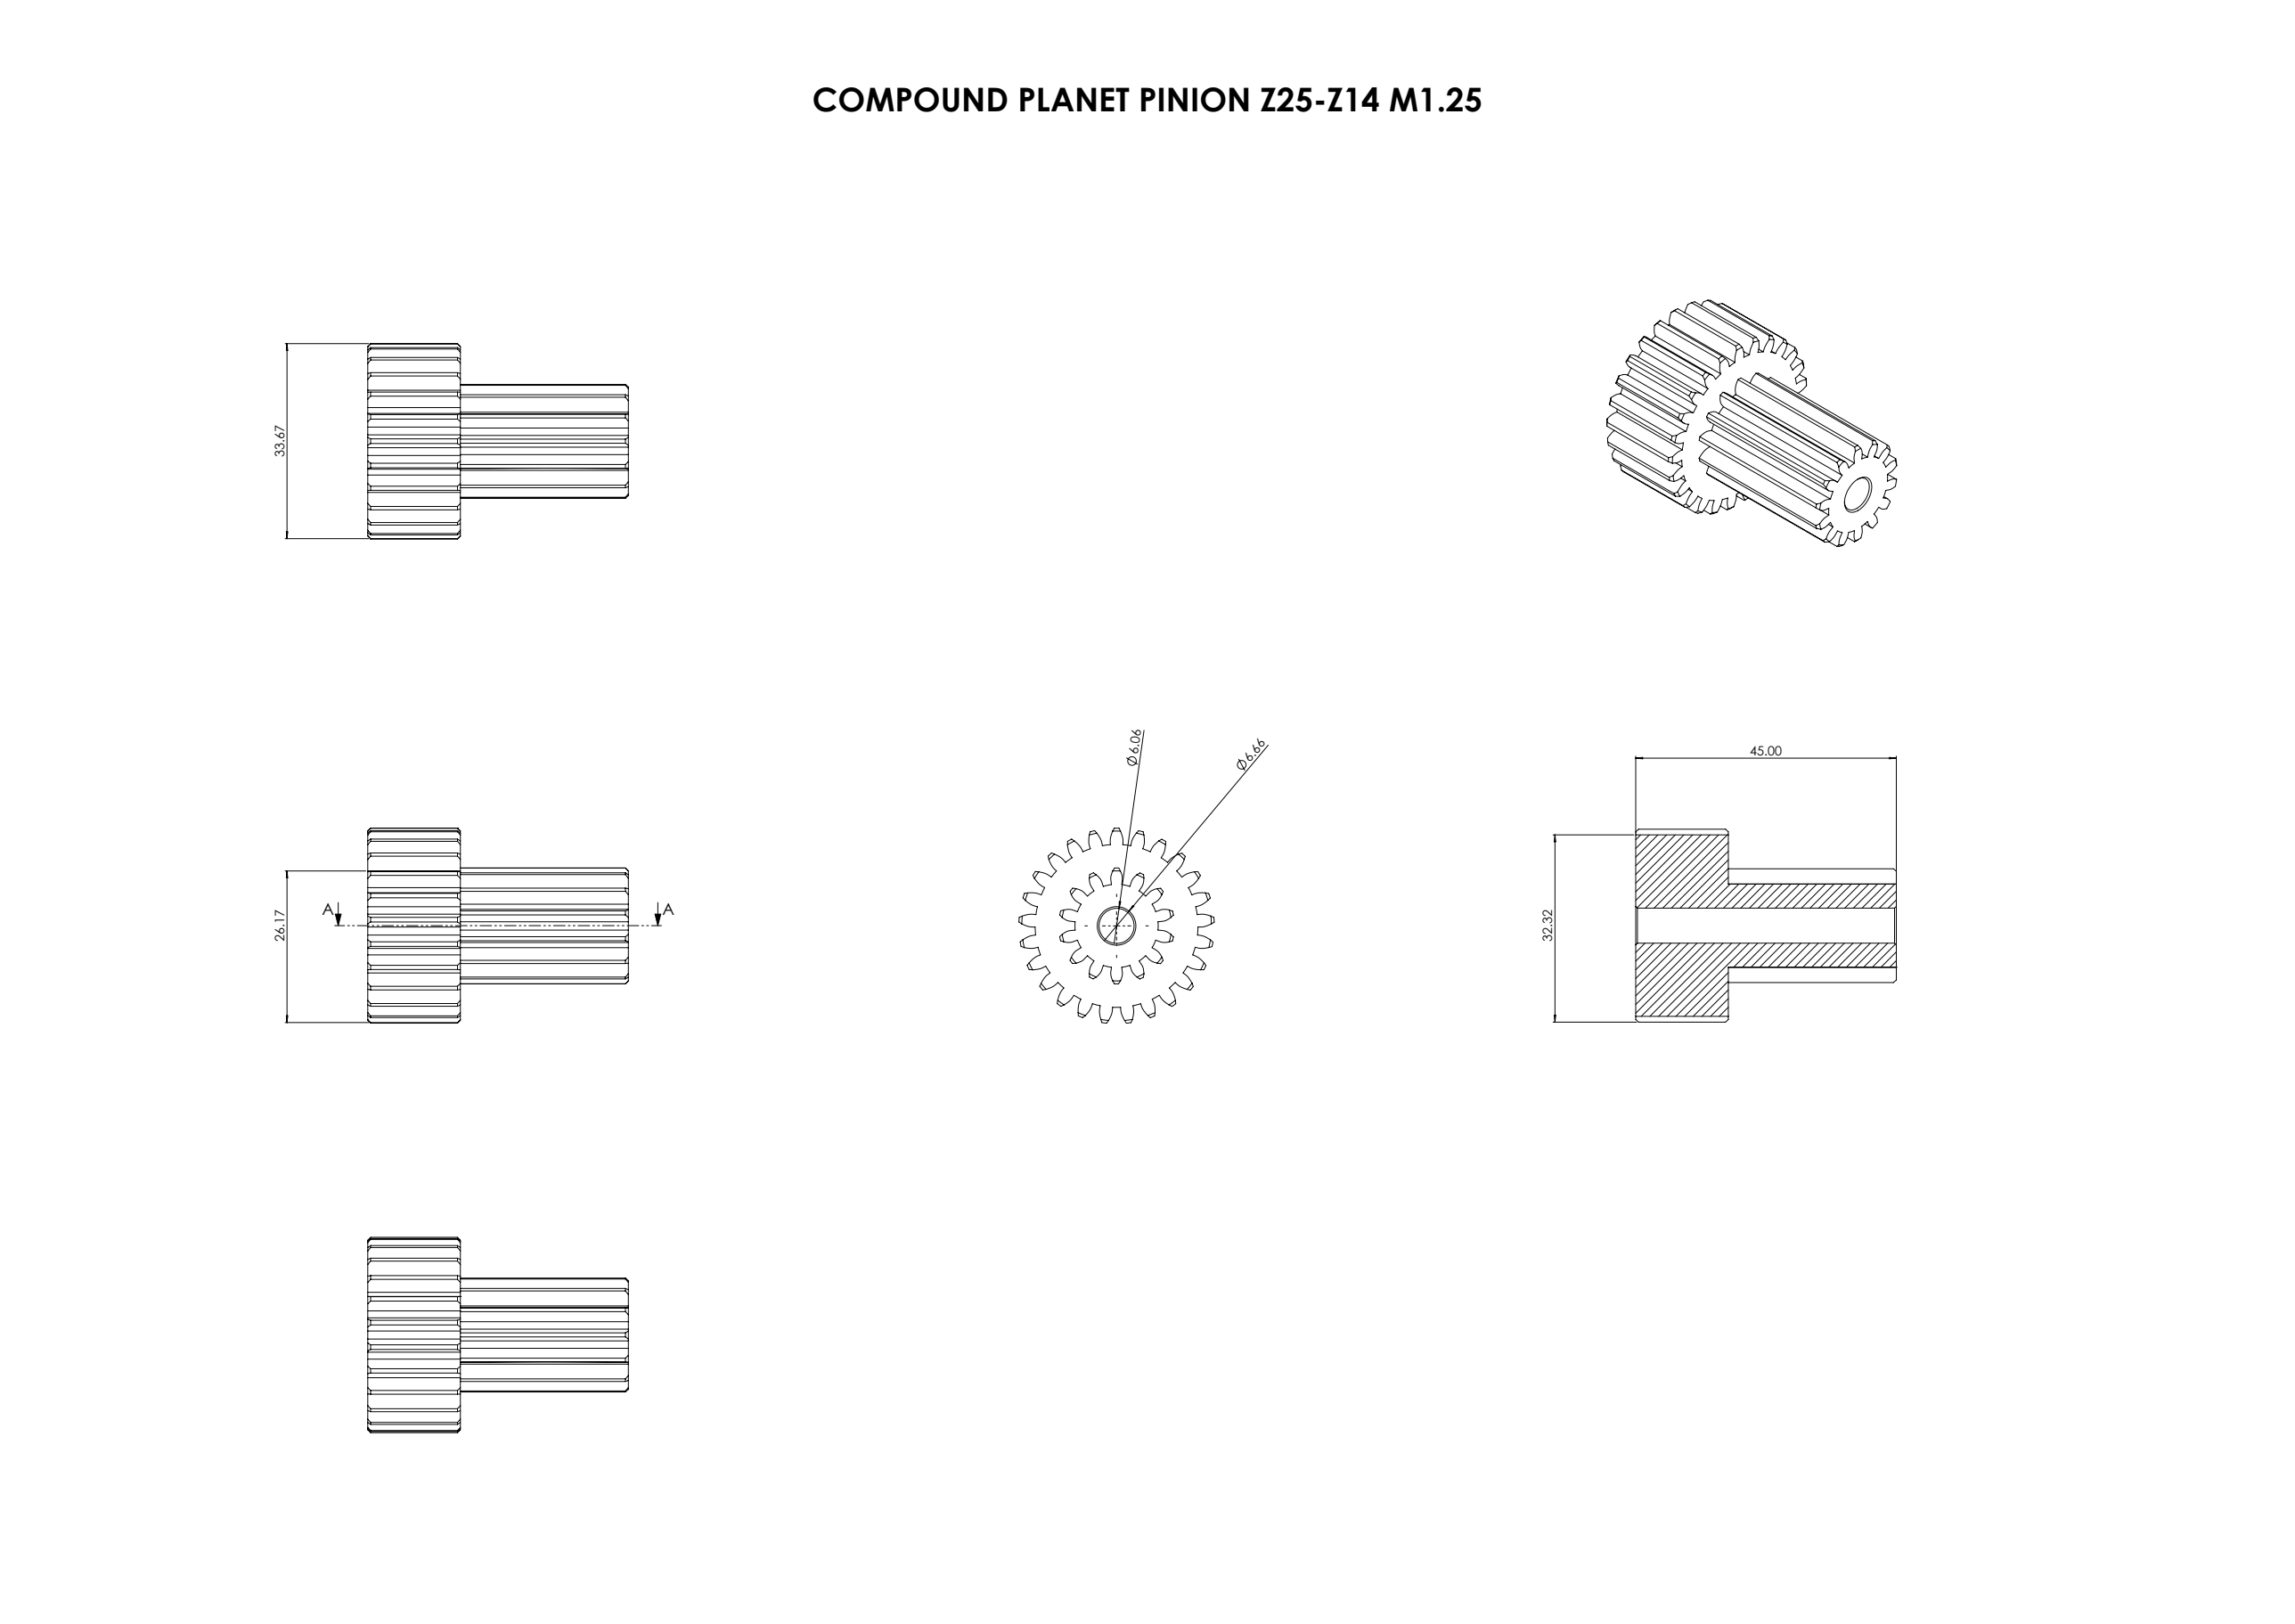
ISO-10303-21;
HEADER;
/* Generated by software containing ST-Developer
 * from STEP Tools, Inc. (www.steptools.com) 
 */

FILE_DESCRIPTION(
/* description */ (''),
/* implementation_level */ '2;1');

FILE_NAME(
/* name */ '03_Compound_Planet_Pinion_Z25-Z14_M1.25.step',
/* time_stamp */ '2026-10-11T13:00:10-07:00',
/* author */ (''),
/* organization */ (''),
/* preprocessor_version */ 'ST-DEVELOPER v20.2',
/* originating_system */ 'Autodesk Translation Framework v15.15.0.0',
/* authorisation */ '');

FILE_SCHEMA (('AUTOMOTIVE_DESIGN { 1 0 10303 214 3 1 1 }'));
ENDSEC;

DATA;
#10=MECHANICAL_DESIGN_GEOMETRIC_PRESENTATION_REPRESENTATION('',(#360),#65563);
#338=SHAPE_REPRESENTATION_RELATIONSHIP('SRR','None',#65616,#349);
#349=ADVANCED_BREP_SHAPE_REPRESENTATION('',(#371),#65554);
#360=STYLED_ITEM('',(#65802),#371);
#371=MANIFOLD_SOLID_BREP('Body1',#20010);
#423=CONICAL_SURFACE('',#21299,3.18,0.785398163397451);
#424=CONICAL_SURFACE('',#21335,3.18,0.785398163397444);
#425=CONICAL_SURFACE('',#21390,9.75,0.785398163397451);
#426=CONICAL_SURFACE('',#21474,9.75,0.785398163397451);
#427=CONICAL_SURFACE('',#21476,9.75,0.785398163397451);
#428=CONICAL_SURFACE('',#21482,9.75,0.785398163397451);
#429=CONICAL_SURFACE('',#21484,9.75,0.785398163397451);
#430=CONICAL_SURFACE('',#21490,9.75,0.785398163397451);
#431=CONICAL_SURFACE('',#21492,9.75,0.785398163397451);
#432=CONICAL_SURFACE('',#21498,9.75,0.785398163397451);
#433=CONICAL_SURFACE('',#21500,9.75,0.785398163397451);
#434=CONICAL_SURFACE('',#21506,9.75,0.785398163397451);
#435=CONICAL_SURFACE('',#21508,9.75,0.785398163397451);
#436=CONICAL_SURFACE('',#21514,9.75,0.785398163397451);
#437=CONICAL_SURFACE('',#21516,9.75,0.785398163397451);
#438=CONICAL_SURFACE('',#21521,16.625,0.785398163397451);
#439=CONICAL_SURFACE('',#21525,16.625,0.785398163397451);
#440=CONICAL_SURFACE('',#21527,16.625,0.785398163397451);
#441=CONICAL_SURFACE('',#21531,16.625,0.785398163397451);
#442=CONICAL_SURFACE('',#21533,16.625,0.785398163397451);
#443=CONICAL_SURFACE('',#21537,16.625,0.785398163397451);
#444=CONICAL_SURFACE('',#21539,16.625,0.785398163397451);
#445=CONICAL_SURFACE('',#21543,16.625,0.785398163397451);
#446=CONICAL_SURFACE('',#21545,16.625,0.785398163397451);
#447=CONICAL_SURFACE('',#21549,16.625,0.785398163397451);
#448=CONICAL_SURFACE('',#21551,16.625,0.785398163397451);
#449=CONICAL_SURFACE('',#21555,16.625,0.785398163397451);
#450=CONICAL_SURFACE('',#21557,16.625,0.785398163397451);
#451=CONICAL_SURFACE('',#21561,16.625,0.785398163397451);
#452=CONICAL_SURFACE('',#21563,16.625,0.785398163397451);
#453=CONICAL_SURFACE('',#21567,16.625,0.785398163397451);
#454=CONICAL_SURFACE('',#21569,16.625,0.785398163397451);
#455=CONICAL_SURFACE('',#21573,16.625,0.785398163397451);
#456=CONICAL_SURFACE('',#21575,16.625,0.785398163397451);
#457=CONICAL_SURFACE('',#21579,16.625,0.785398163397451);
#458=CONICAL_SURFACE('',#21581,16.625,0.785398163397451);
#459=CONICAL_SURFACE('',#21585,16.625,0.785398163397451);
#460=CONICAL_SURFACE('',#21587,16.625,0.785398163397451);
#461=CONICAL_SURFACE('',#21591,16.625,0.785398163397451);
#462=CONICAL_SURFACE('',#21593,16.625,0.785398163397451);
#463=CONICAL_SURFACE('',#21597,16.625,0.785398163397451);
#464=CONICAL_SURFACE('',#21599,16.625,0.785398163397451);
#465=CONICAL_SURFACE('',#21603,16.625,0.785398163397451);
#466=CONICAL_SURFACE('',#21605,16.625,0.785398163397451);
#467=CONICAL_SURFACE('',#21609,16.625,0.785398163397451);
#468=CONICAL_SURFACE('',#21611,16.625,0.785398163397451);
#469=CONICAL_SURFACE('',#21615,16.625,0.785398163397451);
#470=CONICAL_SURFACE('',#21617,16.625,0.785398163397451);
#471=CONICAL_SURFACE('',#21621,16.625,0.785398163397451);
#472=CONICAL_SURFACE('',#21623,16.625,0.785398163397451);
#473=CONICAL_SURFACE('',#21627,16.625,0.785398163397451);
#474=CONICAL_SURFACE('',#21629,16.625,0.785398163397451);
#475=CONICAL_SURFACE('',#21633,16.625,0.785398163397451);
#476=CONICAL_SURFACE('',#21635,16.625,0.785398163397451);
#477=CONICAL_SURFACE('',#21639,16.625,0.785398163397451);
#478=CONICAL_SURFACE('',#21641,16.625,0.785398163397451);
#479=CONICAL_SURFACE('',#21645,16.625,0.785398163397451);
#480=CONICAL_SURFACE('',#21647,16.625,0.785398163397451);
#481=CONICAL_SURFACE('',#21651,16.625,0.785398163397451);
#482=CONICAL_SURFACE('',#21653,16.625,0.785398163397451);
#483=CONICAL_SURFACE('',#21657,16.625,0.785398163397451);
#484=CONICAL_SURFACE('',#21659,16.625,0.785398163397451);
#485=CONICAL_SURFACE('',#21663,16.625,0.785398163397451);
#486=CONICAL_SURFACE('',#21665,16.625,0.785398163397451);
#487=CONICAL_SURFACE('',#21669,16.625,0.785398163397451);
#488=CONICAL_SURFACE('',#21672,9.75,0.785398163397451);
#530=(
BOUNDED_SURFACE()
B_SPLINE_SURFACE(5,1,((#51613,#51614),(#51615,#51616),(#51617,#51618),(#51619,
#51620),(#51621,#51622),(#51623,#51624),(#51625,#51626),(#51627,#51628),
(#51629,#51630),(#51631,#51632),(#51633,#51634),(#51635,#51636),(#51637,
#51638),(#51639,#51640),(#51641,#51642),(#51643,#51644),(#51645,#51646),
(#51647,#51648),(#51649,#51650),(#51651,#51652),(#51653,#51654),(#51655,
#51656),(#51657,#51658),(#51659,#51660),(#51661,#51662),(#51663,#51664),
(#51665,#51666),(#51667,#51668),(#51669,#51670),(#51671,#51672),(#51673,
#51674),(#51675,#51676),(#51677,#51678),(#51679,#51680),(#51681,#51682),
(#51683,#51684),(#51685,#51686),(#51687,#51688),(#51689,#51690),(#51691,
#51692)),.UNSPECIFIED.,.F.,.F.,.F.)
B_SPLINE_SURFACE_WITH_KNOTS((6,1,1,1,1,1,1,1,1,1,1,1,1,1,1,1,1,1,1,1,1,
1,1,1,1,1,1,1,1,1,1,1,1,1,1,6),(2,2),(-1.,-0.971428571428572,-0.942857142857143,
-0.914285714285714,-0.885714285714286,-0.857142857142857,-0.828571428571429,
-0.8,-0.771428571428572,-0.742857142857143,-0.714285714285714,-0.685714285714286,
-0.657142857142857,-0.628571428571429,-0.6,-0.571428571428572,-0.542857142857143,
-0.514285714285714,-0.485714285714286,-0.457142857142857,-0.428571428571429,
-0.4,-0.371428571428571,-0.342857142857143,-0.314285714285714,-0.285714285714286,
-0.257142857142857,-0.228571428571429,-0.2,-0.171428571428571,-0.142857142857143,
-0.114285714285714,-0.0857142857142857,-0.0571428571428571,-0.0285714285714286,
0.),(0.,2.9),.UNSPECIFIED.)
GEOMETRIC_REPRESENTATION_ITEM()
RATIONAL_B_SPLINE_SURFACE(((1.,1.),(1.,1.),(1.,1.),(1.,1.),(1.,1.),(1.,
1.),(1.,1.),(1.,1.),(1.,1.),(1.,1.),(1.,1.),(1.,1.),(1.,1.),(1.,1.),(1.,
1.),(1.,1.),(1.,1.),(1.,1.),(1.,1.),(1.,1.),(1.,1.),(1.,1.),(1.,1.),(1.,
1.),(1.,1.),(1.,1.),(1.,1.),(1.,1.),(1.,1.),(1.,1.),(1.,1.),(1.,1.),(1.,
1.),(1.,1.),(1.,1.),(1.,1.),(1.,1.),(1.,1.),(1.,1.),(1.,1.)))
REPRESENTATION_ITEM('')
SURFACE()
);
#531=(
BOUNDED_SURFACE()
B_SPLINE_SURFACE(5,1,((#51748,#51749),(#51750,#51751),(#51752,#51753),(#51754,
#51755),(#51756,#51757),(#51758,#51759),(#51760,#51761),(#51762,#51763),
(#51764,#51765),(#51766,#51767),(#51768,#51769),(#51770,#51771),(#51772,
#51773),(#51774,#51775),(#51776,#51777),(#51778,#51779),(#51780,#51781),
(#51782,#51783),(#51784,#51785),(#51786,#51787),(#51788,#51789),(#51790,
#51791),(#51792,#51793),(#51794,#51795),(#51796,#51797),(#51798,#51799),
(#51800,#51801),(#51802,#51803),(#51804,#51805),(#51806,#51807),(#51808,
#51809),(#51810,#51811),(#51812,#51813),(#51814,#51815),(#51816,#51817),
(#51818,#51819),(#51820,#51821),(#51822,#51823),(#51824,#51825),(#51826,
#51827)),.UNSPECIFIED.,.F.,.F.,.F.)
B_SPLINE_SURFACE_WITH_KNOTS((6,1,1,1,1,1,1,1,1,1,1,1,1,1,1,1,1,1,1,1,1,
1,1,1,1,1,1,1,1,1,1,1,1,1,1,6),(2,2),(-1.,-0.971428571428572,-0.942857142857143,
-0.914285714285714,-0.885714285714286,-0.857142857142857,-0.828571428571429,
-0.8,-0.771428571428572,-0.742857142857143,-0.714285714285714,-0.685714285714286,
-0.657142857142857,-0.628571428571429,-0.6,-0.571428571428572,-0.542857142857143,
-0.514285714285714,-0.485714285714286,-0.457142857142857,-0.428571428571429,
-0.4,-0.371428571428571,-0.342857142857143,-0.314285714285714,-0.285714285714286,
-0.257142857142857,-0.228571428571429,-0.2,-0.171428571428571,-0.142857142857143,
-0.114285714285714,-0.0857142857142857,-0.0571428571428571,-0.0285714285714286,
0.),(0.,2.9),.UNSPECIFIED.)
GEOMETRIC_REPRESENTATION_ITEM()
RATIONAL_B_SPLINE_SURFACE(((1.,1.),(1.,1.),(1.,1.),(1.,1.),(1.,1.),(1.,
1.),(1.,1.),(1.,1.),(1.,1.),(1.,1.),(1.,1.),(1.,1.),(1.,1.),(1.,1.),(1.,
1.),(1.,1.),(1.,1.),(1.,1.),(1.,1.),(1.,1.),(1.,1.),(1.,1.),(1.,1.),(1.,
1.),(1.,1.),(1.,1.),(1.,1.),(1.,1.),(1.,1.),(1.,1.),(1.,1.),(1.,1.),(1.,
1.),(1.,1.),(1.,1.),(1.,1.),(1.,1.),(1.,1.),(1.,1.),(1.,1.)))
REPRESENTATION_ITEM('')
SURFACE()
);
#532=(
BOUNDED_SURFACE()
B_SPLINE_SURFACE(5,1,((#51889,#51890),(#51891,#51892),(#51893,#51894),(#51895,
#51896),(#51897,#51898),(#51899,#51900),(#51901,#51902),(#51903,#51904),
(#51905,#51906),(#51907,#51908),(#51909,#51910),(#51911,#51912),(#51913,
#51914),(#51915,#51916),(#51917,#51918),(#51919,#51920),(#51921,#51922),
(#51923,#51924),(#51925,#51926),(#51927,#51928),(#51929,#51930),(#51931,
#51932),(#51933,#51934),(#51935,#51936),(#51937,#51938),(#51939,#51940),
(#51941,#51942),(#51943,#51944),(#51945,#51946),(#51947,#51948),(#51949,
#51950),(#51951,#51952),(#51953,#51954),(#51955,#51956),(#51957,#51958),
(#51959,#51960),(#51961,#51962),(#51963,#51964),(#51965,#51966),(#51967,
#51968)),.UNSPECIFIED.,.F.,.F.,.F.)
B_SPLINE_SURFACE_WITH_KNOTS((6,1,1,1,1,1,1,1,1,1,1,1,1,1,1,1,1,1,1,1,1,
1,1,1,1,1,1,1,1,1,1,1,1,1,1,6),(2,2),(-1.,-0.971428571428572,-0.942857142857143,
-0.914285714285714,-0.885714285714286,-0.857142857142857,-0.828571428571429,
-0.8,-0.771428571428572,-0.742857142857143,-0.714285714285714,-0.685714285714286,
-0.657142857142857,-0.628571428571429,-0.6,-0.571428571428572,-0.542857142857143,
-0.514285714285714,-0.485714285714286,-0.457142857142857,-0.428571428571429,
-0.4,-0.371428571428571,-0.342857142857143,-0.314285714285714,-0.285714285714286,
-0.257142857142857,-0.228571428571429,-0.2,-0.171428571428571,-0.142857142857143,
-0.114285714285714,-0.0857142857142857,-0.0571428571428571,-0.0285714285714286,
0.),(0.,2.9),.UNSPECIFIED.)
GEOMETRIC_REPRESENTATION_ITEM()
RATIONAL_B_SPLINE_SURFACE(((1.,1.),(1.,1.),(1.,1.),(1.,1.),(1.,1.),(1.,
1.),(1.,1.),(1.,1.),(1.,1.),(1.,1.),(1.,1.),(1.,1.),(1.,1.),(1.,1.),(1.,
1.),(1.,1.),(1.,1.),(1.,1.),(1.,1.),(1.,1.),(1.,1.),(1.,1.),(1.,1.),(1.,
1.),(1.,1.),(1.,1.),(1.,1.),(1.,1.),(1.,1.),(1.,1.),(1.,1.),(1.,1.),(1.,
1.),(1.,1.),(1.,1.),(1.,1.),(1.,1.),(1.,1.),(1.,1.),(1.,1.)))
REPRESENTATION_ITEM('')
SURFACE()
);
#533=(
BOUNDED_SURFACE()
B_SPLINE_SURFACE(5,1,((#52018,#52019),(#52020,#52021),(#52022,#52023),(#52024,
#52025),(#52026,#52027),(#52028,#52029),(#52030,#52031),(#52032,#52033),
(#52034,#52035),(#52036,#52037),(#52038,#52039),(#52040,#52041),(#52042,
#52043),(#52044,#52045),(#52046,#52047),(#52048,#52049),(#52050,#52051),
(#52052,#52053),(#52054,#52055),(#52056,#52057),(#52058,#52059),(#52060,
#52061),(#52062,#52063),(#52064,#52065),(#52066,#52067),(#52068,#52069),
(#52070,#52071),(#52072,#52073),(#52074,#52075),(#52076,#52077),(#52078,
#52079),(#52080,#52081),(#52082,#52083),(#52084,#52085),(#52086,#52087),
(#52088,#52089),(#52090,#52091),(#52092,#52093),(#52094,#52095),(#52096,
#52097)),.UNSPECIFIED.,.F.,.F.,.F.)
B_SPLINE_SURFACE_WITH_KNOTS((6,1,1,1,1,1,1,1,1,1,1,1,1,1,1,1,1,1,1,1,1,
1,1,1,1,1,1,1,1,1,1,1,1,1,1,6),(2,2),(-1.,-0.971428571428572,-0.942857142857143,
-0.914285714285714,-0.885714285714286,-0.857142857142857,-0.828571428571429,
-0.8,-0.771428571428572,-0.742857142857143,-0.714285714285714,-0.685714285714286,
-0.657142857142857,-0.628571428571429,-0.6,-0.571428571428572,-0.542857142857143,
-0.514285714285714,-0.485714285714286,-0.457142857142857,-0.428571428571429,
-0.4,-0.371428571428571,-0.342857142857143,-0.314285714285714,-0.285714285714286,
-0.257142857142857,-0.228571428571429,-0.2,-0.171428571428571,-0.142857142857143,
-0.114285714285714,-0.0857142857142857,-0.0571428571428571,-0.0285714285714286,
0.),(0.,2.9),.UNSPECIFIED.)
GEOMETRIC_REPRESENTATION_ITEM()
RATIONAL_B_SPLINE_SURFACE(((1.,1.),(1.,1.),(1.,1.),(1.,1.),(1.,1.),(1.,
1.),(1.,1.),(1.,1.),(1.,1.),(1.,1.),(1.,1.),(1.,1.),(1.,1.),(1.,1.),(1.,
1.),(1.,1.),(1.,1.),(1.,1.),(1.,1.),(1.,1.),(1.,1.),(1.,1.),(1.,1.),(1.,
1.),(1.,1.),(1.,1.),(1.,1.),(1.,1.),(1.,1.),(1.,1.),(1.,1.),(1.,1.),(1.,
1.),(1.,1.),(1.,1.),(1.,1.),(1.,1.),(1.,1.),(1.,1.),(1.,1.)))
REPRESENTATION_ITEM('')
SURFACE()
);
#534=(
BOUNDED_SURFACE()
B_SPLINE_SURFACE(5,1,((#54512,#54513),(#54514,#54515),(#54516,#54517),(#54518,
#54519),(#54520,#54521),(#54522,#54523),(#54524,#54525),(#54526,#54527),
(#54528,#54529),(#54530,#54531),(#54532,#54533),(#54534,#54535),(#54536,
#54537),(#54538,#54539),(#54540,#54541),(#54542,#54543),(#54544,#54545),
(#54546,#54547),(#54548,#54549),(#54550,#54551),(#54552,#54553),(#54554,
#54555),(#54556,#54557),(#54558,#54559),(#54560,#54561),(#54562,#54563),
(#54564,#54565),(#54566,#54567),(#54568,#54569),(#54570,#54571),(#54572,
#54573),(#54574,#54575),(#54576,#54577),(#54578,#54579),(#54580,#54581),
(#54582,#54583),(#54584,#54585),(#54586,#54587),(#54588,#54589),(#54590,
#54591)),.UNSPECIFIED.,.F.,.F.,.F.)
B_SPLINE_SURFACE_WITH_KNOTS((6,1,1,1,1,1,1,1,1,1,1,1,1,1,1,1,1,1,1,1,1,
1,1,1,1,1,1,1,1,1,1,1,1,1,1,6),(2,2),(-1.,-0.971428571428572,-0.942857142857143,
-0.914285714285714,-0.885714285714286,-0.857142857142857,-0.828571428571429,
-0.8,-0.771428571428572,-0.742857142857143,-0.714285714285714,-0.685714285714286,
-0.657142857142857,-0.628571428571429,-0.6,-0.571428571428572,-0.542857142857143,
-0.514285714285714,-0.485714285714286,-0.457142857142857,-0.428571428571429,
-0.4,-0.371428571428571,-0.342857142857143,-0.314285714285714,-0.285714285714286,
-0.257142857142857,-0.228571428571429,-0.2,-0.171428571428571,-0.142857142857143,
-0.114285714285714,-0.0857142857142857,-0.0571428571428571,-0.0285714285714286,
0.),(0.,2.9),.UNSPECIFIED.)
GEOMETRIC_REPRESENTATION_ITEM()
RATIONAL_B_SPLINE_SURFACE(((1.,1.),(1.,1.),(1.,1.),(1.,1.),(1.,1.),(1.,
1.),(1.,1.),(1.,1.),(1.,1.),(1.,1.),(1.,1.),(1.,1.),(1.,1.),(1.,1.),(1.,
1.),(1.,1.),(1.,1.),(1.,1.),(1.,1.),(1.,1.),(1.,1.),(1.,1.),(1.,1.),(1.,
1.),(1.,1.),(1.,1.),(1.,1.),(1.,1.),(1.,1.),(1.,1.),(1.,1.),(1.,1.),(1.,
1.),(1.,1.),(1.,1.),(1.,1.),(1.,1.),(1.,1.),(1.,1.),(1.,1.)))
REPRESENTATION_ITEM('')
SURFACE()
);
#535=(
BOUNDED_SURFACE()
B_SPLINE_SURFACE(5,1,((#54595,#54596),(#54597,#54598),(#54599,#54600),(#54601,
#54602),(#54603,#54604),(#54605,#54606),(#54607,#54608),(#54609,#54610),
(#54611,#54612),(#54613,#54614),(#54615,#54616),(#54617,#54618),(#54619,
#54620),(#54621,#54622),(#54623,#54624),(#54625,#54626),(#54627,#54628),
(#54629,#54630),(#54631,#54632),(#54633,#54634),(#54635,#54636),(#54637,
#54638),(#54639,#54640),(#54641,#54642),(#54643,#54644),(#54645,#54646),
(#54647,#54648),(#54649,#54650),(#54651,#54652),(#54653,#54654),(#54655,
#54656),(#54657,#54658),(#54659,#54660),(#54661,#54662),(#54663,#54664),
(#54665,#54666),(#54667,#54668),(#54669,#54670),(#54671,#54672),(#54673,
#54674)),.UNSPECIFIED.,.F.,.F.,.F.)
B_SPLINE_SURFACE_WITH_KNOTS((6,1,1,1,1,1,1,1,1,1,1,1,1,1,1,1,1,1,1,1,1,
1,1,1,1,1,1,1,1,1,1,1,1,1,1,6),(2,2),(-1.,-0.971428571428572,-0.942857142857143,
-0.914285714285714,-0.885714285714286,-0.857142857142857,-0.828571428571429,
-0.8,-0.771428571428572,-0.742857142857143,-0.714285714285714,-0.685714285714286,
-0.657142857142857,-0.628571428571429,-0.6,-0.571428571428572,-0.542857142857143,
-0.514285714285714,-0.485714285714286,-0.457142857142857,-0.428571428571429,
-0.4,-0.371428571428571,-0.342857142857143,-0.314285714285714,-0.285714285714286,
-0.257142857142857,-0.228571428571429,-0.2,-0.171428571428571,-0.142857142857143,
-0.114285714285714,-0.0857142857142857,-0.0571428571428571,-0.0285714285714286,
0.),(0.,2.9),.UNSPECIFIED.)
GEOMETRIC_REPRESENTATION_ITEM()
RATIONAL_B_SPLINE_SURFACE(((1.,1.),(1.,1.),(1.,1.),(1.,1.),(1.,1.),(1.,
1.),(1.,1.),(1.,1.),(1.,1.),(1.,1.),(1.,1.),(1.,1.),(1.,1.),(1.,1.),(1.,
1.),(1.,1.),(1.,1.),(1.,1.),(1.,1.),(1.,1.),(1.,1.),(1.,1.),(1.,1.),(1.,
1.),(1.,1.),(1.,1.),(1.,1.),(1.,1.),(1.,1.),(1.,1.),(1.,1.),(1.,1.),(1.,
1.),(1.,1.),(1.,1.),(1.,1.),(1.,1.),(1.,1.),(1.,1.),(1.,1.)))
REPRESENTATION_ITEM('')
SURFACE()
);
#536=(
BOUNDED_SURFACE()
B_SPLINE_SURFACE(5,1,((#54691,#54692),(#54693,#54694),(#54695,#54696),(#54697,
#54698),(#54699,#54700),(#54701,#54702),(#54703,#54704),(#54705,#54706),
(#54707,#54708),(#54709,#54710),(#54711,#54712),(#54713,#54714),(#54715,
#54716),(#54717,#54718),(#54719,#54720),(#54721,#54722),(#54723,#54724),
(#54725,#54726),(#54727,#54728),(#54729,#54730),(#54731,#54732),(#54733,
#54734),(#54735,#54736),(#54737,#54738),(#54739,#54740),(#54741,#54742),
(#54743,#54744),(#54745,#54746),(#54747,#54748),(#54749,#54750),(#54751,
#54752),(#54753,#54754),(#54755,#54756),(#54757,#54758),(#54759,#54760),
(#54761,#54762),(#54763,#54764),(#54765,#54766),(#54767,#54768),(#54769,
#54770)),.UNSPECIFIED.,.F.,.F.,.F.)
B_SPLINE_SURFACE_WITH_KNOTS((6,1,1,1,1,1,1,1,1,1,1,1,1,1,1,1,1,1,1,1,1,
1,1,1,1,1,1,1,1,1,1,1,1,1,1,6),(2,2),(-1.,-0.971428571428572,-0.942857142857143,
-0.914285714285714,-0.885714285714286,-0.857142857142857,-0.828571428571429,
-0.8,-0.771428571428572,-0.742857142857143,-0.714285714285714,-0.685714285714286,
-0.657142857142857,-0.628571428571429,-0.6,-0.571428571428572,-0.542857142857143,
-0.514285714285714,-0.485714285714286,-0.457142857142857,-0.428571428571429,
-0.4,-0.371428571428571,-0.342857142857143,-0.314285714285714,-0.285714285714286,
-0.257142857142857,-0.228571428571429,-0.2,-0.171428571428571,-0.142857142857143,
-0.114285714285714,-0.0857142857142857,-0.0571428571428571,-0.0285714285714286,
0.),(0.,2.9),.UNSPECIFIED.)
GEOMETRIC_REPRESENTATION_ITEM()
RATIONAL_B_SPLINE_SURFACE(((1.,1.),(1.,1.),(1.,1.),(1.,1.),(1.,1.),(1.,
1.),(1.,1.),(1.,1.),(1.,1.),(1.,1.),(1.,1.),(1.,1.),(1.,1.),(1.,1.),(1.,
1.),(1.,1.),(1.,1.),(1.,1.),(1.,1.),(1.,1.),(1.,1.),(1.,1.),(1.,1.),(1.,
1.),(1.,1.),(1.,1.),(1.,1.),(1.,1.),(1.,1.),(1.,1.),(1.,1.),(1.,1.),(1.,
1.),(1.,1.),(1.,1.),(1.,1.),(1.,1.),(1.,1.),(1.,1.),(1.,1.)))
REPRESENTATION_ITEM('')
SURFACE()
);
#537=(
BOUNDED_SURFACE()
B_SPLINE_SURFACE(5,1,((#54787,#54788),(#54789,#54790),(#54791,#54792),(#54793,
#54794),(#54795,#54796),(#54797,#54798),(#54799,#54800),(#54801,#54802),
(#54803,#54804),(#54805,#54806),(#54807,#54808),(#54809,#54810),(#54811,
#54812),(#54813,#54814),(#54815,#54816),(#54817,#54818),(#54819,#54820),
(#54821,#54822),(#54823,#54824),(#54825,#54826),(#54827,#54828),(#54829,
#54830),(#54831,#54832),(#54833,#54834),(#54835,#54836),(#54837,#54838),
(#54839,#54840),(#54841,#54842),(#54843,#54844),(#54845,#54846),(#54847,
#54848),(#54849,#54850),(#54851,#54852),(#54853,#54854),(#54855,#54856),
(#54857,#54858),(#54859,#54860),(#54861,#54862),(#54863,#54864),(#54865,
#54866)),.UNSPECIFIED.,.F.,.F.,.F.)
B_SPLINE_SURFACE_WITH_KNOTS((6,1,1,1,1,1,1,1,1,1,1,1,1,1,1,1,1,1,1,1,1,
1,1,1,1,1,1,1,1,1,1,1,1,1,1,6),(2,2),(-1.,-0.971428571428572,-0.942857142857143,
-0.914285714285714,-0.885714285714286,-0.857142857142857,-0.828571428571429,
-0.8,-0.771428571428572,-0.742857142857143,-0.714285714285714,-0.685714285714286,
-0.657142857142857,-0.628571428571429,-0.6,-0.571428571428572,-0.542857142857143,
-0.514285714285714,-0.485714285714286,-0.457142857142857,-0.428571428571429,
-0.4,-0.371428571428571,-0.342857142857143,-0.314285714285714,-0.285714285714286,
-0.257142857142857,-0.228571428571429,-0.2,-0.171428571428571,-0.142857142857143,
-0.114285714285714,-0.0857142857142857,-0.0571428571428571,-0.0285714285714286,
0.),(0.,2.9),.UNSPECIFIED.)
GEOMETRIC_REPRESENTATION_ITEM()
RATIONAL_B_SPLINE_SURFACE(((1.,1.),(1.,1.),(1.,1.),(1.,1.),(1.,1.),(1.,
1.),(1.,1.),(1.,1.),(1.,1.),(1.,1.),(1.,1.),(1.,1.),(1.,1.),(1.,1.),(1.,
1.),(1.,1.),(1.,1.),(1.,1.),(1.,1.),(1.,1.),(1.,1.),(1.,1.),(1.,1.),(1.,
1.),(1.,1.),(1.,1.),(1.,1.),(1.,1.),(1.,1.),(1.,1.),(1.,1.),(1.,1.),(1.,
1.),(1.,1.),(1.,1.),(1.,1.),(1.,1.),(1.,1.),(1.,1.),(1.,1.)))
REPRESENTATION_ITEM('')
SURFACE()
);
#538=(
BOUNDED_SURFACE()
B_SPLINE_SURFACE(5,1,((#54898,#54899),(#54900,#54901),(#54902,#54903),(#54904,
#54905),(#54906,#54907),(#54908,#54909),(#54910,#54911),(#54912,#54913),
(#54914,#54915),(#54916,#54917),(#54918,#54919),(#54920,#54921),(#54922,
#54923),(#54924,#54925),(#54926,#54927),(#54928,#54929),(#54930,#54931),
(#54932,#54933),(#54934,#54935),(#54936,#54937),(#54938,#54939),(#54940,
#54941),(#54942,#54943),(#54944,#54945),(#54946,#54947),(#54948,#54949),
(#54950,#54951),(#54952,#54953),(#54954,#54955),(#54956,#54957),(#54958,
#54959),(#54960,#54961),(#54962,#54963),(#54964,#54965),(#54966,#54967),
(#54968,#54969),(#54970,#54971),(#54972,#54973),(#54974,#54975),(#54976,
#54977)),.UNSPECIFIED.,.F.,.F.,.F.)
B_SPLINE_SURFACE_WITH_KNOTS((6,1,1,1,1,1,1,1,1,1,1,1,1,1,1,1,1,1,1,1,1,
1,1,1,1,1,1,1,1,1,1,1,1,1,1,6),(2,2),(-1.,-0.971428571428572,-0.942857142857143,
-0.914285714285714,-0.885714285714286,-0.857142857142857,-0.828571428571429,
-0.8,-0.771428571428572,-0.742857142857143,-0.714285714285714,-0.685714285714286,
-0.657142857142857,-0.628571428571429,-0.6,-0.571428571428572,-0.542857142857143,
-0.514285714285714,-0.485714285714286,-0.457142857142857,-0.428571428571429,
-0.4,-0.371428571428571,-0.342857142857143,-0.314285714285714,-0.285714285714286,
-0.257142857142857,-0.228571428571429,-0.2,-0.171428571428571,-0.142857142857143,
-0.114285714285714,-0.0857142857142857,-0.0571428571428571,-0.0285714285714286,
0.),(0.,2.9),.UNSPECIFIED.)
GEOMETRIC_REPRESENTATION_ITEM()
RATIONAL_B_SPLINE_SURFACE(((1.,1.),(1.,1.),(1.,1.),(1.,1.),(1.,1.),(1.,
1.),(1.,1.),(1.,1.),(1.,1.),(1.,1.),(1.,1.),(1.,1.),(1.,1.),(1.,1.),(1.,
1.),(1.,1.),(1.,1.),(1.,1.),(1.,1.),(1.,1.),(1.,1.),(1.,1.),(1.,1.),(1.,
1.),(1.,1.),(1.,1.),(1.,1.),(1.,1.),(1.,1.),(1.,1.),(1.,1.),(1.,1.),(1.,
1.),(1.,1.),(1.,1.),(1.,1.),(1.,1.),(1.,1.),(1.,1.),(1.,1.)))
REPRESENTATION_ITEM('')
SURFACE()
);
#539=(
BOUNDED_SURFACE()
B_SPLINE_SURFACE(5,1,((#54981,#54982),(#54983,#54984),(#54985,#54986),(#54987,
#54988),(#54989,#54990),(#54991,#54992),(#54993,#54994),(#54995,#54996),
(#54997,#54998),(#54999,#55000),(#55001,#55002),(#55003,#55004),(#55005,
#55006),(#55007,#55008),(#55009,#55010),(#55011,#55012),(#55013,#55014),
(#55015,#55016),(#55017,#55018),(#55019,#55020),(#55021,#55022),(#55023,
#55024),(#55025,#55026),(#55027,#55028),(#55029,#55030),(#55031,#55032),
(#55033,#55034),(#55035,#55036),(#55037,#55038),(#55039,#55040),(#55041,
#55042),(#55043,#55044),(#55045,#55046),(#55047,#55048),(#55049,#55050),
(#55051,#55052),(#55053,#55054),(#55055,#55056),(#55057,#55058),(#55059,
#55060)),.UNSPECIFIED.,.F.,.F.,.F.)
B_SPLINE_SURFACE_WITH_KNOTS((6,1,1,1,1,1,1,1,1,1,1,1,1,1,1,1,1,1,1,1,1,
1,1,1,1,1,1,1,1,1,1,1,1,1,1,6),(2,2),(-1.,-0.971428571428572,-0.942857142857143,
-0.914285714285714,-0.885714285714286,-0.857142857142857,-0.828571428571429,
-0.8,-0.771428571428572,-0.742857142857143,-0.714285714285714,-0.685714285714286,
-0.657142857142857,-0.628571428571429,-0.6,-0.571428571428572,-0.542857142857143,
-0.514285714285714,-0.485714285714286,-0.457142857142857,-0.428571428571429,
-0.4,-0.371428571428571,-0.342857142857143,-0.314285714285714,-0.285714285714286,
-0.257142857142857,-0.228571428571429,-0.2,-0.171428571428571,-0.142857142857143,
-0.114285714285714,-0.0857142857142857,-0.0571428571428571,-0.0285714285714286,
0.),(0.,2.9),.UNSPECIFIED.)
GEOMETRIC_REPRESENTATION_ITEM()
RATIONAL_B_SPLINE_SURFACE(((1.,1.),(1.,1.),(1.,1.),(1.,1.),(1.,1.),(1.,
1.),(1.,1.),(1.,1.),(1.,1.),(1.,1.),(1.,1.),(1.,1.),(1.,1.),(1.,1.),(1.,
1.),(1.,1.),(1.,1.),(1.,1.),(1.,1.),(1.,1.),(1.,1.),(1.,1.),(1.,1.),(1.,
1.),(1.,1.),(1.,1.),(1.,1.),(1.,1.),(1.,1.),(1.,1.),(1.,1.),(1.,1.),(1.,
1.),(1.,1.),(1.,1.),(1.,1.),(1.,1.),(1.,1.),(1.,1.),(1.,1.)))
REPRESENTATION_ITEM('')
SURFACE()
);
#540=(
BOUNDED_SURFACE()
B_SPLINE_SURFACE(5,1,((#55077,#55078),(#55079,#55080),(#55081,#55082),(#55083,
#55084),(#55085,#55086),(#55087,#55088),(#55089,#55090),(#55091,#55092),
(#55093,#55094),(#55095,#55096),(#55097,#55098),(#55099,#55100),(#55101,
#55102),(#55103,#55104),(#55105,#55106),(#55107,#55108),(#55109,#55110),
(#55111,#55112),(#55113,#55114),(#55115,#55116),(#55117,#55118),(#55119,
#55120),(#55121,#55122),(#55123,#55124),(#55125,#55126),(#55127,#55128),
(#55129,#55130),(#55131,#55132),(#55133,#55134),(#55135,#55136),(#55137,
#55138),(#55139,#55140),(#55141,#55142),(#55143,#55144),(#55145,#55146),
(#55147,#55148),(#55149,#55150),(#55151,#55152),(#55153,#55154),(#55155,
#55156)),.UNSPECIFIED.,.F.,.F.,.F.)
B_SPLINE_SURFACE_WITH_KNOTS((6,1,1,1,1,1,1,1,1,1,1,1,1,1,1,1,1,1,1,1,1,
1,1,1,1,1,1,1,1,1,1,1,1,1,1,6),(2,2),(-1.,-0.971428571428572,-0.942857142857143,
-0.914285714285714,-0.885714285714286,-0.857142857142857,-0.828571428571429,
-0.8,-0.771428571428572,-0.742857142857143,-0.714285714285714,-0.685714285714286,
-0.657142857142857,-0.628571428571429,-0.6,-0.571428571428572,-0.542857142857143,
-0.514285714285714,-0.485714285714286,-0.457142857142857,-0.428571428571429,
-0.4,-0.371428571428571,-0.342857142857143,-0.314285714285714,-0.285714285714286,
-0.257142857142857,-0.228571428571429,-0.2,-0.171428571428571,-0.142857142857143,
-0.114285714285714,-0.0857142857142857,-0.0571428571428571,-0.0285714285714286,
0.),(0.,2.9),.UNSPECIFIED.)
GEOMETRIC_REPRESENTATION_ITEM()
RATIONAL_B_SPLINE_SURFACE(((1.,1.),(1.,1.),(1.,1.),(1.,1.),(1.,1.),(1.,
1.),(1.,1.),(1.,1.),(1.,1.),(1.,1.),(1.,1.),(1.,1.),(1.,1.),(1.,1.),(1.,
1.),(1.,1.),(1.,1.),(1.,1.),(1.,1.),(1.,1.),(1.,1.),(1.,1.),(1.,1.),(1.,
1.),(1.,1.),(1.,1.),(1.,1.),(1.,1.),(1.,1.),(1.,1.),(1.,1.),(1.,1.),(1.,
1.),(1.,1.),(1.,1.),(1.,1.),(1.,1.),(1.,1.),(1.,1.),(1.,1.)))
REPRESENTATION_ITEM('')
SURFACE()
);
#541=(
BOUNDED_SURFACE()
B_SPLINE_SURFACE(5,1,((#55173,#55174),(#55175,#55176),(#55177,#55178),(#55179,
#55180),(#55181,#55182),(#55183,#55184),(#55185,#55186),(#55187,#55188),
(#55189,#55190),(#55191,#55192),(#55193,#55194),(#55195,#55196),(#55197,
#55198),(#55199,#55200),(#55201,#55202),(#55203,#55204),(#55205,#55206),
(#55207,#55208),(#55209,#55210),(#55211,#55212),(#55213,#55214),(#55215,
#55216),(#55217,#55218),(#55219,#55220),(#55221,#55222),(#55223,#55224),
(#55225,#55226),(#55227,#55228),(#55229,#55230),(#55231,#55232),(#55233,
#55234),(#55235,#55236),(#55237,#55238),(#55239,#55240),(#55241,#55242),
(#55243,#55244),(#55245,#55246),(#55247,#55248),(#55249,#55250),(#55251,
#55252)),.UNSPECIFIED.,.F.,.F.,.F.)
B_SPLINE_SURFACE_WITH_KNOTS((6,1,1,1,1,1,1,1,1,1,1,1,1,1,1,1,1,1,1,1,1,
1,1,1,1,1,1,1,1,1,1,1,1,1,1,6),(2,2),(-1.,-0.971428571428572,-0.942857142857143,
-0.914285714285714,-0.885714285714286,-0.857142857142857,-0.828571428571429,
-0.8,-0.771428571428572,-0.742857142857143,-0.714285714285714,-0.685714285714286,
-0.657142857142857,-0.628571428571429,-0.6,-0.571428571428572,-0.542857142857143,
-0.514285714285714,-0.485714285714286,-0.457142857142857,-0.428571428571429,
-0.4,-0.371428571428571,-0.342857142857143,-0.314285714285714,-0.285714285714286,
-0.257142857142857,-0.228571428571429,-0.2,-0.171428571428571,-0.142857142857143,
-0.114285714285714,-0.0857142857142857,-0.0571428571428571,-0.0285714285714286,
0.),(0.,2.9),.UNSPECIFIED.)
GEOMETRIC_REPRESENTATION_ITEM()
RATIONAL_B_SPLINE_SURFACE(((1.,1.),(1.,1.),(1.,1.),(1.,1.),(1.,1.),(1.,
1.),(1.,1.),(1.,1.),(1.,1.),(1.,1.),(1.,1.),(1.,1.),(1.,1.),(1.,1.),(1.,
1.),(1.,1.),(1.,1.),(1.,1.),(1.,1.),(1.,1.),(1.,1.),(1.,1.),(1.,1.),(1.,
1.),(1.,1.),(1.,1.),(1.,1.),(1.,1.),(1.,1.),(1.,1.),(1.,1.),(1.,1.),(1.,
1.),(1.,1.),(1.,1.),(1.,1.),(1.,1.),(1.,1.),(1.,1.),(1.,1.)))
REPRESENTATION_ITEM('')
SURFACE()
);
#542=(
BOUNDED_SURFACE()
B_SPLINE_SURFACE(5,1,((#55278,#55279),(#55280,#55281),(#55282,#55283),(#55284,
#55285),(#55286,#55287),(#55288,#55289),(#55290,#55291),(#55292,#55293),
(#55294,#55295),(#55296,#55297),(#55298,#55299),(#55300,#55301),(#55302,
#55303),(#55304,#55305),(#55306,#55307),(#55308,#55309),(#55310,#55311),
(#55312,#55313),(#55314,#55315),(#55316,#55317),(#55318,#55319),(#55320,
#55321),(#55322,#55323),(#55324,#55325),(#55326,#55327),(#55328,#55329),
(#55330,#55331),(#55332,#55333),(#55334,#55335),(#55336,#55337),(#55338,
#55339),(#55340,#55341),(#55342,#55343),(#55344,#55345),(#55346,#55347),
(#55348,#55349),(#55350,#55351),(#55352,#55353),(#55354,#55355),(#55356,
#55357)),.UNSPECIFIED.,.F.,.F.,.F.)
B_SPLINE_SURFACE_WITH_KNOTS((6,1,1,1,1,1,1,1,1,1,1,1,1,1,1,1,1,1,1,1,1,
1,1,1,1,1,1,1,1,1,1,1,1,1,1,6),(2,2),(-1.,-0.971428571428572,-0.942857142857143,
-0.914285714285714,-0.885714285714286,-0.857142857142857,-0.828571428571429,
-0.8,-0.771428571428572,-0.742857142857143,-0.714285714285714,-0.685714285714286,
-0.657142857142857,-0.628571428571429,-0.6,-0.571428571428572,-0.542857142857143,
-0.514285714285714,-0.485714285714286,-0.457142857142857,-0.428571428571429,
-0.4,-0.371428571428571,-0.342857142857143,-0.314285714285714,-0.285714285714286,
-0.257142857142857,-0.228571428571429,-0.2,-0.171428571428571,-0.142857142857143,
-0.114285714285714,-0.0857142857142857,-0.0571428571428571,-0.0285714285714286,
0.),(0.,2.9),.UNSPECIFIED.)
GEOMETRIC_REPRESENTATION_ITEM()
RATIONAL_B_SPLINE_SURFACE(((1.,1.),(1.,1.),(1.,1.),(1.,1.),(1.,1.),(1.,
1.),(1.,1.),(1.,1.),(1.,1.),(1.,1.),(1.,1.),(1.,1.),(1.,1.),(1.,1.),(1.,
1.),(1.,1.),(1.,1.),(1.,1.),(1.,1.),(1.,1.),(1.,1.),(1.,1.),(1.,1.),(1.,
1.),(1.,1.),(1.,1.),(1.,1.),(1.,1.),(1.,1.),(1.,1.),(1.,1.),(1.,1.),(1.,
1.),(1.,1.),(1.,1.),(1.,1.),(1.,1.),(1.,1.),(1.,1.),(1.,1.)))
REPRESENTATION_ITEM('')
SURFACE()
);
#543=(
BOUNDED_SURFACE()
B_SPLINE_SURFACE(5,1,((#55361,#55362),(#55363,#55364),(#55365,#55366),(#55367,
#55368),(#55369,#55370),(#55371,#55372),(#55373,#55374),(#55375,#55376),
(#55377,#55378),(#55379,#55380),(#55381,#55382),(#55383,#55384),(#55385,
#55386),(#55387,#55388),(#55389,#55390),(#55391,#55392),(#55393,#55394),
(#55395,#55396),(#55397,#55398),(#55399,#55400),(#55401,#55402),(#55403,
#55404),(#55405,#55406),(#55407,#55408),(#55409,#55410),(#55411,#55412),
(#55413,#55414),(#55415,#55416),(#55417,#55418),(#55419,#55420),(#55421,
#55422),(#55423,#55424),(#55425,#55426),(#55427,#55428),(#55429,#55430),
(#55431,#55432),(#55433,#55434),(#55435,#55436),(#55437,#55438),(#55439,
#55440)),.UNSPECIFIED.,.F.,.F.,.F.)
B_SPLINE_SURFACE_WITH_KNOTS((6,1,1,1,1,1,1,1,1,1,1,1,1,1,1,1,1,1,1,1,1,
1,1,1,1,1,1,1,1,1,1,1,1,1,1,6),(2,2),(-1.,-0.971428571428572,-0.942857142857143,
-0.914285714285714,-0.885714285714286,-0.857142857142857,-0.828571428571429,
-0.8,-0.771428571428572,-0.742857142857143,-0.714285714285714,-0.685714285714286,
-0.657142857142857,-0.628571428571429,-0.6,-0.571428571428572,-0.542857142857143,
-0.514285714285714,-0.485714285714286,-0.457142857142857,-0.428571428571429,
-0.4,-0.371428571428571,-0.342857142857143,-0.314285714285714,-0.285714285714286,
-0.257142857142857,-0.228571428571429,-0.2,-0.171428571428571,-0.142857142857143,
-0.114285714285714,-0.0857142857142857,-0.0571428571428571,-0.0285714285714286,
0.),(0.,2.9),.UNSPECIFIED.)
GEOMETRIC_REPRESENTATION_ITEM()
RATIONAL_B_SPLINE_SURFACE(((1.,1.),(1.,1.),(1.,1.),(1.,1.),(1.,1.),(1.,
1.),(1.,1.),(1.,1.),(1.,1.),(1.,1.),(1.,1.),(1.,1.),(1.,1.),(1.,1.),(1.,
1.),(1.,1.),(1.,1.),(1.,1.),(1.,1.),(1.,1.),(1.,1.),(1.,1.),(1.,1.),(1.,
1.),(1.,1.),(1.,1.),(1.,1.),(1.,1.),(1.,1.),(1.,1.),(1.,1.),(1.,1.),(1.,
1.),(1.,1.),(1.,1.),(1.,1.),(1.,1.),(1.,1.),(1.,1.),(1.,1.)))
REPRESENTATION_ITEM('')
SURFACE()
);
#544=(
BOUNDED_SURFACE()
B_SPLINE_SURFACE(5,1,((#55457,#55458),(#55459,#55460),(#55461,#55462),(#55463,
#55464),(#55465,#55466),(#55467,#55468),(#55469,#55470),(#55471,#55472),
(#55473,#55474),(#55475,#55476),(#55477,#55478),(#55479,#55480),(#55481,
#55482),(#55483,#55484),(#55485,#55486),(#55487,#55488),(#55489,#55490),
(#55491,#55492),(#55493,#55494),(#55495,#55496),(#55497,#55498),(#55499,
#55500),(#55501,#55502),(#55503,#55504),(#55505,#55506),(#55507,#55508),
(#55509,#55510),(#55511,#55512),(#55513,#55514),(#55515,#55516),(#55517,
#55518),(#55519,#55520),(#55521,#55522),(#55523,#55524),(#55525,#55526),
(#55527,#55528),(#55529,#55530),(#55531,#55532),(#55533,#55534),(#55535,
#55536)),.UNSPECIFIED.,.F.,.F.,.F.)
B_SPLINE_SURFACE_WITH_KNOTS((6,1,1,1,1,1,1,1,1,1,1,1,1,1,1,1,1,1,1,1,1,
1,1,1,1,1,1,1,1,1,1,1,1,1,1,6),(2,2),(-1.,-0.971428571428572,-0.942857142857143,
-0.914285714285714,-0.885714285714286,-0.857142857142857,-0.828571428571429,
-0.8,-0.771428571428572,-0.742857142857143,-0.714285714285714,-0.685714285714286,
-0.657142857142857,-0.628571428571429,-0.6,-0.571428571428572,-0.542857142857143,
-0.514285714285714,-0.485714285714286,-0.457142857142857,-0.428571428571429,
-0.4,-0.371428571428571,-0.342857142857143,-0.314285714285714,-0.285714285714286,
-0.257142857142857,-0.228571428571429,-0.2,-0.171428571428571,-0.142857142857143,
-0.114285714285714,-0.0857142857142857,-0.0571428571428571,-0.0285714285714286,
0.),(0.,2.9),.UNSPECIFIED.)
GEOMETRIC_REPRESENTATION_ITEM()
RATIONAL_B_SPLINE_SURFACE(((1.,1.),(1.,1.),(1.,1.),(1.,1.),(1.,1.),(1.,
1.),(1.,1.),(1.,1.),(1.,1.),(1.,1.),(1.,1.),(1.,1.),(1.,1.),(1.,1.),(1.,
1.),(1.,1.),(1.,1.),(1.,1.),(1.,1.),(1.,1.),(1.,1.),(1.,1.),(1.,1.),(1.,
1.),(1.,1.),(1.,1.),(1.,1.),(1.,1.),(1.,1.),(1.,1.),(1.,1.),(1.,1.),(1.,
1.),(1.,1.),(1.,1.),(1.,1.),(1.,1.),(1.,1.),(1.,1.),(1.,1.)))
REPRESENTATION_ITEM('')
SURFACE()
);
#545=(
BOUNDED_SURFACE()
B_SPLINE_SURFACE(5,1,((#55553,#55554),(#55555,#55556),(#55557,#55558),(#55559,
#55560),(#55561,#55562),(#55563,#55564),(#55565,#55566),(#55567,#55568),
(#55569,#55570),(#55571,#55572),(#55573,#55574),(#55575,#55576),(#55577,
#55578),(#55579,#55580),(#55581,#55582),(#55583,#55584),(#55585,#55586),
(#55587,#55588),(#55589,#55590),(#55591,#55592),(#55593,#55594),(#55595,
#55596),(#55597,#55598),(#55599,#55600),(#55601,#55602),(#55603,#55604),
(#55605,#55606),(#55607,#55608),(#55609,#55610),(#55611,#55612),(#55613,
#55614),(#55615,#55616),(#55617,#55618),(#55619,#55620),(#55621,#55622),
(#55623,#55624),(#55625,#55626),(#55627,#55628),(#55629,#55630),(#55631,
#55632)),.UNSPECIFIED.,.F.,.F.,.F.)
B_SPLINE_SURFACE_WITH_KNOTS((6,1,1,1,1,1,1,1,1,1,1,1,1,1,1,1,1,1,1,1,1,
1,1,1,1,1,1,1,1,1,1,1,1,1,1,6),(2,2),(-1.,-0.971428571428572,-0.942857142857143,
-0.914285714285714,-0.885714285714286,-0.857142857142857,-0.828571428571429,
-0.8,-0.771428571428572,-0.742857142857143,-0.714285714285714,-0.685714285714286,
-0.657142857142857,-0.628571428571429,-0.6,-0.571428571428572,-0.542857142857143,
-0.514285714285714,-0.485714285714286,-0.457142857142857,-0.428571428571429,
-0.4,-0.371428571428571,-0.342857142857143,-0.314285714285714,-0.285714285714286,
-0.257142857142857,-0.228571428571429,-0.2,-0.171428571428571,-0.142857142857143,
-0.114285714285714,-0.0857142857142857,-0.0571428571428571,-0.0285714285714286,
0.),(0.,2.9),.UNSPECIFIED.)
GEOMETRIC_REPRESENTATION_ITEM()
RATIONAL_B_SPLINE_SURFACE(((1.,1.),(1.,1.),(1.,1.),(1.,1.),(1.,1.),(1.,
1.),(1.,1.),(1.,1.),(1.,1.),(1.,1.),(1.,1.),(1.,1.),(1.,1.),(1.,1.),(1.,
1.),(1.,1.),(1.,1.),(1.,1.),(1.,1.),(1.,1.),(1.,1.),(1.,1.),(1.,1.),(1.,
1.),(1.,1.),(1.,1.),(1.,1.),(1.,1.),(1.,1.),(1.,1.),(1.,1.),(1.,1.),(1.,
1.),(1.,1.),(1.,1.),(1.,1.),(1.,1.),(1.,1.),(1.,1.),(1.,1.)))
REPRESENTATION_ITEM('')
SURFACE()
);
#546=(
BOUNDED_SURFACE()
B_SPLINE_SURFACE(5,1,((#55661,#55662),(#55663,#55664),(#55665,#55666),(#55667,
#55668),(#55669,#55670),(#55671,#55672),(#55673,#55674),(#55675,#55676),
(#55677,#55678),(#55679,#55680),(#55681,#55682),(#55683,#55684),(#55685,
#55686),(#55687,#55688),(#55689,#55690),(#55691,#55692),(#55693,#55694),
(#55695,#55696),(#55697,#55698),(#55699,#55700),(#55701,#55702),(#55703,
#55704),(#55705,#55706),(#55707,#55708),(#55709,#55710),(#55711,#55712),
(#55713,#55714),(#55715,#55716),(#55717,#55718),(#55719,#55720),(#55721,
#55722),(#55723,#55724),(#55725,#55726),(#55727,#55728),(#55729,#55730),
(#55731,#55732),(#55733,#55734),(#55735,#55736),(#55737,#55738),(#55739,
#55740)),.UNSPECIFIED.,.F.,.F.,.F.)
B_SPLINE_SURFACE_WITH_KNOTS((6,1,1,1,1,1,1,1,1,1,1,1,1,1,1,1,1,1,1,1,1,
1,1,1,1,1,1,1,1,1,1,1,1,1,1,6),(2,2),(-1.,-0.971428571428572,-0.942857142857143,
-0.914285714285714,-0.885714285714286,-0.857142857142857,-0.828571428571429,
-0.8,-0.771428571428572,-0.742857142857143,-0.714285714285714,-0.685714285714286,
-0.657142857142857,-0.628571428571429,-0.6,-0.571428571428572,-0.542857142857143,
-0.514285714285714,-0.485714285714286,-0.457142857142857,-0.428571428571429,
-0.4,-0.371428571428571,-0.342857142857143,-0.314285714285714,-0.285714285714286,
-0.257142857142857,-0.228571428571429,-0.2,-0.171428571428571,-0.142857142857143,
-0.114285714285714,-0.0857142857142857,-0.0571428571428571,-0.0285714285714286,
0.),(0.,2.9),.UNSPECIFIED.)
GEOMETRIC_REPRESENTATION_ITEM()
RATIONAL_B_SPLINE_SURFACE(((1.,1.),(1.,1.),(1.,1.),(1.,1.),(1.,1.),(1.,
1.),(1.,1.),(1.,1.),(1.,1.),(1.,1.),(1.,1.),(1.,1.),(1.,1.),(1.,1.),(1.,
1.),(1.,1.),(1.,1.),(1.,1.),(1.,1.),(1.,1.),(1.,1.),(1.,1.),(1.,1.),(1.,
1.),(1.,1.),(1.,1.),(1.,1.),(1.,1.),(1.,1.),(1.,1.),(1.,1.),(1.,1.),(1.,
1.),(1.,1.),(1.,1.),(1.,1.),(1.,1.),(1.,1.),(1.,1.),(1.,1.)))
REPRESENTATION_ITEM('')
SURFACE()
);
#547=(
BOUNDED_SURFACE()
B_SPLINE_SURFACE(5,1,((#55744,#55745),(#55746,#55747),(#55748,#55749),(#55750,
#55751),(#55752,#55753),(#55754,#55755),(#55756,#55757),(#55758,#55759),
(#55760,#55761),(#55762,#55763),(#55764,#55765),(#55766,#55767),(#55768,
#55769),(#55770,#55771),(#55772,#55773),(#55774,#55775),(#55776,#55777),
(#55778,#55779),(#55780,#55781),(#55782,#55783),(#55784,#55785),(#55786,
#55787),(#55788,#55789),(#55790,#55791),(#55792,#55793),(#55794,#55795),
(#55796,#55797),(#55798,#55799),(#55800,#55801),(#55802,#55803),(#55804,
#55805),(#55806,#55807),(#55808,#55809),(#55810,#55811),(#55812,#55813),
(#55814,#55815),(#55816,#55817),(#55818,#55819),(#55820,#55821),(#55822,
#55823)),.UNSPECIFIED.,.F.,.F.,.F.)
B_SPLINE_SURFACE_WITH_KNOTS((6,1,1,1,1,1,1,1,1,1,1,1,1,1,1,1,1,1,1,1,1,
1,1,1,1,1,1,1,1,1,1,1,1,1,1,6),(2,2),(-1.,-0.971428571428572,-0.942857142857143,
-0.914285714285714,-0.885714285714286,-0.857142857142857,-0.828571428571429,
-0.8,-0.771428571428572,-0.742857142857143,-0.714285714285714,-0.685714285714286,
-0.657142857142857,-0.628571428571429,-0.6,-0.571428571428572,-0.542857142857143,
-0.514285714285714,-0.485714285714286,-0.457142857142857,-0.428571428571429,
-0.4,-0.371428571428571,-0.342857142857143,-0.314285714285714,-0.285714285714286,
-0.257142857142857,-0.228571428571429,-0.2,-0.171428571428571,-0.142857142857143,
-0.114285714285714,-0.0857142857142857,-0.0571428571428571,-0.0285714285714286,
0.),(0.,2.9),.UNSPECIFIED.)
GEOMETRIC_REPRESENTATION_ITEM()
RATIONAL_B_SPLINE_SURFACE(((1.,1.),(1.,1.),(1.,1.),(1.,1.),(1.,1.),(1.,
1.),(1.,1.),(1.,1.),(1.,1.),(1.,1.),(1.,1.),(1.,1.),(1.,1.),(1.,1.),(1.,
1.),(1.,1.),(1.,1.),(1.,1.),(1.,1.),(1.,1.),(1.,1.),(1.,1.),(1.,1.),(1.,
1.),(1.,1.),(1.,1.),(1.,1.),(1.,1.),(1.,1.),(1.,1.),(1.,1.),(1.,1.),(1.,
1.),(1.,1.),(1.,1.),(1.,1.),(1.,1.),(1.,1.),(1.,1.),(1.,1.)))
REPRESENTATION_ITEM('')
SURFACE()
);
#548=(
BOUNDED_SURFACE()
B_SPLINE_SURFACE(5,1,((#55840,#55841),(#55842,#55843),(#55844,#55845),(#55846,
#55847),(#55848,#55849),(#55850,#55851),(#55852,#55853),(#55854,#55855),
(#55856,#55857),(#55858,#55859),(#55860,#55861),(#55862,#55863),(#55864,
#55865),(#55866,#55867),(#55868,#55869),(#55870,#55871),(#55872,#55873),
(#55874,#55875),(#55876,#55877),(#55878,#55879),(#55880,#55881),(#55882,
#55883),(#55884,#55885),(#55886,#55887),(#55888,#55889),(#55890,#55891),
(#55892,#55893),(#55894,#55895),(#55896,#55897),(#55898,#55899),(#55900,
#55901),(#55902,#55903),(#55904,#55905),(#55906,#55907),(#55908,#55909),
(#55910,#55911),(#55912,#55913),(#55914,#55915),(#55916,#55917),(#55918,
#55919)),.UNSPECIFIED.,.F.,.F.,.F.)
B_SPLINE_SURFACE_WITH_KNOTS((6,1,1,1,1,1,1,1,1,1,1,1,1,1,1,1,1,1,1,1,1,
1,1,1,1,1,1,1,1,1,1,1,1,1,1,6),(2,2),(-1.,-0.971428571428572,-0.942857142857143,
-0.914285714285714,-0.885714285714286,-0.857142857142857,-0.828571428571429,
-0.8,-0.771428571428572,-0.742857142857143,-0.714285714285714,-0.685714285714286,
-0.657142857142857,-0.628571428571429,-0.6,-0.571428571428572,-0.542857142857143,
-0.514285714285714,-0.485714285714286,-0.457142857142857,-0.428571428571429,
-0.4,-0.371428571428571,-0.342857142857143,-0.314285714285714,-0.285714285714286,
-0.257142857142857,-0.228571428571429,-0.2,-0.171428571428571,-0.142857142857143,
-0.114285714285714,-0.0857142857142857,-0.0571428571428571,-0.0285714285714286,
0.),(0.,2.9),.UNSPECIFIED.)
GEOMETRIC_REPRESENTATION_ITEM()
RATIONAL_B_SPLINE_SURFACE(((1.,1.),(1.,1.),(1.,1.),(1.,1.),(1.,1.),(1.,
1.),(1.,1.),(1.,1.),(1.,1.),(1.,1.),(1.,1.),(1.,1.),(1.,1.),(1.,1.),(1.,
1.),(1.,1.),(1.,1.),(1.,1.),(1.,1.),(1.,1.),(1.,1.),(1.,1.),(1.,1.),(1.,
1.),(1.,1.),(1.,1.),(1.,1.),(1.,1.),(1.,1.),(1.,1.),(1.,1.),(1.,1.),(1.,
1.),(1.,1.),(1.,1.),(1.,1.),(1.,1.),(1.,1.),(1.,1.),(1.,1.)))
REPRESENTATION_ITEM('')
SURFACE()
);
#549=(
BOUNDED_SURFACE()
B_SPLINE_SURFACE(5,1,((#55936,#55937),(#55938,#55939),(#55940,#55941),(#55942,
#55943),(#55944,#55945),(#55946,#55947),(#55948,#55949),(#55950,#55951),
(#55952,#55953),(#55954,#55955),(#55956,#55957),(#55958,#55959),(#55960,
#55961),(#55962,#55963),(#55964,#55965),(#55966,#55967),(#55968,#55969),
(#55970,#55971),(#55972,#55973),(#55974,#55975),(#55976,#55977),(#55978,
#55979),(#55980,#55981),(#55982,#55983),(#55984,#55985),(#55986,#55987),
(#55988,#55989),(#55990,#55991),(#55992,#55993),(#55994,#55995),(#55996,
#55997),(#55998,#55999),(#56000,#56001),(#56002,#56003),(#56004,#56005),
(#56006,#56007),(#56008,#56009),(#56010,#56011),(#56012,#56013),(#56014,
#56015)),.UNSPECIFIED.,.F.,.F.,.F.)
B_SPLINE_SURFACE_WITH_KNOTS((6,1,1,1,1,1,1,1,1,1,1,1,1,1,1,1,1,1,1,1,1,
1,1,1,1,1,1,1,1,1,1,1,1,1,1,6),(2,2),(-1.,-0.971428571428572,-0.942857142857143,
-0.914285714285714,-0.885714285714286,-0.857142857142857,-0.828571428571429,
-0.8,-0.771428571428572,-0.742857142857143,-0.714285714285714,-0.685714285714286,
-0.657142857142857,-0.628571428571429,-0.6,-0.571428571428572,-0.542857142857143,
-0.514285714285714,-0.485714285714286,-0.457142857142857,-0.428571428571429,
-0.4,-0.371428571428571,-0.342857142857143,-0.314285714285714,-0.285714285714286,
-0.257142857142857,-0.228571428571429,-0.2,-0.171428571428571,-0.142857142857143,
-0.114285714285714,-0.0857142857142857,-0.0571428571428571,-0.0285714285714286,
0.),(0.,2.9),.UNSPECIFIED.)
GEOMETRIC_REPRESENTATION_ITEM()
RATIONAL_B_SPLINE_SURFACE(((1.,1.),(1.,1.),(1.,1.),(1.,1.),(1.,1.),(1.,
1.),(1.,1.),(1.,1.),(1.,1.),(1.,1.),(1.,1.),(1.,1.),(1.,1.),(1.,1.),(1.,
1.),(1.,1.),(1.,1.),(1.,1.),(1.,1.),(1.,1.),(1.,1.),(1.,1.),(1.,1.),(1.,
1.),(1.,1.),(1.,1.),(1.,1.),(1.,1.),(1.,1.),(1.,1.),(1.,1.),(1.,1.),(1.,
1.),(1.,1.),(1.,1.),(1.,1.),(1.,1.),(1.,1.),(1.,1.),(1.,1.)))
REPRESENTATION_ITEM('')
SURFACE()
);
#550=(
BOUNDED_SURFACE()
B_SPLINE_SURFACE(5,1,((#56041,#56042),(#56043,#56044),(#56045,#56046),(#56047,
#56048),(#56049,#56050),(#56051,#56052),(#56053,#56054),(#56055,#56056),
(#56057,#56058),(#56059,#56060),(#56061,#56062),(#56063,#56064),(#56065,
#56066),(#56067,#56068),(#56069,#56070),(#56071,#56072),(#56073,#56074),
(#56075,#56076),(#56077,#56078),(#56079,#56080),(#56081,#56082),(#56083,
#56084),(#56085,#56086),(#56087,#56088),(#56089,#56090),(#56091,#56092),
(#56093,#56094),(#56095,#56096),(#56097,#56098),(#56099,#56100),(#56101,
#56102),(#56103,#56104),(#56105,#56106),(#56107,#56108),(#56109,#56110),
(#56111,#56112),(#56113,#56114),(#56115,#56116),(#56117,#56118),(#56119,
#56120)),.UNSPECIFIED.,.F.,.F.,.F.)
B_SPLINE_SURFACE_WITH_KNOTS((6,1,1,1,1,1,1,1,1,1,1,1,1,1,1,1,1,1,1,1,1,
1,1,1,1,1,1,1,1,1,1,1,1,1,1,6),(2,2),(-1.,-0.971428571428572,-0.942857142857143,
-0.914285714285714,-0.885714285714286,-0.857142857142857,-0.828571428571429,
-0.8,-0.771428571428572,-0.742857142857143,-0.714285714285714,-0.685714285714286,
-0.657142857142857,-0.628571428571429,-0.6,-0.571428571428572,-0.542857142857143,
-0.514285714285714,-0.485714285714286,-0.457142857142857,-0.428571428571429,
-0.4,-0.371428571428571,-0.342857142857143,-0.314285714285714,-0.285714285714286,
-0.257142857142857,-0.228571428571429,-0.2,-0.171428571428571,-0.142857142857143,
-0.114285714285714,-0.0857142857142857,-0.0571428571428571,-0.0285714285714286,
0.),(0.,2.9),.UNSPECIFIED.)
GEOMETRIC_REPRESENTATION_ITEM()
RATIONAL_B_SPLINE_SURFACE(((1.,1.),(1.,1.),(1.,1.),(1.,1.),(1.,1.),(1.,
1.),(1.,1.),(1.,1.),(1.,1.),(1.,1.),(1.,1.),(1.,1.),(1.,1.),(1.,1.),(1.,
1.),(1.,1.),(1.,1.),(1.,1.),(1.,1.),(1.,1.),(1.,1.),(1.,1.),(1.,1.),(1.,
1.),(1.,1.),(1.,1.),(1.,1.),(1.,1.),(1.,1.),(1.,1.),(1.,1.),(1.,1.),(1.,
1.),(1.,1.),(1.,1.),(1.,1.),(1.,1.),(1.,1.),(1.,1.),(1.,1.)))
REPRESENTATION_ITEM('')
SURFACE()
);
#551=(
BOUNDED_SURFACE()
B_SPLINE_SURFACE(5,1,((#56124,#56125),(#56126,#56127),(#56128,#56129),(#56130,
#56131),(#56132,#56133),(#56134,#56135),(#56136,#56137),(#56138,#56139),
(#56140,#56141),(#56142,#56143),(#56144,#56145),(#56146,#56147),(#56148,
#56149),(#56150,#56151),(#56152,#56153),(#56154,#56155),(#56156,#56157),
(#56158,#56159),(#56160,#56161),(#56162,#56163),(#56164,#56165),(#56166,
#56167),(#56168,#56169),(#56170,#56171),(#56172,#56173),(#56174,#56175),
(#56176,#56177),(#56178,#56179),(#56180,#56181),(#56182,#56183),(#56184,
#56185),(#56186,#56187),(#56188,#56189),(#56190,#56191),(#56192,#56193),
(#56194,#56195),(#56196,#56197),(#56198,#56199),(#56200,#56201),(#56202,
#56203)),.UNSPECIFIED.,.F.,.F.,.F.)
B_SPLINE_SURFACE_WITH_KNOTS((6,1,1,1,1,1,1,1,1,1,1,1,1,1,1,1,1,1,1,1,1,
1,1,1,1,1,1,1,1,1,1,1,1,1,1,6),(2,2),(-1.,-0.971428571428572,-0.942857142857143,
-0.914285714285714,-0.885714285714286,-0.857142857142857,-0.828571428571429,
-0.8,-0.771428571428572,-0.742857142857143,-0.714285714285714,-0.685714285714286,
-0.657142857142857,-0.628571428571429,-0.6,-0.571428571428572,-0.542857142857143,
-0.514285714285714,-0.485714285714286,-0.457142857142857,-0.428571428571429,
-0.4,-0.371428571428571,-0.342857142857143,-0.314285714285714,-0.285714285714286,
-0.257142857142857,-0.228571428571429,-0.2,-0.171428571428571,-0.142857142857143,
-0.114285714285714,-0.0857142857142857,-0.0571428571428571,-0.0285714285714286,
0.),(0.,2.9),.UNSPECIFIED.)
GEOMETRIC_REPRESENTATION_ITEM()
RATIONAL_B_SPLINE_SURFACE(((1.,1.),(1.,1.),(1.,1.),(1.,1.),(1.,1.),(1.,
1.),(1.,1.),(1.,1.),(1.,1.),(1.,1.),(1.,1.),(1.,1.),(1.,1.),(1.,1.),(1.,
1.),(1.,1.),(1.,1.),(1.,1.),(1.,1.),(1.,1.),(1.,1.),(1.,1.),(1.,1.),(1.,
1.),(1.,1.),(1.,1.),(1.,1.),(1.,1.),(1.,1.),(1.,1.),(1.,1.),(1.,1.),(1.,
1.),(1.,1.),(1.,1.),(1.,1.),(1.,1.),(1.,1.),(1.,1.),(1.,1.)))
REPRESENTATION_ITEM('')
SURFACE()
);
#552=(
BOUNDED_SURFACE()
B_SPLINE_SURFACE(5,1,((#56220,#56221),(#56222,#56223),(#56224,#56225),(#56226,
#56227),(#56228,#56229),(#56230,#56231),(#56232,#56233),(#56234,#56235),
(#56236,#56237),(#56238,#56239),(#56240,#56241),(#56242,#56243),(#56244,
#56245),(#56246,#56247),(#56248,#56249),(#56250,#56251),(#56252,#56253),
(#56254,#56255),(#56256,#56257),(#56258,#56259),(#56260,#56261),(#56262,
#56263),(#56264,#56265),(#56266,#56267),(#56268,#56269),(#56270,#56271),
(#56272,#56273),(#56274,#56275),(#56276,#56277),(#56278,#56279),(#56280,
#56281),(#56282,#56283),(#56284,#56285),(#56286,#56287),(#56288,#56289),
(#56290,#56291),(#56292,#56293),(#56294,#56295),(#56296,#56297),(#56298,
#56299)),.UNSPECIFIED.,.F.,.F.,.F.)
B_SPLINE_SURFACE_WITH_KNOTS((6,1,1,1,1,1,1,1,1,1,1,1,1,1,1,1,1,1,1,1,1,
1,1,1,1,1,1,1,1,1,1,1,1,1,1,6),(2,2),(-1.,-0.971428571428572,-0.942857142857143,
-0.914285714285714,-0.885714285714286,-0.857142857142857,-0.828571428571429,
-0.8,-0.771428571428572,-0.742857142857143,-0.714285714285714,-0.685714285714286,
-0.657142857142857,-0.628571428571429,-0.6,-0.571428571428572,-0.542857142857143,
-0.514285714285714,-0.485714285714286,-0.457142857142857,-0.428571428571429,
-0.4,-0.371428571428571,-0.342857142857143,-0.314285714285714,-0.285714285714286,
-0.257142857142857,-0.228571428571429,-0.2,-0.171428571428571,-0.142857142857143,
-0.114285714285714,-0.0857142857142857,-0.0571428571428571,-0.0285714285714286,
0.),(0.,2.9),.UNSPECIFIED.)
GEOMETRIC_REPRESENTATION_ITEM()
RATIONAL_B_SPLINE_SURFACE(((1.,1.),(1.,1.),(1.,1.),(1.,1.),(1.,1.),(1.,
1.),(1.,1.),(1.,1.),(1.,1.),(1.,1.),(1.,1.),(1.,1.),(1.,1.),(1.,1.),(1.,
1.),(1.,1.),(1.,1.),(1.,1.),(1.,1.),(1.,1.),(1.,1.),(1.,1.),(1.,1.),(1.,
1.),(1.,1.),(1.,1.),(1.,1.),(1.,1.),(1.,1.),(1.,1.),(1.,1.),(1.,1.),(1.,
1.),(1.,1.),(1.,1.),(1.,1.),(1.,1.),(1.,1.),(1.,1.),(1.,1.)))
REPRESENTATION_ITEM('')
SURFACE()
);
#553=(
BOUNDED_SURFACE()
B_SPLINE_SURFACE(5,1,((#56316,#56317),(#56318,#56319),(#56320,#56321),(#56322,
#56323),(#56324,#56325),(#56326,#56327),(#56328,#56329),(#56330,#56331),
(#56332,#56333),(#56334,#56335),(#56336,#56337),(#56338,#56339),(#56340,
#56341),(#56342,#56343),(#56344,#56345),(#56346,#56347),(#56348,#56349),
(#56350,#56351),(#56352,#56353),(#56354,#56355),(#56356,#56357),(#56358,
#56359),(#56360,#56361),(#56362,#56363),(#56364,#56365),(#56366,#56367),
(#56368,#56369),(#56370,#56371),(#56372,#56373),(#56374,#56375),(#56376,
#56377),(#56378,#56379),(#56380,#56381),(#56382,#56383),(#56384,#56385),
(#56386,#56387),(#56388,#56389),(#56390,#56391),(#56392,#56393),(#56394,
#56395)),.UNSPECIFIED.,.F.,.F.,.F.)
B_SPLINE_SURFACE_WITH_KNOTS((6,1,1,1,1,1,1,1,1,1,1,1,1,1,1,1,1,1,1,1,1,
1,1,1,1,1,1,1,1,1,1,1,1,1,1,6),(2,2),(-1.,-0.971428571428572,-0.942857142857143,
-0.914285714285714,-0.885714285714286,-0.857142857142857,-0.828571428571429,
-0.8,-0.771428571428572,-0.742857142857143,-0.714285714285714,-0.685714285714286,
-0.657142857142857,-0.628571428571429,-0.6,-0.571428571428572,-0.542857142857143,
-0.514285714285714,-0.485714285714286,-0.457142857142857,-0.428571428571429,
-0.4,-0.371428571428571,-0.342857142857143,-0.314285714285714,-0.285714285714286,
-0.257142857142857,-0.228571428571429,-0.2,-0.171428571428571,-0.142857142857143,
-0.114285714285714,-0.0857142857142857,-0.0571428571428571,-0.0285714285714286,
0.),(0.,2.9),.UNSPECIFIED.)
GEOMETRIC_REPRESENTATION_ITEM()
RATIONAL_B_SPLINE_SURFACE(((1.,1.),(1.,1.),(1.,1.),(1.,1.),(1.,1.),(1.,
1.),(1.,1.),(1.,1.),(1.,1.),(1.,1.),(1.,1.),(1.,1.),(1.,1.),(1.,1.),(1.,
1.),(1.,1.),(1.,1.),(1.,1.),(1.,1.),(1.,1.),(1.,1.),(1.,1.),(1.,1.),(1.,
1.),(1.,1.),(1.,1.),(1.,1.),(1.,1.),(1.,1.),(1.,1.),(1.,1.),(1.,1.),(1.,
1.),(1.,1.),(1.,1.),(1.,1.),(1.,1.),(1.,1.),(1.,1.),(1.,1.)))
REPRESENTATION_ITEM('')
SURFACE()
);
#554=(
BOUNDED_SURFACE()
B_SPLINE_SURFACE(5,1,((#56427,#56428),(#56429,#56430),(#56431,#56432),(#56433,
#56434),(#56435,#56436),(#56437,#56438),(#56439,#56440),(#56441,#56442),
(#56443,#56444),(#56445,#56446),(#56447,#56448),(#56449,#56450),(#56451,
#56452),(#56453,#56454),(#56455,#56456),(#56457,#56458),(#56459,#56460),
(#56461,#56462),(#56463,#56464),(#56465,#56466),(#56467,#56468),(#56469,
#56470),(#56471,#56472),(#56473,#56474),(#56475,#56476),(#56477,#56478),
(#56479,#56480),(#56481,#56482),(#56483,#56484),(#56485,#56486),(#56487,
#56488),(#56489,#56490),(#56491,#56492),(#56493,#56494),(#56495,#56496),
(#56497,#56498),(#56499,#56500),(#56501,#56502),(#56503,#56504),(#56505,
#56506)),.UNSPECIFIED.,.F.,.F.,.F.)
B_SPLINE_SURFACE_WITH_KNOTS((6,1,1,1,1,1,1,1,1,1,1,1,1,1,1,1,1,1,1,1,1,
1,1,1,1,1,1,1,1,1,1,1,1,1,1,6),(2,2),(-1.,-0.971428571428572,-0.942857142857143,
-0.914285714285714,-0.885714285714286,-0.857142857142857,-0.828571428571429,
-0.8,-0.771428571428572,-0.742857142857143,-0.714285714285714,-0.685714285714286,
-0.657142857142857,-0.628571428571429,-0.6,-0.571428571428572,-0.542857142857143,
-0.514285714285714,-0.485714285714286,-0.457142857142857,-0.428571428571429,
-0.4,-0.371428571428571,-0.342857142857143,-0.314285714285714,-0.285714285714286,
-0.257142857142857,-0.228571428571429,-0.2,-0.171428571428571,-0.142857142857143,
-0.114285714285714,-0.0857142857142857,-0.0571428571428571,-0.0285714285714286,
0.),(0.,2.9),.UNSPECIFIED.)
GEOMETRIC_REPRESENTATION_ITEM()
RATIONAL_B_SPLINE_SURFACE(((1.,1.),(1.,1.),(1.,1.),(1.,1.),(1.,1.),(1.,
1.),(1.,1.),(1.,1.),(1.,1.),(1.,1.),(1.,1.),(1.,1.),(1.,1.),(1.,1.),(1.,
1.),(1.,1.),(1.,1.),(1.,1.),(1.,1.),(1.,1.),(1.,1.),(1.,1.),(1.,1.),(1.,
1.),(1.,1.),(1.,1.),(1.,1.),(1.,1.),(1.,1.),(1.,1.),(1.,1.),(1.,1.),(1.,
1.),(1.,1.),(1.,1.),(1.,1.),(1.,1.),(1.,1.),(1.,1.),(1.,1.)))
REPRESENTATION_ITEM('')
SURFACE()
);
#555=(
BOUNDED_SURFACE()
B_SPLINE_SURFACE(5,1,((#56510,#56511),(#56512,#56513),(#56514,#56515),(#56516,
#56517),(#56518,#56519),(#56520,#56521),(#56522,#56523),(#56524,#56525),
(#56526,#56527),(#56528,#56529),(#56530,#56531),(#56532,#56533),(#56534,
#56535),(#56536,#56537),(#56538,#56539),(#56540,#56541),(#56542,#56543),
(#56544,#56545),(#56546,#56547),(#56548,#56549),(#56550,#56551),(#56552,
#56553),(#56554,#56555),(#56556,#56557),(#56558,#56559),(#56560,#56561),
(#56562,#56563),(#56564,#56565),(#56566,#56567),(#56568,#56569),(#56570,
#56571),(#56572,#56573),(#56574,#56575),(#56576,#56577),(#56578,#56579),
(#56580,#56581),(#56582,#56583),(#56584,#56585),(#56586,#56587),(#56588,
#56589)),.UNSPECIFIED.,.F.,.F.,.F.)
B_SPLINE_SURFACE_WITH_KNOTS((6,1,1,1,1,1,1,1,1,1,1,1,1,1,1,1,1,1,1,1,1,
1,1,1,1,1,1,1,1,1,1,1,1,1,1,6),(2,2),(-1.,-0.971428571428572,-0.942857142857143,
-0.914285714285714,-0.885714285714286,-0.857142857142857,-0.828571428571429,
-0.8,-0.771428571428572,-0.742857142857143,-0.714285714285714,-0.685714285714286,
-0.657142857142857,-0.628571428571429,-0.6,-0.571428571428572,-0.542857142857143,
-0.514285714285714,-0.485714285714286,-0.457142857142857,-0.428571428571429,
-0.4,-0.371428571428571,-0.342857142857143,-0.314285714285714,-0.285714285714286,
-0.257142857142857,-0.228571428571429,-0.2,-0.171428571428571,-0.142857142857143,
-0.114285714285714,-0.0857142857142857,-0.0571428571428571,-0.0285714285714286,
0.),(0.,2.9),.UNSPECIFIED.)
GEOMETRIC_REPRESENTATION_ITEM()
RATIONAL_B_SPLINE_SURFACE(((1.,1.),(1.,1.),(1.,1.),(1.,1.),(1.,1.),(1.,
1.),(1.,1.),(1.,1.),(1.,1.),(1.,1.),(1.,1.),(1.,1.),(1.,1.),(1.,1.),(1.,
1.),(1.,1.),(1.,1.),(1.,1.),(1.,1.),(1.,1.),(1.,1.),(1.,1.),(1.,1.),(1.,
1.),(1.,1.),(1.,1.),(1.,1.),(1.,1.),(1.,1.),(1.,1.),(1.,1.),(1.,1.),(1.,
1.),(1.,1.),(1.,1.),(1.,1.),(1.,1.),(1.,1.),(1.,1.),(1.,1.)))
REPRESENTATION_ITEM('')
SURFACE()
);
#556=(
BOUNDED_SURFACE()
B_SPLINE_SURFACE(5,1,((#56606,#56607),(#56608,#56609),(#56610,#56611),(#56612,
#56613),(#56614,#56615),(#56616,#56617),(#56618,#56619),(#56620,#56621),
(#56622,#56623),(#56624,#56625),(#56626,#56627),(#56628,#56629),(#56630,
#56631),(#56632,#56633),(#56634,#56635),(#56636,#56637),(#56638,#56639),
(#56640,#56641),(#56642,#56643),(#56644,#56645),(#56646,#56647),(#56648,
#56649),(#56650,#56651),(#56652,#56653),(#56654,#56655),(#56656,#56657),
(#56658,#56659),(#56660,#56661),(#56662,#56663),(#56664,#56665),(#56666,
#56667),(#56668,#56669),(#56670,#56671),(#56672,#56673),(#56674,#56675),
(#56676,#56677),(#56678,#56679),(#56680,#56681),(#56682,#56683),(#56684,
#56685)),.UNSPECIFIED.,.F.,.F.,.F.)
B_SPLINE_SURFACE_WITH_KNOTS((6,1,1,1,1,1,1,1,1,1,1,1,1,1,1,1,1,1,1,1,1,
1,1,1,1,1,1,1,1,1,1,1,1,1,1,6),(2,2),(-1.,-0.971428571428572,-0.942857142857143,
-0.914285714285714,-0.885714285714286,-0.857142857142857,-0.828571428571429,
-0.8,-0.771428571428572,-0.742857142857143,-0.714285714285714,-0.685714285714286,
-0.657142857142857,-0.628571428571429,-0.6,-0.571428571428572,-0.542857142857143,
-0.514285714285714,-0.485714285714286,-0.457142857142857,-0.428571428571429,
-0.4,-0.371428571428571,-0.342857142857143,-0.314285714285714,-0.285714285714286,
-0.257142857142857,-0.228571428571429,-0.2,-0.171428571428571,-0.142857142857143,
-0.114285714285714,-0.0857142857142857,-0.0571428571428571,-0.0285714285714286,
0.),(0.,2.9),.UNSPECIFIED.)
GEOMETRIC_REPRESENTATION_ITEM()
RATIONAL_B_SPLINE_SURFACE(((1.,1.),(1.,1.),(1.,1.),(1.,1.),(1.,1.),(1.,
1.),(1.,1.),(1.,1.),(1.,1.),(1.,1.),(1.,1.),(1.,1.),(1.,1.),(1.,1.),(1.,
1.),(1.,1.),(1.,1.),(1.,1.),(1.,1.),(1.,1.),(1.,1.),(1.,1.),(1.,1.),(1.,
1.),(1.,1.),(1.,1.),(1.,1.),(1.,1.),(1.,1.),(1.,1.),(1.,1.),(1.,1.),(1.,
1.),(1.,1.),(1.,1.),(1.,1.),(1.,1.),(1.,1.),(1.,1.),(1.,1.)))
REPRESENTATION_ITEM('')
SURFACE()
);
#557=(
BOUNDED_SURFACE()
B_SPLINE_SURFACE(5,1,((#56700,#56701),(#56702,#56703),(#56704,#56705),(#56706,
#56707),(#56708,#56709),(#56710,#56711),(#56712,#56713),(#56714,#56715),
(#56716,#56717),(#56718,#56719),(#56720,#56721),(#56722,#56723),(#56724,
#56725),(#56726,#56727),(#56728,#56729),(#56730,#56731),(#56732,#56733),
(#56734,#56735),(#56736,#56737),(#56738,#56739),(#56740,#56741),(#56742,
#56743),(#56744,#56745),(#56746,#56747),(#56748,#56749),(#56750,#56751),
(#56752,#56753),(#56754,#56755),(#56756,#56757),(#56758,#56759),(#56760,
#56761),(#56762,#56763),(#56764,#56765),(#56766,#56767),(#56768,#56769),
(#56770,#56771),(#56772,#56773),(#56774,#56775),(#56776,#56777),(#56778,
#56779)),.UNSPECIFIED.,.F.,.F.,.F.)
B_SPLINE_SURFACE_WITH_KNOTS((6,1,1,1,1,1,1,1,1,1,1,1,1,1,1,1,1,1,1,1,1,
1,1,1,1,1,1,1,1,1,1,1,1,1,1,6),(2,2),(-1.,-0.971428571428572,-0.942857142857143,
-0.914285714285714,-0.885714285714286,-0.857142857142857,-0.828571428571429,
-0.8,-0.771428571428572,-0.742857142857143,-0.714285714285714,-0.685714285714286,
-0.657142857142857,-0.628571428571429,-0.6,-0.571428571428572,-0.542857142857143,
-0.514285714285714,-0.485714285714286,-0.457142857142857,-0.428571428571429,
-0.4,-0.371428571428571,-0.342857142857143,-0.314285714285714,-0.285714285714286,
-0.257142857142857,-0.228571428571429,-0.2,-0.171428571428571,-0.142857142857143,
-0.114285714285714,-0.0857142857142857,-0.0571428571428571,-0.0285714285714286,
0.),(0.,2.9),.UNSPECIFIED.)
GEOMETRIC_REPRESENTATION_ITEM()
RATIONAL_B_SPLINE_SURFACE(((1.,1.),(1.,1.),(1.,1.),(1.,1.),(1.,1.),(1.,
1.),(1.,1.),(1.,1.),(1.,1.),(1.,1.),(1.,1.),(1.,1.),(1.,1.),(1.,1.),(1.,
1.),(1.,1.),(1.,1.),(1.,1.),(1.,1.),(1.,1.),(1.,1.),(1.,1.),(1.,1.),(1.,
1.),(1.,1.),(1.,1.),(1.,1.),(1.,1.),(1.,1.),(1.,1.),(1.,1.),(1.,1.),(1.,
1.),(1.,1.),(1.,1.),(1.,1.),(1.,1.),(1.,1.),(1.,1.),(1.,1.)))
REPRESENTATION_ITEM('')
SURFACE()
);
#558=(
BOUNDED_SURFACE()
B_SPLINE_SURFACE(5,1,((#56780,#56781),(#56782,#56783),(#56784,#56785),(#56786,
#56787),(#56788,#56789),(#56790,#56791),(#56792,#56793),(#56794,#56795),
(#56796,#56797),(#56798,#56799),(#56800,#56801),(#56802,#56803),(#56804,
#56805),(#56806,#56807),(#56808,#56809),(#56810,#56811),(#56812,#56813),
(#56814,#56815),(#56816,#56817),(#56818,#56819),(#56820,#56821),(#56822,
#56823),(#56824,#56825),(#56826,#56827),(#56828,#56829),(#56830,#56831),
(#56832,#56833),(#56834,#56835),(#56836,#56837),(#56838,#56839),(#56840,
#56841),(#56842,#56843),(#56844,#56845),(#56846,#56847),(#56848,#56849),
(#56850,#56851),(#56852,#56853),(#56854,#56855),(#56856,#56857),(#56858,
#56859)),.UNSPECIFIED.,.F.,.F.,.F.)
B_SPLINE_SURFACE_WITH_KNOTS((6,1,1,1,1,1,1,1,1,1,1,1,1,1,1,1,1,1,1,1,1,
1,1,1,1,1,1,1,1,1,1,1,1,1,1,6),(2,2),(-1.,-0.971428571428572,-0.942857142857143,
-0.914285714285714,-0.885714285714286,-0.857142857142857,-0.828571428571429,
-0.8,-0.771428571428572,-0.742857142857143,-0.714285714285714,-0.685714285714286,
-0.657142857142857,-0.628571428571429,-0.6,-0.571428571428572,-0.542857142857143,
-0.514285714285714,-0.485714285714286,-0.457142857142857,-0.428571428571429,
-0.4,-0.371428571428571,-0.342857142857143,-0.314285714285714,-0.285714285714286,
-0.257142857142857,-0.228571428571429,-0.2,-0.171428571428571,-0.142857142857143,
-0.114285714285714,-0.0857142857142857,-0.0571428571428571,-0.0285714285714286,
0.),(0.,1.6),.UNSPECIFIED.)
GEOMETRIC_REPRESENTATION_ITEM()
RATIONAL_B_SPLINE_SURFACE(((1.,1.),(1.,1.),(1.,1.),(1.,1.),(1.,1.),(1.,
1.),(1.,1.),(1.,1.),(1.,1.),(1.,1.),(1.,1.),(1.,1.),(1.,1.),(1.,1.),(1.,
1.),(1.,1.),(1.,1.),(1.,1.),(1.,1.),(1.,1.),(1.,1.),(1.,1.),(1.,1.),(1.,
1.),(1.,1.),(1.,1.),(1.,1.),(1.,1.),(1.,1.),(1.,1.),(1.,1.),(1.,1.),(1.,
1.),(1.,1.),(1.,1.),(1.,1.),(1.,1.),(1.,1.),(1.,1.),(1.,1.)))
REPRESENTATION_ITEM('')
SURFACE()
);
#559=(
BOUNDED_SURFACE()
B_SPLINE_SURFACE(5,1,((#56879,#56880),(#56881,#56882),(#56883,#56884),(#56885,
#56886),(#56887,#56888),(#56889,#56890),(#56891,#56892),(#56893,#56894),
(#56895,#56896),(#56897,#56898),(#56899,#56900),(#56901,#56902),(#56903,
#56904),(#56905,#56906),(#56907,#56908),(#56909,#56910),(#56911,#56912),
(#56913,#56914),(#56915,#56916),(#56917,#56918),(#56919,#56920),(#56921,
#56922),(#56923,#56924),(#56925,#56926),(#56927,#56928),(#56929,#56930),
(#56931,#56932),(#56933,#56934),(#56935,#56936),(#56937,#56938),(#56939,
#56940),(#56941,#56942),(#56943,#56944),(#56945,#56946),(#56947,#56948),
(#56949,#56950),(#56951,#56952),(#56953,#56954),(#56955,#56956),(#56957,
#56958)),.UNSPECIFIED.,.F.,.F.,.F.)
B_SPLINE_SURFACE_WITH_KNOTS((6,1,1,1,1,1,1,1,1,1,1,1,1,1,1,1,1,1,1,1,1,
1,1,1,1,1,1,1,1,1,1,1,1,1,1,6),(2,2),(-1.,-0.971428571428572,-0.942857142857143,
-0.914285714285714,-0.885714285714286,-0.857142857142857,-0.828571428571429,
-0.8,-0.771428571428572,-0.742857142857143,-0.714285714285714,-0.685714285714286,
-0.657142857142857,-0.628571428571429,-0.6,-0.571428571428572,-0.542857142857143,
-0.514285714285714,-0.485714285714286,-0.457142857142857,-0.428571428571429,
-0.4,-0.371428571428571,-0.342857142857143,-0.314285714285714,-0.285714285714286,
-0.257142857142857,-0.228571428571429,-0.2,-0.171428571428571,-0.142857142857143,
-0.114285714285714,-0.0857142857142857,-0.0571428571428571,-0.0285714285714286,
0.),(0.,1.6),.UNSPECIFIED.)
GEOMETRIC_REPRESENTATION_ITEM()
RATIONAL_B_SPLINE_SURFACE(((1.,1.),(1.,1.),(1.,1.),(1.,1.),(1.,1.),(1.,
1.),(1.,1.),(1.,1.),(1.,1.),(1.,1.),(1.,1.),(1.,1.),(1.,1.),(1.,1.),(1.,
1.),(1.,1.),(1.,1.),(1.,1.),(1.,1.),(1.,1.),(1.,1.),(1.,1.),(1.,1.),(1.,
1.),(1.,1.),(1.,1.),(1.,1.),(1.,1.),(1.,1.),(1.,1.),(1.,1.),(1.,1.),(1.,
1.),(1.,1.),(1.,1.),(1.,1.),(1.,1.),(1.,1.),(1.,1.),(1.,1.)))
REPRESENTATION_ITEM('')
SURFACE()
);
#560=(
BOUNDED_SURFACE()
B_SPLINE_SURFACE(5,1,((#57004,#57005),(#57006,#57007),(#57008,#57009),(#57010,
#57011),(#57012,#57013),(#57014,#57015),(#57016,#57017),(#57018,#57019),
(#57020,#57021),(#57022,#57023),(#57024,#57025),(#57026,#57027),(#57028,
#57029),(#57030,#57031),(#57032,#57033),(#57034,#57035),(#57036,#57037),
(#57038,#57039),(#57040,#57041),(#57042,#57043),(#57044,#57045),(#57046,
#57047),(#57048,#57049),(#57050,#57051),(#57052,#57053),(#57054,#57055),
(#57056,#57057),(#57058,#57059),(#57060,#57061),(#57062,#57063),(#57064,
#57065),(#57066,#57067),(#57068,#57069),(#57070,#57071),(#57072,#57073),
(#57074,#57075),(#57076,#57077),(#57078,#57079),(#57080,#57081),(#57082,
#57083)),.UNSPECIFIED.,.F.,.F.,.F.)
B_SPLINE_SURFACE_WITH_KNOTS((6,1,1,1,1,1,1,1,1,1,1,1,1,1,1,1,1,1,1,1,1,
1,1,1,1,1,1,1,1,1,1,1,1,1,1,6),(2,2),(-1.,-0.971428571428572,-0.942857142857143,
-0.914285714285714,-0.885714285714286,-0.857142857142857,-0.828571428571429,
-0.8,-0.771428571428572,-0.742857142857143,-0.714285714285714,-0.685714285714286,
-0.657142857142857,-0.628571428571429,-0.6,-0.571428571428572,-0.542857142857143,
-0.514285714285714,-0.485714285714286,-0.457142857142857,-0.428571428571429,
-0.4,-0.371428571428571,-0.342857142857143,-0.314285714285714,-0.285714285714286,
-0.257142857142857,-0.228571428571429,-0.2,-0.171428571428571,-0.142857142857143,
-0.114285714285714,-0.0857142857142857,-0.0571428571428571,-0.0285714285714286,
0.),(0.,1.6),.UNSPECIFIED.)
GEOMETRIC_REPRESENTATION_ITEM()
RATIONAL_B_SPLINE_SURFACE(((1.,1.),(1.,1.),(1.,1.),(1.,1.),(1.,1.),(1.,
1.),(1.,1.),(1.,1.),(1.,1.),(1.,1.),(1.,1.),(1.,1.),(1.,1.),(1.,1.),(1.,
1.),(1.,1.),(1.,1.),(1.,1.),(1.,1.),(1.,1.),(1.,1.),(1.,1.),(1.,1.),(1.,
1.),(1.,1.),(1.,1.),(1.,1.),(1.,1.),(1.,1.),(1.,1.),(1.,1.),(1.,1.),(1.,
1.),(1.,1.),(1.,1.),(1.,1.),(1.,1.),(1.,1.),(1.,1.),(1.,1.)))
REPRESENTATION_ITEM('')
SURFACE()
);
#561=(
BOUNDED_SURFACE()
B_SPLINE_SURFACE(5,1,((#57103,#57104),(#57105,#57106),(#57107,#57108),(#57109,
#57110),(#57111,#57112),(#57113,#57114),(#57115,#57116),(#57117,#57118),
(#57119,#57120),(#57121,#57122),(#57123,#57124),(#57125,#57126),(#57127,
#57128),(#57129,#57130),(#57131,#57132),(#57133,#57134),(#57135,#57136),
(#57137,#57138),(#57139,#57140),(#57141,#57142),(#57143,#57144),(#57145,
#57146),(#57147,#57148),(#57149,#57150),(#57151,#57152),(#57153,#57154),
(#57155,#57156),(#57157,#57158),(#57159,#57160),(#57161,#57162),(#57163,
#57164),(#57165,#57166),(#57167,#57168),(#57169,#57170),(#57171,#57172),
(#57173,#57174),(#57175,#57176),(#57177,#57178),(#57179,#57180),(#57181,
#57182)),.UNSPECIFIED.,.F.,.F.,.F.)
B_SPLINE_SURFACE_WITH_KNOTS((6,1,1,1,1,1,1,1,1,1,1,1,1,1,1,1,1,1,1,1,1,
1,1,1,1,1,1,1,1,1,1,1,1,1,1,6),(2,2),(-1.,-0.971428571428572,-0.942857142857143,
-0.914285714285714,-0.885714285714286,-0.857142857142857,-0.828571428571429,
-0.8,-0.771428571428572,-0.742857142857143,-0.714285714285714,-0.685714285714286,
-0.657142857142857,-0.628571428571429,-0.6,-0.571428571428572,-0.542857142857143,
-0.514285714285714,-0.485714285714286,-0.457142857142857,-0.428571428571429,
-0.4,-0.371428571428571,-0.342857142857143,-0.314285714285714,-0.285714285714286,
-0.257142857142857,-0.228571428571429,-0.2,-0.171428571428571,-0.142857142857143,
-0.114285714285714,-0.0857142857142857,-0.0571428571428571,-0.0285714285714286,
0.),(0.,1.6),.UNSPECIFIED.)
GEOMETRIC_REPRESENTATION_ITEM()
RATIONAL_B_SPLINE_SURFACE(((1.,1.),(1.,1.),(1.,1.),(1.,1.),(1.,1.),(1.,
1.),(1.,1.),(1.,1.),(1.,1.),(1.,1.),(1.,1.),(1.,1.),(1.,1.),(1.,1.),(1.,
1.),(1.,1.),(1.,1.),(1.,1.),(1.,1.),(1.,1.),(1.,1.),(1.,1.),(1.,1.),(1.,
1.),(1.,1.),(1.,1.),(1.,1.),(1.,1.),(1.,1.),(1.,1.),(1.,1.),(1.,1.),(1.,
1.),(1.,1.),(1.,1.),(1.,1.),(1.,1.),(1.,1.),(1.,1.),(1.,1.)))
REPRESENTATION_ITEM('')
SURFACE()
);
#562=(
BOUNDED_SURFACE()
B_SPLINE_SURFACE(5,1,((#57202,#57203),(#57204,#57205),(#57206,#57207),(#57208,
#57209),(#57210,#57211),(#57212,#57213),(#57214,#57215),(#57216,#57217),
(#57218,#57219),(#57220,#57221),(#57222,#57223),(#57224,#57225),(#57226,
#57227),(#57228,#57229),(#57230,#57231),(#57232,#57233),(#57234,#57235),
(#57236,#57237),(#57238,#57239),(#57240,#57241),(#57242,#57243),(#57244,
#57245),(#57246,#57247),(#57248,#57249),(#57250,#57251),(#57252,#57253),
(#57254,#57255),(#57256,#57257),(#57258,#57259),(#57260,#57261),(#57262,
#57263),(#57264,#57265),(#57266,#57267),(#57268,#57269),(#57270,#57271),
(#57272,#57273),(#57274,#57275),(#57276,#57277),(#57278,#57279),(#57280,
#57281)),.UNSPECIFIED.,.F.,.F.,.F.)
B_SPLINE_SURFACE_WITH_KNOTS((6,1,1,1,1,1,1,1,1,1,1,1,1,1,1,1,1,1,1,1,1,
1,1,1,1,1,1,1,1,1,1,1,1,1,1,6),(2,2),(-1.,-0.971428571428572,-0.942857142857143,
-0.914285714285714,-0.885714285714286,-0.857142857142857,-0.828571428571429,
-0.8,-0.771428571428572,-0.742857142857143,-0.714285714285714,-0.685714285714286,
-0.657142857142857,-0.628571428571429,-0.6,-0.571428571428572,-0.542857142857143,
-0.514285714285714,-0.485714285714286,-0.457142857142857,-0.428571428571429,
-0.4,-0.371428571428571,-0.342857142857143,-0.314285714285714,-0.285714285714286,
-0.257142857142857,-0.228571428571429,-0.2,-0.171428571428571,-0.142857142857143,
-0.114285714285714,-0.0857142857142857,-0.0571428571428571,-0.0285714285714286,
0.),(0.,1.6),.UNSPECIFIED.)
GEOMETRIC_REPRESENTATION_ITEM()
RATIONAL_B_SPLINE_SURFACE(((1.,1.),(1.,1.),(1.,1.),(1.,1.),(1.,1.),(1.,
1.),(1.,1.),(1.,1.),(1.,1.),(1.,1.),(1.,1.),(1.,1.),(1.,1.),(1.,1.),(1.,
1.),(1.,1.),(1.,1.),(1.,1.),(1.,1.),(1.,1.),(1.,1.),(1.,1.),(1.,1.),(1.,
1.),(1.,1.),(1.,1.),(1.,1.),(1.,1.),(1.,1.),(1.,1.),(1.,1.),(1.,1.),(1.,
1.),(1.,1.),(1.,1.),(1.,1.),(1.,1.),(1.,1.),(1.,1.),(1.,1.)))
REPRESENTATION_ITEM('')
SURFACE()
);
#563=(
BOUNDED_SURFACE()
B_SPLINE_SURFACE(5,1,((#57301,#57302),(#57303,#57304),(#57305,#57306),(#57307,
#57308),(#57309,#57310),(#57311,#57312),(#57313,#57314),(#57315,#57316),
(#57317,#57318),(#57319,#57320),(#57321,#57322),(#57323,#57324),(#57325,
#57326),(#57327,#57328),(#57329,#57330),(#57331,#57332),(#57333,#57334),
(#57335,#57336),(#57337,#57338),(#57339,#57340),(#57341,#57342),(#57343,
#57344),(#57345,#57346),(#57347,#57348),(#57349,#57350),(#57351,#57352),
(#57353,#57354),(#57355,#57356),(#57357,#57358),(#57359,#57360),(#57361,
#57362),(#57363,#57364),(#57365,#57366),(#57367,#57368),(#57369,#57370),
(#57371,#57372),(#57373,#57374),(#57375,#57376),(#57377,#57378),(#57379,
#57380)),.UNSPECIFIED.,.F.,.F.,.F.)
B_SPLINE_SURFACE_WITH_KNOTS((6,1,1,1,1,1,1,1,1,1,1,1,1,1,1,1,1,1,1,1,1,
1,1,1,1,1,1,1,1,1,1,1,1,1,1,6),(2,2),(-1.,-0.971428571428572,-0.942857142857143,
-0.914285714285714,-0.885714285714286,-0.857142857142857,-0.828571428571429,
-0.8,-0.771428571428572,-0.742857142857143,-0.714285714285714,-0.685714285714286,
-0.657142857142857,-0.628571428571429,-0.6,-0.571428571428572,-0.542857142857143,
-0.514285714285714,-0.485714285714286,-0.457142857142857,-0.428571428571429,
-0.4,-0.371428571428571,-0.342857142857143,-0.314285714285714,-0.285714285714286,
-0.257142857142857,-0.228571428571429,-0.2,-0.171428571428571,-0.142857142857143,
-0.114285714285714,-0.0857142857142857,-0.0571428571428571,-0.0285714285714286,
0.),(0.,1.6),.UNSPECIFIED.)
GEOMETRIC_REPRESENTATION_ITEM()
RATIONAL_B_SPLINE_SURFACE(((1.,1.),(1.,1.),(1.,1.),(1.,1.),(1.,1.),(1.,
1.),(1.,1.),(1.,1.),(1.,1.),(1.,1.),(1.,1.),(1.,1.),(1.,1.),(1.,1.),(1.,
1.),(1.,1.),(1.,1.),(1.,1.),(1.,1.),(1.,1.),(1.,1.),(1.,1.),(1.,1.),(1.,
1.),(1.,1.),(1.,1.),(1.,1.),(1.,1.),(1.,1.),(1.,1.),(1.,1.),(1.,1.),(1.,
1.),(1.,1.),(1.,1.),(1.,1.),(1.,1.),(1.,1.),(1.,1.),(1.,1.)))
REPRESENTATION_ITEM('')
SURFACE()
);
#564=(
BOUNDED_SURFACE()
B_SPLINE_SURFACE(5,1,((#57400,#57401),(#57402,#57403),(#57404,#57405),(#57406,
#57407),(#57408,#57409),(#57410,#57411),(#57412,#57413),(#57414,#57415),
(#57416,#57417),(#57418,#57419),(#57420,#57421),(#57422,#57423),(#57424,
#57425),(#57426,#57427),(#57428,#57429),(#57430,#57431),(#57432,#57433),
(#57434,#57435),(#57436,#57437),(#57438,#57439),(#57440,#57441),(#57442,
#57443),(#57444,#57445),(#57446,#57447),(#57448,#57449),(#57450,#57451),
(#57452,#57453),(#57454,#57455),(#57456,#57457),(#57458,#57459),(#57460,
#57461),(#57462,#57463),(#57464,#57465),(#57466,#57467),(#57468,#57469),
(#57470,#57471),(#57472,#57473),(#57474,#57475),(#57476,#57477),(#57478,
#57479)),.UNSPECIFIED.,.F.,.F.,.F.)
B_SPLINE_SURFACE_WITH_KNOTS((6,1,1,1,1,1,1,1,1,1,1,1,1,1,1,1,1,1,1,1,1,
1,1,1,1,1,1,1,1,1,1,1,1,1,1,6),(2,2),(-1.,-0.971428571428572,-0.942857142857143,
-0.914285714285714,-0.885714285714286,-0.857142857142857,-0.828571428571429,
-0.8,-0.771428571428572,-0.742857142857143,-0.714285714285714,-0.685714285714286,
-0.657142857142857,-0.628571428571429,-0.6,-0.571428571428572,-0.542857142857143,
-0.514285714285714,-0.485714285714286,-0.457142857142857,-0.428571428571429,
-0.4,-0.371428571428571,-0.342857142857143,-0.314285714285714,-0.285714285714286,
-0.257142857142857,-0.228571428571429,-0.2,-0.171428571428571,-0.142857142857143,
-0.114285714285714,-0.0857142857142857,-0.0571428571428571,-0.0285714285714286,
0.),(0.,1.6),.UNSPECIFIED.)
GEOMETRIC_REPRESENTATION_ITEM()
RATIONAL_B_SPLINE_SURFACE(((1.,1.),(1.,1.),(1.,1.),(1.,1.),(1.,1.),(1.,
1.),(1.,1.),(1.,1.),(1.,1.),(1.,1.),(1.,1.),(1.,1.),(1.,1.),(1.,1.),(1.,
1.),(1.,1.),(1.,1.),(1.,1.),(1.,1.),(1.,1.),(1.,1.),(1.,1.),(1.,1.),(1.,
1.),(1.,1.),(1.,1.),(1.,1.),(1.,1.),(1.,1.),(1.,1.),(1.,1.),(1.,1.),(1.,
1.),(1.,1.),(1.,1.),(1.,1.),(1.,1.),(1.,1.),(1.,1.),(1.,1.)))
REPRESENTATION_ITEM('')
SURFACE()
);
#565=(
BOUNDED_SURFACE()
B_SPLINE_SURFACE(5,1,((#57499,#57500),(#57501,#57502),(#57503,#57504),(#57505,
#57506),(#57507,#57508),(#57509,#57510),(#57511,#57512),(#57513,#57514),
(#57515,#57516),(#57517,#57518),(#57519,#57520),(#57521,#57522),(#57523,
#57524),(#57525,#57526),(#57527,#57528),(#57529,#57530),(#57531,#57532),
(#57533,#57534),(#57535,#57536),(#57537,#57538),(#57539,#57540),(#57541,
#57542),(#57543,#57544),(#57545,#57546),(#57547,#57548),(#57549,#57550),
(#57551,#57552),(#57553,#57554),(#57555,#57556),(#57557,#57558),(#57559,
#57560),(#57561,#57562),(#57563,#57564),(#57565,#57566),(#57567,#57568),
(#57569,#57570),(#57571,#57572),(#57573,#57574),(#57575,#57576),(#57577,
#57578)),.UNSPECIFIED.,.F.,.F.,.F.)
B_SPLINE_SURFACE_WITH_KNOTS((6,1,1,1,1,1,1,1,1,1,1,1,1,1,1,1,1,1,1,1,1,
1,1,1,1,1,1,1,1,1,1,1,1,1,1,6),(2,2),(-1.,-0.971428571428572,-0.942857142857143,
-0.914285714285714,-0.885714285714286,-0.857142857142857,-0.828571428571429,
-0.8,-0.771428571428572,-0.742857142857143,-0.714285714285714,-0.685714285714286,
-0.657142857142857,-0.628571428571429,-0.6,-0.571428571428572,-0.542857142857143,
-0.514285714285714,-0.485714285714286,-0.457142857142857,-0.428571428571429,
-0.4,-0.371428571428571,-0.342857142857143,-0.314285714285714,-0.285714285714286,
-0.257142857142857,-0.228571428571429,-0.2,-0.171428571428571,-0.142857142857143,
-0.114285714285714,-0.0857142857142857,-0.0571428571428571,-0.0285714285714286,
0.),(0.,1.6),.UNSPECIFIED.)
GEOMETRIC_REPRESENTATION_ITEM()
RATIONAL_B_SPLINE_SURFACE(((1.,1.),(1.,1.),(1.,1.),(1.,1.),(1.,1.),(1.,
1.),(1.,1.),(1.,1.),(1.,1.),(1.,1.),(1.,1.),(1.,1.),(1.,1.),(1.,1.),(1.,
1.),(1.,1.),(1.,1.),(1.,1.),(1.,1.),(1.,1.),(1.,1.),(1.,1.),(1.,1.),(1.,
1.),(1.,1.),(1.,1.),(1.,1.),(1.,1.),(1.,1.),(1.,1.),(1.,1.),(1.,1.),(1.,
1.),(1.,1.),(1.,1.),(1.,1.),(1.,1.),(1.,1.),(1.,1.),(1.,1.)))
REPRESENTATION_ITEM('')
SURFACE()
);
#566=(
BOUNDED_SURFACE()
B_SPLINE_SURFACE(5,1,((#57598,#57599),(#57600,#57601),(#57602,#57603),(#57604,
#57605),(#57606,#57607),(#57608,#57609),(#57610,#57611),(#57612,#57613),
(#57614,#57615),(#57616,#57617),(#57618,#57619),(#57620,#57621),(#57622,
#57623),(#57624,#57625),(#57626,#57627),(#57628,#57629),(#57630,#57631),
(#57632,#57633),(#57634,#57635),(#57636,#57637),(#57638,#57639),(#57640,
#57641),(#57642,#57643),(#57644,#57645),(#57646,#57647),(#57648,#57649),
(#57650,#57651),(#57652,#57653),(#57654,#57655),(#57656,#57657),(#57658,
#57659),(#57660,#57661),(#57662,#57663),(#57664,#57665),(#57666,#57667),
(#57668,#57669),(#57670,#57671),(#57672,#57673),(#57674,#57675),(#57676,
#57677)),.UNSPECIFIED.,.F.,.F.,.F.)
B_SPLINE_SURFACE_WITH_KNOTS((6,1,1,1,1,1,1,1,1,1,1,1,1,1,1,1,1,1,1,1,1,
1,1,1,1,1,1,1,1,1,1,1,1,1,1,6),(2,2),(-1.,-0.971428571428572,-0.942857142857143,
-0.914285714285714,-0.885714285714286,-0.857142857142857,-0.828571428571429,
-0.8,-0.771428571428572,-0.742857142857143,-0.714285714285714,-0.685714285714286,
-0.657142857142857,-0.628571428571429,-0.6,-0.571428571428572,-0.542857142857143,
-0.514285714285714,-0.485714285714286,-0.457142857142857,-0.428571428571429,
-0.4,-0.371428571428571,-0.342857142857143,-0.314285714285714,-0.285714285714286,
-0.257142857142857,-0.228571428571429,-0.2,-0.171428571428571,-0.142857142857143,
-0.114285714285714,-0.0857142857142857,-0.0571428571428571,-0.0285714285714286,
0.),(0.,1.6),.UNSPECIFIED.)
GEOMETRIC_REPRESENTATION_ITEM()
RATIONAL_B_SPLINE_SURFACE(((1.,1.),(1.,1.),(1.,1.),(1.,1.),(1.,1.),(1.,
1.),(1.,1.),(1.,1.),(1.,1.),(1.,1.),(1.,1.),(1.,1.),(1.,1.),(1.,1.),(1.,
1.),(1.,1.),(1.,1.),(1.,1.),(1.,1.),(1.,1.),(1.,1.),(1.,1.),(1.,1.),(1.,
1.),(1.,1.),(1.,1.),(1.,1.),(1.,1.),(1.,1.),(1.,1.),(1.,1.),(1.,1.),(1.,
1.),(1.,1.),(1.,1.),(1.,1.),(1.,1.),(1.,1.),(1.,1.),(1.,1.)))
REPRESENTATION_ITEM('')
SURFACE()
);
#567=(
BOUNDED_SURFACE()
B_SPLINE_SURFACE(5,1,((#57697,#57698),(#57699,#57700),(#57701,#57702),(#57703,
#57704),(#57705,#57706),(#57707,#57708),(#57709,#57710),(#57711,#57712),
(#57713,#57714),(#57715,#57716),(#57717,#57718),(#57719,#57720),(#57721,
#57722),(#57723,#57724),(#57725,#57726),(#57727,#57728),(#57729,#57730),
(#57731,#57732),(#57733,#57734),(#57735,#57736),(#57737,#57738),(#57739,
#57740),(#57741,#57742),(#57743,#57744),(#57745,#57746),(#57747,#57748),
(#57749,#57750),(#57751,#57752),(#57753,#57754),(#57755,#57756),(#57757,
#57758),(#57759,#57760),(#57761,#57762),(#57763,#57764),(#57765,#57766),
(#57767,#57768),(#57769,#57770),(#57771,#57772),(#57773,#57774),(#57775,
#57776)),.UNSPECIFIED.,.F.,.F.,.F.)
B_SPLINE_SURFACE_WITH_KNOTS((6,1,1,1,1,1,1,1,1,1,1,1,1,1,1,1,1,1,1,1,1,
1,1,1,1,1,1,1,1,1,1,1,1,1,1,6),(2,2),(-1.,-0.971428571428572,-0.942857142857143,
-0.914285714285714,-0.885714285714286,-0.857142857142857,-0.828571428571429,
-0.8,-0.771428571428572,-0.742857142857143,-0.714285714285714,-0.685714285714286,
-0.657142857142857,-0.628571428571429,-0.6,-0.571428571428572,-0.542857142857143,
-0.514285714285714,-0.485714285714286,-0.457142857142857,-0.428571428571429,
-0.4,-0.371428571428571,-0.342857142857143,-0.314285714285714,-0.285714285714286,
-0.257142857142857,-0.228571428571429,-0.2,-0.171428571428571,-0.142857142857143,
-0.114285714285714,-0.0857142857142857,-0.0571428571428571,-0.0285714285714286,
0.),(0.,1.6),.UNSPECIFIED.)
GEOMETRIC_REPRESENTATION_ITEM()
RATIONAL_B_SPLINE_SURFACE(((1.,1.),(1.,1.),(1.,1.),(1.,1.),(1.,1.),(1.,
1.),(1.,1.),(1.,1.),(1.,1.),(1.,1.),(1.,1.),(1.,1.),(1.,1.),(1.,1.),(1.,
1.),(1.,1.),(1.,1.),(1.,1.),(1.,1.),(1.,1.),(1.,1.),(1.,1.),(1.,1.),(1.,
1.),(1.,1.),(1.,1.),(1.,1.),(1.,1.),(1.,1.),(1.,1.),(1.,1.),(1.,1.),(1.,
1.),(1.,1.),(1.,1.),(1.,1.),(1.,1.),(1.,1.),(1.,1.),(1.,1.)))
REPRESENTATION_ITEM('')
SURFACE()
);
#568=(
BOUNDED_SURFACE()
B_SPLINE_SURFACE(5,1,((#57796,#57797),(#57798,#57799),(#57800,#57801),(#57802,
#57803),(#57804,#57805),(#57806,#57807),(#57808,#57809),(#57810,#57811),
(#57812,#57813),(#57814,#57815),(#57816,#57817),(#57818,#57819),(#57820,
#57821),(#57822,#57823),(#57824,#57825),(#57826,#57827),(#57828,#57829),
(#57830,#57831),(#57832,#57833),(#57834,#57835),(#57836,#57837),(#57838,
#57839),(#57840,#57841),(#57842,#57843),(#57844,#57845),(#57846,#57847),
(#57848,#57849),(#57850,#57851),(#57852,#57853),(#57854,#57855),(#57856,
#57857),(#57858,#57859),(#57860,#57861),(#57862,#57863),(#57864,#57865),
(#57866,#57867),(#57868,#57869),(#57870,#57871),(#57872,#57873),(#57874,
#57875)),.UNSPECIFIED.,.F.,.F.,.F.)
B_SPLINE_SURFACE_WITH_KNOTS((6,1,1,1,1,1,1,1,1,1,1,1,1,1,1,1,1,1,1,1,1,
1,1,1,1,1,1,1,1,1,1,1,1,1,1,6),(2,2),(-1.,-0.971428571428572,-0.942857142857143,
-0.914285714285714,-0.885714285714286,-0.857142857142857,-0.828571428571429,
-0.8,-0.771428571428572,-0.742857142857143,-0.714285714285714,-0.685714285714286,
-0.657142857142857,-0.628571428571429,-0.6,-0.571428571428572,-0.542857142857143,
-0.514285714285714,-0.485714285714286,-0.457142857142857,-0.428571428571429,
-0.4,-0.371428571428571,-0.342857142857143,-0.314285714285714,-0.285714285714286,
-0.257142857142857,-0.228571428571429,-0.2,-0.171428571428571,-0.142857142857143,
-0.114285714285714,-0.0857142857142857,-0.0571428571428571,-0.0285714285714286,
0.),(0.,1.6),.UNSPECIFIED.)
GEOMETRIC_REPRESENTATION_ITEM()
RATIONAL_B_SPLINE_SURFACE(((1.,1.),(1.,1.),(1.,1.),(1.,1.),(1.,1.),(1.,
1.),(1.,1.),(1.,1.),(1.,1.),(1.,1.),(1.,1.),(1.,1.),(1.,1.),(1.,1.),(1.,
1.),(1.,1.),(1.,1.),(1.,1.),(1.,1.),(1.,1.),(1.,1.),(1.,1.),(1.,1.),(1.,
1.),(1.,1.),(1.,1.),(1.,1.),(1.,1.),(1.,1.),(1.,1.),(1.,1.),(1.,1.),(1.,
1.),(1.,1.),(1.,1.),(1.,1.),(1.,1.),(1.,1.),(1.,1.),(1.,1.)))
REPRESENTATION_ITEM('')
SURFACE()
);
#569=(
BOUNDED_SURFACE()
B_SPLINE_SURFACE(5,1,((#57895,#57896),(#57897,#57898),(#57899,#57900),(#57901,
#57902),(#57903,#57904),(#57905,#57906),(#57907,#57908),(#57909,#57910),
(#57911,#57912),(#57913,#57914),(#57915,#57916),(#57917,#57918),(#57919,
#57920),(#57921,#57922),(#57923,#57924),(#57925,#57926),(#57927,#57928),
(#57929,#57930),(#57931,#57932),(#57933,#57934),(#57935,#57936),(#57937,
#57938),(#57939,#57940),(#57941,#57942),(#57943,#57944),(#57945,#57946),
(#57947,#57948),(#57949,#57950),(#57951,#57952),(#57953,#57954),(#57955,
#57956),(#57957,#57958),(#57959,#57960),(#57961,#57962),(#57963,#57964),
(#57965,#57966),(#57967,#57968),(#57969,#57970),(#57971,#57972),(#57973,
#57974)),.UNSPECIFIED.,.F.,.F.,.F.)
B_SPLINE_SURFACE_WITH_KNOTS((6,1,1,1,1,1,1,1,1,1,1,1,1,1,1,1,1,1,1,1,1,
1,1,1,1,1,1,1,1,1,1,1,1,1,1,6),(2,2),(-1.,-0.971428571428572,-0.942857142857143,
-0.914285714285714,-0.885714285714286,-0.857142857142857,-0.828571428571429,
-0.8,-0.771428571428572,-0.742857142857143,-0.714285714285714,-0.685714285714286,
-0.657142857142857,-0.628571428571429,-0.6,-0.571428571428572,-0.542857142857143,
-0.514285714285714,-0.485714285714286,-0.457142857142857,-0.428571428571429,
-0.4,-0.371428571428571,-0.342857142857143,-0.314285714285714,-0.285714285714286,
-0.257142857142857,-0.228571428571429,-0.2,-0.171428571428571,-0.142857142857143,
-0.114285714285714,-0.0857142857142857,-0.0571428571428571,-0.0285714285714286,
0.),(0.,1.6),.UNSPECIFIED.)
GEOMETRIC_REPRESENTATION_ITEM()
RATIONAL_B_SPLINE_SURFACE(((1.,1.),(1.,1.),(1.,1.),(1.,1.),(1.,1.),(1.,
1.),(1.,1.),(1.,1.),(1.,1.),(1.,1.),(1.,1.),(1.,1.),(1.,1.),(1.,1.),(1.,
1.),(1.,1.),(1.,1.),(1.,1.),(1.,1.),(1.,1.),(1.,1.),(1.,1.),(1.,1.),(1.,
1.),(1.,1.),(1.,1.),(1.,1.),(1.,1.),(1.,1.),(1.,1.),(1.,1.),(1.,1.),(1.,
1.),(1.,1.),(1.,1.),(1.,1.),(1.,1.),(1.,1.),(1.,1.),(1.,1.)))
REPRESENTATION_ITEM('')
SURFACE()
);
#570=(
BOUNDED_SURFACE()
B_SPLINE_SURFACE(5,1,((#58006,#58007),(#58008,#58009),(#58010,#58011),(#58012,
#58013),(#58014,#58015),(#58016,#58017),(#58018,#58019),(#58020,#58021),
(#58022,#58023),(#58024,#58025),(#58026,#58027),(#58028,#58029),(#58030,
#58031),(#58032,#58033),(#58034,#58035),(#58036,#58037),(#58038,#58039),
(#58040,#58041),(#58042,#58043),(#58044,#58045),(#58046,#58047),(#58048,
#58049),(#58050,#58051),(#58052,#58053),(#58054,#58055),(#58056,#58057),
(#58058,#58059),(#58060,#58061),(#58062,#58063),(#58064,#58065),(#58066,
#58067),(#58068,#58069),(#58070,#58071),(#58072,#58073),(#58074,#58075),
(#58076,#58077),(#58078,#58079),(#58080,#58081),(#58082,#58083),(#58084,
#58085)),.UNSPECIFIED.,.F.,.F.,.F.)
B_SPLINE_SURFACE_WITH_KNOTS((6,1,1,1,1,1,1,1,1,1,1,1,1,1,1,1,1,1,1,1,1,
1,1,1,1,1,1,1,1,1,1,1,1,1,1,6),(2,2),(-1.,-0.971428571428572,-0.942857142857143,
-0.914285714285714,-0.885714285714286,-0.857142857142857,-0.828571428571429,
-0.8,-0.771428571428572,-0.742857142857143,-0.714285714285714,-0.685714285714286,
-0.657142857142857,-0.628571428571429,-0.6,-0.571428571428572,-0.542857142857143,
-0.514285714285714,-0.485714285714286,-0.457142857142857,-0.428571428571429,
-0.4,-0.371428571428571,-0.342857142857143,-0.314285714285714,-0.285714285714286,
-0.257142857142857,-0.228571428571429,-0.2,-0.171428571428571,-0.142857142857143,
-0.114285714285714,-0.0857142857142857,-0.0571428571428571,-0.0285714285714286,
0.),(0.,1.6),.UNSPECIFIED.)
GEOMETRIC_REPRESENTATION_ITEM()
RATIONAL_B_SPLINE_SURFACE(((1.,1.),(1.,1.),(1.,1.),(1.,1.),(1.,1.),(1.,
1.),(1.,1.),(1.,1.),(1.,1.),(1.,1.),(1.,1.),(1.,1.),(1.,1.),(1.,1.),(1.,
1.),(1.,1.),(1.,1.),(1.,1.),(1.,1.),(1.,1.),(1.,1.),(1.,1.),(1.,1.),(1.,
1.),(1.,1.),(1.,1.),(1.,1.),(1.,1.),(1.,1.),(1.,1.),(1.,1.),(1.,1.),(1.,
1.),(1.,1.),(1.,1.),(1.,1.),(1.,1.),(1.,1.),(1.,1.),(1.,1.)))
REPRESENTATION_ITEM('')
SURFACE()
);
#571=(
BOUNDED_SURFACE()
B_SPLINE_SURFACE(5,1,((#58120,#58121),(#58122,#58123),(#58124,#58125),(#58126,
#58127),(#58128,#58129),(#58130,#58131),(#58132,#58133),(#58134,#58135),
(#58136,#58137),(#58138,#58139),(#58140,#58141),(#58142,#58143),(#58144,
#58145),(#58146,#58147),(#58148,#58149),(#58150,#58151),(#58152,#58153),
(#58154,#58155),(#58156,#58157),(#58158,#58159),(#58160,#58161),(#58162,
#58163),(#58164,#58165),(#58166,#58167),(#58168,#58169),(#58170,#58171),
(#58172,#58173),(#58174,#58175),(#58176,#58177),(#58178,#58179),(#58180,
#58181),(#58182,#58183),(#58184,#58185),(#58186,#58187),(#58188,#58189),
(#58190,#58191),(#58192,#58193),(#58194,#58195),(#58196,#58197),(#58198,
#58199)),.UNSPECIFIED.,.F.,.F.,.F.)
B_SPLINE_SURFACE_WITH_KNOTS((6,1,1,1,1,1,1,1,1,1,1,1,1,1,1,1,1,1,1,1,1,
1,1,1,1,1,1,1,1,1,1,1,1,1,1,6),(2,2),(-1.,-0.971428571428572,-0.942857142857143,
-0.914285714285714,-0.885714285714286,-0.857142857142857,-0.828571428571429,
-0.8,-0.771428571428572,-0.742857142857143,-0.714285714285714,-0.685714285714286,
-0.657142857142857,-0.628571428571429,-0.6,-0.571428571428572,-0.542857142857143,
-0.514285714285714,-0.485714285714286,-0.457142857142857,-0.428571428571429,
-0.4,-0.371428571428571,-0.342857142857143,-0.314285714285714,-0.285714285714286,
-0.257142857142857,-0.228571428571429,-0.2,-0.171428571428571,-0.142857142857143,
-0.114285714285714,-0.0857142857142857,-0.0571428571428571,-0.0285714285714286,
0.),(0.,1.6),.UNSPECIFIED.)
GEOMETRIC_REPRESENTATION_ITEM()
RATIONAL_B_SPLINE_SURFACE(((1.,1.),(1.,1.),(1.,1.),(1.,1.),(1.,1.),(1.,
1.),(1.,1.),(1.,1.),(1.,1.),(1.,1.),(1.,1.),(1.,1.),(1.,1.),(1.,1.),(1.,
1.),(1.,1.),(1.,1.),(1.,1.),(1.,1.),(1.,1.),(1.,1.),(1.,1.),(1.,1.),(1.,
1.),(1.,1.),(1.,1.),(1.,1.),(1.,1.),(1.,1.),(1.,1.),(1.,1.),(1.,1.),(1.,
1.),(1.,1.),(1.,1.),(1.,1.),(1.,1.),(1.,1.),(1.,1.),(1.,1.)))
REPRESENTATION_ITEM('')
SURFACE()
);
#572=(
BOUNDED_SURFACE()
B_SPLINE_SURFACE(5,1,((#58219,#58220),(#58221,#58222),(#58223,#58224),(#58225,
#58226),(#58227,#58228),(#58229,#58230),(#58231,#58232),(#58233,#58234),
(#58235,#58236),(#58237,#58238),(#58239,#58240),(#58241,#58242),(#58243,
#58244),(#58245,#58246),(#58247,#58248),(#58249,#58250),(#58251,#58252),
(#58253,#58254),(#58255,#58256),(#58257,#58258),(#58259,#58260),(#58261,
#58262),(#58263,#58264),(#58265,#58266),(#58267,#58268),(#58269,#58270),
(#58271,#58272),(#58273,#58274),(#58275,#58276),(#58277,#58278),(#58279,
#58280),(#58281,#58282),(#58283,#58284),(#58285,#58286),(#58287,#58288),
(#58289,#58290),(#58291,#58292),(#58293,#58294),(#58295,#58296),(#58297,
#58298)),.UNSPECIFIED.,.F.,.F.,.F.)
B_SPLINE_SURFACE_WITH_KNOTS((6,1,1,1,1,1,1,1,1,1,1,1,1,1,1,1,1,1,1,1,1,
1,1,1,1,1,1,1,1,1,1,1,1,1,1,6),(2,2),(-1.,-0.971428571428572,-0.942857142857143,
-0.914285714285714,-0.885714285714286,-0.857142857142857,-0.828571428571429,
-0.8,-0.771428571428572,-0.742857142857143,-0.714285714285714,-0.685714285714286,
-0.657142857142857,-0.628571428571429,-0.6,-0.571428571428572,-0.542857142857143,
-0.514285714285714,-0.485714285714286,-0.457142857142857,-0.428571428571429,
-0.4,-0.371428571428571,-0.342857142857143,-0.314285714285714,-0.285714285714286,
-0.257142857142857,-0.228571428571429,-0.2,-0.171428571428571,-0.142857142857143,
-0.114285714285714,-0.0857142857142857,-0.0571428571428571,-0.0285714285714286,
0.),(0.,1.6),.UNSPECIFIED.)
GEOMETRIC_REPRESENTATION_ITEM()
RATIONAL_B_SPLINE_SURFACE(((1.,1.),(1.,1.),(1.,1.),(1.,1.),(1.,1.),(1.,
1.),(1.,1.),(1.,1.),(1.,1.),(1.,1.),(1.,1.),(1.,1.),(1.,1.),(1.,1.),(1.,
1.),(1.,1.),(1.,1.),(1.,1.),(1.,1.),(1.,1.),(1.,1.),(1.,1.),(1.,1.),(1.,
1.),(1.,1.),(1.,1.),(1.,1.),(1.,1.),(1.,1.),(1.,1.),(1.,1.),(1.,1.),(1.,
1.),(1.,1.),(1.,1.),(1.,1.),(1.,1.),(1.,1.),(1.,1.),(1.,1.)))
REPRESENTATION_ITEM('')
SURFACE()
);
#573=(
BOUNDED_SURFACE()
B_SPLINE_SURFACE(5,1,((#58318,#58319),(#58320,#58321),(#58322,#58323),(#58324,
#58325),(#58326,#58327),(#58328,#58329),(#58330,#58331),(#58332,#58333),
(#58334,#58335),(#58336,#58337),(#58338,#58339),(#58340,#58341),(#58342,
#58343),(#58344,#58345),(#58346,#58347),(#58348,#58349),(#58350,#58351),
(#58352,#58353),(#58354,#58355),(#58356,#58357),(#58358,#58359),(#58360,
#58361),(#58362,#58363),(#58364,#58365),(#58366,#58367),(#58368,#58369),
(#58370,#58371),(#58372,#58373),(#58374,#58375),(#58376,#58377),(#58378,
#58379),(#58380,#58381),(#58382,#58383),(#58384,#58385),(#58386,#58387),
(#58388,#58389),(#58390,#58391),(#58392,#58393),(#58394,#58395),(#58396,
#58397)),.UNSPECIFIED.,.F.,.F.,.F.)
B_SPLINE_SURFACE_WITH_KNOTS((6,1,1,1,1,1,1,1,1,1,1,1,1,1,1,1,1,1,1,1,1,
1,1,1,1,1,1,1,1,1,1,1,1,1,1,6),(2,2),(-1.,-0.971428571428572,-0.942857142857143,
-0.914285714285714,-0.885714285714286,-0.857142857142857,-0.828571428571429,
-0.8,-0.771428571428572,-0.742857142857143,-0.714285714285714,-0.685714285714286,
-0.657142857142857,-0.628571428571429,-0.6,-0.571428571428572,-0.542857142857143,
-0.514285714285714,-0.485714285714286,-0.457142857142857,-0.428571428571429,
-0.4,-0.371428571428571,-0.342857142857143,-0.314285714285714,-0.285714285714286,
-0.257142857142857,-0.228571428571429,-0.2,-0.171428571428571,-0.142857142857143,
-0.114285714285714,-0.0857142857142857,-0.0571428571428571,-0.0285714285714286,
0.),(0.,1.6),.UNSPECIFIED.)
GEOMETRIC_REPRESENTATION_ITEM()
RATIONAL_B_SPLINE_SURFACE(((1.,1.),(1.,1.),(1.,1.),(1.,1.),(1.,1.),(1.,
1.),(1.,1.),(1.,1.),(1.,1.),(1.,1.),(1.,1.),(1.,1.),(1.,1.),(1.,1.),(1.,
1.),(1.,1.),(1.,1.),(1.,1.),(1.,1.),(1.,1.),(1.,1.),(1.,1.),(1.,1.),(1.,
1.),(1.,1.),(1.,1.),(1.,1.),(1.,1.),(1.,1.),(1.,1.),(1.,1.),(1.,1.),(1.,
1.),(1.,1.),(1.,1.),(1.,1.),(1.,1.),(1.,1.),(1.,1.),(1.,1.)))
REPRESENTATION_ITEM('')
SURFACE()
);
#574=(
BOUNDED_SURFACE()
B_SPLINE_SURFACE(5,1,((#58417,#58418),(#58419,#58420),(#58421,#58422),(#58423,
#58424),(#58425,#58426),(#58427,#58428),(#58429,#58430),(#58431,#58432),
(#58433,#58434),(#58435,#58436),(#58437,#58438),(#58439,#58440),(#58441,
#58442),(#58443,#58444),(#58445,#58446),(#58447,#58448),(#58449,#58450),
(#58451,#58452),(#58453,#58454),(#58455,#58456),(#58457,#58458),(#58459,
#58460),(#58461,#58462),(#58463,#58464),(#58465,#58466),(#58467,#58468),
(#58469,#58470),(#58471,#58472),(#58473,#58474),(#58475,#58476),(#58477,
#58478),(#58479,#58480),(#58481,#58482),(#58483,#58484),(#58485,#58486),
(#58487,#58488),(#58489,#58490),(#58491,#58492),(#58493,#58494),(#58495,
#58496)),.UNSPECIFIED.,.F.,.F.,.F.)
B_SPLINE_SURFACE_WITH_KNOTS((6,1,1,1,1,1,1,1,1,1,1,1,1,1,1,1,1,1,1,1,1,
1,1,1,1,1,1,1,1,1,1,1,1,1,1,6),(2,2),(-1.,-0.971428571428572,-0.942857142857143,
-0.914285714285714,-0.885714285714286,-0.857142857142857,-0.828571428571429,
-0.8,-0.771428571428572,-0.742857142857143,-0.714285714285714,-0.685714285714286,
-0.657142857142857,-0.628571428571429,-0.6,-0.571428571428572,-0.542857142857143,
-0.514285714285714,-0.485714285714286,-0.457142857142857,-0.428571428571429,
-0.4,-0.371428571428571,-0.342857142857143,-0.314285714285714,-0.285714285714286,
-0.257142857142857,-0.228571428571429,-0.2,-0.171428571428571,-0.142857142857143,
-0.114285714285714,-0.0857142857142857,-0.0571428571428571,-0.0285714285714286,
0.),(0.,1.6),.UNSPECIFIED.)
GEOMETRIC_REPRESENTATION_ITEM()
RATIONAL_B_SPLINE_SURFACE(((1.,1.),(1.,1.),(1.,1.),(1.,1.),(1.,1.),(1.,
1.),(1.,1.),(1.,1.),(1.,1.),(1.,1.),(1.,1.),(1.,1.),(1.,1.),(1.,1.),(1.,
1.),(1.,1.),(1.,1.),(1.,1.),(1.,1.),(1.,1.),(1.,1.),(1.,1.),(1.,1.),(1.,
1.),(1.,1.),(1.,1.),(1.,1.),(1.,1.),(1.,1.),(1.,1.),(1.,1.),(1.,1.),(1.,
1.),(1.,1.),(1.,1.),(1.,1.),(1.,1.),(1.,1.),(1.,1.),(1.,1.)))
REPRESENTATION_ITEM('')
SURFACE()
);
#575=(
BOUNDED_SURFACE()
B_SPLINE_SURFACE(5,1,((#58516,#58517),(#58518,#58519),(#58520,#58521),(#58522,
#58523),(#58524,#58525),(#58526,#58527),(#58528,#58529),(#58530,#58531),
(#58532,#58533),(#58534,#58535),(#58536,#58537),(#58538,#58539),(#58540,
#58541),(#58542,#58543),(#58544,#58545),(#58546,#58547),(#58548,#58549),
(#58550,#58551),(#58552,#58553),(#58554,#58555),(#58556,#58557),(#58558,
#58559),(#58560,#58561),(#58562,#58563),(#58564,#58565),(#58566,#58567),
(#58568,#58569),(#58570,#58571),(#58572,#58573),(#58574,#58575),(#58576,
#58577),(#58578,#58579),(#58580,#58581),(#58582,#58583),(#58584,#58585),
(#58586,#58587),(#58588,#58589),(#58590,#58591),(#58592,#58593),(#58594,
#58595)),.UNSPECIFIED.,.F.,.F.,.F.)
B_SPLINE_SURFACE_WITH_KNOTS((6,1,1,1,1,1,1,1,1,1,1,1,1,1,1,1,1,1,1,1,1,
1,1,1,1,1,1,1,1,1,1,1,1,1,1,6),(2,2),(-1.,-0.971428571428572,-0.942857142857143,
-0.914285714285714,-0.885714285714286,-0.857142857142857,-0.828571428571429,
-0.8,-0.771428571428572,-0.742857142857143,-0.714285714285714,-0.685714285714286,
-0.657142857142857,-0.628571428571429,-0.6,-0.571428571428572,-0.542857142857143,
-0.514285714285714,-0.485714285714286,-0.457142857142857,-0.428571428571429,
-0.4,-0.371428571428571,-0.342857142857143,-0.314285714285714,-0.285714285714286,
-0.257142857142857,-0.228571428571429,-0.2,-0.171428571428571,-0.142857142857143,
-0.114285714285714,-0.0857142857142857,-0.0571428571428571,-0.0285714285714286,
0.),(0.,1.6),.UNSPECIFIED.)
GEOMETRIC_REPRESENTATION_ITEM()
RATIONAL_B_SPLINE_SURFACE(((1.,1.),(1.,1.),(1.,1.),(1.,1.),(1.,1.),(1.,
1.),(1.,1.),(1.,1.),(1.,1.),(1.,1.),(1.,1.),(1.,1.),(1.,1.),(1.,1.),(1.,
1.),(1.,1.),(1.,1.),(1.,1.),(1.,1.),(1.,1.),(1.,1.),(1.,1.),(1.,1.),(1.,
1.),(1.,1.),(1.,1.),(1.,1.),(1.,1.),(1.,1.),(1.,1.),(1.,1.),(1.,1.),(1.,
1.),(1.,1.),(1.,1.),(1.,1.),(1.,1.),(1.,1.),(1.,1.),(1.,1.)))
REPRESENTATION_ITEM('')
SURFACE()
);
#576=(
BOUNDED_SURFACE()
B_SPLINE_SURFACE(5,1,((#58615,#58616),(#58617,#58618),(#58619,#58620),(#58621,
#58622),(#58623,#58624),(#58625,#58626),(#58627,#58628),(#58629,#58630),
(#58631,#58632),(#58633,#58634),(#58635,#58636),(#58637,#58638),(#58639,
#58640),(#58641,#58642),(#58643,#58644),(#58645,#58646),(#58647,#58648),
(#58649,#58650),(#58651,#58652),(#58653,#58654),(#58655,#58656),(#58657,
#58658),(#58659,#58660),(#58661,#58662),(#58663,#58664),(#58665,#58666),
(#58667,#58668),(#58669,#58670),(#58671,#58672),(#58673,#58674),(#58675,
#58676),(#58677,#58678),(#58679,#58680),(#58681,#58682),(#58683,#58684),
(#58685,#58686),(#58687,#58688),(#58689,#58690),(#58691,#58692),(#58693,
#58694)),.UNSPECIFIED.,.F.,.F.,.F.)
B_SPLINE_SURFACE_WITH_KNOTS((6,1,1,1,1,1,1,1,1,1,1,1,1,1,1,1,1,1,1,1,1,
1,1,1,1,1,1,1,1,1,1,1,1,1,1,6),(2,2),(-1.,-0.971428571428572,-0.942857142857143,
-0.914285714285714,-0.885714285714286,-0.857142857142857,-0.828571428571429,
-0.8,-0.771428571428572,-0.742857142857143,-0.714285714285714,-0.685714285714286,
-0.657142857142857,-0.628571428571429,-0.6,-0.571428571428572,-0.542857142857143,
-0.514285714285714,-0.485714285714286,-0.457142857142857,-0.428571428571429,
-0.4,-0.371428571428571,-0.342857142857143,-0.314285714285714,-0.285714285714286,
-0.257142857142857,-0.228571428571429,-0.2,-0.171428571428571,-0.142857142857143,
-0.114285714285714,-0.0857142857142857,-0.0571428571428571,-0.0285714285714286,
0.),(0.,1.6),.UNSPECIFIED.)
GEOMETRIC_REPRESENTATION_ITEM()
RATIONAL_B_SPLINE_SURFACE(((1.,1.),(1.,1.),(1.,1.),(1.,1.),(1.,1.),(1.,
1.),(1.,1.),(1.,1.),(1.,1.),(1.,1.),(1.,1.),(1.,1.),(1.,1.),(1.,1.),(1.,
1.),(1.,1.),(1.,1.),(1.,1.),(1.,1.),(1.,1.),(1.,1.),(1.,1.),(1.,1.),(1.,
1.),(1.,1.),(1.,1.),(1.,1.),(1.,1.),(1.,1.),(1.,1.),(1.,1.),(1.,1.),(1.,
1.),(1.,1.),(1.,1.),(1.,1.),(1.,1.),(1.,1.),(1.,1.),(1.,1.)))
REPRESENTATION_ITEM('')
SURFACE()
);
#577=(
BOUNDED_SURFACE()
B_SPLINE_SURFACE(5,1,((#58714,#58715),(#58716,#58717),(#58718,#58719),(#58720,
#58721),(#58722,#58723),(#58724,#58725),(#58726,#58727),(#58728,#58729),
(#58730,#58731),(#58732,#58733),(#58734,#58735),(#58736,#58737),(#58738,
#58739),(#58740,#58741),(#58742,#58743),(#58744,#58745),(#58746,#58747),
(#58748,#58749),(#58750,#58751),(#58752,#58753),(#58754,#58755),(#58756,
#58757),(#58758,#58759),(#58760,#58761),(#58762,#58763),(#58764,#58765),
(#58766,#58767),(#58768,#58769),(#58770,#58771),(#58772,#58773),(#58774,
#58775),(#58776,#58777),(#58778,#58779),(#58780,#58781),(#58782,#58783),
(#58784,#58785),(#58786,#58787),(#58788,#58789),(#58790,#58791),(#58792,
#58793)),.UNSPECIFIED.,.F.,.F.,.F.)
B_SPLINE_SURFACE_WITH_KNOTS((6,1,1,1,1,1,1,1,1,1,1,1,1,1,1,1,1,1,1,1,1,
1,1,1,1,1,1,1,1,1,1,1,1,1,1,6),(2,2),(-1.,-0.971428571428572,-0.942857142857143,
-0.914285714285714,-0.885714285714286,-0.857142857142857,-0.828571428571429,
-0.8,-0.771428571428572,-0.742857142857143,-0.714285714285714,-0.685714285714286,
-0.657142857142857,-0.628571428571429,-0.6,-0.571428571428572,-0.542857142857143,
-0.514285714285714,-0.485714285714286,-0.457142857142857,-0.428571428571429,
-0.4,-0.371428571428571,-0.342857142857143,-0.314285714285714,-0.285714285714286,
-0.257142857142857,-0.228571428571429,-0.2,-0.171428571428571,-0.142857142857143,
-0.114285714285714,-0.0857142857142857,-0.0571428571428571,-0.0285714285714286,
0.),(0.,1.6),.UNSPECIFIED.)
GEOMETRIC_REPRESENTATION_ITEM()
RATIONAL_B_SPLINE_SURFACE(((1.,1.),(1.,1.),(1.,1.),(1.,1.),(1.,1.),(1.,
1.),(1.,1.),(1.,1.),(1.,1.),(1.,1.),(1.,1.),(1.,1.),(1.,1.),(1.,1.),(1.,
1.),(1.,1.),(1.,1.),(1.,1.),(1.,1.),(1.,1.),(1.,1.),(1.,1.),(1.,1.),(1.,
1.),(1.,1.),(1.,1.),(1.,1.),(1.,1.),(1.,1.),(1.,1.),(1.,1.),(1.,1.),(1.,
1.),(1.,1.),(1.,1.),(1.,1.),(1.,1.),(1.,1.),(1.,1.),(1.,1.)))
REPRESENTATION_ITEM('')
SURFACE()
);
#578=(
BOUNDED_SURFACE()
B_SPLINE_SURFACE(5,1,((#58813,#58814),(#58815,#58816),(#58817,#58818),(#58819,
#58820),(#58821,#58822),(#58823,#58824),(#58825,#58826),(#58827,#58828),
(#58829,#58830),(#58831,#58832),(#58833,#58834),(#58835,#58836),(#58837,
#58838),(#58839,#58840),(#58841,#58842),(#58843,#58844),(#58845,#58846),
(#58847,#58848),(#58849,#58850),(#58851,#58852),(#58853,#58854),(#58855,
#58856),(#58857,#58858),(#58859,#58860),(#58861,#58862),(#58863,#58864),
(#58865,#58866),(#58867,#58868),(#58869,#58870),(#58871,#58872),(#58873,
#58874),(#58875,#58876),(#58877,#58878),(#58879,#58880),(#58881,#58882),
(#58883,#58884),(#58885,#58886),(#58887,#58888),(#58889,#58890),(#58891,
#58892)),.UNSPECIFIED.,.F.,.F.,.F.)
B_SPLINE_SURFACE_WITH_KNOTS((6,1,1,1,1,1,1,1,1,1,1,1,1,1,1,1,1,1,1,1,1,
1,1,1,1,1,1,1,1,1,1,1,1,1,1,6),(2,2),(-1.,-0.971428571428572,-0.942857142857143,
-0.914285714285714,-0.885714285714286,-0.857142857142857,-0.828571428571429,
-0.8,-0.771428571428572,-0.742857142857143,-0.714285714285714,-0.685714285714286,
-0.657142857142857,-0.628571428571429,-0.6,-0.571428571428572,-0.542857142857143,
-0.514285714285714,-0.485714285714286,-0.457142857142857,-0.428571428571429,
-0.4,-0.371428571428571,-0.342857142857143,-0.314285714285714,-0.285714285714286,
-0.257142857142857,-0.228571428571429,-0.2,-0.171428571428571,-0.142857142857143,
-0.114285714285714,-0.0857142857142857,-0.0571428571428571,-0.0285714285714286,
0.),(0.,1.6),.UNSPECIFIED.)
GEOMETRIC_REPRESENTATION_ITEM()
RATIONAL_B_SPLINE_SURFACE(((1.,1.),(1.,1.),(1.,1.),(1.,1.),(1.,1.),(1.,
1.),(1.,1.),(1.,1.),(1.,1.),(1.,1.),(1.,1.),(1.,1.),(1.,1.),(1.,1.),(1.,
1.),(1.,1.),(1.,1.),(1.,1.),(1.,1.),(1.,1.),(1.,1.),(1.,1.),(1.,1.),(1.,
1.),(1.,1.),(1.,1.),(1.,1.),(1.,1.),(1.,1.),(1.,1.),(1.,1.),(1.,1.),(1.,
1.),(1.,1.),(1.,1.),(1.,1.),(1.,1.),(1.,1.),(1.,1.),(1.,1.)))
REPRESENTATION_ITEM('')
SURFACE()
);
#579=(
BOUNDED_SURFACE()
B_SPLINE_SURFACE(5,1,((#58912,#58913),(#58914,#58915),(#58916,#58917),(#58918,
#58919),(#58920,#58921),(#58922,#58923),(#58924,#58925),(#58926,#58927),
(#58928,#58929),(#58930,#58931),(#58932,#58933),(#58934,#58935),(#58936,
#58937),(#58938,#58939),(#58940,#58941),(#58942,#58943),(#58944,#58945),
(#58946,#58947),(#58948,#58949),(#58950,#58951),(#58952,#58953),(#58954,
#58955),(#58956,#58957),(#58958,#58959),(#58960,#58961),(#58962,#58963),
(#58964,#58965),(#58966,#58967),(#58968,#58969),(#58970,#58971),(#58972,
#58973),(#58974,#58975),(#58976,#58977),(#58978,#58979),(#58980,#58981),
(#58982,#58983),(#58984,#58985),(#58986,#58987),(#58988,#58989),(#58990,
#58991)),.UNSPECIFIED.,.F.,.F.,.F.)
B_SPLINE_SURFACE_WITH_KNOTS((6,1,1,1,1,1,1,1,1,1,1,1,1,1,1,1,1,1,1,1,1,
1,1,1,1,1,1,1,1,1,1,1,1,1,1,6),(2,2),(-1.,-0.971428571428572,-0.942857142857143,
-0.914285714285714,-0.885714285714286,-0.857142857142857,-0.828571428571429,
-0.8,-0.771428571428572,-0.742857142857143,-0.714285714285714,-0.685714285714286,
-0.657142857142857,-0.628571428571429,-0.6,-0.571428571428572,-0.542857142857143,
-0.514285714285714,-0.485714285714286,-0.457142857142857,-0.428571428571429,
-0.4,-0.371428571428571,-0.342857142857143,-0.314285714285714,-0.285714285714286,
-0.257142857142857,-0.228571428571429,-0.2,-0.171428571428571,-0.142857142857143,
-0.114285714285714,-0.0857142857142857,-0.0571428571428571,-0.0285714285714286,
0.),(0.,1.6),.UNSPECIFIED.)
GEOMETRIC_REPRESENTATION_ITEM()
RATIONAL_B_SPLINE_SURFACE(((1.,1.),(1.,1.),(1.,1.),(1.,1.),(1.,1.),(1.,
1.),(1.,1.),(1.,1.),(1.,1.),(1.,1.),(1.,1.),(1.,1.),(1.,1.),(1.,1.),(1.,
1.),(1.,1.),(1.,1.),(1.,1.),(1.,1.),(1.,1.),(1.,1.),(1.,1.),(1.,1.),(1.,
1.),(1.,1.),(1.,1.),(1.,1.),(1.,1.),(1.,1.),(1.,1.),(1.,1.),(1.,1.),(1.,
1.),(1.,1.),(1.,1.),(1.,1.),(1.,1.),(1.,1.),(1.,1.),(1.,1.)))
REPRESENTATION_ITEM('')
SURFACE()
);
#580=(
BOUNDED_SURFACE()
B_SPLINE_SURFACE(5,1,((#59011,#59012),(#59013,#59014),(#59015,#59016),(#59017,
#59018),(#59019,#59020),(#59021,#59022),(#59023,#59024),(#59025,#59026),
(#59027,#59028),(#59029,#59030),(#59031,#59032),(#59033,#59034),(#59035,
#59036),(#59037,#59038),(#59039,#59040),(#59041,#59042),(#59043,#59044),
(#59045,#59046),(#59047,#59048),(#59049,#59050),(#59051,#59052),(#59053,
#59054),(#59055,#59056),(#59057,#59058),(#59059,#59060),(#59061,#59062),
(#59063,#59064),(#59065,#59066),(#59067,#59068),(#59069,#59070),(#59071,
#59072),(#59073,#59074),(#59075,#59076),(#59077,#59078),(#59079,#59080),
(#59081,#59082),(#59083,#59084),(#59085,#59086),(#59087,#59088),(#59089,
#59090)),.UNSPECIFIED.,.F.,.F.,.F.)
B_SPLINE_SURFACE_WITH_KNOTS((6,1,1,1,1,1,1,1,1,1,1,1,1,1,1,1,1,1,1,1,1,
1,1,1,1,1,1,1,1,1,1,1,1,1,1,6),(2,2),(-1.,-0.971428571428572,-0.942857142857143,
-0.914285714285714,-0.885714285714286,-0.857142857142857,-0.828571428571429,
-0.8,-0.771428571428572,-0.742857142857143,-0.714285714285714,-0.685714285714286,
-0.657142857142857,-0.628571428571429,-0.6,-0.571428571428572,-0.542857142857143,
-0.514285714285714,-0.485714285714286,-0.457142857142857,-0.428571428571429,
-0.4,-0.371428571428571,-0.342857142857143,-0.314285714285714,-0.285714285714286,
-0.257142857142857,-0.228571428571429,-0.2,-0.171428571428571,-0.142857142857143,
-0.114285714285714,-0.0857142857142857,-0.0571428571428571,-0.0285714285714286,
0.),(0.,1.6),.UNSPECIFIED.)
GEOMETRIC_REPRESENTATION_ITEM()
RATIONAL_B_SPLINE_SURFACE(((1.,1.),(1.,1.),(1.,1.),(1.,1.),(1.,1.),(1.,
1.),(1.,1.),(1.,1.),(1.,1.),(1.,1.),(1.,1.),(1.,1.),(1.,1.),(1.,1.),(1.,
1.),(1.,1.),(1.,1.),(1.,1.),(1.,1.),(1.,1.),(1.,1.),(1.,1.),(1.,1.),(1.,
1.),(1.,1.),(1.,1.),(1.,1.),(1.,1.),(1.,1.),(1.,1.),(1.,1.),(1.,1.),(1.,
1.),(1.,1.),(1.,1.),(1.,1.),(1.,1.),(1.,1.),(1.,1.),(1.,1.)))
REPRESENTATION_ITEM('')
SURFACE()
);
#581=(
BOUNDED_SURFACE()
B_SPLINE_SURFACE(5,1,((#59110,#59111),(#59112,#59113),(#59114,#59115),(#59116,
#59117),(#59118,#59119),(#59120,#59121),(#59122,#59123),(#59124,#59125),
(#59126,#59127),(#59128,#59129),(#59130,#59131),(#59132,#59133),(#59134,
#59135),(#59136,#59137),(#59138,#59139),(#59140,#59141),(#59142,#59143),
(#59144,#59145),(#59146,#59147),(#59148,#59149),(#59150,#59151),(#59152,
#59153),(#59154,#59155),(#59156,#59157),(#59158,#59159),(#59160,#59161),
(#59162,#59163),(#59164,#59165),(#59166,#59167),(#59168,#59169),(#59170,
#59171),(#59172,#59173),(#59174,#59175),(#59176,#59177),(#59178,#59179),
(#59180,#59181),(#59182,#59183),(#59184,#59185),(#59186,#59187),(#59188,
#59189)),.UNSPECIFIED.,.F.,.F.,.F.)
B_SPLINE_SURFACE_WITH_KNOTS((6,1,1,1,1,1,1,1,1,1,1,1,1,1,1,1,1,1,1,1,1,
1,1,1,1,1,1,1,1,1,1,1,1,1,1,6),(2,2),(-1.,-0.971428571428572,-0.942857142857143,
-0.914285714285714,-0.885714285714286,-0.857142857142857,-0.828571428571429,
-0.8,-0.771428571428572,-0.742857142857143,-0.714285714285714,-0.685714285714286,
-0.657142857142857,-0.628571428571429,-0.6,-0.571428571428572,-0.542857142857143,
-0.514285714285714,-0.485714285714286,-0.457142857142857,-0.428571428571429,
-0.4,-0.371428571428571,-0.342857142857143,-0.314285714285714,-0.285714285714286,
-0.257142857142857,-0.228571428571429,-0.2,-0.171428571428571,-0.142857142857143,
-0.114285714285714,-0.0857142857142857,-0.0571428571428571,-0.0285714285714286,
0.),(0.,1.6),.UNSPECIFIED.)
GEOMETRIC_REPRESENTATION_ITEM()
RATIONAL_B_SPLINE_SURFACE(((1.,1.),(1.,1.),(1.,1.),(1.,1.),(1.,1.),(1.,
1.),(1.,1.),(1.,1.),(1.,1.),(1.,1.),(1.,1.),(1.,1.),(1.,1.),(1.,1.),(1.,
1.),(1.,1.),(1.,1.),(1.,1.),(1.,1.),(1.,1.),(1.,1.),(1.,1.),(1.,1.),(1.,
1.),(1.,1.),(1.,1.),(1.,1.),(1.,1.),(1.,1.),(1.,1.),(1.,1.),(1.,1.),(1.,
1.),(1.,1.),(1.,1.),(1.,1.),(1.,1.),(1.,1.),(1.,1.),(1.,1.)))
REPRESENTATION_ITEM('')
SURFACE()
);
#582=(
BOUNDED_SURFACE()
B_SPLINE_SURFACE(5,1,((#59221,#59222),(#59223,#59224),(#59225,#59226),(#59227,
#59228),(#59229,#59230),(#59231,#59232),(#59233,#59234),(#59235,#59236),
(#59237,#59238),(#59239,#59240),(#59241,#59242),(#59243,#59244),(#59245,
#59246),(#59247,#59248),(#59249,#59250),(#59251,#59252),(#59253,#59254),
(#59255,#59256),(#59257,#59258),(#59259,#59260),(#59261,#59262),(#59263,
#59264),(#59265,#59266),(#59267,#59268),(#59269,#59270),(#59271,#59272),
(#59273,#59274),(#59275,#59276),(#59277,#59278),(#59279,#59280),(#59281,
#59282),(#59283,#59284),(#59285,#59286),(#59287,#59288),(#59289,#59290),
(#59291,#59292),(#59293,#59294),(#59295,#59296),(#59297,#59298),(#59299,
#59300)),.UNSPECIFIED.,.F.,.F.,.F.)
B_SPLINE_SURFACE_WITH_KNOTS((6,1,1,1,1,1,1,1,1,1,1,1,1,1,1,1,1,1,1,1,1,
1,1,1,1,1,1,1,1,1,1,1,1,1,1,6),(2,2),(-1.,-0.971428571428572,-0.942857142857143,
-0.914285714285714,-0.885714285714286,-0.857142857142857,-0.828571428571429,
-0.8,-0.771428571428572,-0.742857142857143,-0.714285714285714,-0.685714285714286,
-0.657142857142857,-0.628571428571429,-0.6,-0.571428571428572,-0.542857142857143,
-0.514285714285714,-0.485714285714286,-0.457142857142857,-0.428571428571429,
-0.4,-0.371428571428571,-0.342857142857143,-0.314285714285714,-0.285714285714286,
-0.257142857142857,-0.228571428571429,-0.2,-0.171428571428571,-0.142857142857143,
-0.114285714285714,-0.0857142857142857,-0.0571428571428571,-0.0285714285714286,
0.),(0.,1.6),.UNSPECIFIED.)
GEOMETRIC_REPRESENTATION_ITEM()
RATIONAL_B_SPLINE_SURFACE(((1.,1.),(1.,1.),(1.,1.),(1.,1.),(1.,1.),(1.,
1.),(1.,1.),(1.,1.),(1.,1.),(1.,1.),(1.,1.),(1.,1.),(1.,1.),(1.,1.),(1.,
1.),(1.,1.),(1.,1.),(1.,1.),(1.,1.),(1.,1.),(1.,1.),(1.,1.),(1.,1.),(1.,
1.),(1.,1.),(1.,1.),(1.,1.),(1.,1.),(1.,1.),(1.,1.),(1.,1.),(1.,1.),(1.,
1.),(1.,1.),(1.,1.),(1.,1.),(1.,1.),(1.,1.),(1.,1.),(1.,1.)))
REPRESENTATION_ITEM('')
SURFACE()
);
#583=(
BOUNDED_SURFACE()
B_SPLINE_SURFACE(5,1,((#59324,#59325),(#59326,#59327),(#59328,#59329),(#59330,
#59331),(#59332,#59333),(#59334,#59335),(#59336,#59337),(#59338,#59339),
(#59340,#59341),(#59342,#59343),(#59344,#59345),(#59346,#59347),(#59348,
#59349),(#59350,#59351),(#59352,#59353),(#59354,#59355),(#59356,#59357),
(#59358,#59359),(#59360,#59361),(#59362,#59363),(#59364,#59365),(#59366,
#59367),(#59368,#59369),(#59370,#59371),(#59372,#59373),(#59374,#59375),
(#59376,#59377),(#59378,#59379),(#59380,#59381),(#59382,#59383),(#59384,
#59385),(#59386,#59387),(#59388,#59389),(#59390,#59391),(#59392,#59393),
(#59394,#59395),(#59396,#59397),(#59398,#59399),(#59400,#59401),(#59402,
#59403)),.UNSPECIFIED.,.F.,.F.,.F.)
B_SPLINE_SURFACE_WITH_KNOTS((6,1,1,1,1,1,1,1,1,1,1,1,1,1,1,1,1,1,1,1,1,
1,1,1,1,1,1,1,1,1,1,1,1,1,1,6),(2,2),(-1.,-0.971428571428572,-0.942857142857143,
-0.914285714285714,-0.885714285714286,-0.857142857142857,-0.828571428571429,
-0.8,-0.771428571428572,-0.742857142857143,-0.714285714285714,-0.685714285714286,
-0.657142857142857,-0.628571428571429,-0.6,-0.571428571428572,-0.542857142857143,
-0.514285714285714,-0.485714285714286,-0.457142857142857,-0.428571428571429,
-0.4,-0.371428571428571,-0.342857142857143,-0.314285714285714,-0.285714285714286,
-0.257142857142857,-0.228571428571429,-0.2,-0.171428571428571,-0.142857142857143,
-0.114285714285714,-0.0857142857142857,-0.0571428571428571,-0.0285714285714286,
0.),(0.,1.6),.UNSPECIFIED.)
GEOMETRIC_REPRESENTATION_ITEM()
RATIONAL_B_SPLINE_SURFACE(((1.,1.),(1.,1.),(1.,1.),(1.,1.),(1.,1.),(1.,
1.),(1.,1.),(1.,1.),(1.,1.),(1.,1.),(1.,1.),(1.,1.),(1.,1.),(1.,1.),(1.,
1.),(1.,1.),(1.,1.),(1.,1.),(1.,1.),(1.,1.),(1.,1.),(1.,1.),(1.,1.),(1.,
1.),(1.,1.),(1.,1.),(1.,1.),(1.,1.),(1.,1.),(1.,1.),(1.,1.),(1.,1.),(1.,
1.),(1.,1.),(1.,1.),(1.,1.),(1.,1.),(1.,1.),(1.,1.),(1.,1.)))
REPRESENTATION_ITEM('')
SURFACE()
);
#584=(
BOUNDED_SURFACE()
B_SPLINE_SURFACE(5,1,((#59435,#59436),(#59437,#59438),(#59439,#59440),(#59441,
#59442),(#59443,#59444),(#59445,#59446),(#59447,#59448),(#59449,#59450),
(#59451,#59452),(#59453,#59454),(#59455,#59456),(#59457,#59458),(#59459,
#59460),(#59461,#59462),(#59463,#59464),(#59465,#59466),(#59467,#59468),
(#59469,#59470),(#59471,#59472),(#59473,#59474),(#59475,#59476),(#59477,
#59478),(#59479,#59480),(#59481,#59482),(#59483,#59484),(#59485,#59486),
(#59487,#59488),(#59489,#59490),(#59491,#59492),(#59493,#59494),(#59495,
#59496),(#59497,#59498),(#59499,#59500),(#59501,#59502),(#59503,#59504),
(#59505,#59506),(#59507,#59508),(#59509,#59510),(#59511,#59512),(#59513,
#59514)),.UNSPECIFIED.,.F.,.F.,.F.)
B_SPLINE_SURFACE_WITH_KNOTS((6,1,1,1,1,1,1,1,1,1,1,1,1,1,1,1,1,1,1,1,1,
1,1,1,1,1,1,1,1,1,1,1,1,1,1,6),(2,2),(-1.,-0.971428571428572,-0.942857142857143,
-0.914285714285714,-0.885714285714286,-0.857142857142857,-0.828571428571429,
-0.8,-0.771428571428572,-0.742857142857143,-0.714285714285714,-0.685714285714286,
-0.657142857142857,-0.628571428571429,-0.6,-0.571428571428572,-0.542857142857143,
-0.514285714285714,-0.485714285714286,-0.457142857142857,-0.428571428571429,
-0.4,-0.371428571428571,-0.342857142857143,-0.314285714285714,-0.285714285714286,
-0.257142857142857,-0.228571428571429,-0.2,-0.171428571428571,-0.142857142857143,
-0.114285714285714,-0.0857142857142857,-0.0571428571428571,-0.0285714285714286,
0.),(0.,1.6),.UNSPECIFIED.)
GEOMETRIC_REPRESENTATION_ITEM()
RATIONAL_B_SPLINE_SURFACE(((1.,1.),(1.,1.),(1.,1.),(1.,1.),(1.,1.),(1.,
1.),(1.,1.),(1.,1.),(1.,1.),(1.,1.),(1.,1.),(1.,1.),(1.,1.),(1.,1.),(1.,
1.),(1.,1.),(1.,1.),(1.,1.),(1.,1.),(1.,1.),(1.,1.),(1.,1.),(1.,1.),(1.,
1.),(1.,1.),(1.,1.),(1.,1.),(1.,1.),(1.,1.),(1.,1.),(1.,1.),(1.,1.),(1.,
1.),(1.,1.),(1.,1.),(1.,1.),(1.,1.),(1.,1.),(1.,1.),(1.,1.)))
REPRESENTATION_ITEM('')
SURFACE()
);
#585=(
BOUNDED_SURFACE()
B_SPLINE_SURFACE(5,1,((#59534,#59535),(#59536,#59537),(#59538,#59539),(#59540,
#59541),(#59542,#59543),(#59544,#59545),(#59546,#59547),(#59548,#59549),
(#59550,#59551),(#59552,#59553),(#59554,#59555),(#59556,#59557),(#59558,
#59559),(#59560,#59561),(#59562,#59563),(#59564,#59565),(#59566,#59567),
(#59568,#59569),(#59570,#59571),(#59572,#59573),(#59574,#59575),(#59576,
#59577),(#59578,#59579),(#59580,#59581),(#59582,#59583),(#59584,#59585),
(#59586,#59587),(#59588,#59589),(#59590,#59591),(#59592,#59593),(#59594,
#59595),(#59596,#59597),(#59598,#59599),(#59600,#59601),(#59602,#59603),
(#59604,#59605),(#59606,#59607),(#59608,#59609),(#59610,#59611),(#59612,
#59613)),.UNSPECIFIED.,.F.,.F.,.F.)
B_SPLINE_SURFACE_WITH_KNOTS((6,1,1,1,1,1,1,1,1,1,1,1,1,1,1,1,1,1,1,1,1,
1,1,1,1,1,1,1,1,1,1,1,1,1,1,6),(2,2),(-1.,-0.971428571428572,-0.942857142857143,
-0.914285714285714,-0.885714285714286,-0.857142857142857,-0.828571428571429,
-0.8,-0.771428571428572,-0.742857142857143,-0.714285714285714,-0.685714285714286,
-0.657142857142857,-0.628571428571429,-0.6,-0.571428571428572,-0.542857142857143,
-0.514285714285714,-0.485714285714286,-0.457142857142857,-0.428571428571429,
-0.4,-0.371428571428571,-0.342857142857143,-0.314285714285714,-0.285714285714286,
-0.257142857142857,-0.228571428571429,-0.2,-0.171428571428571,-0.142857142857143,
-0.114285714285714,-0.0857142857142857,-0.0571428571428571,-0.0285714285714286,
0.),(0.,1.6),.UNSPECIFIED.)
GEOMETRIC_REPRESENTATION_ITEM()
RATIONAL_B_SPLINE_SURFACE(((1.,1.),(1.,1.),(1.,1.),(1.,1.),(1.,1.),(1.,
1.),(1.,1.),(1.,1.),(1.,1.),(1.,1.),(1.,1.),(1.,1.),(1.,1.),(1.,1.),(1.,
1.),(1.,1.),(1.,1.),(1.,1.),(1.,1.),(1.,1.),(1.,1.),(1.,1.),(1.,1.),(1.,
1.),(1.,1.),(1.,1.),(1.,1.),(1.,1.),(1.,1.),(1.,1.),(1.,1.),(1.,1.),(1.,
1.),(1.,1.),(1.,1.),(1.,1.),(1.,1.),(1.,1.),(1.,1.),(1.,1.)))
REPRESENTATION_ITEM('')
SURFACE()
);
#586=(
BOUNDED_SURFACE()
B_SPLINE_SURFACE(5,1,((#59633,#59634),(#59635,#59636),(#59637,#59638),(#59639,
#59640),(#59641,#59642),(#59643,#59644),(#59645,#59646),(#59647,#59648),
(#59649,#59650),(#59651,#59652),(#59653,#59654),(#59655,#59656),(#59657,
#59658),(#59659,#59660),(#59661,#59662),(#59663,#59664),(#59665,#59666),
(#59667,#59668),(#59669,#59670),(#59671,#59672),(#59673,#59674),(#59675,
#59676),(#59677,#59678),(#59679,#59680),(#59681,#59682),(#59683,#59684),
(#59685,#59686),(#59687,#59688),(#59689,#59690),(#59691,#59692),(#59693,
#59694),(#59695,#59696),(#59697,#59698),(#59699,#59700),(#59701,#59702),
(#59703,#59704),(#59705,#59706),(#59707,#59708),(#59709,#59710),(#59711,
#59712)),.UNSPECIFIED.,.F.,.F.,.F.)
B_SPLINE_SURFACE_WITH_KNOTS((6,1,1,1,1,1,1,1,1,1,1,1,1,1,1,1,1,1,1,1,1,
1,1,1,1,1,1,1,1,1,1,1,1,1,1,6),(2,2),(-1.,-0.971428571428572,-0.942857142857143,
-0.914285714285714,-0.885714285714286,-0.857142857142857,-0.828571428571429,
-0.8,-0.771428571428572,-0.742857142857143,-0.714285714285714,-0.685714285714286,
-0.657142857142857,-0.628571428571429,-0.6,-0.571428571428572,-0.542857142857143,
-0.514285714285714,-0.485714285714286,-0.457142857142857,-0.428571428571429,
-0.4,-0.371428571428571,-0.342857142857143,-0.314285714285714,-0.285714285714286,
-0.257142857142857,-0.228571428571429,-0.2,-0.171428571428571,-0.142857142857143,
-0.114285714285714,-0.0857142857142857,-0.0571428571428571,-0.0285714285714286,
0.),(0.,1.6),.UNSPECIFIED.)
GEOMETRIC_REPRESENTATION_ITEM()
RATIONAL_B_SPLINE_SURFACE(((1.,1.),(1.,1.),(1.,1.),(1.,1.),(1.,1.),(1.,
1.),(1.,1.),(1.,1.),(1.,1.),(1.,1.),(1.,1.),(1.,1.),(1.,1.),(1.,1.),(1.,
1.),(1.,1.),(1.,1.),(1.,1.),(1.,1.),(1.,1.),(1.,1.),(1.,1.),(1.,1.),(1.,
1.),(1.,1.),(1.,1.),(1.,1.),(1.,1.),(1.,1.),(1.,1.),(1.,1.),(1.,1.),(1.,
1.),(1.,1.),(1.,1.),(1.,1.),(1.,1.),(1.,1.),(1.,1.),(1.,1.)))
REPRESENTATION_ITEM('')
SURFACE()
);
#587=(
BOUNDED_SURFACE()
B_SPLINE_SURFACE(5,1,((#59732,#59733),(#59734,#59735),(#59736,#59737),(#59738,
#59739),(#59740,#59741),(#59742,#59743),(#59744,#59745),(#59746,#59747),
(#59748,#59749),(#59750,#59751),(#59752,#59753),(#59754,#59755),(#59756,
#59757),(#59758,#59759),(#59760,#59761),(#59762,#59763),(#59764,#59765),
(#59766,#59767),(#59768,#59769),(#59770,#59771),(#59772,#59773),(#59774,
#59775),(#59776,#59777),(#59778,#59779),(#59780,#59781),(#59782,#59783),
(#59784,#59785),(#59786,#59787),(#59788,#59789),(#59790,#59791),(#59792,
#59793),(#59794,#59795),(#59796,#59797),(#59798,#59799),(#59800,#59801),
(#59802,#59803),(#59804,#59805),(#59806,#59807),(#59808,#59809),(#59810,
#59811)),.UNSPECIFIED.,.F.,.F.,.F.)
B_SPLINE_SURFACE_WITH_KNOTS((6,1,1,1,1,1,1,1,1,1,1,1,1,1,1,1,1,1,1,1,1,
1,1,1,1,1,1,1,1,1,1,1,1,1,1,6),(2,2),(-1.,-0.971428571428572,-0.942857142857143,
-0.914285714285714,-0.885714285714286,-0.857142857142857,-0.828571428571429,
-0.8,-0.771428571428572,-0.742857142857143,-0.714285714285714,-0.685714285714286,
-0.657142857142857,-0.628571428571429,-0.6,-0.571428571428572,-0.542857142857143,
-0.514285714285714,-0.485714285714286,-0.457142857142857,-0.428571428571429,
-0.4,-0.371428571428571,-0.342857142857143,-0.314285714285714,-0.285714285714286,
-0.257142857142857,-0.228571428571429,-0.2,-0.171428571428571,-0.142857142857143,
-0.114285714285714,-0.0857142857142857,-0.0571428571428571,-0.0285714285714286,
0.),(0.,1.6),.UNSPECIFIED.)
GEOMETRIC_REPRESENTATION_ITEM()
RATIONAL_B_SPLINE_SURFACE(((1.,1.),(1.,1.),(1.,1.),(1.,1.),(1.,1.),(1.,
1.),(1.,1.),(1.,1.),(1.,1.),(1.,1.),(1.,1.),(1.,1.),(1.,1.),(1.,1.),(1.,
1.),(1.,1.),(1.,1.),(1.,1.),(1.,1.),(1.,1.),(1.,1.),(1.,1.),(1.,1.),(1.,
1.),(1.,1.),(1.,1.),(1.,1.),(1.,1.),(1.,1.),(1.,1.),(1.,1.),(1.,1.),(1.,
1.),(1.,1.),(1.,1.),(1.,1.),(1.,1.),(1.,1.),(1.,1.),(1.,1.)))
REPRESENTATION_ITEM('')
SURFACE()
);
#588=(
BOUNDED_SURFACE()
B_SPLINE_SURFACE(5,1,((#59831,#59832),(#59833,#59834),(#59835,#59836),(#59837,
#59838),(#59839,#59840),(#59841,#59842),(#59843,#59844),(#59845,#59846),
(#59847,#59848),(#59849,#59850),(#59851,#59852),(#59853,#59854),(#59855,
#59856),(#59857,#59858),(#59859,#59860),(#59861,#59862),(#59863,#59864),
(#59865,#59866),(#59867,#59868),(#59869,#59870),(#59871,#59872),(#59873,
#59874),(#59875,#59876),(#59877,#59878),(#59879,#59880),(#59881,#59882),
(#59883,#59884),(#59885,#59886),(#59887,#59888),(#59889,#59890),(#59891,
#59892),(#59893,#59894),(#59895,#59896),(#59897,#59898),(#59899,#59900),
(#59901,#59902),(#59903,#59904),(#59905,#59906),(#59907,#59908),(#59909,
#59910)),.UNSPECIFIED.,.F.,.F.,.F.)
B_SPLINE_SURFACE_WITH_KNOTS((6,1,1,1,1,1,1,1,1,1,1,1,1,1,1,1,1,1,1,1,1,
1,1,1,1,1,1,1,1,1,1,1,1,1,1,6),(2,2),(-1.,-0.971428571428572,-0.942857142857143,
-0.914285714285714,-0.885714285714286,-0.857142857142857,-0.828571428571429,
-0.8,-0.771428571428572,-0.742857142857143,-0.714285714285714,-0.685714285714286,
-0.657142857142857,-0.628571428571429,-0.6,-0.571428571428572,-0.542857142857143,
-0.514285714285714,-0.485714285714286,-0.457142857142857,-0.428571428571429,
-0.4,-0.371428571428571,-0.342857142857143,-0.314285714285714,-0.285714285714286,
-0.257142857142857,-0.228571428571429,-0.2,-0.171428571428571,-0.142857142857143,
-0.114285714285714,-0.0857142857142857,-0.0571428571428571,-0.0285714285714286,
0.),(0.,1.6),.UNSPECIFIED.)
GEOMETRIC_REPRESENTATION_ITEM()
RATIONAL_B_SPLINE_SURFACE(((1.,1.),(1.,1.),(1.,1.),(1.,1.),(1.,1.),(1.,
1.),(1.,1.),(1.,1.),(1.,1.),(1.,1.),(1.,1.),(1.,1.),(1.,1.),(1.,1.),(1.,
1.),(1.,1.),(1.,1.),(1.,1.),(1.,1.),(1.,1.),(1.,1.),(1.,1.),(1.,1.),(1.,
1.),(1.,1.),(1.,1.),(1.,1.),(1.,1.),(1.,1.),(1.,1.),(1.,1.),(1.,1.),(1.,
1.),(1.,1.),(1.,1.),(1.,1.),(1.,1.),(1.,1.),(1.,1.),(1.,1.)))
REPRESENTATION_ITEM('')
SURFACE()
);
#589=(
BOUNDED_SURFACE()
B_SPLINE_SURFACE(5,1,((#59930,#59931),(#59932,#59933),(#59934,#59935),(#59936,
#59937),(#59938,#59939),(#59940,#59941),(#59942,#59943),(#59944,#59945),
(#59946,#59947),(#59948,#59949),(#59950,#59951),(#59952,#59953),(#59954,
#59955),(#59956,#59957),(#59958,#59959),(#59960,#59961),(#59962,#59963),
(#59964,#59965),(#59966,#59967),(#59968,#59969),(#59970,#59971),(#59972,
#59973),(#59974,#59975),(#59976,#59977),(#59978,#59979),(#59980,#59981),
(#59982,#59983),(#59984,#59985),(#59986,#59987),(#59988,#59989),(#59990,
#59991),(#59992,#59993),(#59994,#59995),(#59996,#59997),(#59998,#59999),
(#60000,#60001),(#60002,#60003),(#60004,#60005),(#60006,#60007),(#60008,
#60009)),.UNSPECIFIED.,.F.,.F.,.F.)
B_SPLINE_SURFACE_WITH_KNOTS((6,1,1,1,1,1,1,1,1,1,1,1,1,1,1,1,1,1,1,1,1,
1,1,1,1,1,1,1,1,1,1,1,1,1,1,6),(2,2),(-1.,-0.971428571428572,-0.942857142857143,
-0.914285714285714,-0.885714285714286,-0.857142857142857,-0.828571428571429,
-0.8,-0.771428571428572,-0.742857142857143,-0.714285714285714,-0.685714285714286,
-0.657142857142857,-0.628571428571429,-0.6,-0.571428571428572,-0.542857142857143,
-0.514285714285714,-0.485714285714286,-0.457142857142857,-0.428571428571429,
-0.4,-0.371428571428571,-0.342857142857143,-0.314285714285714,-0.285714285714286,
-0.257142857142857,-0.228571428571429,-0.2,-0.171428571428571,-0.142857142857143,
-0.114285714285714,-0.0857142857142857,-0.0571428571428571,-0.0285714285714286,
0.),(0.,1.6),.UNSPECIFIED.)
GEOMETRIC_REPRESENTATION_ITEM()
RATIONAL_B_SPLINE_SURFACE(((1.,1.),(1.,1.),(1.,1.),(1.,1.),(1.,1.),(1.,
1.),(1.,1.),(1.,1.),(1.,1.),(1.,1.),(1.,1.),(1.,1.),(1.,1.),(1.,1.),(1.,
1.),(1.,1.),(1.,1.),(1.,1.),(1.,1.),(1.,1.),(1.,1.),(1.,1.),(1.,1.),(1.,
1.),(1.,1.),(1.,1.),(1.,1.),(1.,1.),(1.,1.),(1.,1.),(1.,1.),(1.,1.),(1.,
1.),(1.,1.),(1.,1.),(1.,1.),(1.,1.),(1.,1.),(1.,1.),(1.,1.)))
REPRESENTATION_ITEM('')
SURFACE()
);
#590=(
BOUNDED_SURFACE()
B_SPLINE_SURFACE(5,1,((#60029,#60030),(#60031,#60032),(#60033,#60034),(#60035,
#60036),(#60037,#60038),(#60039,#60040),(#60041,#60042),(#60043,#60044),
(#60045,#60046),(#60047,#60048),(#60049,#60050),(#60051,#60052),(#60053,
#60054),(#60055,#60056),(#60057,#60058),(#60059,#60060),(#60061,#60062),
(#60063,#60064),(#60065,#60066),(#60067,#60068),(#60069,#60070),(#60071,
#60072),(#60073,#60074),(#60075,#60076),(#60077,#60078),(#60079,#60080),
(#60081,#60082),(#60083,#60084),(#60085,#60086),(#60087,#60088),(#60089,
#60090),(#60091,#60092),(#60093,#60094),(#60095,#60096),(#60097,#60098),
(#60099,#60100),(#60101,#60102),(#60103,#60104),(#60105,#60106),(#60107,
#60108)),.UNSPECIFIED.,.F.,.F.,.F.)
B_SPLINE_SURFACE_WITH_KNOTS((6,1,1,1,1,1,1,1,1,1,1,1,1,1,1,1,1,1,1,1,1,
1,1,1,1,1,1,1,1,1,1,1,1,1,1,6),(2,2),(-1.,-0.971428571428572,-0.942857142857143,
-0.914285714285714,-0.885714285714286,-0.857142857142857,-0.828571428571429,
-0.8,-0.771428571428572,-0.742857142857143,-0.714285714285714,-0.685714285714286,
-0.657142857142857,-0.628571428571429,-0.6,-0.571428571428572,-0.542857142857143,
-0.514285714285714,-0.485714285714286,-0.457142857142857,-0.428571428571429,
-0.4,-0.371428571428571,-0.342857142857143,-0.314285714285714,-0.285714285714286,
-0.257142857142857,-0.228571428571429,-0.2,-0.171428571428571,-0.142857142857143,
-0.114285714285714,-0.0857142857142857,-0.0571428571428571,-0.0285714285714286,
0.),(0.,1.6),.UNSPECIFIED.)
GEOMETRIC_REPRESENTATION_ITEM()
RATIONAL_B_SPLINE_SURFACE(((1.,1.),(1.,1.),(1.,1.),(1.,1.),(1.,1.),(1.,
1.),(1.,1.),(1.,1.),(1.,1.),(1.,1.),(1.,1.),(1.,1.),(1.,1.),(1.,1.),(1.,
1.),(1.,1.),(1.,1.),(1.,1.),(1.,1.),(1.,1.),(1.,1.),(1.,1.),(1.,1.),(1.,
1.),(1.,1.),(1.,1.),(1.,1.),(1.,1.),(1.,1.),(1.,1.),(1.,1.),(1.,1.),(1.,
1.),(1.,1.),(1.,1.),(1.,1.),(1.,1.),(1.,1.),(1.,1.),(1.,1.)))
REPRESENTATION_ITEM('')
SURFACE()
);
#591=(
BOUNDED_SURFACE()
B_SPLINE_SURFACE(5,1,((#60128,#60129),(#60130,#60131),(#60132,#60133),(#60134,
#60135),(#60136,#60137),(#60138,#60139),(#60140,#60141),(#60142,#60143),
(#60144,#60145),(#60146,#60147),(#60148,#60149),(#60150,#60151),(#60152,
#60153),(#60154,#60155),(#60156,#60157),(#60158,#60159),(#60160,#60161),
(#60162,#60163),(#60164,#60165),(#60166,#60167),(#60168,#60169),(#60170,
#60171),(#60172,#60173),(#60174,#60175),(#60176,#60177),(#60178,#60179),
(#60180,#60181),(#60182,#60183),(#60184,#60185),(#60186,#60187),(#60188,
#60189),(#60190,#60191),(#60192,#60193),(#60194,#60195),(#60196,#60197),
(#60198,#60199),(#60200,#60201),(#60202,#60203),(#60204,#60205),(#60206,
#60207)),.UNSPECIFIED.,.F.,.F.,.F.)
B_SPLINE_SURFACE_WITH_KNOTS((6,1,1,1,1,1,1,1,1,1,1,1,1,1,1,1,1,1,1,1,1,
1,1,1,1,1,1,1,1,1,1,1,1,1,1,6),(2,2),(-1.,-0.971428571428572,-0.942857142857143,
-0.914285714285714,-0.885714285714286,-0.857142857142857,-0.828571428571429,
-0.8,-0.771428571428572,-0.742857142857143,-0.714285714285714,-0.685714285714286,
-0.657142857142857,-0.628571428571429,-0.6,-0.571428571428572,-0.542857142857143,
-0.514285714285714,-0.485714285714286,-0.457142857142857,-0.428571428571429,
-0.4,-0.371428571428571,-0.342857142857143,-0.314285714285714,-0.285714285714286,
-0.257142857142857,-0.228571428571429,-0.2,-0.171428571428571,-0.142857142857143,
-0.114285714285714,-0.0857142857142857,-0.0571428571428571,-0.0285714285714286,
0.),(0.,1.6),.UNSPECIFIED.)
GEOMETRIC_REPRESENTATION_ITEM()
RATIONAL_B_SPLINE_SURFACE(((1.,1.),(1.,1.),(1.,1.),(1.,1.),(1.,1.),(1.,
1.),(1.,1.),(1.,1.),(1.,1.),(1.,1.),(1.,1.),(1.,1.),(1.,1.),(1.,1.),(1.,
1.),(1.,1.),(1.,1.),(1.,1.),(1.,1.),(1.,1.),(1.,1.),(1.,1.),(1.,1.),(1.,
1.),(1.,1.),(1.,1.),(1.,1.),(1.,1.),(1.,1.),(1.,1.),(1.,1.),(1.,1.),(1.,
1.),(1.,1.),(1.,1.),(1.,1.),(1.,1.),(1.,1.),(1.,1.),(1.,1.)))
REPRESENTATION_ITEM('')
SURFACE()
);
#592=(
BOUNDED_SURFACE()
B_SPLINE_SURFACE(5,1,((#60227,#60228),(#60229,#60230),(#60231,#60232),(#60233,
#60234),(#60235,#60236),(#60237,#60238),(#60239,#60240),(#60241,#60242),
(#60243,#60244),(#60245,#60246),(#60247,#60248),(#60249,#60250),(#60251,
#60252),(#60253,#60254),(#60255,#60256),(#60257,#60258),(#60259,#60260),
(#60261,#60262),(#60263,#60264),(#60265,#60266),(#60267,#60268),(#60269,
#60270),(#60271,#60272),(#60273,#60274),(#60275,#60276),(#60277,#60278),
(#60279,#60280),(#60281,#60282),(#60283,#60284),(#60285,#60286),(#60287,
#60288),(#60289,#60290),(#60291,#60292),(#60293,#60294),(#60295,#60296),
(#60297,#60298),(#60299,#60300),(#60301,#60302),(#60303,#60304),(#60305,
#60306)),.UNSPECIFIED.,.F.,.F.,.F.)
B_SPLINE_SURFACE_WITH_KNOTS((6,1,1,1,1,1,1,1,1,1,1,1,1,1,1,1,1,1,1,1,1,
1,1,1,1,1,1,1,1,1,1,1,1,1,1,6),(2,2),(-1.,-0.971428571428572,-0.942857142857143,
-0.914285714285714,-0.885714285714286,-0.857142857142857,-0.828571428571429,
-0.8,-0.771428571428572,-0.742857142857143,-0.714285714285714,-0.685714285714286,
-0.657142857142857,-0.628571428571429,-0.6,-0.571428571428572,-0.542857142857143,
-0.514285714285714,-0.485714285714286,-0.457142857142857,-0.428571428571429,
-0.4,-0.371428571428571,-0.342857142857143,-0.314285714285714,-0.285714285714286,
-0.257142857142857,-0.228571428571429,-0.2,-0.171428571428571,-0.142857142857143,
-0.114285714285714,-0.0857142857142857,-0.0571428571428571,-0.0285714285714286,
0.),(0.,1.6),.UNSPECIFIED.)
GEOMETRIC_REPRESENTATION_ITEM()
RATIONAL_B_SPLINE_SURFACE(((1.,1.),(1.,1.),(1.,1.),(1.,1.),(1.,1.),(1.,
1.),(1.,1.),(1.,1.),(1.,1.),(1.,1.),(1.,1.),(1.,1.),(1.,1.),(1.,1.),(1.,
1.),(1.,1.),(1.,1.),(1.,1.),(1.,1.),(1.,1.),(1.,1.),(1.,1.),(1.,1.),(1.,
1.),(1.,1.),(1.,1.),(1.,1.),(1.,1.),(1.,1.),(1.,1.),(1.,1.),(1.,1.),(1.,
1.),(1.,1.),(1.,1.),(1.,1.),(1.,1.),(1.,1.),(1.,1.),(1.,1.)))
REPRESENTATION_ITEM('')
SURFACE()
);
#593=(
BOUNDED_SURFACE()
B_SPLINE_SURFACE(5,1,((#60326,#60327),(#60328,#60329),(#60330,#60331),(#60332,
#60333),(#60334,#60335),(#60336,#60337),(#60338,#60339),(#60340,#60341),
(#60342,#60343),(#60344,#60345),(#60346,#60347),(#60348,#60349),(#60350,
#60351),(#60352,#60353),(#60354,#60355),(#60356,#60357),(#60358,#60359),
(#60360,#60361),(#60362,#60363),(#60364,#60365),(#60366,#60367),(#60368,
#60369),(#60370,#60371),(#60372,#60373),(#60374,#60375),(#60376,#60377),
(#60378,#60379),(#60380,#60381),(#60382,#60383),(#60384,#60385),(#60386,
#60387),(#60388,#60389),(#60390,#60391),(#60392,#60393),(#60394,#60395),
(#60396,#60397),(#60398,#60399),(#60400,#60401),(#60402,#60403),(#60404,
#60405)),.UNSPECIFIED.,.F.,.F.,.F.)
B_SPLINE_SURFACE_WITH_KNOTS((6,1,1,1,1,1,1,1,1,1,1,1,1,1,1,1,1,1,1,1,1,
1,1,1,1,1,1,1,1,1,1,1,1,1,1,6),(2,2),(-1.,-0.971428571428572,-0.942857142857143,
-0.914285714285714,-0.885714285714286,-0.857142857142857,-0.828571428571429,
-0.8,-0.771428571428572,-0.742857142857143,-0.714285714285714,-0.685714285714286,
-0.657142857142857,-0.628571428571429,-0.6,-0.571428571428572,-0.542857142857143,
-0.514285714285714,-0.485714285714286,-0.457142857142857,-0.428571428571429,
-0.4,-0.371428571428571,-0.342857142857143,-0.314285714285714,-0.285714285714286,
-0.257142857142857,-0.228571428571429,-0.2,-0.171428571428571,-0.142857142857143,
-0.114285714285714,-0.0857142857142857,-0.0571428571428571,-0.0285714285714286,
0.),(0.,1.6),.UNSPECIFIED.)
GEOMETRIC_REPRESENTATION_ITEM()
RATIONAL_B_SPLINE_SURFACE(((1.,1.),(1.,1.),(1.,1.),(1.,1.),(1.,1.),(1.,
1.),(1.,1.),(1.,1.),(1.,1.),(1.,1.),(1.,1.),(1.,1.),(1.,1.),(1.,1.),(1.,
1.),(1.,1.),(1.,1.),(1.,1.),(1.,1.),(1.,1.),(1.,1.),(1.,1.),(1.,1.),(1.,
1.),(1.,1.),(1.,1.),(1.,1.),(1.,1.),(1.,1.),(1.,1.),(1.,1.),(1.,1.),(1.,
1.),(1.,1.),(1.,1.),(1.,1.),(1.,1.),(1.,1.),(1.,1.),(1.,1.)))
REPRESENTATION_ITEM('')
SURFACE()
);
#594=(
BOUNDED_SURFACE()
B_SPLINE_SURFACE(5,1,((#60437,#60438),(#60439,#60440),(#60441,#60442),(#60443,
#60444),(#60445,#60446),(#60447,#60448),(#60449,#60450),(#60451,#60452),
(#60453,#60454),(#60455,#60456),(#60457,#60458),(#60459,#60460),(#60461,
#60462),(#60463,#60464),(#60465,#60466),(#60467,#60468),(#60469,#60470),
(#60471,#60472),(#60473,#60474),(#60475,#60476),(#60477,#60478),(#60479,
#60480),(#60481,#60482),(#60483,#60484),(#60485,#60486),(#60487,#60488),
(#60489,#60490),(#60491,#60492),(#60493,#60494),(#60495,#60496),(#60497,
#60498),(#60499,#60500),(#60501,#60502),(#60503,#60504),(#60505,#60506),
(#60507,#60508),(#60509,#60510),(#60511,#60512),(#60513,#60514),(#60515,
#60516)),.UNSPECIFIED.,.F.,.F.,.F.)
B_SPLINE_SURFACE_WITH_KNOTS((6,1,1,1,1,1,1,1,1,1,1,1,1,1,1,1,1,1,1,1,1,
1,1,1,1,1,1,1,1,1,1,1,1,1,1,6),(2,2),(-1.,-0.971428571428572,-0.942857142857143,
-0.914285714285714,-0.885714285714286,-0.857142857142857,-0.828571428571429,
-0.8,-0.771428571428572,-0.742857142857143,-0.714285714285714,-0.685714285714286,
-0.657142857142857,-0.628571428571429,-0.6,-0.571428571428572,-0.542857142857143,
-0.514285714285714,-0.485714285714286,-0.457142857142857,-0.428571428571429,
-0.4,-0.371428571428571,-0.342857142857143,-0.314285714285714,-0.285714285714286,
-0.257142857142857,-0.228571428571429,-0.2,-0.171428571428571,-0.142857142857143,
-0.114285714285714,-0.0857142857142857,-0.0571428571428571,-0.0285714285714286,
0.),(0.,1.6),.UNSPECIFIED.)
GEOMETRIC_REPRESENTATION_ITEM()
RATIONAL_B_SPLINE_SURFACE(((1.,1.),(1.,1.),(1.,1.),(1.,1.),(1.,1.),(1.,
1.),(1.,1.),(1.,1.),(1.,1.),(1.,1.),(1.,1.),(1.,1.),(1.,1.),(1.,1.),(1.,
1.),(1.,1.),(1.,1.),(1.,1.),(1.,1.),(1.,1.),(1.,1.),(1.,1.),(1.,1.),(1.,
1.),(1.,1.),(1.,1.),(1.,1.),(1.,1.),(1.,1.),(1.,1.),(1.,1.),(1.,1.),(1.,
1.),(1.,1.),(1.,1.),(1.,1.),(1.,1.),(1.,1.),(1.,1.),(1.,1.)))
REPRESENTATION_ITEM('')
SURFACE()
);
#595=(
BOUNDED_SURFACE()
B_SPLINE_SURFACE(5,1,((#60538,#60539),(#60540,#60541),(#60542,#60543),(#60544,
#60545),(#60546,#60547),(#60548,#60549),(#60550,#60551),(#60552,#60553),
(#60554,#60555),(#60556,#60557),(#60558,#60559),(#60560,#60561),(#60562,
#60563),(#60564,#60565),(#60566,#60567),(#60568,#60569),(#60570,#60571),
(#60572,#60573),(#60574,#60575),(#60576,#60577),(#60578,#60579),(#60580,
#60581),(#60582,#60583),(#60584,#60585),(#60586,#60587),(#60588,#60589),
(#60590,#60591),(#60592,#60593),(#60594,#60595),(#60596,#60597),(#60598,
#60599),(#60600,#60601),(#60602,#60603),(#60604,#60605),(#60606,#60607),
(#60608,#60609),(#60610,#60611),(#60612,#60613),(#60614,#60615),(#60616,
#60617)),.UNSPECIFIED.,.F.,.F.,.F.)
B_SPLINE_SURFACE_WITH_KNOTS((6,1,1,1,1,1,1,1,1,1,1,1,1,1,1,1,1,1,1,1,1,
1,1,1,1,1,1,1,1,1,1,1,1,1,1,6),(2,2),(-1.,-0.971428571428572,-0.942857142857143,
-0.914285714285714,-0.885714285714286,-0.857142857142857,-0.828571428571429,
-0.8,-0.771428571428572,-0.742857142857143,-0.714285714285714,-0.685714285714286,
-0.657142857142857,-0.628571428571429,-0.6,-0.571428571428572,-0.542857142857143,
-0.514285714285714,-0.485714285714286,-0.457142857142857,-0.428571428571429,
-0.4,-0.371428571428571,-0.342857142857143,-0.314285714285714,-0.285714285714286,
-0.257142857142857,-0.228571428571429,-0.2,-0.171428571428571,-0.142857142857143,
-0.114285714285714,-0.0857142857142857,-0.0571428571428571,-0.0285714285714286,
0.),(0.,1.6),.UNSPECIFIED.)
GEOMETRIC_REPRESENTATION_ITEM()
RATIONAL_B_SPLINE_SURFACE(((1.,1.),(1.,1.),(1.,1.),(1.,1.),(1.,1.),(1.,
1.),(1.,1.),(1.,1.),(1.,1.),(1.,1.),(1.,1.),(1.,1.),(1.,1.),(1.,1.),(1.,
1.),(1.,1.),(1.,1.),(1.,1.),(1.,1.),(1.,1.),(1.,1.),(1.,1.),(1.,1.),(1.,
1.),(1.,1.),(1.,1.),(1.,1.),(1.,1.),(1.,1.),(1.,1.),(1.,1.),(1.,1.),(1.,
1.),(1.,1.),(1.,1.),(1.,1.),(1.,1.),(1.,1.),(1.,1.),(1.,1.)))
REPRESENTATION_ITEM('')
SURFACE()
);
#596=(
BOUNDED_SURFACE()
B_SPLINE_SURFACE(5,1,((#60649,#60650),(#60651,#60652),(#60653,#60654),(#60655,
#60656),(#60657,#60658),(#60659,#60660),(#60661,#60662),(#60663,#60664),
(#60665,#60666),(#60667,#60668),(#60669,#60670),(#60671,#60672),(#60673,
#60674),(#60675,#60676),(#60677,#60678),(#60679,#60680),(#60681,#60682),
(#60683,#60684),(#60685,#60686),(#60687,#60688),(#60689,#60690),(#60691,
#60692),(#60693,#60694),(#60695,#60696),(#60697,#60698),(#60699,#60700),
(#60701,#60702),(#60703,#60704),(#60705,#60706),(#60707,#60708),(#60709,
#60710),(#60711,#60712),(#60713,#60714),(#60715,#60716),(#60717,#60718),
(#60719,#60720),(#60721,#60722),(#60723,#60724),(#60725,#60726),(#60727,
#60728)),.UNSPECIFIED.,.F.,.F.,.F.)
B_SPLINE_SURFACE_WITH_KNOTS((6,1,1,1,1,1,1,1,1,1,1,1,1,1,1,1,1,1,1,1,1,
1,1,1,1,1,1,1,1,1,1,1,1,1,1,6),(2,2),(-1.,-0.971428571428572,-0.942857142857143,
-0.914285714285714,-0.885714285714286,-0.857142857142857,-0.828571428571429,
-0.8,-0.771428571428572,-0.742857142857143,-0.714285714285714,-0.685714285714286,
-0.657142857142857,-0.628571428571429,-0.6,-0.571428571428572,-0.542857142857143,
-0.514285714285714,-0.485714285714286,-0.457142857142857,-0.428571428571429,
-0.4,-0.371428571428571,-0.342857142857143,-0.314285714285714,-0.285714285714286,
-0.257142857142857,-0.228571428571429,-0.2,-0.171428571428571,-0.142857142857143,
-0.114285714285714,-0.0857142857142857,-0.0571428571428571,-0.0285714285714286,
0.),(0.,1.6),.UNSPECIFIED.)
GEOMETRIC_REPRESENTATION_ITEM()
RATIONAL_B_SPLINE_SURFACE(((1.,1.),(1.,1.),(1.,1.),(1.,1.),(1.,1.),(1.,
1.),(1.,1.),(1.,1.),(1.,1.),(1.,1.),(1.,1.),(1.,1.),(1.,1.),(1.,1.),(1.,
1.),(1.,1.),(1.,1.),(1.,1.),(1.,1.),(1.,1.),(1.,1.),(1.,1.),(1.,1.),(1.,
1.),(1.,1.),(1.,1.),(1.,1.),(1.,1.),(1.,1.),(1.,1.),(1.,1.),(1.,1.),(1.,
1.),(1.,1.),(1.,1.),(1.,1.),(1.,1.),(1.,1.),(1.,1.),(1.,1.)))
REPRESENTATION_ITEM('')
SURFACE()
);
#597=(
BOUNDED_SURFACE()
B_SPLINE_SURFACE(5,1,((#60748,#60749),(#60750,#60751),(#60752,#60753),(#60754,
#60755),(#60756,#60757),(#60758,#60759),(#60760,#60761),(#60762,#60763),
(#60764,#60765),(#60766,#60767),(#60768,#60769),(#60770,#60771),(#60772,
#60773),(#60774,#60775),(#60776,#60777),(#60778,#60779),(#60780,#60781),
(#60782,#60783),(#60784,#60785),(#60786,#60787),(#60788,#60789),(#60790,
#60791),(#60792,#60793),(#60794,#60795),(#60796,#60797),(#60798,#60799),
(#60800,#60801),(#60802,#60803),(#60804,#60805),(#60806,#60807),(#60808,
#60809),(#60810,#60811),(#60812,#60813),(#60814,#60815),(#60816,#60817),
(#60818,#60819),(#60820,#60821),(#60822,#60823),(#60824,#60825),(#60826,
#60827)),.UNSPECIFIED.,.F.,.F.,.F.)
B_SPLINE_SURFACE_WITH_KNOTS((6,1,1,1,1,1,1,1,1,1,1,1,1,1,1,1,1,1,1,1,1,
1,1,1,1,1,1,1,1,1,1,1,1,1,1,6),(2,2),(-1.,-0.971428571428572,-0.942857142857143,
-0.914285714285714,-0.885714285714286,-0.857142857142857,-0.828571428571429,
-0.8,-0.771428571428572,-0.742857142857143,-0.714285714285714,-0.685714285714286,
-0.657142857142857,-0.628571428571429,-0.6,-0.571428571428572,-0.542857142857143,
-0.514285714285714,-0.485714285714286,-0.457142857142857,-0.428571428571429,
-0.4,-0.371428571428571,-0.342857142857143,-0.314285714285714,-0.285714285714286,
-0.257142857142857,-0.228571428571429,-0.2,-0.171428571428571,-0.142857142857143,
-0.114285714285714,-0.0857142857142857,-0.0571428571428571,-0.0285714285714286,
0.),(0.,1.6),.UNSPECIFIED.)
GEOMETRIC_REPRESENTATION_ITEM()
RATIONAL_B_SPLINE_SURFACE(((1.,1.),(1.,1.),(1.,1.),(1.,1.),(1.,1.),(1.,
1.),(1.,1.),(1.,1.),(1.,1.),(1.,1.),(1.,1.),(1.,1.),(1.,1.),(1.,1.),(1.,
1.),(1.,1.),(1.,1.),(1.,1.),(1.,1.),(1.,1.),(1.,1.),(1.,1.),(1.,1.),(1.,
1.),(1.,1.),(1.,1.),(1.,1.),(1.,1.),(1.,1.),(1.,1.),(1.,1.),(1.,1.),(1.,
1.),(1.,1.),(1.,1.),(1.,1.),(1.,1.),(1.,1.),(1.,1.),(1.,1.)))
REPRESENTATION_ITEM('')
SURFACE()
);
#598=(
BOUNDED_SURFACE()
B_SPLINE_SURFACE(5,1,((#60847,#60848),(#60849,#60850),(#60851,#60852),(#60853,
#60854),(#60855,#60856),(#60857,#60858),(#60859,#60860),(#60861,#60862),
(#60863,#60864),(#60865,#60866),(#60867,#60868),(#60869,#60870),(#60871,
#60872),(#60873,#60874),(#60875,#60876),(#60877,#60878),(#60879,#60880),
(#60881,#60882),(#60883,#60884),(#60885,#60886),(#60887,#60888),(#60889,
#60890),(#60891,#60892),(#60893,#60894),(#60895,#60896),(#60897,#60898),
(#60899,#60900),(#60901,#60902),(#60903,#60904),(#60905,#60906),(#60907,
#60908),(#60909,#60910),(#60911,#60912),(#60913,#60914),(#60915,#60916),
(#60917,#60918),(#60919,#60920),(#60921,#60922),(#60923,#60924),(#60925,
#60926)),.UNSPECIFIED.,.F.,.F.,.F.)
B_SPLINE_SURFACE_WITH_KNOTS((6,1,1,1,1,1,1,1,1,1,1,1,1,1,1,1,1,1,1,1,1,
1,1,1,1,1,1,1,1,1,1,1,1,1,1,6),(2,2),(-1.,-0.971428571428572,-0.942857142857143,
-0.914285714285714,-0.885714285714286,-0.857142857142857,-0.828571428571429,
-0.8,-0.771428571428572,-0.742857142857143,-0.714285714285714,-0.685714285714286,
-0.657142857142857,-0.628571428571429,-0.6,-0.571428571428572,-0.542857142857143,
-0.514285714285714,-0.485714285714286,-0.457142857142857,-0.428571428571429,
-0.4,-0.371428571428571,-0.342857142857143,-0.314285714285714,-0.285714285714286,
-0.257142857142857,-0.228571428571429,-0.2,-0.171428571428571,-0.142857142857143,
-0.114285714285714,-0.0857142857142857,-0.0571428571428571,-0.0285714285714286,
0.),(0.,1.6),.UNSPECIFIED.)
GEOMETRIC_REPRESENTATION_ITEM()
RATIONAL_B_SPLINE_SURFACE(((1.,1.),(1.,1.),(1.,1.),(1.,1.),(1.,1.),(1.,
1.),(1.,1.),(1.,1.),(1.,1.),(1.,1.),(1.,1.),(1.,1.),(1.,1.),(1.,1.),(1.,
1.),(1.,1.),(1.,1.),(1.,1.),(1.,1.),(1.,1.),(1.,1.),(1.,1.),(1.,1.),(1.,
1.),(1.,1.),(1.,1.),(1.,1.),(1.,1.),(1.,1.),(1.,1.),(1.,1.),(1.,1.),(1.,
1.),(1.,1.),(1.,1.),(1.,1.),(1.,1.),(1.,1.),(1.,1.),(1.,1.)))
REPRESENTATION_ITEM('')
SURFACE()
);
#599=(
BOUNDED_SURFACE()
B_SPLINE_SURFACE(5,1,((#60946,#60947),(#60948,#60949),(#60950,#60951),(#60952,
#60953),(#60954,#60955),(#60956,#60957),(#60958,#60959),(#60960,#60961),
(#60962,#60963),(#60964,#60965),(#60966,#60967),(#60968,#60969),(#60970,
#60971),(#60972,#60973),(#60974,#60975),(#60976,#60977),(#60978,#60979),
(#60980,#60981),(#60982,#60983),(#60984,#60985),(#60986,#60987),(#60988,
#60989),(#60990,#60991),(#60992,#60993),(#60994,#60995),(#60996,#60997),
(#60998,#60999),(#61000,#61001),(#61002,#61003),(#61004,#61005),(#61006,
#61007),(#61008,#61009),(#61010,#61011),(#61012,#61013),(#61014,#61015),
(#61016,#61017),(#61018,#61019),(#61020,#61021),(#61022,#61023),(#61024,
#61025)),.UNSPECIFIED.,.F.,.F.,.F.)
B_SPLINE_SURFACE_WITH_KNOTS((6,1,1,1,1,1,1,1,1,1,1,1,1,1,1,1,1,1,1,1,1,
1,1,1,1,1,1,1,1,1,1,1,1,1,1,6),(2,2),(-1.,-0.971428571428572,-0.942857142857143,
-0.914285714285714,-0.885714285714286,-0.857142857142857,-0.828571428571429,
-0.8,-0.771428571428572,-0.742857142857143,-0.714285714285714,-0.685714285714286,
-0.657142857142857,-0.628571428571429,-0.6,-0.571428571428572,-0.542857142857143,
-0.514285714285714,-0.485714285714286,-0.457142857142857,-0.428571428571429,
-0.4,-0.371428571428571,-0.342857142857143,-0.314285714285714,-0.285714285714286,
-0.257142857142857,-0.228571428571429,-0.2,-0.171428571428571,-0.142857142857143,
-0.114285714285714,-0.0857142857142857,-0.0571428571428571,-0.0285714285714286,
0.),(0.,1.6),.UNSPECIFIED.)
GEOMETRIC_REPRESENTATION_ITEM()
RATIONAL_B_SPLINE_SURFACE(((1.,1.),(1.,1.),(1.,1.),(1.,1.),(1.,1.),(1.,
1.),(1.,1.),(1.,1.),(1.,1.),(1.,1.),(1.,1.),(1.,1.),(1.,1.),(1.,1.),(1.,
1.),(1.,1.),(1.,1.),(1.,1.),(1.,1.),(1.,1.),(1.,1.),(1.,1.),(1.,1.),(1.,
1.),(1.,1.),(1.,1.),(1.,1.),(1.,1.),(1.,1.),(1.,1.),(1.,1.),(1.,1.),(1.,
1.),(1.,1.),(1.,1.),(1.,1.),(1.,1.),(1.,1.),(1.,1.),(1.,1.)))
REPRESENTATION_ITEM('')
SURFACE()
);
#600=(
BOUNDED_SURFACE()
B_SPLINE_SURFACE(5,1,((#61045,#61046),(#61047,#61048),(#61049,#61050),(#61051,
#61052),(#61053,#61054),(#61055,#61056),(#61057,#61058),(#61059,#61060),
(#61061,#61062),(#61063,#61064),(#61065,#61066),(#61067,#61068),(#61069,
#61070),(#61071,#61072),(#61073,#61074),(#61075,#61076),(#61077,#61078),
(#61079,#61080),(#61081,#61082),(#61083,#61084),(#61085,#61086),(#61087,
#61088),(#61089,#61090),(#61091,#61092),(#61093,#61094),(#61095,#61096),
(#61097,#61098),(#61099,#61100),(#61101,#61102),(#61103,#61104),(#61105,
#61106),(#61107,#61108),(#61109,#61110),(#61111,#61112),(#61113,#61114),
(#61115,#61116),(#61117,#61118),(#61119,#61120),(#61121,#61122),(#61123,
#61124)),.UNSPECIFIED.,.F.,.F.,.F.)
B_SPLINE_SURFACE_WITH_KNOTS((6,1,1,1,1,1,1,1,1,1,1,1,1,1,1,1,1,1,1,1,1,
1,1,1,1,1,1,1,1,1,1,1,1,1,1,6),(2,2),(-1.,-0.971428571428572,-0.942857142857143,
-0.914285714285714,-0.885714285714286,-0.857142857142857,-0.828571428571429,
-0.8,-0.771428571428572,-0.742857142857143,-0.714285714285714,-0.685714285714286,
-0.657142857142857,-0.628571428571429,-0.6,-0.571428571428572,-0.542857142857143,
-0.514285714285714,-0.485714285714286,-0.457142857142857,-0.428571428571429,
-0.4,-0.371428571428571,-0.342857142857143,-0.314285714285714,-0.285714285714286,
-0.257142857142857,-0.228571428571429,-0.2,-0.171428571428571,-0.142857142857143,
-0.114285714285714,-0.0857142857142857,-0.0571428571428571,-0.0285714285714286,
0.),(0.,1.6),.UNSPECIFIED.)
GEOMETRIC_REPRESENTATION_ITEM()
RATIONAL_B_SPLINE_SURFACE(((1.,1.),(1.,1.),(1.,1.),(1.,1.),(1.,1.),(1.,
1.),(1.,1.),(1.,1.),(1.,1.),(1.,1.),(1.,1.),(1.,1.),(1.,1.),(1.,1.),(1.,
1.),(1.,1.),(1.,1.),(1.,1.),(1.,1.),(1.,1.),(1.,1.),(1.,1.),(1.,1.),(1.,
1.),(1.,1.),(1.,1.),(1.,1.),(1.,1.),(1.,1.),(1.,1.),(1.,1.),(1.,1.),(1.,
1.),(1.,1.),(1.,1.),(1.,1.),(1.,1.),(1.,1.),(1.,1.),(1.,1.)))
REPRESENTATION_ITEM('')
SURFACE()
);
#601=(
BOUNDED_SURFACE()
B_SPLINE_SURFACE(5,1,((#61144,#61145),(#61146,#61147),(#61148,#61149),(#61150,
#61151),(#61152,#61153),(#61154,#61155),(#61156,#61157),(#61158,#61159),
(#61160,#61161),(#61162,#61163),(#61164,#61165),(#61166,#61167),(#61168,
#61169),(#61170,#61171),(#61172,#61173),(#61174,#61175),(#61176,#61177),
(#61178,#61179),(#61180,#61181),(#61182,#61183),(#61184,#61185),(#61186,
#61187),(#61188,#61189),(#61190,#61191),(#61192,#61193),(#61194,#61195),
(#61196,#61197),(#61198,#61199),(#61200,#61201),(#61202,#61203),(#61204,
#61205),(#61206,#61207),(#61208,#61209),(#61210,#61211),(#61212,#61213),
(#61214,#61215),(#61216,#61217),(#61218,#61219),(#61220,#61221),(#61222,
#61223)),.UNSPECIFIED.,.F.,.F.,.F.)
B_SPLINE_SURFACE_WITH_KNOTS((6,1,1,1,1,1,1,1,1,1,1,1,1,1,1,1,1,1,1,1,1,
1,1,1,1,1,1,1,1,1,1,1,1,1,1,6),(2,2),(-1.,-0.971428571428572,-0.942857142857143,
-0.914285714285714,-0.885714285714286,-0.857142857142857,-0.828571428571429,
-0.8,-0.771428571428572,-0.742857142857143,-0.714285714285714,-0.685714285714286,
-0.657142857142857,-0.628571428571429,-0.6,-0.571428571428572,-0.542857142857143,
-0.514285714285714,-0.485714285714286,-0.457142857142857,-0.428571428571429,
-0.4,-0.371428571428571,-0.342857142857143,-0.314285714285714,-0.285714285714286,
-0.257142857142857,-0.228571428571429,-0.2,-0.171428571428571,-0.142857142857143,
-0.114285714285714,-0.0857142857142857,-0.0571428571428571,-0.0285714285714286,
0.),(0.,1.6),.UNSPECIFIED.)
GEOMETRIC_REPRESENTATION_ITEM()
RATIONAL_B_SPLINE_SURFACE(((1.,1.),(1.,1.),(1.,1.),(1.,1.),(1.,1.),(1.,
1.),(1.,1.),(1.,1.),(1.,1.),(1.,1.),(1.,1.),(1.,1.),(1.,1.),(1.,1.),(1.,
1.),(1.,1.),(1.,1.),(1.,1.),(1.,1.),(1.,1.),(1.,1.),(1.,1.),(1.,1.),(1.,
1.),(1.,1.),(1.,1.),(1.,1.),(1.,1.),(1.,1.),(1.,1.),(1.,1.),(1.,1.),(1.,
1.),(1.,1.),(1.,1.),(1.,1.),(1.,1.),(1.,1.),(1.,1.),(1.,1.)))
REPRESENTATION_ITEM('')
SURFACE()
);
#602=(
BOUNDED_SURFACE()
B_SPLINE_SURFACE(5,1,((#61243,#61244),(#61245,#61246),(#61247,#61248),(#61249,
#61250),(#61251,#61252),(#61253,#61254),(#61255,#61256),(#61257,#61258),
(#61259,#61260),(#61261,#61262),(#61263,#61264),(#61265,#61266),(#61267,
#61268),(#61269,#61270),(#61271,#61272),(#61273,#61274),(#61275,#61276),
(#61277,#61278),(#61279,#61280),(#61281,#61282),(#61283,#61284),(#61285,
#61286),(#61287,#61288),(#61289,#61290),(#61291,#61292),(#61293,#61294),
(#61295,#61296),(#61297,#61298),(#61299,#61300),(#61301,#61302),(#61303,
#61304),(#61305,#61306),(#61307,#61308),(#61309,#61310),(#61311,#61312),
(#61313,#61314),(#61315,#61316),(#61317,#61318),(#61319,#61320),(#61321,
#61322)),.UNSPECIFIED.,.F.,.F.,.F.)
B_SPLINE_SURFACE_WITH_KNOTS((6,1,1,1,1,1,1,1,1,1,1,1,1,1,1,1,1,1,1,1,1,
1,1,1,1,1,1,1,1,1,1,1,1,1,1,6),(2,2),(-1.,-0.971428571428572,-0.942857142857143,
-0.914285714285714,-0.885714285714286,-0.857142857142857,-0.828571428571429,
-0.8,-0.771428571428572,-0.742857142857143,-0.714285714285714,-0.685714285714286,
-0.657142857142857,-0.628571428571429,-0.6,-0.571428571428572,-0.542857142857143,
-0.514285714285714,-0.485714285714286,-0.457142857142857,-0.428571428571429,
-0.4,-0.371428571428571,-0.342857142857143,-0.314285714285714,-0.285714285714286,
-0.257142857142857,-0.228571428571429,-0.2,-0.171428571428571,-0.142857142857143,
-0.114285714285714,-0.0857142857142857,-0.0571428571428571,-0.0285714285714286,
0.),(0.,1.6),.UNSPECIFIED.)
GEOMETRIC_REPRESENTATION_ITEM()
RATIONAL_B_SPLINE_SURFACE(((1.,1.),(1.,1.),(1.,1.),(1.,1.),(1.,1.),(1.,
1.),(1.,1.),(1.,1.),(1.,1.),(1.,1.),(1.,1.),(1.,1.),(1.,1.),(1.,1.),(1.,
1.),(1.,1.),(1.,1.),(1.,1.),(1.,1.),(1.,1.),(1.,1.),(1.,1.),(1.,1.),(1.,
1.),(1.,1.),(1.,1.),(1.,1.),(1.,1.),(1.,1.),(1.,1.),(1.,1.),(1.,1.),(1.,
1.),(1.,1.),(1.,1.),(1.,1.),(1.,1.),(1.,1.),(1.,1.),(1.,1.)))
REPRESENTATION_ITEM('')
SURFACE()
);
#603=(
BOUNDED_SURFACE()
B_SPLINE_SURFACE(5,1,((#61342,#61343),(#61344,#61345),(#61346,#61347),(#61348,
#61349),(#61350,#61351),(#61352,#61353),(#61354,#61355),(#61356,#61357),
(#61358,#61359),(#61360,#61361),(#61362,#61363),(#61364,#61365),(#61366,
#61367),(#61368,#61369),(#61370,#61371),(#61372,#61373),(#61374,#61375),
(#61376,#61377),(#61378,#61379),(#61380,#61381),(#61382,#61383),(#61384,
#61385),(#61386,#61387),(#61388,#61389),(#61390,#61391),(#61392,#61393),
(#61394,#61395),(#61396,#61397),(#61398,#61399),(#61400,#61401),(#61402,
#61403),(#61404,#61405),(#61406,#61407),(#61408,#61409),(#61410,#61411),
(#61412,#61413),(#61414,#61415),(#61416,#61417),(#61418,#61419),(#61420,
#61421)),.UNSPECIFIED.,.F.,.F.,.F.)
B_SPLINE_SURFACE_WITH_KNOTS((6,1,1,1,1,1,1,1,1,1,1,1,1,1,1,1,1,1,1,1,1,
1,1,1,1,1,1,1,1,1,1,1,1,1,1,6),(2,2),(-1.,-0.971428571428572,-0.942857142857143,
-0.914285714285714,-0.885714285714286,-0.857142857142857,-0.828571428571429,
-0.8,-0.771428571428572,-0.742857142857143,-0.714285714285714,-0.685714285714286,
-0.657142857142857,-0.628571428571429,-0.6,-0.571428571428572,-0.542857142857143,
-0.514285714285714,-0.485714285714286,-0.457142857142857,-0.428571428571429,
-0.4,-0.371428571428571,-0.342857142857143,-0.314285714285714,-0.285714285714286,
-0.257142857142857,-0.228571428571429,-0.2,-0.171428571428571,-0.142857142857143,
-0.114285714285714,-0.0857142857142857,-0.0571428571428571,-0.0285714285714286,
0.),(0.,1.6),.UNSPECIFIED.)
GEOMETRIC_REPRESENTATION_ITEM()
RATIONAL_B_SPLINE_SURFACE(((1.,1.),(1.,1.),(1.,1.),(1.,1.),(1.,1.),(1.,
1.),(1.,1.),(1.,1.),(1.,1.),(1.,1.),(1.,1.),(1.,1.),(1.,1.),(1.,1.),(1.,
1.),(1.,1.),(1.,1.),(1.,1.),(1.,1.),(1.,1.),(1.,1.),(1.,1.),(1.,1.),(1.,
1.),(1.,1.),(1.,1.),(1.,1.),(1.,1.),(1.,1.),(1.,1.),(1.,1.),(1.,1.),(1.,
1.),(1.,1.),(1.,1.),(1.,1.),(1.,1.),(1.,1.),(1.,1.),(1.,1.)))
REPRESENTATION_ITEM('')
SURFACE()
);
#604=(
BOUNDED_SURFACE()
B_SPLINE_SURFACE(5,1,((#61441,#61442),(#61443,#61444),(#61445,#61446),(#61447,
#61448),(#61449,#61450),(#61451,#61452),(#61453,#61454),(#61455,#61456),
(#61457,#61458),(#61459,#61460),(#61461,#61462),(#61463,#61464),(#61465,
#61466),(#61467,#61468),(#61469,#61470),(#61471,#61472),(#61473,#61474),
(#61475,#61476),(#61477,#61478),(#61479,#61480),(#61481,#61482),(#61483,
#61484),(#61485,#61486),(#61487,#61488),(#61489,#61490),(#61491,#61492),
(#61493,#61494),(#61495,#61496),(#61497,#61498),(#61499,#61500),(#61501,
#61502),(#61503,#61504),(#61505,#61506),(#61507,#61508),(#61509,#61510),
(#61511,#61512),(#61513,#61514),(#61515,#61516),(#61517,#61518),(#61519,
#61520)),.UNSPECIFIED.,.F.,.F.,.F.)
B_SPLINE_SURFACE_WITH_KNOTS((6,1,1,1,1,1,1,1,1,1,1,1,1,1,1,1,1,1,1,1,1,
1,1,1,1,1,1,1,1,1,1,1,1,1,1,6),(2,2),(-1.,-0.971428571428572,-0.942857142857143,
-0.914285714285714,-0.885714285714286,-0.857142857142857,-0.828571428571429,
-0.8,-0.771428571428572,-0.742857142857143,-0.714285714285714,-0.685714285714286,
-0.657142857142857,-0.628571428571429,-0.6,-0.571428571428572,-0.542857142857143,
-0.514285714285714,-0.485714285714286,-0.457142857142857,-0.428571428571429,
-0.4,-0.371428571428571,-0.342857142857143,-0.314285714285714,-0.285714285714286,
-0.257142857142857,-0.228571428571429,-0.2,-0.171428571428571,-0.142857142857143,
-0.114285714285714,-0.0857142857142857,-0.0571428571428571,-0.0285714285714286,
0.),(0.,1.6),.UNSPECIFIED.)
GEOMETRIC_REPRESENTATION_ITEM()
RATIONAL_B_SPLINE_SURFACE(((1.,1.),(1.,1.),(1.,1.),(1.,1.),(1.,1.),(1.,
1.),(1.,1.),(1.,1.),(1.,1.),(1.,1.),(1.,1.),(1.,1.),(1.,1.),(1.,1.),(1.,
1.),(1.,1.),(1.,1.),(1.,1.),(1.,1.),(1.,1.),(1.,1.),(1.,1.),(1.,1.),(1.,
1.),(1.,1.),(1.,1.),(1.,1.),(1.,1.),(1.,1.),(1.,1.),(1.,1.),(1.,1.),(1.,
1.),(1.,1.),(1.,1.),(1.,1.),(1.,1.),(1.,1.),(1.,1.),(1.,1.)))
REPRESENTATION_ITEM('')
SURFACE()
);
#605=(
BOUNDED_SURFACE()
B_SPLINE_SURFACE(5,1,((#61540,#61541),(#61542,#61543),(#61544,#61545),(#61546,
#61547),(#61548,#61549),(#61550,#61551),(#61552,#61553),(#61554,#61555),
(#61556,#61557),(#61558,#61559),(#61560,#61561),(#61562,#61563),(#61564,
#61565),(#61566,#61567),(#61568,#61569),(#61570,#61571),(#61572,#61573),
(#61574,#61575),(#61576,#61577),(#61578,#61579),(#61580,#61581),(#61582,
#61583),(#61584,#61585),(#61586,#61587),(#61588,#61589),(#61590,#61591),
(#61592,#61593),(#61594,#61595),(#61596,#61597),(#61598,#61599),(#61600,
#61601),(#61602,#61603),(#61604,#61605),(#61606,#61607),(#61608,#61609),
(#61610,#61611),(#61612,#61613),(#61614,#61615),(#61616,#61617),(#61618,
#61619)),.UNSPECIFIED.,.F.,.F.,.F.)
B_SPLINE_SURFACE_WITH_KNOTS((6,1,1,1,1,1,1,1,1,1,1,1,1,1,1,1,1,1,1,1,1,
1,1,1,1,1,1,1,1,1,1,1,1,1,1,6),(2,2),(-1.,-0.971428571428572,-0.942857142857143,
-0.914285714285714,-0.885714285714286,-0.857142857142857,-0.828571428571429,
-0.8,-0.771428571428572,-0.742857142857143,-0.714285714285714,-0.685714285714286,
-0.657142857142857,-0.628571428571429,-0.6,-0.571428571428572,-0.542857142857143,
-0.514285714285714,-0.485714285714286,-0.457142857142857,-0.428571428571429,
-0.4,-0.371428571428571,-0.342857142857143,-0.314285714285714,-0.285714285714286,
-0.257142857142857,-0.228571428571429,-0.2,-0.171428571428571,-0.142857142857143,
-0.114285714285714,-0.0857142857142857,-0.0571428571428571,-0.0285714285714286,
0.),(0.,1.6),.UNSPECIFIED.)
GEOMETRIC_REPRESENTATION_ITEM()
RATIONAL_B_SPLINE_SURFACE(((1.,1.),(1.,1.),(1.,1.),(1.,1.),(1.,1.),(1.,
1.),(1.,1.),(1.,1.),(1.,1.),(1.,1.),(1.,1.),(1.,1.),(1.,1.),(1.,1.),(1.,
1.),(1.,1.),(1.,1.),(1.,1.),(1.,1.),(1.,1.),(1.,1.),(1.,1.),(1.,1.),(1.,
1.),(1.,1.),(1.,1.),(1.,1.),(1.,1.),(1.,1.),(1.,1.),(1.,1.),(1.,1.),(1.,
1.),(1.,1.),(1.,1.),(1.,1.),(1.,1.),(1.,1.),(1.,1.),(1.,1.)))
REPRESENTATION_ITEM('')
SURFACE()
);
#606=(
BOUNDED_SURFACE()
B_SPLINE_SURFACE(5,1,((#61639,#61640),(#61641,#61642),(#61643,#61644),(#61645,
#61646),(#61647,#61648),(#61649,#61650),(#61651,#61652),(#61653,#61654),
(#61655,#61656),(#61657,#61658),(#61659,#61660),(#61661,#61662),(#61663,
#61664),(#61665,#61666),(#61667,#61668),(#61669,#61670),(#61671,#61672),
(#61673,#61674),(#61675,#61676),(#61677,#61678),(#61679,#61680),(#61681,
#61682),(#61683,#61684),(#61685,#61686),(#61687,#61688),(#61689,#61690),
(#61691,#61692),(#61693,#61694),(#61695,#61696),(#61697,#61698),(#61699,
#61700),(#61701,#61702),(#61703,#61704),(#61705,#61706),(#61707,#61708),
(#61709,#61710),(#61711,#61712),(#61713,#61714),(#61715,#61716),(#61717,
#61718)),.UNSPECIFIED.,.F.,.F.,.F.)
B_SPLINE_SURFACE_WITH_KNOTS((6,1,1,1,1,1,1,1,1,1,1,1,1,1,1,1,1,1,1,1,1,
1,1,1,1,1,1,1,1,1,1,1,1,1,1,6),(2,2),(-1.,-0.971428571428572,-0.942857142857143,
-0.914285714285714,-0.885714285714286,-0.857142857142857,-0.828571428571429,
-0.8,-0.771428571428572,-0.742857142857143,-0.714285714285714,-0.685714285714286,
-0.657142857142857,-0.628571428571429,-0.6,-0.571428571428572,-0.542857142857143,
-0.514285714285714,-0.485714285714286,-0.457142857142857,-0.428571428571429,
-0.4,-0.371428571428571,-0.342857142857143,-0.314285714285714,-0.285714285714286,
-0.257142857142857,-0.228571428571429,-0.2,-0.171428571428571,-0.142857142857143,
-0.114285714285714,-0.0857142857142857,-0.0571428571428571,-0.0285714285714286,
0.),(0.,1.6),.UNSPECIFIED.)
GEOMETRIC_REPRESENTATION_ITEM()
RATIONAL_B_SPLINE_SURFACE(((1.,1.),(1.,1.),(1.,1.),(1.,1.),(1.,1.),(1.,
1.),(1.,1.),(1.,1.),(1.,1.),(1.,1.),(1.,1.),(1.,1.),(1.,1.),(1.,1.),(1.,
1.),(1.,1.),(1.,1.),(1.,1.),(1.,1.),(1.,1.),(1.,1.),(1.,1.),(1.,1.),(1.,
1.),(1.,1.),(1.,1.),(1.,1.),(1.,1.),(1.,1.),(1.,1.),(1.,1.),(1.,1.),(1.,
1.),(1.,1.),(1.,1.),(1.,1.),(1.,1.),(1.,1.),(1.,1.),(1.,1.)))
REPRESENTATION_ITEM('')
SURFACE()
);
#607=(
BOUNDED_SURFACE()
B_SPLINE_SURFACE(5,1,((#61738,#61739),(#61740,#61741),(#61742,#61743),(#61744,
#61745),(#61746,#61747),(#61748,#61749),(#61750,#61751),(#61752,#61753),
(#61754,#61755),(#61756,#61757),(#61758,#61759),(#61760,#61761),(#61762,
#61763),(#61764,#61765),(#61766,#61767),(#61768,#61769),(#61770,#61771),
(#61772,#61773),(#61774,#61775),(#61776,#61777),(#61778,#61779),(#61780,
#61781),(#61782,#61783),(#61784,#61785),(#61786,#61787),(#61788,#61789),
(#61790,#61791),(#61792,#61793),(#61794,#61795),(#61796,#61797),(#61798,
#61799),(#61800,#61801),(#61802,#61803),(#61804,#61805),(#61806,#61807),
(#61808,#61809),(#61810,#61811),(#61812,#61813),(#61814,#61815),(#61816,
#61817)),.UNSPECIFIED.,.F.,.F.,.F.)
B_SPLINE_SURFACE_WITH_KNOTS((6,1,1,1,1,1,1,1,1,1,1,1,1,1,1,1,1,1,1,1,1,
1,1,1,1,1,1,1,1,1,1,1,1,1,1,6),(2,2),(-1.,-0.971428571428572,-0.942857142857143,
-0.914285714285714,-0.885714285714286,-0.857142857142857,-0.828571428571429,
-0.8,-0.771428571428572,-0.742857142857143,-0.714285714285714,-0.685714285714286,
-0.657142857142857,-0.628571428571429,-0.6,-0.571428571428572,-0.542857142857143,
-0.514285714285714,-0.485714285714286,-0.457142857142857,-0.428571428571429,
-0.4,-0.371428571428571,-0.342857142857143,-0.314285714285714,-0.285714285714286,
-0.257142857142857,-0.228571428571429,-0.2,-0.171428571428571,-0.142857142857143,
-0.114285714285714,-0.0857142857142857,-0.0571428571428571,-0.0285714285714286,
0.),(0.,1.6),.UNSPECIFIED.)
GEOMETRIC_REPRESENTATION_ITEM()
RATIONAL_B_SPLINE_SURFACE(((1.,1.),(1.,1.),(1.,1.),(1.,1.),(1.,1.),(1.,
1.),(1.,1.),(1.,1.),(1.,1.),(1.,1.),(1.,1.),(1.,1.),(1.,1.),(1.,1.),(1.,
1.),(1.,1.),(1.,1.),(1.,1.),(1.,1.),(1.,1.),(1.,1.),(1.,1.),(1.,1.),(1.,
1.),(1.,1.),(1.,1.),(1.,1.),(1.,1.),(1.,1.),(1.,1.),(1.,1.),(1.,1.),(1.,
1.),(1.,1.),(1.,1.),(1.,1.),(1.,1.),(1.,1.),(1.,1.),(1.,1.)))
REPRESENTATION_ITEM('')
SURFACE()
);
#672=(
BOUNDED_CURVE()
B_SPLINE_CURVE(5,(#49245,#49246,#49247,#49248,#49249,#49250,#49251,#49252,
#49253,#49254,#49255,#49256,#49257,#49258,#49259,#49260,#49261,#49262,#49263,
#49264,#49265,#49266,#49267,#49268,#49269),.UNSPECIFIED.,.F.,.F.)
B_SPLINE_CURVE_WITH_KNOTS((6,1,1,1,1,1,1,1,1,1,1,1,1,1,1,1,1,1,1,1,6),(0.437678095034471,
0.457142857142857,0.485714285714286,0.514285714285714,0.542857142857143,
0.571428571428572,0.6,0.628571428571429,0.657142857142857,0.685714285714286,
0.714285714285714,0.742857142857143,0.771428571428572,0.8,0.828571428571429,
0.857142857142857,0.885714285714286,0.914285714285714,0.942857142857143,
0.971428571428572,1.),.UNSPECIFIED.)
CURVE()
GEOMETRIC_REPRESENTATION_ITEM()
RATIONAL_B_SPLINE_CURVE((1.,1.,1.,1.,1.,1.,1.,1.,1.,1.,1.,1.,1.,1.,1.,1.,
1.,1.,1.,1.,1.,1.,1.,1.,1.))
REPRESENTATION_ITEM('')
);
#673=(
BOUNDED_CURVE()
B_SPLINE_CURVE(5,(#49273,#49274,#49275,#49276,#49277,#49278,#49279,#49280,
#49281,#49282,#49283,#49284,#49285,#49286,#49287,#49288,#49289,#49290,#49291,
#49292,#49293,#49294,#49295,#49296,#49297,#49298,#49299,#49300,#49301),
 .UNSPECIFIED.,.F.,.F.)
B_SPLINE_CURVE_WITH_KNOTS((6,1,1,1,1,1,1,1,1,1,1,1,1,1,1,1,1,1,1,1,1,1,
1,1,6),(0.,0.0285714285714286,0.0571428571428571,0.0857142857142857,0.114285714285714,
0.142857142857143,0.171428571428571,0.2,0.228571428571429,0.257142857142857,
0.285714285714286,0.314285714285714,0.342857142857143,0.371428571428571,
0.4,0.428571428571429,0.457142857142857,0.485714285714286,0.514285714285714,
0.542857142857143,0.571428571428572,0.6,0.628571428571429,0.657142857142857,
0.666463158655954),.UNSPECIFIED.)
CURVE()
GEOMETRIC_REPRESENTATION_ITEM()
RATIONAL_B_SPLINE_CURVE((1.,1.,1.,1.,1.,1.,1.,1.,1.,1.,1.,1.,1.,1.,1.,1.,
1.,1.,1.,1.,1.,1.,1.,1.,1.,1.,1.,1.,1.))
REPRESENTATION_ITEM('')
);
#674=(
BOUNDED_CURVE()
B_SPLINE_CURVE(5,(#49305,#49306,#49307,#49308,#49309,#49310,#49311,#49312,
#49313,#49314,#49315,#49316,#49317,#49318,#49319,#49320,#49321,#49322,#49323,
#49324,#49325,#49326,#49327,#49328,#49329),.UNSPECIFIED.,.F.,.F.)
B_SPLINE_CURVE_WITH_KNOTS((6,1,1,1,1,1,1,1,1,1,1,1,1,1,1,1,1,1,1,1,6),(0.437678095034471,
0.457142857142857,0.485714285714286,0.514285714285714,0.542857142857143,
0.571428571428572,0.6,0.628571428571429,0.657142857142857,0.685714285714286,
0.714285714285714,0.742857142857143,0.771428571428572,0.8,0.828571428571429,
0.857142857142857,0.885714285714286,0.914285714285714,0.942857142857143,
0.971428571428572,1.),.UNSPECIFIED.)
CURVE()
GEOMETRIC_REPRESENTATION_ITEM()
RATIONAL_B_SPLINE_CURVE((1.,1.,1.,1.,1.,1.,1.,1.,1.,1.,1.,1.,1.,1.,1.,1.,
1.,1.,1.,1.,1.,1.,1.,1.,1.))
REPRESENTATION_ITEM('')
);
#675=(
BOUNDED_CURVE()
B_SPLINE_CURVE(5,(#49333,#49334,#49335,#49336,#49337,#49338,#49339,#49340,
#49341,#49342,#49343,#49344,#49345,#49346,#49347,#49348,#49349,#49350,#49351,
#49352,#49353,#49354,#49355,#49356,#49357,#49358,#49359,#49360,#49361),
 .UNSPECIFIED.,.F.,.F.)
B_SPLINE_CURVE_WITH_KNOTS((6,1,1,1,1,1,1,1,1,1,1,1,1,1,1,1,1,1,1,1,1,1,
1,1,6),(0.,0.0285714285714286,0.0571428571428571,0.0857142857142857,0.114285714285714,
0.142857142857143,0.171428571428571,0.2,0.228571428571429,0.257142857142857,
0.285714285714286,0.314285714285714,0.342857142857143,0.371428571428571,
0.4,0.428571428571429,0.457142857142857,0.485714285714286,0.514285714285714,
0.542857142857143,0.571428571428572,0.6,0.628571428571429,0.657142857142857,
0.666463158655954),.UNSPECIFIED.)
CURVE()
GEOMETRIC_REPRESENTATION_ITEM()
RATIONAL_B_SPLINE_CURVE((1.,1.,1.,1.,1.,1.,1.,1.,1.,1.,1.,1.,1.,1.,1.,1.,
1.,1.,1.,1.,1.,1.,1.,1.,1.,1.,1.,1.,1.))
REPRESENTATION_ITEM('')
);
#676=(
BOUNDED_CURVE()
B_SPLINE_CURVE(5,(#49365,#49366,#49367,#49368,#49369,#49370,#49371,#49372,
#49373,#49374,#49375,#49376,#49377,#49378,#49379,#49380,#49381,#49382,#49383,
#49384,#49385,#49386,#49387,#49388,#49389),.UNSPECIFIED.,.F.,.F.)
B_SPLINE_CURVE_WITH_KNOTS((6,1,1,1,1,1,1,1,1,1,1,1,1,1,1,1,1,1,1,1,6),(0.437678095034471,
0.457142857142857,0.485714285714286,0.514285714285714,0.542857142857143,
0.571428571428572,0.6,0.628571428571429,0.657142857142857,0.685714285714286,
0.714285714285714,0.742857142857143,0.771428571428572,0.8,0.828571428571429,
0.857142857142857,0.885714285714286,0.914285714285714,0.942857142857143,
0.971428571428572,1.),.UNSPECIFIED.)
CURVE()
GEOMETRIC_REPRESENTATION_ITEM()
RATIONAL_B_SPLINE_CURVE((1.,1.,1.,1.,1.,1.,1.,1.,1.,1.,1.,1.,1.,1.,1.,1.,
1.,1.,1.,1.,1.,1.,1.,1.,1.))
REPRESENTATION_ITEM('')
);
#677=(
BOUNDED_CURVE()
B_SPLINE_CURVE(5,(#49393,#49394,#49395,#49396,#49397,#49398,#49399,#49400,
#49401,#49402,#49403,#49404,#49405,#49406,#49407,#49408,#49409,#49410,#49411,
#49412,#49413,#49414,#49415,#49416,#49417,#49418,#49419,#49420,#49421),
 .UNSPECIFIED.,.F.,.F.)
B_SPLINE_CURVE_WITH_KNOTS((6,1,1,1,1,1,1,1,1,1,1,1,1,1,1,1,1,1,1,1,1,1,
1,1,6),(0.,0.0285714285714286,0.0571428571428571,0.0857142857142857,0.114285714285714,
0.142857142857143,0.171428571428571,0.2,0.228571428571429,0.257142857142857,
0.285714285714286,0.314285714285714,0.342857142857143,0.371428571428571,
0.4,0.428571428571429,0.457142857142857,0.485714285714286,0.514285714285714,
0.542857142857143,0.571428571428572,0.6,0.628571428571429,0.657142857142857,
0.666463158655955),.UNSPECIFIED.)
CURVE()
GEOMETRIC_REPRESENTATION_ITEM()
RATIONAL_B_SPLINE_CURVE((1.,1.,1.,1.,1.,1.,1.,1.,1.,1.,1.,1.,1.,1.,1.,1.,
1.,1.,1.,1.,1.,1.,1.,1.,1.,1.,1.,1.,1.))
REPRESENTATION_ITEM('')
);
#678=(
BOUNDED_CURVE()
B_SPLINE_CURVE(5,(#49425,#49426,#49427,#49428,#49429,#49430,#49431,#49432,
#49433,#49434,#49435,#49436,#49437,#49438,#49439,#49440,#49441,#49442,#49443,
#49444,#49445,#49446,#49447,#49448,#49449),.UNSPECIFIED.,.F.,.F.)
B_SPLINE_CURVE_WITH_KNOTS((6,1,1,1,1,1,1,1,1,1,1,1,1,1,1,1,1,1,1,1,6),(0.437678095034471,
0.457142857142857,0.485714285714286,0.514285714285714,0.542857142857143,
0.571428571428572,0.6,0.628571428571429,0.657142857142857,0.685714285714286,
0.714285714285714,0.742857142857143,0.771428571428572,0.8,0.828571428571429,
0.857142857142857,0.885714285714286,0.914285714285714,0.942857142857143,
0.971428571428572,1.),.UNSPECIFIED.)
CURVE()
GEOMETRIC_REPRESENTATION_ITEM()
RATIONAL_B_SPLINE_CURVE((1.,1.,1.,1.,1.,1.,1.,1.,1.,1.,1.,1.,1.,1.,1.,1.,
1.,1.,1.,1.,1.,1.,1.,1.,1.))
REPRESENTATION_ITEM('')
);
#679=(
BOUNDED_CURVE()
B_SPLINE_CURVE(5,(#49453,#49454,#49455,#49456,#49457,#49458,#49459,#49460,
#49461,#49462,#49463,#49464,#49465,#49466,#49467,#49468,#49469,#49470,#49471,
#49472,#49473,#49474,#49475,#49476,#49477,#49478,#49479,#49480,#49481),
 .UNSPECIFIED.,.F.,.F.)
B_SPLINE_CURVE_WITH_KNOTS((6,1,1,1,1,1,1,1,1,1,1,1,1,1,1,1,1,1,1,1,1,1,
1,1,6),(0.,0.0285714285714286,0.0571428571428571,0.0857142857142857,0.114285714285714,
0.142857142857143,0.171428571428571,0.2,0.228571428571429,0.257142857142857,
0.285714285714286,0.314285714285714,0.342857142857143,0.371428571428571,
0.4,0.428571428571429,0.457142857142857,0.485714285714286,0.514285714285714,
0.542857142857143,0.571428571428572,0.6,0.628571428571429,0.657142857142857,
0.666463158655954),.UNSPECIFIED.)
CURVE()
GEOMETRIC_REPRESENTATION_ITEM()
RATIONAL_B_SPLINE_CURVE((1.,1.,1.,1.,1.,1.,1.,1.,1.,1.,1.,1.,1.,1.,1.,1.,
1.,1.,1.,1.,1.,1.,1.,1.,1.,1.,1.,1.,1.))
REPRESENTATION_ITEM('')
);
#680=(
BOUNDED_CURVE()
B_SPLINE_CURVE(5,(#49485,#49486,#49487,#49488,#49489,#49490,#49491,#49492,
#49493,#49494,#49495,#49496,#49497,#49498,#49499,#49500,#49501,#49502,#49503,
#49504,#49505,#49506,#49507,#49508,#49509),.UNSPECIFIED.,.F.,.F.)
B_SPLINE_CURVE_WITH_KNOTS((6,1,1,1,1,1,1,1,1,1,1,1,1,1,1,1,1,1,1,1,6),(0.437678095034471,
0.457142857142857,0.485714285714286,0.514285714285714,0.542857142857143,
0.571428571428572,0.6,0.628571428571429,0.657142857142857,0.685714285714286,
0.714285714285714,0.742857142857143,0.771428571428572,0.8,0.828571428571429,
0.857142857142857,0.885714285714286,0.914285714285714,0.942857142857143,
0.971428571428572,1.),.UNSPECIFIED.)
CURVE()
GEOMETRIC_REPRESENTATION_ITEM()
RATIONAL_B_SPLINE_CURVE((1.,1.,1.,1.,1.,1.,1.,1.,1.,1.,1.,1.,1.,1.,1.,1.,
1.,1.,1.,1.,1.,1.,1.,1.,1.))
REPRESENTATION_ITEM('')
);
#681=(
BOUNDED_CURVE()
B_SPLINE_CURVE(5,(#49513,#49514,#49515,#49516,#49517,#49518,#49519,#49520,
#49521,#49522,#49523,#49524,#49525,#49526,#49527,#49528,#49529,#49530,#49531,
#49532,#49533,#49534,#49535,#49536,#49537,#49538,#49539,#49540,#49541),
 .UNSPECIFIED.,.F.,.F.)
B_SPLINE_CURVE_WITH_KNOTS((6,1,1,1,1,1,1,1,1,1,1,1,1,1,1,1,1,1,1,1,1,1,
1,1,6),(0.,0.0285714285714286,0.0571428571428571,0.0857142857142857,0.114285714285714,
0.142857142857143,0.171428571428571,0.2,0.228571428571429,0.257142857142857,
0.285714285714286,0.314285714285714,0.342857142857143,0.371428571428571,
0.4,0.428571428571429,0.457142857142857,0.485714285714286,0.514285714285714,
0.542857142857143,0.571428571428572,0.6,0.628571428571429,0.657142857142857,
0.666463158655954),.UNSPECIFIED.)
CURVE()
GEOMETRIC_REPRESENTATION_ITEM()
RATIONAL_B_SPLINE_CURVE((1.,1.,1.,1.,1.,1.,1.,1.,1.,1.,1.,1.,1.,1.,1.,1.,
1.,1.,1.,1.,1.,1.,1.,1.,1.,1.,1.,1.,1.))
REPRESENTATION_ITEM('')
);
#682=(
BOUNDED_CURVE()
B_SPLINE_CURVE(5,(#49545,#49546,#49547,#49548,#49549,#49550,#49551,#49552,
#49553,#49554,#49555,#49556,#49557,#49558,#49559,#49560,#49561,#49562,#49563,
#49564,#49565,#49566,#49567,#49568,#49569),.UNSPECIFIED.,.F.,.F.)
B_SPLINE_CURVE_WITH_KNOTS((6,1,1,1,1,1,1,1,1,1,1,1,1,1,1,1,1,1,1,1,6),(0.437678095034471,
0.457142857142857,0.485714285714286,0.514285714285714,0.542857142857143,
0.571428571428572,0.6,0.628571428571429,0.657142857142857,0.685714285714286,
0.714285714285714,0.742857142857143,0.771428571428572,0.8,0.828571428571429,
0.857142857142857,0.885714285714286,0.914285714285714,0.942857142857143,
0.971428571428572,1.),.UNSPECIFIED.)
CURVE()
GEOMETRIC_REPRESENTATION_ITEM()
RATIONAL_B_SPLINE_CURVE((1.,1.,1.,1.,1.,1.,1.,1.,1.,1.,1.,1.,1.,1.,1.,1.,
1.,1.,1.,1.,1.,1.,1.,1.,1.))
REPRESENTATION_ITEM('')
);
#683=(
BOUNDED_CURVE()
B_SPLINE_CURVE(5,(#49573,#49574,#49575,#49576,#49577,#49578,#49579,#49580,
#49581,#49582,#49583,#49584,#49585,#49586,#49587,#49588,#49589,#49590,#49591,
#49592,#49593,#49594,#49595,#49596,#49597,#49598,#49599,#49600,#49601),
 .UNSPECIFIED.,.F.,.F.)
B_SPLINE_CURVE_WITH_KNOTS((6,1,1,1,1,1,1,1,1,1,1,1,1,1,1,1,1,1,1,1,1,1,
1,1,6),(0.,0.0285714285714286,0.0571428571428571,0.0857142857142857,0.114285714285714,
0.142857142857143,0.171428571428571,0.2,0.228571428571429,0.257142857142857,
0.285714285714286,0.314285714285714,0.342857142857143,0.371428571428571,
0.4,0.428571428571429,0.457142857142857,0.485714285714286,0.514285714285714,
0.542857142857143,0.571428571428572,0.6,0.628571428571429,0.657142857142857,
0.666463158655954),.UNSPECIFIED.)
CURVE()
GEOMETRIC_REPRESENTATION_ITEM()
RATIONAL_B_SPLINE_CURVE((1.,1.,1.,1.,1.,1.,1.,1.,1.,1.,1.,1.,1.,1.,1.,1.,
1.,1.,1.,1.,1.,1.,1.,1.,1.,1.,1.,1.,1.))
REPRESENTATION_ITEM('')
);
#684=(
BOUNDED_CURVE()
B_SPLINE_CURVE(5,(#49605,#49606,#49607,#49608,#49609,#49610,#49611,#49612,
#49613,#49614,#49615,#49616,#49617,#49618,#49619,#49620,#49621,#49622,#49623,
#49624,#49625,#49626,#49627,#49628,#49629),.UNSPECIFIED.,.F.,.F.)
B_SPLINE_CURVE_WITH_KNOTS((6,1,1,1,1,1,1,1,1,1,1,1,1,1,1,1,1,1,1,1,6),(0.437678095034471,
0.457142857142857,0.485714285714286,0.514285714285714,0.542857142857143,
0.571428571428572,0.6,0.628571428571429,0.657142857142857,0.685714285714286,
0.714285714285714,0.742857142857143,0.771428571428572,0.8,0.828571428571429,
0.857142857142857,0.885714285714286,0.914285714285714,0.942857142857143,
0.971428571428572,1.),.UNSPECIFIED.)
CURVE()
GEOMETRIC_REPRESENTATION_ITEM()
RATIONAL_B_SPLINE_CURVE((1.,1.,1.,1.,1.,1.,1.,1.,1.,1.,1.,1.,1.,1.,1.,1.,
1.,1.,1.,1.,1.,1.,1.,1.,1.))
REPRESENTATION_ITEM('')
);
#685=(
BOUNDED_CURVE()
B_SPLINE_CURVE(5,(#49633,#49634,#49635,#49636,#49637,#49638,#49639,#49640,
#49641,#49642,#49643,#49644,#49645,#49646,#49647,#49648,#49649,#49650,#49651,
#49652,#49653,#49654,#49655,#49656,#49657,#49658,#49659,#49660,#49661),
 .UNSPECIFIED.,.F.,.F.)
B_SPLINE_CURVE_WITH_KNOTS((6,1,1,1,1,1,1,1,1,1,1,1,1,1,1,1,1,1,1,1,1,1,
1,1,6),(0.,0.0285714285714286,0.0571428571428571,0.0857142857142857,0.114285714285714,
0.142857142857143,0.171428571428571,0.2,0.228571428571429,0.257142857142857,
0.285714285714286,0.314285714285714,0.342857142857143,0.371428571428571,
0.4,0.428571428571429,0.457142857142857,0.485714285714286,0.514285714285714,
0.542857142857143,0.571428571428572,0.6,0.628571428571429,0.657142857142857,
0.666463158655955),.UNSPECIFIED.)
CURVE()
GEOMETRIC_REPRESENTATION_ITEM()
RATIONAL_B_SPLINE_CURVE((1.,1.,1.,1.,1.,1.,1.,1.,1.,1.,1.,1.,1.,1.,1.,1.,
1.,1.,1.,1.,1.,1.,1.,1.,1.,1.,1.,1.,1.))
REPRESENTATION_ITEM('')
);
#686=(
BOUNDED_CURVE()
B_SPLINE_CURVE(5,(#49665,#49666,#49667,#49668,#49669,#49670,#49671,#49672,
#49673,#49674,#49675,#49676,#49677,#49678,#49679,#49680,#49681,#49682,#49683,
#49684,#49685,#49686,#49687,#49688,#49689),.UNSPECIFIED.,.F.,.F.)
B_SPLINE_CURVE_WITH_KNOTS((6,1,1,1,1,1,1,1,1,1,1,1,1,1,1,1,1,1,1,1,6),(0.437678095034471,
0.457142857142857,0.485714285714286,0.514285714285714,0.542857142857143,
0.571428571428572,0.6,0.628571428571429,0.657142857142857,0.685714285714286,
0.714285714285714,0.742857142857143,0.771428571428572,0.8,0.828571428571429,
0.857142857142857,0.885714285714286,0.914285714285714,0.942857142857143,
0.971428571428572,1.),.UNSPECIFIED.)
CURVE()
GEOMETRIC_REPRESENTATION_ITEM()
RATIONAL_B_SPLINE_CURVE((1.,1.,1.,1.,1.,1.,1.,1.,1.,1.,1.,1.,1.,1.,1.,1.,
1.,1.,1.,1.,1.,1.,1.,1.,1.))
REPRESENTATION_ITEM('')
);
#687=(
BOUNDED_CURVE()
B_SPLINE_CURVE(5,(#49693,#49694,#49695,#49696,#49697,#49698,#49699,#49700,
#49701,#49702,#49703,#49704,#49705,#49706,#49707,#49708,#49709,#49710,#49711,
#49712,#49713,#49714,#49715,#49716,#49717,#49718,#49719,#49720,#49721),
 .UNSPECIFIED.,.F.,.F.)
B_SPLINE_CURVE_WITH_KNOTS((6,1,1,1,1,1,1,1,1,1,1,1,1,1,1,1,1,1,1,1,1,1,
1,1,6),(0.,0.0285714285714286,0.0571428571428571,0.0857142857142857,0.114285714285714,
0.142857142857143,0.171428571428571,0.2,0.228571428571429,0.257142857142857,
0.285714285714286,0.314285714285714,0.342857142857143,0.371428571428571,
0.4,0.428571428571429,0.457142857142857,0.485714285714286,0.514285714285714,
0.542857142857143,0.571428571428572,0.6,0.628571428571429,0.657142857142857,
0.666463158655954),.UNSPECIFIED.)
CURVE()
GEOMETRIC_REPRESENTATION_ITEM()
RATIONAL_B_SPLINE_CURVE((1.,1.,1.,1.,1.,1.,1.,1.,1.,1.,1.,1.,1.,1.,1.,1.,
1.,1.,1.,1.,1.,1.,1.,1.,1.,1.,1.,1.,1.))
REPRESENTATION_ITEM('')
);
#688=(
BOUNDED_CURVE()
B_SPLINE_CURVE(5,(#49725,#49726,#49727,#49728,#49729,#49730,#49731,#49732,
#49733,#49734,#49735,#49736,#49737,#49738,#49739,#49740,#49741,#49742,#49743,
#49744,#49745,#49746,#49747,#49748,#49749),.UNSPECIFIED.,.F.,.F.)
B_SPLINE_CURVE_WITH_KNOTS((6,1,1,1,1,1,1,1,1,1,1,1,1,1,1,1,1,1,1,1,6),(0.437678095034471,
0.457142857142857,0.485714285714286,0.514285714285714,0.542857142857143,
0.571428571428572,0.6,0.628571428571429,0.657142857142857,0.685714285714286,
0.714285714285714,0.742857142857143,0.771428571428572,0.8,0.828571428571429,
0.857142857142857,0.885714285714286,0.914285714285714,0.942857142857143,
0.971428571428572,1.),.UNSPECIFIED.)
CURVE()
GEOMETRIC_REPRESENTATION_ITEM()
RATIONAL_B_SPLINE_CURVE((1.,1.,1.,1.,1.,1.,1.,1.,1.,1.,1.,1.,1.,1.,1.,1.,
1.,1.,1.,1.,1.,1.,1.,1.,1.))
REPRESENTATION_ITEM('')
);
#689=(
BOUNDED_CURVE()
B_SPLINE_CURVE(5,(#49753,#49754,#49755,#49756,#49757,#49758,#49759,#49760,
#49761,#49762,#49763,#49764,#49765,#49766,#49767,#49768,#49769,#49770,#49771,
#49772,#49773,#49774,#49775,#49776,#49777,#49778,#49779,#49780,#49781),
 .UNSPECIFIED.,.F.,.F.)
B_SPLINE_CURVE_WITH_KNOTS((6,1,1,1,1,1,1,1,1,1,1,1,1,1,1,1,1,1,1,1,1,1,
1,1,6),(0.,0.0285714285714286,0.0571428571428571,0.0857142857142857,0.114285714285714,
0.142857142857143,0.171428571428571,0.2,0.228571428571429,0.257142857142857,
0.285714285714286,0.314285714285714,0.342857142857143,0.371428571428571,
0.4,0.428571428571429,0.457142857142857,0.485714285714286,0.514285714285714,
0.542857142857143,0.571428571428572,0.6,0.628571428571429,0.657142857142857,
0.666463158655955),.UNSPECIFIED.)
CURVE()
GEOMETRIC_REPRESENTATION_ITEM()
RATIONAL_B_SPLINE_CURVE((1.,1.,1.,1.,1.,1.,1.,1.,1.,1.,1.,1.,1.,1.,1.,1.,
1.,1.,1.,1.,1.,1.,1.,1.,1.,1.,1.,1.,1.))
REPRESENTATION_ITEM('')
);
#690=(
BOUNDED_CURVE()
B_SPLINE_CURVE(5,(#49785,#49786,#49787,#49788,#49789,#49790,#49791,#49792,
#49793,#49794,#49795,#49796,#49797,#49798,#49799,#49800,#49801,#49802,#49803,
#49804,#49805,#49806,#49807,#49808,#49809),.UNSPECIFIED.,.F.,.F.)
B_SPLINE_CURVE_WITH_KNOTS((6,1,1,1,1,1,1,1,1,1,1,1,1,1,1,1,1,1,1,1,6),(0.437678095034471,
0.457142857142857,0.485714285714286,0.514285714285714,0.542857142857143,
0.571428571428572,0.6,0.628571428571429,0.657142857142857,0.685714285714286,
0.714285714285714,0.742857142857143,0.771428571428572,0.8,0.828571428571429,
0.857142857142857,0.885714285714286,0.914285714285714,0.942857142857143,
0.971428571428572,1.),.UNSPECIFIED.)
CURVE()
GEOMETRIC_REPRESENTATION_ITEM()
RATIONAL_B_SPLINE_CURVE((1.,1.,1.,1.,1.,1.,1.,1.,1.,1.,1.,1.,1.,1.,1.,1.,
1.,1.,1.,1.,1.,1.,1.,1.,1.))
REPRESENTATION_ITEM('')
);
#691=(
BOUNDED_CURVE()
B_SPLINE_CURVE(5,(#49813,#49814,#49815,#49816,#49817,#49818,#49819,#49820,
#49821,#49822,#49823,#49824,#49825,#49826,#49827,#49828,#49829,#49830,#49831,
#49832,#49833,#49834,#49835,#49836,#49837,#49838,#49839,#49840,#49841),
 .UNSPECIFIED.,.F.,.F.)
B_SPLINE_CURVE_WITH_KNOTS((6,1,1,1,1,1,1,1,1,1,1,1,1,1,1,1,1,1,1,1,1,1,
1,1,6),(0.,0.0285714285714286,0.0571428571428571,0.0857142857142857,0.114285714285714,
0.142857142857143,0.171428571428571,0.2,0.228571428571429,0.257142857142857,
0.285714285714286,0.314285714285714,0.342857142857143,0.371428571428571,
0.4,0.428571428571429,0.457142857142857,0.485714285714286,0.514285714285714,
0.542857142857143,0.571428571428572,0.6,0.628571428571429,0.657142857142857,
0.666463158655954),.UNSPECIFIED.)
CURVE()
GEOMETRIC_REPRESENTATION_ITEM()
RATIONAL_B_SPLINE_CURVE((1.,1.,1.,1.,1.,1.,1.,1.,1.,1.,1.,1.,1.,1.,1.,1.,
1.,1.,1.,1.,1.,1.,1.,1.,1.,1.,1.,1.,1.))
REPRESENTATION_ITEM('')
);
#692=(
BOUNDED_CURVE()
B_SPLINE_CURVE(5,(#49845,#49846,#49847,#49848,#49849,#49850,#49851,#49852,
#49853,#49854,#49855,#49856,#49857,#49858,#49859,#49860,#49861,#49862,#49863,
#49864,#49865,#49866,#49867,#49868,#49869),.UNSPECIFIED.,.F.,.F.)
B_SPLINE_CURVE_WITH_KNOTS((6,1,1,1,1,1,1,1,1,1,1,1,1,1,1,1,1,1,1,1,6),(0.437678095034471,
0.457142857142857,0.485714285714286,0.514285714285714,0.542857142857143,
0.571428571428572,0.6,0.628571428571429,0.657142857142857,0.685714285714286,
0.714285714285714,0.742857142857143,0.771428571428572,0.8,0.828571428571429,
0.857142857142857,0.885714285714286,0.914285714285714,0.942857142857143,
0.971428571428572,1.),.UNSPECIFIED.)
CURVE()
GEOMETRIC_REPRESENTATION_ITEM()
RATIONAL_B_SPLINE_CURVE((1.,1.,1.,1.,1.,1.,1.,1.,1.,1.,1.,1.,1.,1.,1.,1.,
1.,1.,1.,1.,1.,1.,1.,1.,1.))
REPRESENTATION_ITEM('')
);
#693=(
BOUNDED_CURVE()
B_SPLINE_CURVE(5,(#49873,#49874,#49875,#49876,#49877,#49878,#49879,#49880,
#49881,#49882,#49883,#49884,#49885,#49886,#49887,#49888,#49889,#49890,#49891,
#49892,#49893,#49894,#49895,#49896,#49897,#49898,#49899,#49900,#49901),
 .UNSPECIFIED.,.F.,.F.)
B_SPLINE_CURVE_WITH_KNOTS((6,1,1,1,1,1,1,1,1,1,1,1,1,1,1,1,1,1,1,1,1,1,
1,1,6),(0.,0.0285714285714286,0.0571428571428571,0.0857142857142857,0.114285714285714,
0.142857142857143,0.171428571428571,0.2,0.228571428571429,0.257142857142857,
0.285714285714286,0.314285714285714,0.342857142857143,0.371428571428571,
0.4,0.428571428571429,0.457142857142857,0.485714285714286,0.514285714285714,
0.542857142857143,0.571428571428572,0.6,0.628571428571429,0.657142857142857,
0.666463158655955),.UNSPECIFIED.)
CURVE()
GEOMETRIC_REPRESENTATION_ITEM()
RATIONAL_B_SPLINE_CURVE((1.,1.,1.,1.,1.,1.,1.,1.,1.,1.,1.,1.,1.,1.,1.,1.,
1.,1.,1.,1.,1.,1.,1.,1.,1.,1.,1.,1.,1.))
REPRESENTATION_ITEM('')
);
#694=(
BOUNDED_CURVE()
B_SPLINE_CURVE(5,(#49905,#49906,#49907,#49908,#49909,#49910,#49911,#49912,
#49913,#49914,#49915,#49916,#49917,#49918,#49919,#49920,#49921,#49922,#49923,
#49924,#49925,#49926,#49927,#49928,#49929),.UNSPECIFIED.,.F.,.F.)
B_SPLINE_CURVE_WITH_KNOTS((6,1,1,1,1,1,1,1,1,1,1,1,1,1,1,1,1,1,1,1,6),(0.437678095034471,
0.457142857142857,0.485714285714286,0.514285714285714,0.542857142857143,
0.571428571428572,0.6,0.628571428571429,0.657142857142857,0.685714285714286,
0.714285714285714,0.742857142857143,0.771428571428572,0.8,0.828571428571429,
0.857142857142857,0.885714285714286,0.914285714285714,0.942857142857143,
0.971428571428572,1.),.UNSPECIFIED.)
CURVE()
GEOMETRIC_REPRESENTATION_ITEM()
RATIONAL_B_SPLINE_CURVE((1.,1.,1.,1.,1.,1.,1.,1.,1.,1.,1.,1.,1.,1.,1.,1.,
1.,1.,1.,1.,1.,1.,1.,1.,1.))
REPRESENTATION_ITEM('')
);
#695=(
BOUNDED_CURVE()
B_SPLINE_CURVE(5,(#49933,#49934,#49935,#49936,#49937,#49938,#49939,#49940,
#49941,#49942,#49943,#49944,#49945,#49946,#49947,#49948,#49949,#49950,#49951,
#49952,#49953,#49954,#49955,#49956,#49957,#49958,#49959,#49960,#49961),
 .UNSPECIFIED.,.F.,.F.)
B_SPLINE_CURVE_WITH_KNOTS((6,1,1,1,1,1,1,1,1,1,1,1,1,1,1,1,1,1,1,1,1,1,
1,1,6),(0.,0.0285714285714286,0.0571428571428571,0.0857142857142857,0.114285714285714,
0.142857142857143,0.171428571428571,0.2,0.228571428571429,0.257142857142857,
0.285714285714286,0.314285714285714,0.342857142857143,0.371428571428571,
0.4,0.428571428571429,0.457142857142857,0.485714285714286,0.514285714285714,
0.542857142857143,0.571428571428572,0.6,0.628571428571429,0.657142857142857,
0.666463158655955),.UNSPECIFIED.)
CURVE()
GEOMETRIC_REPRESENTATION_ITEM()
RATIONAL_B_SPLINE_CURVE((1.,1.,1.,1.,1.,1.,1.,1.,1.,1.,1.,1.,1.,1.,1.,1.,
1.,1.,1.,1.,1.,1.,1.,1.,1.,1.,1.,1.,1.))
REPRESENTATION_ITEM('')
);
#696=(
BOUNDED_CURVE()
B_SPLINE_CURVE(5,(#49965,#49966,#49967,#49968,#49969,#49970,#49971,#49972,
#49973,#49974,#49975,#49976,#49977,#49978,#49979,#49980,#49981,#49982,#49983,
#49984,#49985,#49986,#49987,#49988,#49989),.UNSPECIFIED.,.F.,.F.)
B_SPLINE_CURVE_WITH_KNOTS((6,1,1,1,1,1,1,1,1,1,1,1,1,1,1,1,1,1,1,1,6),(0.437678095034471,
0.457142857142857,0.485714285714286,0.514285714285714,0.542857142857143,
0.571428571428572,0.6,0.628571428571429,0.657142857142857,0.685714285714286,
0.714285714285714,0.742857142857143,0.771428571428572,0.8,0.828571428571429,
0.857142857142857,0.885714285714286,0.914285714285714,0.942857142857143,
0.971428571428572,1.),.UNSPECIFIED.)
CURVE()
GEOMETRIC_REPRESENTATION_ITEM()
RATIONAL_B_SPLINE_CURVE((1.,1.,1.,1.,1.,1.,1.,1.,1.,1.,1.,1.,1.,1.,1.,1.,
1.,1.,1.,1.,1.,1.,1.,1.,1.))
REPRESENTATION_ITEM('')
);
#697=(
BOUNDED_CURVE()
B_SPLINE_CURVE(5,(#49993,#49994,#49995,#49996,#49997,#49998,#49999,#50000,
#50001,#50002,#50003,#50004,#50005,#50006,#50007,#50008,#50009,#50010,#50011,
#50012,#50013,#50014,#50015,#50016,#50017,#50018,#50019,#50020,#50021),
 .UNSPECIFIED.,.F.,.F.)
B_SPLINE_CURVE_WITH_KNOTS((6,1,1,1,1,1,1,1,1,1,1,1,1,1,1,1,1,1,1,1,1,1,
1,1,6),(0.,0.0285714285714286,0.0571428571428571,0.0857142857142857,0.114285714285714,
0.142857142857143,0.171428571428571,0.2,0.228571428571429,0.257142857142857,
0.285714285714286,0.314285714285714,0.342857142857143,0.371428571428571,
0.4,0.428571428571429,0.457142857142857,0.485714285714286,0.514285714285714,
0.542857142857143,0.571428571428572,0.6,0.628571428571429,0.657142857142857,
0.666463158655954),.UNSPECIFIED.)
CURVE()
GEOMETRIC_REPRESENTATION_ITEM()
RATIONAL_B_SPLINE_CURVE((1.,1.,1.,1.,1.,1.,1.,1.,1.,1.,1.,1.,1.,1.,1.,1.,
1.,1.,1.,1.,1.,1.,1.,1.,1.,1.,1.,1.,1.))
REPRESENTATION_ITEM('')
);
#698=(
BOUNDED_CURVE()
B_SPLINE_CURVE(5,(#50025,#50026,#50027,#50028,#50029,#50030,#50031,#50032,
#50033,#50034,#50035,#50036,#50037,#50038,#50039,#50040,#50041,#50042,#50043,
#50044,#50045,#50046,#50047,#50048,#50049),.UNSPECIFIED.,.F.,.F.)
B_SPLINE_CURVE_WITH_KNOTS((6,1,1,1,1,1,1,1,1,1,1,1,1,1,1,1,1,1,1,1,6),(0.437678095034471,
0.457142857142857,0.485714285714286,0.514285714285714,0.542857142857143,
0.571428571428572,0.6,0.628571428571429,0.657142857142857,0.685714285714286,
0.714285714285714,0.742857142857143,0.771428571428572,0.8,0.828571428571429,
0.857142857142857,0.885714285714286,0.914285714285714,0.942857142857143,
0.971428571428572,1.),.UNSPECIFIED.)
CURVE()
GEOMETRIC_REPRESENTATION_ITEM()
RATIONAL_B_SPLINE_CURVE((1.,1.,1.,1.,1.,1.,1.,1.,1.,1.,1.,1.,1.,1.,1.,1.,
1.,1.,1.,1.,1.,1.,1.,1.,1.))
REPRESENTATION_ITEM('')
);
#699=(
BOUNDED_CURVE()
B_SPLINE_CURVE(5,(#50053,#50054,#50055,#50056,#50057,#50058,#50059,#50060,
#50061,#50062,#50063,#50064,#50065,#50066,#50067,#50068,#50069,#50070,#50071,
#50072,#50073,#50074,#50075,#50076,#50077,#50078,#50079,#50080,#50081),
 .UNSPECIFIED.,.F.,.F.)
B_SPLINE_CURVE_WITH_KNOTS((6,1,1,1,1,1,1,1,1,1,1,1,1,1,1,1,1,1,1,1,1,1,
1,1,6),(0.,0.0285714285714286,0.0571428571428571,0.0857142857142857,0.114285714285714,
0.142857142857143,0.171428571428571,0.2,0.228571428571429,0.257142857142857,
0.285714285714286,0.314285714285714,0.342857142857143,0.371428571428571,
0.4,0.428571428571429,0.457142857142857,0.485714285714286,0.514285714285714,
0.542857142857143,0.571428571428572,0.6,0.628571428571429,0.657142857142857,
0.666463158655955),.UNSPECIFIED.)
CURVE()
GEOMETRIC_REPRESENTATION_ITEM()
RATIONAL_B_SPLINE_CURVE((1.,1.,1.,1.,1.,1.,1.,1.,1.,1.,1.,1.,1.,1.,1.,1.,
1.,1.,1.,1.,1.,1.,1.,1.,1.,1.,1.,1.,1.))
REPRESENTATION_ITEM('')
);
#700=(
BOUNDED_CURVE()
B_SPLINE_CURVE(5,(#50090,#50091,#50092,#50093,#50094,#50095,#50096,#50097,
#50098,#50099,#50100,#50101,#50102,#50103,#50104,#50105,#50106,#50107,#50108,
#50109,#50110,#50111,#50112,#50113,#50114,#50115,#50116,#50117,#50118),
 .UNSPECIFIED.,.F.,.F.)
B_SPLINE_CURVE_WITH_KNOTS((6,1,1,1,1,1,1,1,1,1,1,1,1,1,1,1,1,1,1,1,1,1,
1,1,6),(-0.670627588953113,-0.657142857142857,-0.628571428571429,-0.6,-0.571428571428572,
-0.542857142857143,-0.514285714285714,-0.485714285714286,-0.457142857142857,
-0.428571428571429,-0.4,-0.371428571428571,-0.342857142857143,-0.314285714285714,
-0.285714285714286,-0.257142857142857,-0.228571428571429,-0.2,-0.171428571428571,
-0.142857142857143,-0.114285714285714,-0.0857142857142857,-0.0571428571428571,
-0.0285714285714286,0.),.UNSPECIFIED.)
CURVE()
GEOMETRIC_REPRESENTATION_ITEM()
RATIONAL_B_SPLINE_CURVE((1.,1.,1.,1.,1.,1.,1.,1.,1.,1.,1.,1.,1.,1.,1.,1.,
1.,1.,1.,1.,1.,1.,1.,1.,1.,1.,1.,1.,1.))
REPRESENTATION_ITEM('')
);
#701=(
BOUNDED_CURVE()
B_SPLINE_CURVE(5,(#50122,#50123,#50124,#50125,#50126,#50127,#50128,#50129,
#50130,#50131,#50132,#50133,#50134,#50135,#50136,#50137,#50138,#50139,#50140,
#50141,#50142,#50143,#50144,#50145,#50146,#50147),.UNSPECIFIED.,.F.,.F.)
B_SPLINE_CURVE_WITH_KNOTS((6,1,1,1,1,1,1,1,1,1,1,1,1,1,1,1,1,1,1,1,1,6),
(-1.,-0.971428571428572,-0.942857142857143,-0.914285714285714,-0.885714285714286,
-0.857142857142857,-0.828571428571429,-0.8,-0.771428571428572,-0.742857142857143,
-0.714285714285714,-0.685714285714286,-0.657142857142857,-0.628571428571429,
-0.6,-0.571428571428572,-0.542857142857143,-0.514285714285714,-0.485714285714286,
-0.457142857142857,-0.428571428571429,-0.428061295609926),.UNSPECIFIED.)
CURVE()
GEOMETRIC_REPRESENTATION_ITEM()
RATIONAL_B_SPLINE_CURVE((1.,1.,1.,1.,1.,1.,1.,1.,1.,1.,1.,1.,1.,1.,1.,1.,
1.,1.,1.,1.,1.,1.,1.,1.,1.,1.))
REPRESENTATION_ITEM('')
);
#702=(
BOUNDED_CURVE()
B_SPLINE_CURVE(5,(#50151,#50152,#50153,#50154,#50155,#50156,#50157,#50158,
#50159,#50160,#50161,#50162,#50163,#50164,#50165,#50166,#50167,#50168,#50169,
#50170,#50171,#50172,#50173,#50174,#50175,#50176,#50177,#50178,#50179),
 .UNSPECIFIED.,.F.,.F.)
B_SPLINE_CURVE_WITH_KNOTS((6,1,1,1,1,1,1,1,1,1,1,1,1,1,1,1,1,1,1,1,1,1,
1,1,6),(-0.670627588953112,-0.657142857142857,-0.628571428571429,-0.6,-0.571428571428572,
-0.542857142857143,-0.514285714285714,-0.485714285714286,-0.457142857142857,
-0.428571428571429,-0.4,-0.371428571428571,-0.342857142857143,-0.314285714285714,
-0.285714285714286,-0.257142857142857,-0.228571428571429,-0.2,-0.171428571428571,
-0.142857142857143,-0.114285714285714,-0.0857142857142857,-0.0571428571428571,
-0.0285714285714286,0.),.UNSPECIFIED.)
CURVE()
GEOMETRIC_REPRESENTATION_ITEM()
RATIONAL_B_SPLINE_CURVE((1.,1.,1.,1.,1.,1.,1.,1.,1.,1.,1.,1.,1.,1.,1.,1.,
1.,1.,1.,1.,1.,1.,1.,1.,1.,1.,1.,1.,1.))
REPRESENTATION_ITEM('')
);
#703=(
BOUNDED_CURVE()
B_SPLINE_CURVE(5,(#50183,#50184,#50185,#50186,#50187,#50188,#50189,#50190,
#50191,#50192,#50193,#50194,#50195,#50196,#50197,#50198,#50199,#50200,#50201,
#50202,#50203,#50204,#50205,#50206,#50207,#50208),.UNSPECIFIED.,.F.,.F.)
B_SPLINE_CURVE_WITH_KNOTS((6,1,1,1,1,1,1,1,1,1,1,1,1,1,1,1,1,1,1,1,1,6),
(-1.,-0.971428571428572,-0.942857142857143,-0.914285714285714,-0.885714285714286,
-0.857142857142857,-0.828571428571429,-0.8,-0.771428571428572,-0.742857142857143,
-0.714285714285714,-0.685714285714286,-0.657142857142857,-0.628571428571429,
-0.6,-0.571428571428572,-0.542857142857143,-0.514285714285714,-0.485714285714286,
-0.457142857142857,-0.428571428571429,-0.428061295609925),.UNSPECIFIED.)
CURVE()
GEOMETRIC_REPRESENTATION_ITEM()
RATIONAL_B_SPLINE_CURVE((1.,1.,1.,1.,1.,1.,1.,1.,1.,1.,1.,1.,1.,1.,1.,1.,
1.,1.,1.,1.,1.,1.,1.,1.,1.,1.))
REPRESENTATION_ITEM('')
);
#704=(
BOUNDED_CURVE()
B_SPLINE_CURVE(5,(#50212,#50213,#50214,#50215,#50216,#50217,#50218,#50219,
#50220,#50221,#50222,#50223,#50224,#50225,#50226,#50227,#50228,#50229,#50230,
#50231,#50232,#50233,#50234,#50235,#50236,#50237,#50238,#50239,#50240),
 .UNSPECIFIED.,.F.,.F.)
B_SPLINE_CURVE_WITH_KNOTS((6,1,1,1,1,1,1,1,1,1,1,1,1,1,1,1,1,1,1,1,1,1,
1,1,6),(-0.670627588953112,-0.657142857142857,-0.628571428571429,-0.6,-0.571428571428572,
-0.542857142857143,-0.514285714285714,-0.485714285714286,-0.457142857142857,
-0.428571428571429,-0.4,-0.371428571428571,-0.342857142857143,-0.314285714285714,
-0.285714285714286,-0.257142857142857,-0.228571428571429,-0.2,-0.171428571428571,
-0.142857142857143,-0.114285714285714,-0.0857142857142857,-0.0571428571428571,
-0.0285714285714286,0.),.UNSPECIFIED.)
CURVE()
GEOMETRIC_REPRESENTATION_ITEM()
RATIONAL_B_SPLINE_CURVE((1.,1.,1.,1.,1.,1.,1.,1.,1.,1.,1.,1.,1.,1.,1.,1.,
1.,1.,1.,1.,1.,1.,1.,1.,1.,1.,1.,1.,1.))
REPRESENTATION_ITEM('')
);
#705=(
BOUNDED_CURVE()
B_SPLINE_CURVE(5,(#50244,#50245,#50246,#50247,#50248,#50249,#50250,#50251,
#50252,#50253,#50254,#50255,#50256,#50257,#50258,#50259,#50260,#50261,#50262,
#50263,#50264,#50265,#50266,#50267,#50268,#50269),.UNSPECIFIED.,.F.,.F.)
B_SPLINE_CURVE_WITH_KNOTS((6,1,1,1,1,1,1,1,1,1,1,1,1,1,1,1,1,1,1,1,1,6),
(-1.,-0.971428571428572,-0.942857142857143,-0.914285714285714,-0.885714285714286,
-0.857142857142857,-0.828571428571429,-0.8,-0.771428571428572,-0.742857142857143,
-0.714285714285714,-0.685714285714286,-0.657142857142857,-0.628571428571429,
-0.6,-0.571428571428572,-0.542857142857143,-0.514285714285714,-0.485714285714286,
-0.457142857142857,-0.428571428571429,-0.428061295609925),.UNSPECIFIED.)
CURVE()
GEOMETRIC_REPRESENTATION_ITEM()
RATIONAL_B_SPLINE_CURVE((1.,1.,1.,1.,1.,1.,1.,1.,1.,1.,1.,1.,1.,1.,1.,1.,
1.,1.,1.,1.,1.,1.,1.,1.,1.,1.))
REPRESENTATION_ITEM('')
);
#706=(
BOUNDED_CURVE()
B_SPLINE_CURVE(5,(#50273,#50274,#50275,#50276,#50277,#50278,#50279,#50280,
#50281,#50282,#50283,#50284,#50285,#50286,#50287,#50288,#50289,#50290,#50291,
#50292,#50293,#50294,#50295,#50296,#50297,#50298,#50299,#50300,#50301),
 .UNSPECIFIED.,.F.,.F.)
B_SPLINE_CURVE_WITH_KNOTS((6,1,1,1,1,1,1,1,1,1,1,1,1,1,1,1,1,1,1,1,1,1,
1,1,6),(-0.670627588953113,-0.657142857142857,-0.628571428571429,-0.6,-0.571428571428572,
-0.542857142857143,-0.514285714285714,-0.485714285714286,-0.457142857142857,
-0.428571428571429,-0.4,-0.371428571428571,-0.342857142857143,-0.314285714285714,
-0.285714285714286,-0.257142857142857,-0.228571428571429,-0.2,-0.171428571428571,
-0.142857142857143,-0.114285714285714,-0.0857142857142857,-0.0571428571428571,
-0.0285714285714286,0.),.UNSPECIFIED.)
CURVE()
GEOMETRIC_REPRESENTATION_ITEM()
RATIONAL_B_SPLINE_CURVE((1.,1.,1.,1.,1.,1.,1.,1.,1.,1.,1.,1.,1.,1.,1.,1.,
1.,1.,1.,1.,1.,1.,1.,1.,1.,1.,1.,1.,1.))
REPRESENTATION_ITEM('')
);
#707=(
BOUNDED_CURVE()
B_SPLINE_CURVE(5,(#50305,#50306,#50307,#50308,#50309,#50310,#50311,#50312,
#50313,#50314,#50315,#50316,#50317,#50318,#50319,#50320,#50321,#50322,#50323,
#50324,#50325,#50326,#50327,#50328,#50329,#50330),.UNSPECIFIED.,.F.,.F.)
B_SPLINE_CURVE_WITH_KNOTS((6,1,1,1,1,1,1,1,1,1,1,1,1,1,1,1,1,1,1,1,1,6),
(-1.,-0.971428571428572,-0.942857142857143,-0.914285714285714,-0.885714285714286,
-0.857142857142857,-0.828571428571429,-0.8,-0.771428571428572,-0.742857142857143,
-0.714285714285714,-0.685714285714286,-0.657142857142857,-0.628571428571429,
-0.6,-0.571428571428572,-0.542857142857143,-0.514285714285714,-0.485714285714286,
-0.457142857142857,-0.428571428571429,-0.428061295609926),.UNSPECIFIED.)
CURVE()
GEOMETRIC_REPRESENTATION_ITEM()
RATIONAL_B_SPLINE_CURVE((1.,1.,1.,1.,1.,1.,1.,1.,1.,1.,1.,1.,1.,1.,1.,1.,
1.,1.,1.,1.,1.,1.,1.,1.,1.,1.))
REPRESENTATION_ITEM('')
);
#708=(
BOUNDED_CURVE()
B_SPLINE_CURVE(5,(#50334,#50335,#50336,#50337,#50338,#50339,#50340,#50341,
#50342,#50343,#50344,#50345,#50346,#50347,#50348,#50349,#50350,#50351,#50352,
#50353,#50354,#50355,#50356,#50357,#50358,#50359,#50360,#50361,#50362),
 .UNSPECIFIED.,.F.,.F.)
B_SPLINE_CURVE_WITH_KNOTS((6,1,1,1,1,1,1,1,1,1,1,1,1,1,1,1,1,1,1,1,1,1,
1,1,6),(-0.670627588953112,-0.657142857142857,-0.628571428571429,-0.6,-0.571428571428572,
-0.542857142857143,-0.514285714285714,-0.485714285714286,-0.457142857142857,
-0.428571428571429,-0.4,-0.371428571428571,-0.342857142857143,-0.314285714285714,
-0.285714285714286,-0.257142857142857,-0.228571428571429,-0.2,-0.171428571428571,
-0.142857142857143,-0.114285714285714,-0.0857142857142857,-0.0571428571428571,
-0.0285714285714286,0.),.UNSPECIFIED.)
CURVE()
GEOMETRIC_REPRESENTATION_ITEM()
RATIONAL_B_SPLINE_CURVE((1.,1.,1.,1.,1.,1.,1.,1.,1.,1.,1.,1.,1.,1.,1.,1.,
1.,1.,1.,1.,1.,1.,1.,1.,1.,1.,1.,1.,1.))
REPRESENTATION_ITEM('')
);
#709=(
BOUNDED_CURVE()
B_SPLINE_CURVE(5,(#50366,#50367,#50368,#50369,#50370,#50371,#50372,#50373,
#50374,#50375,#50376,#50377,#50378,#50379,#50380,#50381,#50382,#50383,#50384,
#50385,#50386,#50387,#50388,#50389,#50390,#50391),.UNSPECIFIED.,.F.,.F.)
B_SPLINE_CURVE_WITH_KNOTS((6,1,1,1,1,1,1,1,1,1,1,1,1,1,1,1,1,1,1,1,1,6),
(-1.,-0.971428571428572,-0.942857142857143,-0.914285714285714,-0.885714285714286,
-0.857142857142857,-0.828571428571429,-0.8,-0.771428571428572,-0.742857142857143,
-0.714285714285714,-0.685714285714286,-0.657142857142857,-0.628571428571429,
-0.6,-0.571428571428572,-0.542857142857143,-0.514285714285714,-0.485714285714286,
-0.457142857142857,-0.428571428571429,-0.428061295609926),.UNSPECIFIED.)
CURVE()
GEOMETRIC_REPRESENTATION_ITEM()
RATIONAL_B_SPLINE_CURVE((1.,1.,1.,1.,1.,1.,1.,1.,1.,1.,1.,1.,1.,1.,1.,1.,
1.,1.,1.,1.,1.,1.,1.,1.,1.,1.))
REPRESENTATION_ITEM('')
);
#710=(
BOUNDED_CURVE()
B_SPLINE_CURVE(5,(#50395,#50396,#50397,#50398,#50399,#50400,#50401,#50402,
#50403,#50404,#50405,#50406,#50407,#50408,#50409,#50410,#50411,#50412,#50413,
#50414,#50415,#50416,#50417,#50418,#50419,#50420,#50421,#50422,#50423),
 .UNSPECIFIED.,.F.,.F.)
B_SPLINE_CURVE_WITH_KNOTS((6,1,1,1,1,1,1,1,1,1,1,1,1,1,1,1,1,1,1,1,1,1,
1,1,6),(-0.670627588953113,-0.657142857142857,-0.628571428571429,-0.6,-0.571428571428572,
-0.542857142857143,-0.514285714285714,-0.485714285714286,-0.457142857142857,
-0.428571428571429,-0.4,-0.371428571428571,-0.342857142857143,-0.314285714285714,
-0.285714285714286,-0.257142857142857,-0.228571428571429,-0.2,-0.171428571428571,
-0.142857142857143,-0.114285714285714,-0.0857142857142857,-0.0571428571428571,
-0.0285714285714286,0.),.UNSPECIFIED.)
CURVE()
GEOMETRIC_REPRESENTATION_ITEM()
RATIONAL_B_SPLINE_CURVE((1.,1.,1.,1.,1.,1.,1.,1.,1.,1.,1.,1.,1.,1.,1.,1.,
1.,1.,1.,1.,1.,1.,1.,1.,1.,1.,1.,1.,1.))
REPRESENTATION_ITEM('')
);
#711=(
BOUNDED_CURVE()
B_SPLINE_CURVE(5,(#50427,#50428,#50429,#50430,#50431,#50432,#50433,#50434,
#50435,#50436,#50437,#50438,#50439,#50440,#50441,#50442,#50443,#50444,#50445,
#50446,#50447,#50448,#50449,#50450,#50451,#50452),.UNSPECIFIED.,.F.,.F.)
B_SPLINE_CURVE_WITH_KNOTS((6,1,1,1,1,1,1,1,1,1,1,1,1,1,1,1,1,1,1,1,1,6),
(-1.,-0.971428571428572,-0.942857142857143,-0.914285714285714,-0.885714285714286,
-0.857142857142857,-0.828571428571429,-0.8,-0.771428571428572,-0.742857142857143,
-0.714285714285714,-0.685714285714286,-0.657142857142857,-0.628571428571429,
-0.6,-0.571428571428572,-0.542857142857143,-0.514285714285714,-0.485714285714286,
-0.457142857142857,-0.428571428571429,-0.428061295609926),.UNSPECIFIED.)
CURVE()
GEOMETRIC_REPRESENTATION_ITEM()
RATIONAL_B_SPLINE_CURVE((1.,1.,1.,1.,1.,1.,1.,1.,1.,1.,1.,1.,1.,1.,1.,1.,
1.,1.,1.,1.,1.,1.,1.,1.,1.,1.))
REPRESENTATION_ITEM('')
);
#712=(
BOUNDED_CURVE()
B_SPLINE_CURVE(5,(#50456,#50457,#50458,#50459,#50460,#50461,#50462,#50463,
#50464,#50465,#50466,#50467,#50468,#50469,#50470,#50471,#50472,#50473,#50474,
#50475,#50476,#50477,#50478,#50479,#50480,#50481,#50482,#50483,#50484),
 .UNSPECIFIED.,.F.,.F.)
B_SPLINE_CURVE_WITH_KNOTS((6,1,1,1,1,1,1,1,1,1,1,1,1,1,1,1,1,1,1,1,1,1,
1,1,6),(-0.670627588953112,-0.657142857142857,-0.628571428571429,-0.6,-0.571428571428572,
-0.542857142857143,-0.514285714285714,-0.485714285714286,-0.457142857142857,
-0.428571428571429,-0.4,-0.371428571428571,-0.342857142857143,-0.314285714285714,
-0.285714285714286,-0.257142857142857,-0.228571428571429,-0.2,-0.171428571428571,
-0.142857142857143,-0.114285714285714,-0.0857142857142857,-0.0571428571428571,
-0.0285714285714286,0.),.UNSPECIFIED.)
CURVE()
GEOMETRIC_REPRESENTATION_ITEM()
RATIONAL_B_SPLINE_CURVE((1.,1.,1.,1.,1.,1.,1.,1.,1.,1.,1.,1.,1.,1.,1.,1.,
1.,1.,1.,1.,1.,1.,1.,1.,1.,1.,1.,1.,1.))
REPRESENTATION_ITEM('')
);
#713=(
BOUNDED_CURVE()
B_SPLINE_CURVE(5,(#50488,#50489,#50490,#50491,#50492,#50493,#50494,#50495,
#50496,#50497,#50498,#50499,#50500,#50501,#50502,#50503,#50504,#50505,#50506,
#50507,#50508,#50509,#50510,#50511,#50512,#50513),.UNSPECIFIED.,.F.,.F.)
B_SPLINE_CURVE_WITH_KNOTS((6,1,1,1,1,1,1,1,1,1,1,1,1,1,1,1,1,1,1,1,1,6),
(-1.,-0.971428571428572,-0.942857142857143,-0.914285714285714,-0.885714285714286,
-0.857142857142857,-0.828571428571429,-0.8,-0.771428571428572,-0.742857142857143,
-0.714285714285714,-0.685714285714286,-0.657142857142857,-0.628571428571429,
-0.6,-0.571428571428572,-0.542857142857143,-0.514285714285714,-0.485714285714286,
-0.457142857142857,-0.428571428571429,-0.428061295609925),.UNSPECIFIED.)
CURVE()
GEOMETRIC_REPRESENTATION_ITEM()
RATIONAL_B_SPLINE_CURVE((1.,1.,1.,1.,1.,1.,1.,1.,1.,1.,1.,1.,1.,1.,1.,1.,
1.,1.,1.,1.,1.,1.,1.,1.,1.,1.))
REPRESENTATION_ITEM('')
);
#714=(
BOUNDED_CURVE()
B_SPLINE_CURVE(5,(#50517,#50518,#50519,#50520,#50521,#50522,#50523,#50524,
#50525,#50526,#50527,#50528,#50529,#50530,#50531,#50532,#50533,#50534,#50535,
#50536,#50537,#50538,#50539,#50540,#50541,#50542,#50543,#50544,#50545),
 .UNSPECIFIED.,.F.,.F.)
B_SPLINE_CURVE_WITH_KNOTS((6,1,1,1,1,1,1,1,1,1,1,1,1,1,1,1,1,1,1,1,1,1,
1,1,6),(-0.670627588953113,-0.657142857142857,-0.628571428571429,-0.6,-0.571428571428572,
-0.542857142857143,-0.514285714285714,-0.485714285714286,-0.457142857142857,
-0.428571428571429,-0.4,-0.371428571428571,-0.342857142857143,-0.314285714285714,
-0.285714285714286,-0.257142857142857,-0.228571428571429,-0.2,-0.171428571428571,
-0.142857142857143,-0.114285714285714,-0.0857142857142857,-0.0571428571428571,
-0.0285714285714286,0.),.UNSPECIFIED.)
CURVE()
GEOMETRIC_REPRESENTATION_ITEM()
RATIONAL_B_SPLINE_CURVE((1.,1.,1.,1.,1.,1.,1.,1.,1.,1.,1.,1.,1.,1.,1.,1.,
1.,1.,1.,1.,1.,1.,1.,1.,1.,1.,1.,1.,1.))
REPRESENTATION_ITEM('')
);
#715=(
BOUNDED_CURVE()
B_SPLINE_CURVE(5,(#50549,#50550,#50551,#50552,#50553,#50554,#50555,#50556,
#50557,#50558,#50559,#50560,#50561,#50562,#50563,#50564,#50565,#50566,#50567,
#50568,#50569,#50570,#50571,#50572,#50573,#50574),.UNSPECIFIED.,.F.,.F.)
B_SPLINE_CURVE_WITH_KNOTS((6,1,1,1,1,1,1,1,1,1,1,1,1,1,1,1,1,1,1,1,1,6),
(-1.,-0.971428571428572,-0.942857142857143,-0.914285714285714,-0.885714285714286,
-0.857142857142857,-0.828571428571429,-0.8,-0.771428571428572,-0.742857142857143,
-0.714285714285714,-0.685714285714286,-0.657142857142857,-0.628571428571429,
-0.6,-0.571428571428572,-0.542857142857143,-0.514285714285714,-0.485714285714286,
-0.457142857142857,-0.428571428571429,-0.428061295609925),.UNSPECIFIED.)
CURVE()
GEOMETRIC_REPRESENTATION_ITEM()
RATIONAL_B_SPLINE_CURVE((1.,1.,1.,1.,1.,1.,1.,1.,1.,1.,1.,1.,1.,1.,1.,1.,
1.,1.,1.,1.,1.,1.,1.,1.,1.,1.))
REPRESENTATION_ITEM('')
);
#716=(
BOUNDED_CURVE()
B_SPLINE_CURVE(5,(#50578,#50579,#50580,#50581,#50582,#50583,#50584,#50585,
#50586,#50587,#50588,#50589,#50590,#50591,#50592,#50593,#50594,#50595,#50596,
#50597,#50598,#50599,#50600,#50601,#50602,#50603,#50604,#50605,#50606),
 .UNSPECIFIED.,.F.,.F.)
B_SPLINE_CURVE_WITH_KNOTS((6,1,1,1,1,1,1,1,1,1,1,1,1,1,1,1,1,1,1,1,1,1,
1,1,6),(-0.670627588953113,-0.657142857142857,-0.628571428571429,-0.6,-0.571428571428572,
-0.542857142857143,-0.514285714285714,-0.485714285714286,-0.457142857142857,
-0.428571428571429,-0.4,-0.371428571428571,-0.342857142857143,-0.314285714285714,
-0.285714285714286,-0.257142857142857,-0.228571428571429,-0.2,-0.171428571428571,
-0.142857142857143,-0.114285714285714,-0.0857142857142857,-0.0571428571428571,
-0.0285714285714286,0.),.UNSPECIFIED.)
CURVE()
GEOMETRIC_REPRESENTATION_ITEM()
RATIONAL_B_SPLINE_CURVE((1.,1.,1.,1.,1.,1.,1.,1.,1.,1.,1.,1.,1.,1.,1.,1.,
1.,1.,1.,1.,1.,1.,1.,1.,1.,1.,1.,1.,1.))
REPRESENTATION_ITEM('')
);
#717=(
BOUNDED_CURVE()
B_SPLINE_CURVE(5,(#50610,#50611,#50612,#50613,#50614,#50615,#50616,#50617,
#50618,#50619,#50620,#50621,#50622,#50623,#50624,#50625,#50626,#50627,#50628,
#50629,#50630,#50631,#50632,#50633,#50634,#50635),.UNSPECIFIED.,.F.,.F.)
B_SPLINE_CURVE_WITH_KNOTS((6,1,1,1,1,1,1,1,1,1,1,1,1,1,1,1,1,1,1,1,1,6),
(-1.,-0.971428571428572,-0.942857142857143,-0.914285714285714,-0.885714285714286,
-0.857142857142857,-0.828571428571429,-0.8,-0.771428571428572,-0.742857142857143,
-0.714285714285714,-0.685714285714286,-0.657142857142857,-0.628571428571429,
-0.6,-0.571428571428572,-0.542857142857143,-0.514285714285714,-0.485714285714286,
-0.457142857142857,-0.428571428571429,-0.428061295609926),.UNSPECIFIED.)
CURVE()
GEOMETRIC_REPRESENTATION_ITEM()
RATIONAL_B_SPLINE_CURVE((1.,1.,1.,1.,1.,1.,1.,1.,1.,1.,1.,1.,1.,1.,1.,1.,
1.,1.,1.,1.,1.,1.,1.,1.,1.,1.))
REPRESENTATION_ITEM('')
);
#718=(
BOUNDED_CURVE()
B_SPLINE_CURVE(5,(#50639,#50640,#50641,#50642,#50643,#50644,#50645,#50646,
#50647,#50648,#50649,#50650,#50651,#50652,#50653,#50654,#50655,#50656,#50657,
#50658,#50659,#50660,#50661,#50662,#50663,#50664,#50665,#50666,#50667),
 .UNSPECIFIED.,.F.,.F.)
B_SPLINE_CURVE_WITH_KNOTS((6,1,1,1,1,1,1,1,1,1,1,1,1,1,1,1,1,1,1,1,1,1,
1,1,6),(-0.670627588953112,-0.657142857142857,-0.628571428571429,-0.6,-0.571428571428572,
-0.542857142857143,-0.514285714285714,-0.485714285714286,-0.457142857142857,
-0.428571428571429,-0.4,-0.371428571428571,-0.342857142857143,-0.314285714285714,
-0.285714285714286,-0.257142857142857,-0.228571428571429,-0.2,-0.171428571428571,
-0.142857142857143,-0.114285714285714,-0.0857142857142857,-0.0571428571428571,
-0.0285714285714286,0.),.UNSPECIFIED.)
CURVE()
GEOMETRIC_REPRESENTATION_ITEM()
RATIONAL_B_SPLINE_CURVE((1.,1.,1.,1.,1.,1.,1.,1.,1.,1.,1.,1.,1.,1.,1.,1.,
1.,1.,1.,1.,1.,1.,1.,1.,1.,1.,1.,1.,1.))
REPRESENTATION_ITEM('')
);
#719=(
BOUNDED_CURVE()
B_SPLINE_CURVE(5,(#50671,#50672,#50673,#50674,#50675,#50676,#50677,#50678,
#50679,#50680,#50681,#50682,#50683,#50684,#50685,#50686,#50687,#50688,#50689,
#50690,#50691,#50692,#50693,#50694,#50695,#50696),.UNSPECIFIED.,.F.,.F.)
B_SPLINE_CURVE_WITH_KNOTS((6,1,1,1,1,1,1,1,1,1,1,1,1,1,1,1,1,1,1,1,1,6),
(-1.,-0.971428571428572,-0.942857142857143,-0.914285714285714,-0.885714285714286,
-0.857142857142857,-0.828571428571429,-0.8,-0.771428571428572,-0.742857142857143,
-0.714285714285714,-0.685714285714286,-0.657142857142857,-0.628571428571429,
-0.6,-0.571428571428572,-0.542857142857143,-0.514285714285714,-0.485714285714286,
-0.457142857142857,-0.428571428571429,-0.428061295609926),.UNSPECIFIED.)
CURVE()
GEOMETRIC_REPRESENTATION_ITEM()
RATIONAL_B_SPLINE_CURVE((1.,1.,1.,1.,1.,1.,1.,1.,1.,1.,1.,1.,1.,1.,1.,1.,
1.,1.,1.,1.,1.,1.,1.,1.,1.,1.))
REPRESENTATION_ITEM('')
);
#720=(
BOUNDED_CURVE()
B_SPLINE_CURVE(5,(#50700,#50701,#50702,#50703,#50704,#50705,#50706,#50707,
#50708,#50709,#50710,#50711,#50712,#50713,#50714,#50715,#50716,#50717,#50718,
#50719,#50720,#50721,#50722,#50723,#50724,#50725,#50726,#50727,#50728),
 .UNSPECIFIED.,.F.,.F.)
B_SPLINE_CURVE_WITH_KNOTS((6,1,1,1,1,1,1,1,1,1,1,1,1,1,1,1,1,1,1,1,1,1,
1,1,6),(-0.670627588953112,-0.657142857142857,-0.628571428571429,-0.6,-0.571428571428572,
-0.542857142857143,-0.514285714285714,-0.485714285714286,-0.457142857142857,
-0.428571428571429,-0.4,-0.371428571428571,-0.342857142857143,-0.314285714285714,
-0.285714285714286,-0.257142857142857,-0.228571428571429,-0.2,-0.171428571428571,
-0.142857142857143,-0.114285714285714,-0.0857142857142857,-0.0571428571428571,
-0.0285714285714286,0.),.UNSPECIFIED.)
CURVE()
GEOMETRIC_REPRESENTATION_ITEM()
RATIONAL_B_SPLINE_CURVE((1.,1.,1.,1.,1.,1.,1.,1.,1.,1.,1.,1.,1.,1.,1.,1.,
1.,1.,1.,1.,1.,1.,1.,1.,1.,1.,1.,1.,1.))
REPRESENTATION_ITEM('')
);
#721=(
BOUNDED_CURVE()
B_SPLINE_CURVE(5,(#50732,#50733,#50734,#50735,#50736,#50737,#50738,#50739,
#50740,#50741,#50742,#50743,#50744,#50745,#50746,#50747,#50748,#50749,#50750,
#50751,#50752,#50753,#50754,#50755,#50756,#50757),.UNSPECIFIED.,.F.,.F.)
B_SPLINE_CURVE_WITH_KNOTS((6,1,1,1,1,1,1,1,1,1,1,1,1,1,1,1,1,1,1,1,1,6),
(-1.,-0.971428571428572,-0.942857142857143,-0.914285714285714,-0.885714285714286,
-0.857142857142857,-0.828571428571429,-0.8,-0.771428571428572,-0.742857142857143,
-0.714285714285714,-0.685714285714286,-0.657142857142857,-0.628571428571429,
-0.6,-0.571428571428572,-0.542857142857143,-0.514285714285714,-0.485714285714286,
-0.457142857142857,-0.428571428571429,-0.428061295609926),.UNSPECIFIED.)
CURVE()
GEOMETRIC_REPRESENTATION_ITEM()
RATIONAL_B_SPLINE_CURVE((1.,1.,1.,1.,1.,1.,1.,1.,1.,1.,1.,1.,1.,1.,1.,1.,
1.,1.,1.,1.,1.,1.,1.,1.,1.,1.))
REPRESENTATION_ITEM('')
);
#722=(
BOUNDED_CURVE()
B_SPLINE_CURVE(5,(#50761,#50762,#50763,#50764,#50765,#50766,#50767,#50768,
#50769,#50770,#50771,#50772,#50773,#50774,#50775,#50776,#50777,#50778,#50779,
#50780,#50781,#50782,#50783,#50784,#50785,#50786,#50787,#50788,#50789),
 .UNSPECIFIED.,.F.,.F.)
B_SPLINE_CURVE_WITH_KNOTS((6,1,1,1,1,1,1,1,1,1,1,1,1,1,1,1,1,1,1,1,1,1,
1,1,6),(-0.670627588953112,-0.657142857142857,-0.628571428571429,-0.6,-0.571428571428572,
-0.542857142857143,-0.514285714285714,-0.485714285714286,-0.457142857142857,
-0.428571428571429,-0.4,-0.371428571428571,-0.342857142857143,-0.314285714285714,
-0.285714285714286,-0.257142857142857,-0.228571428571429,-0.2,-0.171428571428571,
-0.142857142857143,-0.114285714285714,-0.0857142857142857,-0.0571428571428571,
-0.0285714285714286,0.),.UNSPECIFIED.)
CURVE()
GEOMETRIC_REPRESENTATION_ITEM()
RATIONAL_B_SPLINE_CURVE((1.,1.,1.,1.,1.,1.,1.,1.,1.,1.,1.,1.,1.,1.,1.,1.,
1.,1.,1.,1.,1.,1.,1.,1.,1.,1.,1.,1.,1.))
REPRESENTATION_ITEM('')
);
#723=(
BOUNDED_CURVE()
B_SPLINE_CURVE(5,(#50793,#50794,#50795,#50796,#50797,#50798,#50799,#50800,
#50801,#50802,#50803,#50804,#50805,#50806,#50807,#50808,#50809,#50810,#50811,
#50812,#50813,#50814,#50815,#50816,#50817,#50818),.UNSPECIFIED.,.F.,.F.)
B_SPLINE_CURVE_WITH_KNOTS((6,1,1,1,1,1,1,1,1,1,1,1,1,1,1,1,1,1,1,1,1,6),
(-1.,-0.971428571428572,-0.942857142857143,-0.914285714285714,-0.885714285714286,
-0.857142857142857,-0.828571428571429,-0.8,-0.771428571428572,-0.742857142857143,
-0.714285714285714,-0.685714285714286,-0.657142857142857,-0.628571428571429,
-0.6,-0.571428571428572,-0.542857142857143,-0.514285714285714,-0.485714285714286,
-0.457142857142857,-0.428571428571429,-0.428061295609926),.UNSPECIFIED.)
CURVE()
GEOMETRIC_REPRESENTATION_ITEM()
RATIONAL_B_SPLINE_CURVE((1.,1.,1.,1.,1.,1.,1.,1.,1.,1.,1.,1.,1.,1.,1.,1.,
1.,1.,1.,1.,1.,1.,1.,1.,1.,1.))
REPRESENTATION_ITEM('')
);
#724=(
BOUNDED_CURVE()
B_SPLINE_CURVE(5,(#50822,#50823,#50824,#50825,#50826,#50827,#50828,#50829,
#50830,#50831,#50832,#50833,#50834,#50835,#50836,#50837,#50838,#50839,#50840,
#50841,#50842,#50843,#50844,#50845,#50846,#50847,#50848,#50849,#50850),
 .UNSPECIFIED.,.F.,.F.)
B_SPLINE_CURVE_WITH_KNOTS((6,1,1,1,1,1,1,1,1,1,1,1,1,1,1,1,1,1,1,1,1,1,
1,1,6),(-0.670627588953112,-0.657142857142857,-0.628571428571429,-0.6,-0.571428571428572,
-0.542857142857143,-0.514285714285714,-0.485714285714286,-0.457142857142857,
-0.428571428571429,-0.4,-0.371428571428571,-0.342857142857143,-0.314285714285714,
-0.285714285714286,-0.257142857142857,-0.228571428571429,-0.2,-0.171428571428571,
-0.142857142857143,-0.114285714285714,-0.0857142857142857,-0.0571428571428571,
-0.0285714285714286,0.),.UNSPECIFIED.)
CURVE()
GEOMETRIC_REPRESENTATION_ITEM()
RATIONAL_B_SPLINE_CURVE((1.,1.,1.,1.,1.,1.,1.,1.,1.,1.,1.,1.,1.,1.,1.,1.,
1.,1.,1.,1.,1.,1.,1.,1.,1.,1.,1.,1.,1.))
REPRESENTATION_ITEM('')
);
#725=(
BOUNDED_CURVE()
B_SPLINE_CURVE(5,(#50854,#50855,#50856,#50857,#50858,#50859,#50860,#50861,
#50862,#50863,#50864,#50865,#50866,#50867,#50868,#50869,#50870,#50871,#50872,
#50873,#50874,#50875,#50876,#50877,#50878,#50879),.UNSPECIFIED.,.F.,.F.)
B_SPLINE_CURVE_WITH_KNOTS((6,1,1,1,1,1,1,1,1,1,1,1,1,1,1,1,1,1,1,1,1,6),
(-1.,-0.971428571428572,-0.942857142857143,-0.914285714285714,-0.885714285714286,
-0.857142857142857,-0.828571428571429,-0.8,-0.771428571428572,-0.742857142857143,
-0.714285714285714,-0.685714285714286,-0.657142857142857,-0.628571428571429,
-0.6,-0.571428571428572,-0.542857142857143,-0.514285714285714,-0.485714285714286,
-0.457142857142857,-0.428571428571429,-0.428061295609926),.UNSPECIFIED.)
CURVE()
GEOMETRIC_REPRESENTATION_ITEM()
RATIONAL_B_SPLINE_CURVE((1.,1.,1.,1.,1.,1.,1.,1.,1.,1.,1.,1.,1.,1.,1.,1.,
1.,1.,1.,1.,1.,1.,1.,1.,1.,1.))
REPRESENTATION_ITEM('')
);
#726=(
BOUNDED_CURVE()
B_SPLINE_CURVE(5,(#50883,#50884,#50885,#50886,#50887,#50888,#50889,#50890,
#50891,#50892,#50893,#50894,#50895,#50896,#50897,#50898,#50899,#50900,#50901,
#50902,#50903,#50904,#50905,#50906,#50907,#50908,#50909,#50910,#50911),
 .UNSPECIFIED.,.F.,.F.)
B_SPLINE_CURVE_WITH_KNOTS((6,1,1,1,1,1,1,1,1,1,1,1,1,1,1,1,1,1,1,1,1,1,
1,1,6),(-0.670627588953112,-0.657142857142857,-0.628571428571429,-0.6,-0.571428571428572,
-0.542857142857143,-0.514285714285714,-0.485714285714286,-0.457142857142857,
-0.428571428571429,-0.4,-0.371428571428571,-0.342857142857143,-0.314285714285714,
-0.285714285714286,-0.257142857142857,-0.228571428571429,-0.2,-0.171428571428571,
-0.142857142857143,-0.114285714285714,-0.0857142857142857,-0.0571428571428571,
-0.0285714285714286,0.),.UNSPECIFIED.)
CURVE()
GEOMETRIC_REPRESENTATION_ITEM()
RATIONAL_B_SPLINE_CURVE((1.,1.,1.,1.,1.,1.,1.,1.,1.,1.,1.,1.,1.,1.,1.,1.,
1.,1.,1.,1.,1.,1.,1.,1.,1.,1.,1.,1.,1.))
REPRESENTATION_ITEM('')
);
#727=(
BOUNDED_CURVE()
B_SPLINE_CURVE(5,(#50915,#50916,#50917,#50918,#50919,#50920,#50921,#50922,
#50923,#50924,#50925,#50926,#50927,#50928,#50929,#50930,#50931,#50932,#50933,
#50934,#50935,#50936,#50937,#50938,#50939,#50940),.UNSPECIFIED.,.F.,.F.)
B_SPLINE_CURVE_WITH_KNOTS((6,1,1,1,1,1,1,1,1,1,1,1,1,1,1,1,1,1,1,1,1,6),
(-1.,-0.971428571428572,-0.942857142857143,-0.914285714285714,-0.885714285714286,
-0.857142857142857,-0.828571428571429,-0.8,-0.771428571428572,-0.742857142857143,
-0.714285714285714,-0.685714285714286,-0.657142857142857,-0.628571428571429,
-0.6,-0.571428571428572,-0.542857142857143,-0.514285714285714,-0.485714285714286,
-0.457142857142857,-0.428571428571429,-0.428061295609925),.UNSPECIFIED.)
CURVE()
GEOMETRIC_REPRESENTATION_ITEM()
RATIONAL_B_SPLINE_CURVE((1.,1.,1.,1.,1.,1.,1.,1.,1.,1.,1.,1.,1.,1.,1.,1.,
1.,1.,1.,1.,1.,1.,1.,1.,1.,1.))
REPRESENTATION_ITEM('')
);
#728=(
BOUNDED_CURVE()
B_SPLINE_CURVE(5,(#50944,#50945,#50946,#50947,#50948,#50949,#50950,#50951,
#50952,#50953,#50954,#50955,#50956,#50957,#50958,#50959,#50960,#50961,#50962,
#50963,#50964,#50965,#50966,#50967,#50968,#50969,#50970,#50971,#50972),
 .UNSPECIFIED.,.F.,.F.)
B_SPLINE_CURVE_WITH_KNOTS((6,1,1,1,1,1,1,1,1,1,1,1,1,1,1,1,1,1,1,1,1,1,
1,1,6),(-0.670627588953112,-0.657142857142857,-0.628571428571429,-0.6,-0.571428571428572,
-0.542857142857143,-0.514285714285714,-0.485714285714286,-0.457142857142857,
-0.428571428571429,-0.4,-0.371428571428571,-0.342857142857143,-0.314285714285714,
-0.285714285714286,-0.257142857142857,-0.228571428571429,-0.2,-0.171428571428571,
-0.142857142857143,-0.114285714285714,-0.0857142857142857,-0.0571428571428571,
-0.0285714285714286,0.),.UNSPECIFIED.)
CURVE()
GEOMETRIC_REPRESENTATION_ITEM()
RATIONAL_B_SPLINE_CURVE((1.,1.,1.,1.,1.,1.,1.,1.,1.,1.,1.,1.,1.,1.,1.,1.,
1.,1.,1.,1.,1.,1.,1.,1.,1.,1.,1.,1.,1.))
REPRESENTATION_ITEM('')
);
#729=(
BOUNDED_CURVE()
B_SPLINE_CURVE(5,(#50976,#50977,#50978,#50979,#50980,#50981,#50982,#50983,
#50984,#50985,#50986,#50987,#50988,#50989,#50990,#50991,#50992,#50993,#50994,
#50995,#50996,#50997,#50998,#50999,#51000,#51001),.UNSPECIFIED.,.F.,.F.)
B_SPLINE_CURVE_WITH_KNOTS((6,1,1,1,1,1,1,1,1,1,1,1,1,1,1,1,1,1,1,1,1,6),
(-1.,-0.971428571428572,-0.942857142857143,-0.914285714285714,-0.885714285714286,
-0.857142857142857,-0.828571428571429,-0.8,-0.771428571428572,-0.742857142857143,
-0.714285714285714,-0.685714285714286,-0.657142857142857,-0.628571428571429,
-0.6,-0.571428571428572,-0.542857142857143,-0.514285714285714,-0.485714285714286,
-0.457142857142857,-0.428571428571429,-0.428061295609926),.UNSPECIFIED.)
CURVE()
GEOMETRIC_REPRESENTATION_ITEM()
RATIONAL_B_SPLINE_CURVE((1.,1.,1.,1.,1.,1.,1.,1.,1.,1.,1.,1.,1.,1.,1.,1.,
1.,1.,1.,1.,1.,1.,1.,1.,1.,1.))
REPRESENTATION_ITEM('')
);
#730=(
BOUNDED_CURVE()
B_SPLINE_CURVE(5,(#51005,#51006,#51007,#51008,#51009,#51010,#51011,#51012,
#51013,#51014,#51015,#51016,#51017,#51018,#51019,#51020,#51021,#51022,#51023,
#51024,#51025,#51026,#51027,#51028,#51029,#51030,#51031,#51032,#51033),
 .UNSPECIFIED.,.F.,.F.)
B_SPLINE_CURVE_WITH_KNOTS((6,1,1,1,1,1,1,1,1,1,1,1,1,1,1,1,1,1,1,1,1,1,
1,1,6),(-0.670627588953112,-0.657142857142857,-0.628571428571429,-0.6,-0.571428571428572,
-0.542857142857143,-0.514285714285714,-0.485714285714286,-0.457142857142857,
-0.428571428571429,-0.4,-0.371428571428571,-0.342857142857143,-0.314285714285714,
-0.285714285714286,-0.257142857142857,-0.228571428571429,-0.2,-0.171428571428571,
-0.142857142857143,-0.114285714285714,-0.0857142857142857,-0.0571428571428571,
-0.0285714285714286,0.),.UNSPECIFIED.)
CURVE()
GEOMETRIC_REPRESENTATION_ITEM()
RATIONAL_B_SPLINE_CURVE((1.,1.,1.,1.,1.,1.,1.,1.,1.,1.,1.,1.,1.,1.,1.,1.,
1.,1.,1.,1.,1.,1.,1.,1.,1.,1.,1.,1.,1.))
REPRESENTATION_ITEM('')
);
#731=(
BOUNDED_CURVE()
B_SPLINE_CURVE(5,(#51037,#51038,#51039,#51040,#51041,#51042,#51043,#51044,
#51045,#51046,#51047,#51048,#51049,#51050,#51051,#51052,#51053,#51054,#51055,
#51056,#51057,#51058,#51059,#51060,#51061,#51062),.UNSPECIFIED.,.F.,.F.)
B_SPLINE_CURVE_WITH_KNOTS((6,1,1,1,1,1,1,1,1,1,1,1,1,1,1,1,1,1,1,1,1,6),
(-1.,-0.971428571428572,-0.942857142857143,-0.914285714285714,-0.885714285714286,
-0.857142857142857,-0.828571428571429,-0.8,-0.771428571428572,-0.742857142857143,
-0.714285714285714,-0.685714285714286,-0.657142857142857,-0.628571428571429,
-0.6,-0.571428571428572,-0.542857142857143,-0.514285714285714,-0.485714285714286,
-0.457142857142857,-0.428571428571429,-0.428061295609927),.UNSPECIFIED.)
CURVE()
GEOMETRIC_REPRESENTATION_ITEM()
RATIONAL_B_SPLINE_CURVE((1.,1.,1.,1.,1.,1.,1.,1.,1.,1.,1.,1.,1.,1.,1.,1.,
1.,1.,1.,1.,1.,1.,1.,1.,1.,1.))
REPRESENTATION_ITEM('')
);
#732=(
BOUNDED_CURVE()
B_SPLINE_CURVE(5,(#51066,#51067,#51068,#51069,#51070,#51071,#51072,#51073,
#51074,#51075,#51076,#51077,#51078,#51079,#51080,#51081,#51082,#51083,#51084,
#51085,#51086,#51087,#51088,#51089,#51090,#51091,#51092,#51093,#51094),
 .UNSPECIFIED.,.F.,.F.)
B_SPLINE_CURVE_WITH_KNOTS((6,1,1,1,1,1,1,1,1,1,1,1,1,1,1,1,1,1,1,1,1,1,
1,1,6),(-0.670627588953113,-0.657142857142857,-0.628571428571429,-0.6,-0.571428571428572,
-0.542857142857143,-0.514285714285714,-0.485714285714286,-0.457142857142857,
-0.428571428571429,-0.4,-0.371428571428571,-0.342857142857143,-0.314285714285714,
-0.285714285714286,-0.257142857142857,-0.228571428571429,-0.2,-0.171428571428571,
-0.142857142857143,-0.114285714285714,-0.0857142857142857,-0.0571428571428571,
-0.0285714285714286,0.),.UNSPECIFIED.)
CURVE()
GEOMETRIC_REPRESENTATION_ITEM()
RATIONAL_B_SPLINE_CURVE((1.,1.,1.,1.,1.,1.,1.,1.,1.,1.,1.,1.,1.,1.,1.,1.,
1.,1.,1.,1.,1.,1.,1.,1.,1.,1.,1.,1.,1.))
REPRESENTATION_ITEM('')
);
#733=(
BOUNDED_CURVE()
B_SPLINE_CURVE(5,(#51098,#51099,#51100,#51101,#51102,#51103,#51104,#51105,
#51106,#51107,#51108,#51109,#51110,#51111,#51112,#51113,#51114,#51115,#51116,
#51117,#51118,#51119,#51120,#51121,#51122,#51123),.UNSPECIFIED.,.F.,.F.)
B_SPLINE_CURVE_WITH_KNOTS((6,1,1,1,1,1,1,1,1,1,1,1,1,1,1,1,1,1,1,1,1,6),
(-1.,-0.971428571428572,-0.942857142857143,-0.914285714285714,-0.885714285714286,
-0.857142857142857,-0.828571428571429,-0.8,-0.771428571428572,-0.742857142857143,
-0.714285714285714,-0.685714285714286,-0.657142857142857,-0.628571428571429,
-0.6,-0.571428571428572,-0.542857142857143,-0.514285714285714,-0.485714285714286,
-0.457142857142857,-0.428571428571429,-0.428061295609925),.UNSPECIFIED.)
CURVE()
GEOMETRIC_REPRESENTATION_ITEM()
RATIONAL_B_SPLINE_CURVE((1.,1.,1.,1.,1.,1.,1.,1.,1.,1.,1.,1.,1.,1.,1.,1.,
1.,1.,1.,1.,1.,1.,1.,1.,1.,1.))
REPRESENTATION_ITEM('')
);
#734=(
BOUNDED_CURVE()
B_SPLINE_CURVE(5,(#51127,#51128,#51129,#51130,#51131,#51132,#51133,#51134,
#51135,#51136,#51137,#51138,#51139,#51140,#51141,#51142,#51143,#51144,#51145,
#51146,#51147,#51148,#51149,#51150,#51151,#51152,#51153,#51154,#51155),
 .UNSPECIFIED.,.F.,.F.)
B_SPLINE_CURVE_WITH_KNOTS((6,1,1,1,1,1,1,1,1,1,1,1,1,1,1,1,1,1,1,1,1,1,
1,1,6),(-0.670627588953113,-0.657142857142857,-0.628571428571429,-0.6,-0.571428571428572,
-0.542857142857143,-0.514285714285714,-0.485714285714286,-0.457142857142857,
-0.428571428571429,-0.4,-0.371428571428571,-0.342857142857143,-0.314285714285714,
-0.285714285714286,-0.257142857142857,-0.228571428571429,-0.2,-0.171428571428571,
-0.142857142857143,-0.114285714285714,-0.0857142857142857,-0.0571428571428571,
-0.0285714285714286,0.),.UNSPECIFIED.)
CURVE()
GEOMETRIC_REPRESENTATION_ITEM()
RATIONAL_B_SPLINE_CURVE((1.,1.,1.,1.,1.,1.,1.,1.,1.,1.,1.,1.,1.,1.,1.,1.,
1.,1.,1.,1.,1.,1.,1.,1.,1.,1.,1.,1.,1.))
REPRESENTATION_ITEM('')
);
#735=(
BOUNDED_CURVE()
B_SPLINE_CURVE(5,(#51159,#51160,#51161,#51162,#51163,#51164,#51165,#51166,
#51167,#51168,#51169,#51170,#51171,#51172,#51173,#51174,#51175,#51176,#51177,
#51178,#51179,#51180,#51181,#51182,#51183,#51184),.UNSPECIFIED.,.F.,.F.)
B_SPLINE_CURVE_WITH_KNOTS((6,1,1,1,1,1,1,1,1,1,1,1,1,1,1,1,1,1,1,1,1,6),
(-1.,-0.971428571428572,-0.942857142857143,-0.914285714285714,-0.885714285714286,
-0.857142857142857,-0.828571428571429,-0.8,-0.771428571428572,-0.742857142857143,
-0.714285714285714,-0.685714285714286,-0.657142857142857,-0.628571428571429,
-0.6,-0.571428571428572,-0.542857142857143,-0.514285714285714,-0.485714285714286,
-0.457142857142857,-0.428571428571429,-0.428061295609926),.UNSPECIFIED.)
CURVE()
GEOMETRIC_REPRESENTATION_ITEM()
RATIONAL_B_SPLINE_CURVE((1.,1.,1.,1.,1.,1.,1.,1.,1.,1.,1.,1.,1.,1.,1.,1.,
1.,1.,1.,1.,1.,1.,1.,1.,1.,1.))
REPRESENTATION_ITEM('')
);
#736=(
BOUNDED_CURVE()
B_SPLINE_CURVE(5,(#51188,#51189,#51190,#51191,#51192,#51193,#51194,#51195,
#51196,#51197,#51198,#51199,#51200,#51201,#51202,#51203,#51204,#51205,#51206,
#51207,#51208,#51209,#51210,#51211,#51212,#51213,#51214,#51215,#51216),
 .UNSPECIFIED.,.F.,.F.)
B_SPLINE_CURVE_WITH_KNOTS((6,1,1,1,1,1,1,1,1,1,1,1,1,1,1,1,1,1,1,1,1,1,
1,1,6),(-0.670627588953112,-0.657142857142857,-0.628571428571429,-0.6,-0.571428571428572,
-0.542857142857143,-0.514285714285714,-0.485714285714286,-0.457142857142857,
-0.428571428571429,-0.4,-0.371428571428571,-0.342857142857143,-0.314285714285714,
-0.285714285714286,-0.257142857142857,-0.228571428571429,-0.2,-0.171428571428571,
-0.142857142857143,-0.114285714285714,-0.0857142857142857,-0.0571428571428571,
-0.0285714285714286,0.),.UNSPECIFIED.)
CURVE()
GEOMETRIC_REPRESENTATION_ITEM()
RATIONAL_B_SPLINE_CURVE((1.,1.,1.,1.,1.,1.,1.,1.,1.,1.,1.,1.,1.,1.,1.,1.,
1.,1.,1.,1.,1.,1.,1.,1.,1.,1.,1.,1.,1.))
REPRESENTATION_ITEM('')
);
#737=(
BOUNDED_CURVE()
B_SPLINE_CURVE(5,(#51220,#51221,#51222,#51223,#51224,#51225,#51226,#51227,
#51228,#51229,#51230,#51231,#51232,#51233,#51234,#51235,#51236,#51237,#51238,
#51239,#51240,#51241,#51242,#51243,#51244,#51245),.UNSPECIFIED.,.F.,.F.)
B_SPLINE_CURVE_WITH_KNOTS((6,1,1,1,1,1,1,1,1,1,1,1,1,1,1,1,1,1,1,1,1,6),
(-1.,-0.971428571428572,-0.942857142857143,-0.914285714285714,-0.885714285714286,
-0.857142857142857,-0.828571428571429,-0.8,-0.771428571428572,-0.742857142857143,
-0.714285714285714,-0.685714285714286,-0.657142857142857,-0.628571428571429,
-0.6,-0.571428571428572,-0.542857142857143,-0.514285714285714,-0.485714285714286,
-0.457142857142857,-0.428571428571429,-0.428061295609926),.UNSPECIFIED.)
CURVE()
GEOMETRIC_REPRESENTATION_ITEM()
RATIONAL_B_SPLINE_CURVE((1.,1.,1.,1.,1.,1.,1.,1.,1.,1.,1.,1.,1.,1.,1.,1.,
1.,1.,1.,1.,1.,1.,1.,1.,1.,1.))
REPRESENTATION_ITEM('')
);
#738=(
BOUNDED_CURVE()
B_SPLINE_CURVE(5,(#51249,#51250,#51251,#51252,#51253,#51254,#51255,#51256,
#51257,#51258,#51259,#51260,#51261,#51262,#51263,#51264,#51265,#51266,#51267,
#51268,#51269,#51270,#51271,#51272,#51273,#51274,#51275,#51276,#51277),
 .UNSPECIFIED.,.F.,.F.)
B_SPLINE_CURVE_WITH_KNOTS((6,1,1,1,1,1,1,1,1,1,1,1,1,1,1,1,1,1,1,1,1,1,
1,1,6),(-0.670627588953113,-0.657142857142857,-0.628571428571429,-0.6,-0.571428571428572,
-0.542857142857143,-0.514285714285714,-0.485714285714286,-0.457142857142857,
-0.428571428571429,-0.4,-0.371428571428571,-0.342857142857143,-0.314285714285714,
-0.285714285714286,-0.257142857142857,-0.228571428571429,-0.2,-0.171428571428571,
-0.142857142857143,-0.114285714285714,-0.0857142857142857,-0.0571428571428571,
-0.0285714285714286,0.),.UNSPECIFIED.)
CURVE()
GEOMETRIC_REPRESENTATION_ITEM()
RATIONAL_B_SPLINE_CURVE((1.,1.,1.,1.,1.,1.,1.,1.,1.,1.,1.,1.,1.,1.,1.,1.,
1.,1.,1.,1.,1.,1.,1.,1.,1.,1.,1.,1.,1.))
REPRESENTATION_ITEM('')
);
#739=(
BOUNDED_CURVE()
B_SPLINE_CURVE(5,(#51281,#51282,#51283,#51284,#51285,#51286,#51287,#51288,
#51289,#51290,#51291,#51292,#51293,#51294,#51295,#51296,#51297,#51298,#51299,
#51300,#51301,#51302,#51303,#51304,#51305,#51306),.UNSPECIFIED.,.F.,.F.)
B_SPLINE_CURVE_WITH_KNOTS((6,1,1,1,1,1,1,1,1,1,1,1,1,1,1,1,1,1,1,1,1,6),
(-1.,-0.971428571428572,-0.942857142857143,-0.914285714285714,-0.885714285714286,
-0.857142857142857,-0.828571428571429,-0.8,-0.771428571428572,-0.742857142857143,
-0.714285714285714,-0.685714285714286,-0.657142857142857,-0.628571428571429,
-0.6,-0.571428571428572,-0.542857142857143,-0.514285714285714,-0.485714285714286,
-0.457142857142857,-0.428571428571429,-0.428061295609926),.UNSPECIFIED.)
CURVE()
GEOMETRIC_REPRESENTATION_ITEM()
RATIONAL_B_SPLINE_CURVE((1.,1.,1.,1.,1.,1.,1.,1.,1.,1.,1.,1.,1.,1.,1.,1.,
1.,1.,1.,1.,1.,1.,1.,1.,1.,1.))
REPRESENTATION_ITEM('')
);
#740=(
BOUNDED_CURVE()
B_SPLINE_CURVE(5,(#51310,#51311,#51312,#51313,#51314,#51315,#51316,#51317,
#51318,#51319,#51320,#51321,#51322,#51323,#51324,#51325,#51326,#51327,#51328,
#51329,#51330,#51331,#51332,#51333,#51334,#51335,#51336,#51337,#51338),
 .UNSPECIFIED.,.F.,.F.)
B_SPLINE_CURVE_WITH_KNOTS((6,1,1,1,1,1,1,1,1,1,1,1,1,1,1,1,1,1,1,1,1,1,
1,1,6),(-0.670627588953113,-0.657142857142857,-0.628571428571429,-0.6,-0.571428571428572,
-0.542857142857143,-0.514285714285714,-0.485714285714286,-0.457142857142857,
-0.428571428571429,-0.4,-0.371428571428571,-0.342857142857143,-0.314285714285714,
-0.285714285714286,-0.257142857142857,-0.228571428571429,-0.2,-0.171428571428571,
-0.142857142857143,-0.114285714285714,-0.0857142857142857,-0.0571428571428571,
-0.0285714285714286,0.),.UNSPECIFIED.)
CURVE()
GEOMETRIC_REPRESENTATION_ITEM()
RATIONAL_B_SPLINE_CURVE((1.,1.,1.,1.,1.,1.,1.,1.,1.,1.,1.,1.,1.,1.,1.,1.,
1.,1.,1.,1.,1.,1.,1.,1.,1.,1.,1.,1.,1.))
REPRESENTATION_ITEM('')
);
#741=(
BOUNDED_CURVE()
B_SPLINE_CURVE(5,(#51342,#51343,#51344,#51345,#51346,#51347,#51348,#51349,
#51350,#51351,#51352,#51353,#51354,#51355,#51356,#51357,#51358,#51359,#51360,
#51361,#51362,#51363,#51364,#51365,#51366,#51367),.UNSPECIFIED.,.F.,.F.)
B_SPLINE_CURVE_WITH_KNOTS((6,1,1,1,1,1,1,1,1,1,1,1,1,1,1,1,1,1,1,1,1,6),
(-1.,-0.971428571428572,-0.942857142857143,-0.914285714285714,-0.885714285714286,
-0.857142857142857,-0.828571428571429,-0.8,-0.771428571428572,-0.742857142857143,
-0.714285714285714,-0.685714285714286,-0.657142857142857,-0.628571428571429,
-0.6,-0.571428571428572,-0.542857142857143,-0.514285714285714,-0.485714285714286,
-0.457142857142857,-0.428571428571429,-0.428061295609926),.UNSPECIFIED.)
CURVE()
GEOMETRIC_REPRESENTATION_ITEM()
RATIONAL_B_SPLINE_CURVE((1.,1.,1.,1.,1.,1.,1.,1.,1.,1.,1.,1.,1.,1.,1.,1.,
1.,1.,1.,1.,1.,1.,1.,1.,1.,1.))
REPRESENTATION_ITEM('')
);
#742=(
BOUNDED_CURVE()
B_SPLINE_CURVE(5,(#51371,#51372,#51373,#51374,#51375,#51376,#51377,#51378,
#51379,#51380,#51381,#51382,#51383,#51384,#51385,#51386,#51387,#51388,#51389,
#51390,#51391,#51392,#51393,#51394,#51395,#51396,#51397,#51398,#51399),
 .UNSPECIFIED.,.F.,.F.)
B_SPLINE_CURVE_WITH_KNOTS((6,1,1,1,1,1,1,1,1,1,1,1,1,1,1,1,1,1,1,1,1,1,
1,1,6),(-0.670627588953112,-0.657142857142857,-0.628571428571429,-0.6,-0.571428571428572,
-0.542857142857143,-0.514285714285714,-0.485714285714286,-0.457142857142857,
-0.428571428571429,-0.4,-0.371428571428571,-0.342857142857143,-0.314285714285714,
-0.285714285714286,-0.257142857142857,-0.228571428571429,-0.2,-0.171428571428571,
-0.142857142857143,-0.114285714285714,-0.0857142857142857,-0.0571428571428571,
-0.0285714285714286,0.),.UNSPECIFIED.)
CURVE()
GEOMETRIC_REPRESENTATION_ITEM()
RATIONAL_B_SPLINE_CURVE((1.,1.,1.,1.,1.,1.,1.,1.,1.,1.,1.,1.,1.,1.,1.,1.,
1.,1.,1.,1.,1.,1.,1.,1.,1.,1.,1.,1.,1.))
REPRESENTATION_ITEM('')
);
#743=(
BOUNDED_CURVE()
B_SPLINE_CURVE(5,(#51403,#51404,#51405,#51406,#51407,#51408,#51409,#51410,
#51411,#51412,#51413,#51414,#51415,#51416,#51417,#51418,#51419,#51420,#51421,
#51422,#51423,#51424,#51425,#51426,#51427,#51428),.UNSPECIFIED.,.F.,.F.)
B_SPLINE_CURVE_WITH_KNOTS((6,1,1,1,1,1,1,1,1,1,1,1,1,1,1,1,1,1,1,1,1,6),
(-1.,-0.971428571428572,-0.942857142857143,-0.914285714285714,-0.885714285714286,
-0.857142857142857,-0.828571428571429,-0.8,-0.771428571428572,-0.742857142857143,
-0.714285714285714,-0.685714285714286,-0.657142857142857,-0.628571428571429,
-0.6,-0.571428571428572,-0.542857142857143,-0.514285714285714,-0.485714285714286,
-0.457142857142857,-0.428571428571429,-0.428061295609926),.UNSPECIFIED.)
CURVE()
GEOMETRIC_REPRESENTATION_ITEM()
RATIONAL_B_SPLINE_CURVE((1.,1.,1.,1.,1.,1.,1.,1.,1.,1.,1.,1.,1.,1.,1.,1.,
1.,1.,1.,1.,1.,1.,1.,1.,1.,1.))
REPRESENTATION_ITEM('')
);
#744=(
BOUNDED_CURVE()
B_SPLINE_CURVE(5,(#51432,#51433,#51434,#51435,#51436,#51437,#51438,#51439,
#51440,#51441,#51442,#51443,#51444,#51445,#51446,#51447,#51448,#51449,#51450,
#51451,#51452,#51453,#51454,#51455,#51456,#51457,#51458,#51459,#51460),
 .UNSPECIFIED.,.F.,.F.)
B_SPLINE_CURVE_WITH_KNOTS((6,1,1,1,1,1,1,1,1,1,1,1,1,1,1,1,1,1,1,1,1,1,
1,1,6),(-0.670627588953113,-0.657142857142857,-0.628571428571429,-0.6,-0.571428571428572,
-0.542857142857143,-0.514285714285714,-0.485714285714286,-0.457142857142857,
-0.428571428571429,-0.4,-0.371428571428571,-0.342857142857143,-0.314285714285714,
-0.285714285714286,-0.257142857142857,-0.228571428571429,-0.2,-0.171428571428571,
-0.142857142857143,-0.114285714285714,-0.0857142857142857,-0.0571428571428571,
-0.0285714285714286,0.),.UNSPECIFIED.)
CURVE()
GEOMETRIC_REPRESENTATION_ITEM()
RATIONAL_B_SPLINE_CURVE((1.,1.,1.,1.,1.,1.,1.,1.,1.,1.,1.,1.,1.,1.,1.,1.,
1.,1.,1.,1.,1.,1.,1.,1.,1.,1.,1.,1.,1.))
REPRESENTATION_ITEM('')
);
#745=(
BOUNDED_CURVE()
B_SPLINE_CURVE(5,(#51464,#51465,#51466,#51467,#51468,#51469,#51470,#51471,
#51472,#51473,#51474,#51475,#51476,#51477,#51478,#51479,#51480,#51481,#51482,
#51483,#51484,#51485,#51486,#51487,#51488,#51489),.UNSPECIFIED.,.F.,.F.)
B_SPLINE_CURVE_WITH_KNOTS((6,1,1,1,1,1,1,1,1,1,1,1,1,1,1,1,1,1,1,1,1,6),
(-1.,-0.971428571428572,-0.942857142857143,-0.914285714285714,-0.885714285714286,
-0.857142857142857,-0.828571428571429,-0.8,-0.771428571428572,-0.742857142857143,
-0.714285714285714,-0.685714285714286,-0.657142857142857,-0.628571428571429,
-0.6,-0.571428571428572,-0.542857142857143,-0.514285714285714,-0.485714285714286,
-0.457142857142857,-0.428571428571429,-0.428061295609926),.UNSPECIFIED.)
CURVE()
GEOMETRIC_REPRESENTATION_ITEM()
RATIONAL_B_SPLINE_CURVE((1.,1.,1.,1.,1.,1.,1.,1.,1.,1.,1.,1.,1.,1.,1.,1.,
1.,1.,1.,1.,1.,1.,1.,1.,1.,1.))
REPRESENTATION_ITEM('')
);
#746=(
BOUNDED_CURVE()
B_SPLINE_CURVE(5,(#51493,#51494,#51495,#51496,#51497,#51498,#51499,#51500,
#51501,#51502,#51503,#51504,#51505,#51506,#51507,#51508,#51509,#51510,#51511,
#51512,#51513,#51514,#51515,#51516,#51517,#51518,#51519,#51520,#51521),
 .UNSPECIFIED.,.F.,.F.)
B_SPLINE_CURVE_WITH_KNOTS((6,1,1,1,1,1,1,1,1,1,1,1,1,1,1,1,1,1,1,1,1,1,
1,1,6),(-0.670627588953113,-0.657142857142857,-0.628571428571429,-0.6,-0.571428571428572,
-0.542857142857143,-0.514285714285714,-0.485714285714286,-0.457142857142857,
-0.428571428571429,-0.4,-0.371428571428571,-0.342857142857143,-0.314285714285714,
-0.285714285714286,-0.257142857142857,-0.228571428571429,-0.2,-0.171428571428571,
-0.142857142857143,-0.114285714285714,-0.0857142857142857,-0.0571428571428571,
-0.0285714285714286,0.),.UNSPECIFIED.)
CURVE()
GEOMETRIC_REPRESENTATION_ITEM()
RATIONAL_B_SPLINE_CURVE((1.,1.,1.,1.,1.,1.,1.,1.,1.,1.,1.,1.,1.,1.,1.,1.,
1.,1.,1.,1.,1.,1.,1.,1.,1.,1.,1.,1.,1.))
REPRESENTATION_ITEM('')
);
#747=(
BOUNDED_CURVE()
B_SPLINE_CURVE(5,(#51525,#51526,#51527,#51528,#51529,#51530,#51531,#51532,
#51533,#51534,#51535,#51536,#51537,#51538,#51539,#51540,#51541,#51542,#51543,
#51544,#51545,#51546,#51547,#51548,#51549,#51550),.UNSPECIFIED.,.F.,.F.)
B_SPLINE_CURVE_WITH_KNOTS((6,1,1,1,1,1,1,1,1,1,1,1,1,1,1,1,1,1,1,1,1,6),
(-1.,-0.971428571428572,-0.942857142857143,-0.914285714285714,-0.885714285714286,
-0.857142857142857,-0.828571428571429,-0.8,-0.771428571428572,-0.742857142857143,
-0.714285714285714,-0.685714285714286,-0.657142857142857,-0.628571428571429,
-0.6,-0.571428571428572,-0.542857142857143,-0.514285714285714,-0.485714285714286,
-0.457142857142857,-0.428571428571429,-0.428061295609925),.UNSPECIFIED.)
CURVE()
GEOMETRIC_REPRESENTATION_ITEM()
RATIONAL_B_SPLINE_CURVE((1.,1.,1.,1.,1.,1.,1.,1.,1.,1.,1.,1.,1.,1.,1.,1.,
1.,1.,1.,1.,1.,1.,1.,1.,1.,1.))
REPRESENTATION_ITEM('')
);
#748=(
BOUNDED_CURVE()
B_SPLINE_CURVE(5,(#51554,#51555,#51556,#51557,#51558,#51559,#51560,#51561,
#51562,#51563,#51564,#51565,#51566,#51567,#51568,#51569,#51570,#51571,#51572,
#51573,#51574,#51575,#51576,#51577,#51578,#51579,#51580,#51581,#51582),
 .UNSPECIFIED.,.F.,.F.)
B_SPLINE_CURVE_WITH_KNOTS((6,1,1,1,1,1,1,1,1,1,1,1,1,1,1,1,1,1,1,1,1,1,
1,1,6),(-0.670627588953112,-0.657142857142857,-0.628571428571429,-0.6,-0.571428571428572,
-0.542857142857143,-0.514285714285714,-0.485714285714286,-0.457142857142857,
-0.428571428571429,-0.4,-0.371428571428571,-0.342857142857143,-0.314285714285714,
-0.285714285714286,-0.257142857142857,-0.228571428571429,-0.2,-0.171428571428571,
-0.142857142857143,-0.114285714285714,-0.0857142857142857,-0.0571428571428571,
-0.0285714285714286,0.),.UNSPECIFIED.)
CURVE()
GEOMETRIC_REPRESENTATION_ITEM()
RATIONAL_B_SPLINE_CURVE((1.,1.,1.,1.,1.,1.,1.,1.,1.,1.,1.,1.,1.,1.,1.,1.,
1.,1.,1.,1.,1.,1.,1.,1.,1.,1.,1.,1.,1.))
REPRESENTATION_ITEM('')
);
#749=(
BOUNDED_CURVE()
B_SPLINE_CURVE(5,(#51586,#51587,#51588,#51589,#51590,#51591,#51592,#51593,
#51594,#51595,#51596,#51597,#51598,#51599,#51600,#51601,#51602,#51603,#51604,
#51605,#51606,#51607,#51608,#51609,#51610,#51611),.UNSPECIFIED.,.F.,.F.)
B_SPLINE_CURVE_WITH_KNOTS((6,1,1,1,1,1,1,1,1,1,1,1,1,1,1,1,1,1,1,1,1,6),
(-1.,-0.971428571428572,-0.942857142857143,-0.914285714285714,-0.885714285714286,
-0.857142857142857,-0.828571428571429,-0.8,-0.771428571428572,-0.742857142857143,
-0.714285714285714,-0.685714285714286,-0.657142857142857,-0.628571428571429,
-0.6,-0.571428571428572,-0.542857142857143,-0.514285714285714,-0.485714285714286,
-0.457142857142857,-0.428571428571429,-0.428061295609926),.UNSPECIFIED.)
CURVE()
GEOMETRIC_REPRESENTATION_ITEM()
RATIONAL_B_SPLINE_CURVE((1.,1.,1.,1.,1.,1.,1.,1.,1.,1.,1.,1.,1.,1.,1.,1.,
1.,1.,1.,1.,1.,1.,1.,1.,1.,1.))
REPRESENTATION_ITEM('')
);
#750=(
BOUNDED_CURVE()
B_SPLINE_CURVE(5,(#51704,#51705,#51706,#51707,#51708,#51709,#51710,#51711,
#51712,#51713,#51714,#51715,#51716,#51717,#51718,#51719,#51720,#51721,#51722,
#51723,#51724,#51725,#51726,#51727,#51728,#51729,#51730,#51731,#51732,#51733,
#51734,#51735,#51736,#51737),.UNSPECIFIED.,.F.,.F.)
B_SPLINE_CURVE_WITH_KNOTS((6,1,1,1,1,1,1,1,1,1,1,1,1,1,1,1,1,1,1,1,1,1,
1,1,1,1,1,1,1,6),(0.,0.0285714285714286,0.0571428571428571,0.0857142857142857,
0.114285714285714,0.142857142857143,0.171428571428571,0.2,0.228571428571429,
0.257142857142857,0.285714285714286,0.314285714285714,0.342857142857143,
0.371428571428571,0.4,0.428571428571429,0.457142857142857,0.485714285714286,
0.514285714285714,0.542857142857143,0.571428571428572,0.6,0.628571428571429,
0.657142857142857,0.685714285714286,0.714285714285714,0.742857142857143,
0.771428571428572,0.8,0.816564825616131),.UNSPECIFIED.)
CURVE()
GEOMETRIC_REPRESENTATION_ITEM()
RATIONAL_B_SPLINE_CURVE((1.,1.,1.,1.,1.,1.,1.,1.,1.,1.,1.,1.,1.,1.,1.,1.,
1.,1.,1.,1.,1.,1.,1.,1.,1.,1.,1.,1.,1.,1.,1.,1.,1.,1.))
REPRESENTATION_ITEM('')
);
#751=(
BOUNDED_CURVE()
B_SPLINE_CURVE(5,(#51842,#51843,#51844,#51845,#51846,#51847,#51848,#51849,
#51850,#51851,#51852,#51853,#51854,#51855,#51856,#51857,#51858,#51859,#51860,
#51861,#51862,#51863,#51864,#51865,#51866,#51867,#51868,#51869,#51870),
 .UNSPECIFIED.,.F.,.F.)
B_SPLINE_CURVE_WITH_KNOTS((6,1,1,1,1,1,1,1,1,1,1,1,1,1,1,1,1,1,1,1,1,1,
1,1,6),(0.315728291775709,0.342857142857143,0.371428571428571,0.4,0.428571428571429,
0.457142857142857,0.485714285714286,0.514285714285714,0.542857142857143,
0.571428571428572,0.6,0.628571428571429,0.657142857142857,0.685714285714286,
0.714285714285714,0.742857142857143,0.771428571428572,0.8,0.828571428571429,
0.857142857142857,0.885714285714286,0.914285714285714,0.942857142857143,
0.971428571428572,1.),.UNSPECIFIED.)
CURVE()
GEOMETRIC_REPRESENTATION_ITEM()
RATIONAL_B_SPLINE_CURVE((1.,1.,1.,1.,1.,1.,1.,1.,1.,1.,1.,1.,1.,1.,1.,1.,
1.,1.,1.,1.,1.,1.,1.,1.,1.,1.,1.,1.,1.))
REPRESENTATION_ITEM('')
);
#752=(
BOUNDED_CURVE()
B_SPLINE_CURVE(5,(#51978,#51979,#51980,#51981,#51982,#51983,#51984,#51985,
#51986,#51987,#51988,#51989,#51990,#51991,#51992,#51993,#51994,#51995,#51996,
#51997,#51998,#51999,#52000,#52001,#52002,#52003,#52004,#52005,#52006),
 .UNSPECIFIED.,.F.,.F.)
B_SPLINE_CURVE_WITH_KNOTS((6,1,1,1,1,1,1,1,1,1,1,1,1,1,1,1,1,1,1,1,1,1,
1,1,6),(0.315728291775709,0.342857142857143,0.371428571428571,0.4,0.428571428571429,
0.457142857142857,0.485714285714286,0.514285714285714,0.542857142857143,
0.571428571428572,0.6,0.628571428571429,0.657142857142857,0.685714285714286,
0.714285714285714,0.742857142857143,0.771428571428572,0.8,0.828571428571429,
0.857142857142857,0.885714285714286,0.914285714285714,0.942857142857143,
0.971428571428572,1.),.UNSPECIFIED.)
CURVE()
GEOMETRIC_REPRESENTATION_ITEM()
RATIONAL_B_SPLINE_CURVE((1.,1.,1.,1.,1.,1.,1.,1.,1.,1.,1.,1.,1.,1.,1.,1.,
1.,1.,1.,1.,1.,1.,1.,1.,1.,1.,1.,1.,1.))
REPRESENTATION_ITEM('')
);
#753=(
BOUNDED_CURVE()
B_SPLINE_CURVE(5,(#52110,#52111,#52112,#52113,#52114,#52115,#52116,#52117,
#52118,#52119,#52120,#52121,#52122,#52123,#52124,#52125,#52126,#52127,#52128,
#52129,#52130,#52131,#52132,#52133,#52134,#52135,#52136,#52137,#52138,#52139,
#52140,#52141,#52142,#52143),.UNSPECIFIED.,.F.,.F.)
B_SPLINE_CURVE_WITH_KNOTS((6,1,1,1,1,1,1,1,1,1,1,1,1,1,1,1,1,1,1,1,1,1,
1,1,1,1,1,1,1,6),(0.,0.0285714285714286,0.0571428571428571,0.0857142857142857,
0.114285714285714,0.142857142857143,0.171428571428571,0.2,0.228571428571429,
0.257142857142857,0.285714285714286,0.314285714285714,0.342857142857143,
0.371428571428571,0.4,0.428571428571429,0.457142857142857,0.485714285714286,
0.514285714285714,0.542857142857143,0.571428571428572,0.6,0.628571428571429,
0.657142857142857,0.685714285714286,0.714285714285714,0.742857142857143,
0.771428571428572,0.8,0.816564825616034),.UNSPECIFIED.)
CURVE()
GEOMETRIC_REPRESENTATION_ITEM()
RATIONAL_B_SPLINE_CURVE((1.,1.,1.,1.,1.,1.,1.,1.,1.,1.,1.,1.,1.,1.,1.,1.,
1.,1.,1.,1.,1.,1.,1.,1.,1.,1.,1.,1.,1.,1.,1.,1.,1.,1.))
REPRESENTATION_ITEM('')
);
#754=(
BOUNDED_CURVE()
B_SPLINE_CURVE(5,(#52147,#52148,#52149,#52150,#52151,#52152,#52153,#52154,
#52155,#52156,#52157,#52158,#52159,#52160,#52161,#52162,#52163,#52164,#52165,
#52166,#52167,#52168,#52169,#52170,#52171,#52172,#52173,#52174,#52175),
 .UNSPECIFIED.,.F.,.F.)
B_SPLINE_CURVE_WITH_KNOTS((6,1,1,1,1,1,1,1,1,1,1,1,1,1,1,1,1,1,1,1,1,1,
1,1,6),(0.,0.0285714285714286,0.0571428571428571,0.0857142857142857,0.114285714285714,
0.142857142857143,0.171428571428571,0.2,0.228571428571429,0.257142857142857,
0.285714285714286,0.314285714285714,0.342857142857143,0.371428571428571,
0.4,0.428571428571429,0.457142857142857,0.485714285714286,0.514285714285714,
0.542857142857143,0.571428571428572,0.6,0.628571428571429,0.657142857142857,
0.670627588953113),.UNSPECIFIED.)
CURVE()
GEOMETRIC_REPRESENTATION_ITEM()
RATIONAL_B_SPLINE_CURVE((1.,1.,1.,1.,1.,1.,1.,1.,1.,1.,1.,1.,1.,1.,1.,1.,
1.,1.,1.,1.,1.,1.,1.,1.,1.,1.,1.,1.,1.))
REPRESENTATION_ITEM('')
);
#755=(
BOUNDED_CURVE()
B_SPLINE_CURVE(5,(#52179,#52180,#52181,#52182,#52183,#52184,#52185,#52186,
#52187,#52188,#52189,#52190,#52191,#52192,#52193,#52194,#52195,#52196,#52197,
#52198,#52199,#52200,#52201,#52202,#52203,#52204),.UNSPECIFIED.,.F.,.F.)
B_SPLINE_CURVE_WITH_KNOTS((6,1,1,1,1,1,1,1,1,1,1,1,1,1,1,1,1,1,1,1,1,6),
(0.428061295609926,0.428571428571429,0.457142857142857,0.485714285714286,
0.514285714285714,0.542857142857143,0.571428571428572,0.6,0.628571428571429,
0.657142857142857,0.685714285714286,0.714285714285714,0.742857142857143,
0.771428571428572,0.8,0.828571428571429,0.857142857142857,0.885714285714286,
0.914285714285714,0.942857142857143,0.971428571428572,1.),.UNSPECIFIED.)
CURVE()
GEOMETRIC_REPRESENTATION_ITEM()
RATIONAL_B_SPLINE_CURVE((1.,1.,1.,1.,1.,1.,1.,1.,1.,1.,1.,1.,1.,1.,1.,1.,
1.,1.,1.,1.,1.,1.,1.,1.,1.,1.))
REPRESENTATION_ITEM('')
);
#756=(
BOUNDED_CURVE()
B_SPLINE_CURVE(5,(#52208,#52209,#52210,#52211,#52212,#52213,#52214,#52215,
#52216,#52217,#52218,#52219,#52220,#52221,#52222,#52223,#52224,#52225,#52226,
#52227,#52228,#52229,#52230,#52231,#52232,#52233,#52234,#52235,#52236),
 .UNSPECIFIED.,.F.,.F.)
B_SPLINE_CURVE_WITH_KNOTS((6,1,1,1,1,1,1,1,1,1,1,1,1,1,1,1,1,1,1,1,1,1,
1,1,6),(0.,0.0285714285714286,0.0571428571428571,0.0857142857142857,0.114285714285714,
0.142857142857143,0.171428571428571,0.2,0.228571428571429,0.257142857142857,
0.285714285714286,0.314285714285714,0.342857142857143,0.371428571428571,
0.4,0.428571428571429,0.457142857142857,0.485714285714286,0.514285714285714,
0.542857142857143,0.571428571428572,0.6,0.628571428571429,0.657142857142857,
0.670627588953112),.UNSPECIFIED.)
CURVE()
GEOMETRIC_REPRESENTATION_ITEM()
RATIONAL_B_SPLINE_CURVE((1.,1.,1.,1.,1.,1.,1.,1.,1.,1.,1.,1.,1.,1.,1.,1.,
1.,1.,1.,1.,1.,1.,1.,1.,1.,1.,1.,1.,1.))
REPRESENTATION_ITEM('')
);
#757=(
BOUNDED_CURVE()
B_SPLINE_CURVE(5,(#52240,#52241,#52242,#52243,#52244,#52245,#52246,#52247,
#52248,#52249,#52250,#52251,#52252,#52253,#52254,#52255,#52256,#52257,#52258,
#52259,#52260,#52261,#52262,#52263,#52264,#52265),.UNSPECIFIED.,.F.,.F.)
B_SPLINE_CURVE_WITH_KNOTS((6,1,1,1,1,1,1,1,1,1,1,1,1,1,1,1,1,1,1,1,1,6),
(0.428061295609925,0.428571428571429,0.457142857142857,0.485714285714286,
0.514285714285714,0.542857142857143,0.571428571428572,0.6,0.628571428571429,
0.657142857142857,0.685714285714286,0.714285714285714,0.742857142857143,
0.771428571428572,0.8,0.828571428571429,0.857142857142857,0.885714285714286,
0.914285714285714,0.942857142857143,0.971428571428572,1.),.UNSPECIFIED.)
CURVE()
GEOMETRIC_REPRESENTATION_ITEM()
RATIONAL_B_SPLINE_CURVE((1.,1.,1.,1.,1.,1.,1.,1.,1.,1.,1.,1.,1.,1.,1.,1.,
1.,1.,1.,1.,1.,1.,1.,1.,1.,1.))
REPRESENTATION_ITEM('')
);
#758=(
BOUNDED_CURVE()
B_SPLINE_CURVE(5,(#52269,#52270,#52271,#52272,#52273,#52274,#52275,#52276,
#52277,#52278,#52279,#52280,#52281,#52282,#52283,#52284,#52285,#52286,#52287,
#52288,#52289,#52290,#52291,#52292,#52293,#52294,#52295,#52296,#52297),
 .UNSPECIFIED.,.F.,.F.)
B_SPLINE_CURVE_WITH_KNOTS((6,1,1,1,1,1,1,1,1,1,1,1,1,1,1,1,1,1,1,1,1,1,
1,1,6),(0.,0.0285714285714286,0.0571428571428571,0.0857142857142857,0.114285714285714,
0.142857142857143,0.171428571428571,0.2,0.228571428571429,0.257142857142857,
0.285714285714286,0.314285714285714,0.342857142857143,0.371428571428571,
0.4,0.428571428571429,0.457142857142857,0.485714285714286,0.514285714285714,
0.542857142857143,0.571428571428572,0.6,0.628571428571429,0.657142857142857,
0.670627588953113),.UNSPECIFIED.)
CURVE()
GEOMETRIC_REPRESENTATION_ITEM()
RATIONAL_B_SPLINE_CURVE((1.,1.,1.,1.,1.,1.,1.,1.,1.,1.,1.,1.,1.,1.,1.,1.,
1.,1.,1.,1.,1.,1.,1.,1.,1.,1.,1.,1.,1.))
REPRESENTATION_ITEM('')
);
#759=(
BOUNDED_CURVE()
B_SPLINE_CURVE(5,(#52301,#52302,#52303,#52304,#52305,#52306,#52307,#52308,
#52309,#52310,#52311,#52312,#52313,#52314,#52315,#52316,#52317,#52318,#52319,
#52320,#52321,#52322,#52323,#52324,#52325,#52326),.UNSPECIFIED.,.F.,.F.)
B_SPLINE_CURVE_WITH_KNOTS((6,1,1,1,1,1,1,1,1,1,1,1,1,1,1,1,1,1,1,1,1,6),
(0.428061295609926,0.428571428571429,0.457142857142857,0.485714285714286,
0.514285714285714,0.542857142857143,0.571428571428572,0.6,0.628571428571429,
0.657142857142857,0.685714285714286,0.714285714285714,0.742857142857143,
0.771428571428572,0.8,0.828571428571429,0.857142857142857,0.885714285714286,
0.914285714285714,0.942857142857143,0.971428571428572,1.),.UNSPECIFIED.)
CURVE()
GEOMETRIC_REPRESENTATION_ITEM()
RATIONAL_B_SPLINE_CURVE((1.,1.,1.,1.,1.,1.,1.,1.,1.,1.,1.,1.,1.,1.,1.,1.,
1.,1.,1.,1.,1.,1.,1.,1.,1.,1.))
REPRESENTATION_ITEM('')
);
#760=(
BOUNDED_CURVE()
B_SPLINE_CURVE(5,(#52330,#52331,#52332,#52333,#52334,#52335,#52336,#52337,
#52338,#52339,#52340,#52341,#52342,#52343,#52344,#52345,#52346,#52347,#52348,
#52349,#52350,#52351,#52352,#52353,#52354,#52355,#52356,#52357,#52358),
 .UNSPECIFIED.,.F.,.F.)
B_SPLINE_CURVE_WITH_KNOTS((6,1,1,1,1,1,1,1,1,1,1,1,1,1,1,1,1,1,1,1,1,1,
1,1,6),(0.,0.0285714285714286,0.0571428571428571,0.0857142857142857,0.114285714285714,
0.142857142857143,0.171428571428571,0.2,0.228571428571429,0.257142857142857,
0.285714285714286,0.314285714285714,0.342857142857143,0.371428571428571,
0.4,0.428571428571429,0.457142857142857,0.485714285714286,0.514285714285714,
0.542857142857143,0.571428571428572,0.6,0.628571428571429,0.657142857142857,
0.670627588953113),.UNSPECIFIED.)
CURVE()
GEOMETRIC_REPRESENTATION_ITEM()
RATIONAL_B_SPLINE_CURVE((1.,1.,1.,1.,1.,1.,1.,1.,1.,1.,1.,1.,1.,1.,1.,1.,
1.,1.,1.,1.,1.,1.,1.,1.,1.,1.,1.,1.,1.))
REPRESENTATION_ITEM('')
);
#761=(
BOUNDED_CURVE()
B_SPLINE_CURVE(5,(#52362,#52363,#52364,#52365,#52366,#52367,#52368,#52369,
#52370,#52371,#52372,#52373,#52374,#52375,#52376,#52377,#52378,#52379,#52380,
#52381,#52382,#52383,#52384,#52385,#52386,#52387),.UNSPECIFIED.,.F.,.F.)
B_SPLINE_CURVE_WITH_KNOTS((6,1,1,1,1,1,1,1,1,1,1,1,1,1,1,1,1,1,1,1,1,6),
(0.428061295609926,0.428571428571429,0.457142857142857,0.485714285714286,
0.514285714285714,0.542857142857143,0.571428571428572,0.6,0.628571428571429,
0.657142857142857,0.685714285714286,0.714285714285714,0.742857142857143,
0.771428571428572,0.8,0.828571428571429,0.857142857142857,0.885714285714286,
0.914285714285714,0.942857142857143,0.971428571428572,1.),.UNSPECIFIED.)
CURVE()
GEOMETRIC_REPRESENTATION_ITEM()
RATIONAL_B_SPLINE_CURVE((1.,1.,1.,1.,1.,1.,1.,1.,1.,1.,1.,1.,1.,1.,1.,1.,
1.,1.,1.,1.,1.,1.,1.,1.,1.,1.))
REPRESENTATION_ITEM('')
);
#762=(
BOUNDED_CURVE()
B_SPLINE_CURVE(5,(#52391,#52392,#52393,#52394,#52395,#52396,#52397,#52398,
#52399,#52400,#52401,#52402,#52403,#52404,#52405,#52406,#52407,#52408,#52409,
#52410,#52411,#52412,#52413,#52414,#52415,#52416,#52417,#52418,#52419),
 .UNSPECIFIED.,.F.,.F.)
B_SPLINE_CURVE_WITH_KNOTS((6,1,1,1,1,1,1,1,1,1,1,1,1,1,1,1,1,1,1,1,1,1,
1,1,6),(0.,0.0285714285714286,0.0571428571428571,0.0857142857142857,0.114285714285714,
0.142857142857143,0.171428571428571,0.2,0.228571428571429,0.257142857142857,
0.285714285714286,0.314285714285714,0.342857142857143,0.371428571428571,
0.4,0.428571428571429,0.457142857142857,0.485714285714286,0.514285714285714,
0.542857142857143,0.571428571428572,0.6,0.628571428571429,0.657142857142857,
0.670627588953112),.UNSPECIFIED.)
CURVE()
GEOMETRIC_REPRESENTATION_ITEM()
RATIONAL_B_SPLINE_CURVE((1.,1.,1.,1.,1.,1.,1.,1.,1.,1.,1.,1.,1.,1.,1.,1.,
1.,1.,1.,1.,1.,1.,1.,1.,1.,1.,1.,1.,1.))
REPRESENTATION_ITEM('')
);
#763=(
BOUNDED_CURVE()
B_SPLINE_CURVE(5,(#52423,#52424,#52425,#52426,#52427,#52428,#52429,#52430,
#52431,#52432,#52433,#52434,#52435,#52436,#52437,#52438,#52439,#52440,#52441,
#52442,#52443,#52444,#52445,#52446,#52447,#52448),.UNSPECIFIED.,.F.,.F.)
B_SPLINE_CURVE_WITH_KNOTS((6,1,1,1,1,1,1,1,1,1,1,1,1,1,1,1,1,1,1,1,1,6),
(0.428061295609926,0.428571428571429,0.457142857142857,0.485714285714286,
0.514285714285714,0.542857142857143,0.571428571428572,0.6,0.628571428571429,
0.657142857142857,0.685714285714286,0.714285714285714,0.742857142857143,
0.771428571428572,0.8,0.828571428571429,0.857142857142857,0.885714285714286,
0.914285714285714,0.942857142857143,0.971428571428572,1.),.UNSPECIFIED.)
CURVE()
GEOMETRIC_REPRESENTATION_ITEM()
RATIONAL_B_SPLINE_CURVE((1.,1.,1.,1.,1.,1.,1.,1.,1.,1.,1.,1.,1.,1.,1.,1.,
1.,1.,1.,1.,1.,1.,1.,1.,1.,1.))
REPRESENTATION_ITEM('')
);
#764=(
BOUNDED_CURVE()
B_SPLINE_CURVE(5,(#52452,#52453,#52454,#52455,#52456,#52457,#52458,#52459,
#52460,#52461,#52462,#52463,#52464,#52465,#52466,#52467,#52468,#52469,#52470,
#52471,#52472,#52473,#52474,#52475,#52476,#52477,#52478,#52479,#52480),
 .UNSPECIFIED.,.F.,.F.)
B_SPLINE_CURVE_WITH_KNOTS((6,1,1,1,1,1,1,1,1,1,1,1,1,1,1,1,1,1,1,1,1,1,
1,1,6),(0.,0.0285714285714286,0.0571428571428571,0.0857142857142857,0.114285714285714,
0.142857142857143,0.171428571428571,0.2,0.228571428571429,0.257142857142857,
0.285714285714286,0.314285714285714,0.342857142857143,0.371428571428571,
0.4,0.428571428571429,0.457142857142857,0.485714285714286,0.514285714285714,
0.542857142857143,0.571428571428572,0.6,0.628571428571429,0.657142857142857,
0.670627588953113),.UNSPECIFIED.)
CURVE()
GEOMETRIC_REPRESENTATION_ITEM()
RATIONAL_B_SPLINE_CURVE((1.,1.,1.,1.,1.,1.,1.,1.,1.,1.,1.,1.,1.,1.,1.,1.,
1.,1.,1.,1.,1.,1.,1.,1.,1.,1.,1.,1.,1.))
REPRESENTATION_ITEM('')
);
#765=(
BOUNDED_CURVE()
B_SPLINE_CURVE(5,(#52484,#52485,#52486,#52487,#52488,#52489,#52490,#52491,
#52492,#52493,#52494,#52495,#52496,#52497,#52498,#52499,#52500,#52501,#52502,
#52503,#52504,#52505,#52506,#52507,#52508,#52509),.UNSPECIFIED.,.F.,.F.)
B_SPLINE_CURVE_WITH_KNOTS((6,1,1,1,1,1,1,1,1,1,1,1,1,1,1,1,1,1,1,1,1,6),
(0.428061295609926,0.428571428571429,0.457142857142857,0.485714285714286,
0.514285714285714,0.542857142857143,0.571428571428572,0.6,0.628571428571429,
0.657142857142857,0.685714285714286,0.714285714285714,0.742857142857143,
0.771428571428572,0.8,0.828571428571429,0.857142857142857,0.885714285714286,
0.914285714285714,0.942857142857143,0.971428571428572,1.),.UNSPECIFIED.)
CURVE()
GEOMETRIC_REPRESENTATION_ITEM()
RATIONAL_B_SPLINE_CURVE((1.,1.,1.,1.,1.,1.,1.,1.,1.,1.,1.,1.,1.,1.,1.,1.,
1.,1.,1.,1.,1.,1.,1.,1.,1.,1.))
REPRESENTATION_ITEM('')
);
#766=(
BOUNDED_CURVE()
B_SPLINE_CURVE(5,(#52513,#52514,#52515,#52516,#52517,#52518,#52519,#52520,
#52521,#52522,#52523,#52524,#52525,#52526,#52527,#52528,#52529,#52530,#52531,
#52532,#52533,#52534,#52535,#52536,#52537,#52538,#52539,#52540,#52541),
 .UNSPECIFIED.,.F.,.F.)
B_SPLINE_CURVE_WITH_KNOTS((6,1,1,1,1,1,1,1,1,1,1,1,1,1,1,1,1,1,1,1,1,1,
1,1,6),(0.,0.0285714285714286,0.0571428571428571,0.0857142857142857,0.114285714285714,
0.142857142857143,0.171428571428571,0.2,0.228571428571429,0.257142857142857,
0.285714285714286,0.314285714285714,0.342857142857143,0.371428571428571,
0.4,0.428571428571429,0.457142857142857,0.485714285714286,0.514285714285714,
0.542857142857143,0.571428571428572,0.6,0.628571428571429,0.657142857142857,
0.670627588953113),.UNSPECIFIED.)
CURVE()
GEOMETRIC_REPRESENTATION_ITEM()
RATIONAL_B_SPLINE_CURVE((1.,1.,1.,1.,1.,1.,1.,1.,1.,1.,1.,1.,1.,1.,1.,1.,
1.,1.,1.,1.,1.,1.,1.,1.,1.,1.,1.,1.,1.))
REPRESENTATION_ITEM('')
);
#767=(
BOUNDED_CURVE()
B_SPLINE_CURVE(5,(#52545,#52546,#52547,#52548,#52549,#52550,#52551,#52552,
#52553,#52554,#52555,#52556,#52557,#52558,#52559,#52560,#52561,#52562,#52563,
#52564,#52565,#52566,#52567,#52568,#52569,#52570),.UNSPECIFIED.,.F.,.F.)
B_SPLINE_CURVE_WITH_KNOTS((6,1,1,1,1,1,1,1,1,1,1,1,1,1,1,1,1,1,1,1,1,6),
(0.428061295609926,0.428571428571429,0.457142857142857,0.485714285714286,
0.514285714285714,0.542857142857143,0.571428571428572,0.6,0.628571428571429,
0.657142857142857,0.685714285714286,0.714285714285714,0.742857142857143,
0.771428571428572,0.8,0.828571428571429,0.857142857142857,0.885714285714286,
0.914285714285714,0.942857142857143,0.971428571428572,1.),.UNSPECIFIED.)
CURVE()
GEOMETRIC_REPRESENTATION_ITEM()
RATIONAL_B_SPLINE_CURVE((1.,1.,1.,1.,1.,1.,1.,1.,1.,1.,1.,1.,1.,1.,1.,1.,
1.,1.,1.,1.,1.,1.,1.,1.,1.,1.))
REPRESENTATION_ITEM('')
);
#768=(
BOUNDED_CURVE()
B_SPLINE_CURVE(5,(#52574,#52575,#52576,#52577,#52578,#52579,#52580,#52581,
#52582,#52583,#52584,#52585,#52586,#52587,#52588,#52589,#52590,#52591,#52592,
#52593,#52594,#52595,#52596,#52597,#52598,#52599,#52600,#52601,#52602),
 .UNSPECIFIED.,.F.,.F.)
B_SPLINE_CURVE_WITH_KNOTS((6,1,1,1,1,1,1,1,1,1,1,1,1,1,1,1,1,1,1,1,1,1,
1,1,6),(0.,0.0285714285714286,0.0571428571428571,0.0857142857142857,0.114285714285714,
0.142857142857143,0.171428571428571,0.2,0.228571428571429,0.257142857142857,
0.285714285714286,0.314285714285714,0.342857142857143,0.371428571428571,
0.4,0.428571428571429,0.457142857142857,0.485714285714286,0.514285714285714,
0.542857142857143,0.571428571428572,0.6,0.628571428571429,0.657142857142857,
0.670627588953112),.UNSPECIFIED.)
CURVE()
GEOMETRIC_REPRESENTATION_ITEM()
RATIONAL_B_SPLINE_CURVE((1.,1.,1.,1.,1.,1.,1.,1.,1.,1.,1.,1.,1.,1.,1.,1.,
1.,1.,1.,1.,1.,1.,1.,1.,1.,1.,1.,1.,1.))
REPRESENTATION_ITEM('')
);
#769=(
BOUNDED_CURVE()
B_SPLINE_CURVE(5,(#52606,#52607,#52608,#52609,#52610,#52611,#52612,#52613,
#52614,#52615,#52616,#52617,#52618,#52619,#52620,#52621,#52622,#52623,#52624,
#52625,#52626,#52627,#52628,#52629,#52630,#52631),.UNSPECIFIED.,.F.,.F.)
B_SPLINE_CURVE_WITH_KNOTS((6,1,1,1,1,1,1,1,1,1,1,1,1,1,1,1,1,1,1,1,1,6),
(0.428061295609926,0.428571428571429,0.457142857142857,0.485714285714286,
0.514285714285714,0.542857142857143,0.571428571428572,0.6,0.628571428571429,
0.657142857142857,0.685714285714286,0.714285714285714,0.742857142857143,
0.771428571428572,0.8,0.828571428571429,0.857142857142857,0.885714285714286,
0.914285714285714,0.942857142857143,0.971428571428572,1.),.UNSPECIFIED.)
CURVE()
GEOMETRIC_REPRESENTATION_ITEM()
RATIONAL_B_SPLINE_CURVE((1.,1.,1.,1.,1.,1.,1.,1.,1.,1.,1.,1.,1.,1.,1.,1.,
1.,1.,1.,1.,1.,1.,1.,1.,1.,1.))
REPRESENTATION_ITEM('')
);
#770=(
BOUNDED_CURVE()
B_SPLINE_CURVE(5,(#52635,#52636,#52637,#52638,#52639,#52640,#52641,#52642,
#52643,#52644,#52645,#52646,#52647,#52648,#52649,#52650,#52651,#52652,#52653,
#52654,#52655,#52656,#52657,#52658,#52659,#52660,#52661,#52662,#52663),
 .UNSPECIFIED.,.F.,.F.)
B_SPLINE_CURVE_WITH_KNOTS((6,1,1,1,1,1,1,1,1,1,1,1,1,1,1,1,1,1,1,1,1,1,
1,1,6),(0.,0.0285714285714286,0.0571428571428571,0.0857142857142857,0.114285714285714,
0.142857142857143,0.171428571428571,0.2,0.228571428571429,0.257142857142857,
0.285714285714286,0.314285714285714,0.342857142857143,0.371428571428571,
0.4,0.428571428571429,0.457142857142857,0.485714285714286,0.514285714285714,
0.542857142857143,0.571428571428572,0.6,0.628571428571429,0.657142857142857,
0.670627588953113),.UNSPECIFIED.)
CURVE()
GEOMETRIC_REPRESENTATION_ITEM()
RATIONAL_B_SPLINE_CURVE((1.,1.,1.,1.,1.,1.,1.,1.,1.,1.,1.,1.,1.,1.,1.,1.,
1.,1.,1.,1.,1.,1.,1.,1.,1.,1.,1.,1.,1.))
REPRESENTATION_ITEM('')
);
#771=(
BOUNDED_CURVE()
B_SPLINE_CURVE(5,(#52667,#52668,#52669,#52670,#52671,#52672,#52673,#52674,
#52675,#52676,#52677,#52678,#52679,#52680,#52681,#52682,#52683,#52684,#52685,
#52686,#52687,#52688,#52689,#52690,#52691,#52692),.UNSPECIFIED.,.F.,.F.)
B_SPLINE_CURVE_WITH_KNOTS((6,1,1,1,1,1,1,1,1,1,1,1,1,1,1,1,1,1,1,1,1,6),
(0.428061295609925,0.428571428571429,0.457142857142857,0.485714285714286,
0.514285714285714,0.542857142857143,0.571428571428572,0.6,0.628571428571429,
0.657142857142857,0.685714285714286,0.714285714285714,0.742857142857143,
0.771428571428572,0.8,0.828571428571429,0.857142857142857,0.885714285714286,
0.914285714285714,0.942857142857143,0.971428571428572,1.),.UNSPECIFIED.)
CURVE()
GEOMETRIC_REPRESENTATION_ITEM()
RATIONAL_B_SPLINE_CURVE((1.,1.,1.,1.,1.,1.,1.,1.,1.,1.,1.,1.,1.,1.,1.,1.,
1.,1.,1.,1.,1.,1.,1.,1.,1.,1.))
REPRESENTATION_ITEM('')
);
#772=(
BOUNDED_CURVE()
B_SPLINE_CURVE(5,(#52696,#52697,#52698,#52699,#52700,#52701,#52702,#52703,
#52704,#52705,#52706,#52707,#52708,#52709,#52710,#52711,#52712,#52713,#52714,
#52715,#52716,#52717,#52718,#52719,#52720,#52721,#52722,#52723,#52724),
 .UNSPECIFIED.,.F.,.F.)
B_SPLINE_CURVE_WITH_KNOTS((6,1,1,1,1,1,1,1,1,1,1,1,1,1,1,1,1,1,1,1,1,1,
1,1,6),(0.,0.0285714285714286,0.0571428571428571,0.0857142857142857,0.114285714285714,
0.142857142857143,0.171428571428571,0.2,0.228571428571429,0.257142857142857,
0.285714285714286,0.314285714285714,0.342857142857143,0.371428571428571,
0.4,0.428571428571429,0.457142857142857,0.485714285714286,0.514285714285714,
0.542857142857143,0.571428571428572,0.6,0.628571428571429,0.657142857142857,
0.670627588953112),.UNSPECIFIED.)
CURVE()
GEOMETRIC_REPRESENTATION_ITEM()
RATIONAL_B_SPLINE_CURVE((1.,1.,1.,1.,1.,1.,1.,1.,1.,1.,1.,1.,1.,1.,1.,1.,
1.,1.,1.,1.,1.,1.,1.,1.,1.,1.,1.,1.,1.))
REPRESENTATION_ITEM('')
);
#773=(
BOUNDED_CURVE()
B_SPLINE_CURVE(5,(#52728,#52729,#52730,#52731,#52732,#52733,#52734,#52735,
#52736,#52737,#52738,#52739,#52740,#52741,#52742,#52743,#52744,#52745,#52746,
#52747,#52748,#52749,#52750,#52751,#52752,#52753),.UNSPECIFIED.,.F.,.F.)
B_SPLINE_CURVE_WITH_KNOTS((6,1,1,1,1,1,1,1,1,1,1,1,1,1,1,1,1,1,1,1,1,6),
(0.428061295609926,0.428571428571429,0.457142857142857,0.485714285714286,
0.514285714285714,0.542857142857143,0.571428571428572,0.6,0.628571428571429,
0.657142857142857,0.685714285714286,0.714285714285714,0.742857142857143,
0.771428571428572,0.8,0.828571428571429,0.857142857142857,0.885714285714286,
0.914285714285714,0.942857142857143,0.971428571428572,1.),.UNSPECIFIED.)
CURVE()
GEOMETRIC_REPRESENTATION_ITEM()
RATIONAL_B_SPLINE_CURVE((1.,1.,1.,1.,1.,1.,1.,1.,1.,1.,1.,1.,1.,1.,1.,1.,
1.,1.,1.,1.,1.,1.,1.,1.,1.,1.))
REPRESENTATION_ITEM('')
);
#774=(
BOUNDED_CURVE()
B_SPLINE_CURVE(5,(#52757,#52758,#52759,#52760,#52761,#52762,#52763,#52764,
#52765,#52766,#52767,#52768,#52769,#52770,#52771,#52772,#52773,#52774,#52775,
#52776,#52777,#52778,#52779,#52780,#52781,#52782,#52783,#52784,#52785),
 .UNSPECIFIED.,.F.,.F.)
B_SPLINE_CURVE_WITH_KNOTS((6,1,1,1,1,1,1,1,1,1,1,1,1,1,1,1,1,1,1,1,1,1,
1,1,6),(0.,0.0285714285714286,0.0571428571428571,0.0857142857142857,0.114285714285714,
0.142857142857143,0.171428571428571,0.2,0.228571428571429,0.257142857142857,
0.285714285714286,0.314285714285714,0.342857142857143,0.371428571428571,
0.4,0.428571428571429,0.457142857142857,0.485714285714286,0.514285714285714,
0.542857142857143,0.571428571428572,0.6,0.628571428571429,0.657142857142857,
0.670627588953112),.UNSPECIFIED.)
CURVE()
GEOMETRIC_REPRESENTATION_ITEM()
RATIONAL_B_SPLINE_CURVE((1.,1.,1.,1.,1.,1.,1.,1.,1.,1.,1.,1.,1.,1.,1.,1.,
1.,1.,1.,1.,1.,1.,1.,1.,1.,1.,1.,1.,1.))
REPRESENTATION_ITEM('')
);
#775=(
BOUNDED_CURVE()
B_SPLINE_CURVE(5,(#52789,#52790,#52791,#52792,#52793,#52794,#52795,#52796,
#52797,#52798,#52799,#52800,#52801,#52802,#52803,#52804,#52805,#52806,#52807,
#52808,#52809,#52810,#52811,#52812,#52813,#52814),.UNSPECIFIED.,.F.,.F.)
B_SPLINE_CURVE_WITH_KNOTS((6,1,1,1,1,1,1,1,1,1,1,1,1,1,1,1,1,1,1,1,1,6),
(0.428061295609925,0.428571428571429,0.457142857142857,0.485714285714286,
0.514285714285714,0.542857142857143,0.571428571428572,0.6,0.628571428571429,
0.657142857142857,0.685714285714286,0.714285714285714,0.742857142857143,
0.771428571428572,0.8,0.828571428571429,0.857142857142857,0.885714285714286,
0.914285714285714,0.942857142857143,0.971428571428572,1.),.UNSPECIFIED.)
CURVE()
GEOMETRIC_REPRESENTATION_ITEM()
RATIONAL_B_SPLINE_CURVE((1.,1.,1.,1.,1.,1.,1.,1.,1.,1.,1.,1.,1.,1.,1.,1.,
1.,1.,1.,1.,1.,1.,1.,1.,1.,1.))
REPRESENTATION_ITEM('')
);
#776=(
BOUNDED_CURVE()
B_SPLINE_CURVE(5,(#52818,#52819,#52820,#52821,#52822,#52823,#52824,#52825,
#52826,#52827,#52828,#52829,#52830,#52831,#52832,#52833,#52834,#52835,#52836,
#52837,#52838,#52839,#52840,#52841,#52842,#52843,#52844,#52845,#52846),
 .UNSPECIFIED.,.F.,.F.)
B_SPLINE_CURVE_WITH_KNOTS((6,1,1,1,1,1,1,1,1,1,1,1,1,1,1,1,1,1,1,1,1,1,
1,1,6),(0.,0.0285714285714286,0.0571428571428571,0.0857142857142857,0.114285714285714,
0.142857142857143,0.171428571428571,0.2,0.228571428571429,0.257142857142857,
0.285714285714286,0.314285714285714,0.342857142857143,0.371428571428571,
0.4,0.428571428571429,0.457142857142857,0.485714285714286,0.514285714285714,
0.542857142857143,0.571428571428572,0.6,0.628571428571429,0.657142857142857,
0.670627588953113),.UNSPECIFIED.)
CURVE()
GEOMETRIC_REPRESENTATION_ITEM()
RATIONAL_B_SPLINE_CURVE((1.,1.,1.,1.,1.,1.,1.,1.,1.,1.,1.,1.,1.,1.,1.,1.,
1.,1.,1.,1.,1.,1.,1.,1.,1.,1.,1.,1.,1.))
REPRESENTATION_ITEM('')
);
#777=(
BOUNDED_CURVE()
B_SPLINE_CURVE(5,(#52850,#52851,#52852,#52853,#52854,#52855,#52856,#52857,
#52858,#52859,#52860,#52861,#52862,#52863,#52864,#52865,#52866,#52867,#52868,
#52869,#52870,#52871,#52872,#52873,#52874,#52875),.UNSPECIFIED.,.F.,.F.)
B_SPLINE_CURVE_WITH_KNOTS((6,1,1,1,1,1,1,1,1,1,1,1,1,1,1,1,1,1,1,1,1,6),
(0.428061295609925,0.428571428571429,0.457142857142857,0.485714285714286,
0.514285714285714,0.542857142857143,0.571428571428572,0.6,0.628571428571429,
0.657142857142857,0.685714285714286,0.714285714285714,0.742857142857143,
0.771428571428572,0.8,0.828571428571429,0.857142857142857,0.885714285714286,
0.914285714285714,0.942857142857143,0.971428571428572,1.),.UNSPECIFIED.)
CURVE()
GEOMETRIC_REPRESENTATION_ITEM()
RATIONAL_B_SPLINE_CURVE((1.,1.,1.,1.,1.,1.,1.,1.,1.,1.,1.,1.,1.,1.,1.,1.,
1.,1.,1.,1.,1.,1.,1.,1.,1.,1.))
REPRESENTATION_ITEM('')
);
#778=(
BOUNDED_CURVE()
B_SPLINE_CURVE(5,(#52879,#52880,#52881,#52882,#52883,#52884,#52885,#52886,
#52887,#52888,#52889,#52890,#52891,#52892,#52893,#52894,#52895,#52896,#52897,
#52898,#52899,#52900,#52901,#52902,#52903,#52904,#52905,#52906,#52907),
 .UNSPECIFIED.,.F.,.F.)
B_SPLINE_CURVE_WITH_KNOTS((6,1,1,1,1,1,1,1,1,1,1,1,1,1,1,1,1,1,1,1,1,1,
1,1,6),(0.,0.0285714285714286,0.0571428571428571,0.0857142857142857,0.114285714285714,
0.142857142857143,0.171428571428571,0.2,0.228571428571429,0.257142857142857,
0.285714285714286,0.314285714285714,0.342857142857143,0.371428571428571,
0.4,0.428571428571429,0.457142857142857,0.485714285714286,0.514285714285714,
0.542857142857143,0.571428571428572,0.6,0.628571428571429,0.657142857142857,
0.670627588953112),.UNSPECIFIED.)
CURVE()
GEOMETRIC_REPRESENTATION_ITEM()
RATIONAL_B_SPLINE_CURVE((1.,1.,1.,1.,1.,1.,1.,1.,1.,1.,1.,1.,1.,1.,1.,1.,
1.,1.,1.,1.,1.,1.,1.,1.,1.,1.,1.,1.,1.))
REPRESENTATION_ITEM('')
);
#779=(
BOUNDED_CURVE()
B_SPLINE_CURVE(5,(#52911,#52912,#52913,#52914,#52915,#52916,#52917,#52918,
#52919,#52920,#52921,#52922,#52923,#52924,#52925,#52926,#52927,#52928,#52929,
#52930,#52931,#52932,#52933,#52934,#52935,#52936),.UNSPECIFIED.,.F.,.F.)
B_SPLINE_CURVE_WITH_KNOTS((6,1,1,1,1,1,1,1,1,1,1,1,1,1,1,1,1,1,1,1,1,6),
(0.428061295609926,0.428571428571429,0.457142857142857,0.485714285714286,
0.514285714285714,0.542857142857143,0.571428571428572,0.6,0.628571428571429,
0.657142857142857,0.685714285714286,0.714285714285714,0.742857142857143,
0.771428571428572,0.8,0.828571428571429,0.857142857142857,0.885714285714286,
0.914285714285714,0.942857142857143,0.971428571428572,1.),.UNSPECIFIED.)
CURVE()
GEOMETRIC_REPRESENTATION_ITEM()
RATIONAL_B_SPLINE_CURVE((1.,1.,1.,1.,1.,1.,1.,1.,1.,1.,1.,1.,1.,1.,1.,1.,
1.,1.,1.,1.,1.,1.,1.,1.,1.,1.))
REPRESENTATION_ITEM('')
);
#780=(
BOUNDED_CURVE()
B_SPLINE_CURVE(5,(#52940,#52941,#52942,#52943,#52944,#52945,#52946,#52947,
#52948,#52949,#52950,#52951,#52952,#52953,#52954,#52955,#52956,#52957,#52958,
#52959,#52960,#52961,#52962,#52963,#52964,#52965,#52966,#52967,#52968),
 .UNSPECIFIED.,.F.,.F.)
B_SPLINE_CURVE_WITH_KNOTS((6,1,1,1,1,1,1,1,1,1,1,1,1,1,1,1,1,1,1,1,1,1,
1,1,6),(0.,0.0285714285714286,0.0571428571428571,0.0857142857142857,0.114285714285714,
0.142857142857143,0.171428571428571,0.2,0.228571428571429,0.257142857142857,
0.285714285714286,0.314285714285714,0.342857142857143,0.371428571428571,
0.4,0.428571428571429,0.457142857142857,0.485714285714286,0.514285714285714,
0.542857142857143,0.571428571428572,0.6,0.628571428571429,0.657142857142857,
0.670627588953112),.UNSPECIFIED.)
CURVE()
GEOMETRIC_REPRESENTATION_ITEM()
RATIONAL_B_SPLINE_CURVE((1.,1.,1.,1.,1.,1.,1.,1.,1.,1.,1.,1.,1.,1.,1.,1.,
1.,1.,1.,1.,1.,1.,1.,1.,1.,1.,1.,1.,1.))
REPRESENTATION_ITEM('')
);
#781=(
BOUNDED_CURVE()
B_SPLINE_CURVE(5,(#52972,#52973,#52974,#52975,#52976,#52977,#52978,#52979,
#52980,#52981,#52982,#52983,#52984,#52985,#52986,#52987,#52988,#52989,#52990,
#52991,#52992,#52993,#52994,#52995,#52996,#52997),.UNSPECIFIED.,.F.,.F.)
B_SPLINE_CURVE_WITH_KNOTS((6,1,1,1,1,1,1,1,1,1,1,1,1,1,1,1,1,1,1,1,1,6),
(0.428061295609926,0.428571428571429,0.457142857142857,0.485714285714286,
0.514285714285714,0.542857142857143,0.571428571428572,0.6,0.628571428571429,
0.657142857142857,0.685714285714286,0.714285714285714,0.742857142857143,
0.771428571428572,0.8,0.828571428571429,0.857142857142857,0.885714285714286,
0.914285714285714,0.942857142857143,0.971428571428572,1.),.UNSPECIFIED.)
CURVE()
GEOMETRIC_REPRESENTATION_ITEM()
RATIONAL_B_SPLINE_CURVE((1.,1.,1.,1.,1.,1.,1.,1.,1.,1.,1.,1.,1.,1.,1.,1.,
1.,1.,1.,1.,1.,1.,1.,1.,1.,1.))
REPRESENTATION_ITEM('')
);
#782=(
BOUNDED_CURVE()
B_SPLINE_CURVE(5,(#53001,#53002,#53003,#53004,#53005,#53006,#53007,#53008,
#53009,#53010,#53011,#53012,#53013,#53014,#53015,#53016,#53017,#53018,#53019,
#53020,#53021,#53022,#53023,#53024,#53025,#53026,#53027,#53028,#53029),
 .UNSPECIFIED.,.F.,.F.)
B_SPLINE_CURVE_WITH_KNOTS((6,1,1,1,1,1,1,1,1,1,1,1,1,1,1,1,1,1,1,1,1,1,
1,1,6),(0.,0.0285714285714286,0.0571428571428571,0.0857142857142857,0.114285714285714,
0.142857142857143,0.171428571428571,0.2,0.228571428571429,0.257142857142857,
0.285714285714286,0.314285714285714,0.342857142857143,0.371428571428571,
0.4,0.428571428571429,0.457142857142857,0.485714285714286,0.514285714285714,
0.542857142857143,0.571428571428572,0.6,0.628571428571429,0.657142857142857,
0.670627588953112),.UNSPECIFIED.)
CURVE()
GEOMETRIC_REPRESENTATION_ITEM()
RATIONAL_B_SPLINE_CURVE((1.,1.,1.,1.,1.,1.,1.,1.,1.,1.,1.,1.,1.,1.,1.,1.,
1.,1.,1.,1.,1.,1.,1.,1.,1.,1.,1.,1.,1.))
REPRESENTATION_ITEM('')
);
#783=(
BOUNDED_CURVE()
B_SPLINE_CURVE(5,(#53033,#53034,#53035,#53036,#53037,#53038,#53039,#53040,
#53041,#53042,#53043,#53044,#53045,#53046,#53047,#53048,#53049,#53050,#53051,
#53052,#53053,#53054,#53055,#53056,#53057,#53058),.UNSPECIFIED.,.F.,.F.)
B_SPLINE_CURVE_WITH_KNOTS((6,1,1,1,1,1,1,1,1,1,1,1,1,1,1,1,1,1,1,1,1,6),
(0.428061295609926,0.428571428571429,0.457142857142857,0.485714285714286,
0.514285714285714,0.542857142857143,0.571428571428572,0.6,0.628571428571429,
0.657142857142857,0.685714285714286,0.714285714285714,0.742857142857143,
0.771428571428572,0.8,0.828571428571429,0.857142857142857,0.885714285714286,
0.914285714285714,0.942857142857143,0.971428571428572,1.),.UNSPECIFIED.)
CURVE()
GEOMETRIC_REPRESENTATION_ITEM()
RATIONAL_B_SPLINE_CURVE((1.,1.,1.,1.,1.,1.,1.,1.,1.,1.,1.,1.,1.,1.,1.,1.,
1.,1.,1.,1.,1.,1.,1.,1.,1.,1.))
REPRESENTATION_ITEM('')
);
#784=(
BOUNDED_CURVE()
B_SPLINE_CURVE(5,(#53062,#53063,#53064,#53065,#53066,#53067,#53068,#53069,
#53070,#53071,#53072,#53073,#53074,#53075,#53076,#53077,#53078,#53079,#53080,
#53081,#53082,#53083,#53084,#53085,#53086,#53087,#53088,#53089,#53090),
 .UNSPECIFIED.,.F.,.F.)
B_SPLINE_CURVE_WITH_KNOTS((6,1,1,1,1,1,1,1,1,1,1,1,1,1,1,1,1,1,1,1,1,1,
1,1,6),(0.,0.0285714285714286,0.0571428571428571,0.0857142857142857,0.114285714285714,
0.142857142857143,0.171428571428571,0.2,0.228571428571429,0.257142857142857,
0.285714285714286,0.314285714285714,0.342857142857143,0.371428571428571,
0.4,0.428571428571429,0.457142857142857,0.485714285714286,0.514285714285714,
0.542857142857143,0.571428571428572,0.6,0.628571428571429,0.657142857142857,
0.670627588953113),.UNSPECIFIED.)
CURVE()
GEOMETRIC_REPRESENTATION_ITEM()
RATIONAL_B_SPLINE_CURVE((1.,1.,1.,1.,1.,1.,1.,1.,1.,1.,1.,1.,1.,1.,1.,1.,
1.,1.,1.,1.,1.,1.,1.,1.,1.,1.,1.,1.,1.))
REPRESENTATION_ITEM('')
);
#785=(
BOUNDED_CURVE()
B_SPLINE_CURVE(5,(#53094,#53095,#53096,#53097,#53098,#53099,#53100,#53101,
#53102,#53103,#53104,#53105,#53106,#53107,#53108,#53109,#53110,#53111,#53112,
#53113,#53114,#53115,#53116,#53117,#53118,#53119),.UNSPECIFIED.,.F.,.F.)
B_SPLINE_CURVE_WITH_KNOTS((6,1,1,1,1,1,1,1,1,1,1,1,1,1,1,1,1,1,1,1,1,6),
(0.428061295609926,0.428571428571429,0.457142857142857,0.485714285714286,
0.514285714285714,0.542857142857143,0.571428571428572,0.6,0.628571428571429,
0.657142857142857,0.685714285714286,0.714285714285714,0.742857142857143,
0.771428571428572,0.8,0.828571428571429,0.857142857142857,0.885714285714286,
0.914285714285714,0.942857142857143,0.971428571428572,1.),.UNSPECIFIED.)
CURVE()
GEOMETRIC_REPRESENTATION_ITEM()
RATIONAL_B_SPLINE_CURVE((1.,1.,1.,1.,1.,1.,1.,1.,1.,1.,1.,1.,1.,1.,1.,1.,
1.,1.,1.,1.,1.,1.,1.,1.,1.,1.))
REPRESENTATION_ITEM('')
);
#786=(
BOUNDED_CURVE()
B_SPLINE_CURVE(5,(#53123,#53124,#53125,#53126,#53127,#53128,#53129,#53130,
#53131,#53132,#53133,#53134,#53135,#53136,#53137,#53138,#53139,#53140,#53141,
#53142,#53143,#53144,#53145,#53146,#53147,#53148,#53149,#53150,#53151),
 .UNSPECIFIED.,.F.,.F.)
B_SPLINE_CURVE_WITH_KNOTS((6,1,1,1,1,1,1,1,1,1,1,1,1,1,1,1,1,1,1,1,1,1,
1,1,6),(0.,0.0285714285714286,0.0571428571428571,0.0857142857142857,0.114285714285714,
0.142857142857143,0.171428571428571,0.2,0.228571428571429,0.257142857142857,
0.285714285714286,0.314285714285714,0.342857142857143,0.371428571428571,
0.4,0.428571428571429,0.457142857142857,0.485714285714286,0.514285714285714,
0.542857142857143,0.571428571428572,0.6,0.628571428571429,0.657142857142857,
0.670627588953111),.UNSPECIFIED.)
CURVE()
GEOMETRIC_REPRESENTATION_ITEM()
RATIONAL_B_SPLINE_CURVE((1.,1.,1.,1.,1.,1.,1.,1.,1.,1.,1.,1.,1.,1.,1.,1.,
1.,1.,1.,1.,1.,1.,1.,1.,1.,1.,1.,1.,1.))
REPRESENTATION_ITEM('')
);
#787=(
BOUNDED_CURVE()
B_SPLINE_CURVE(5,(#53155,#53156,#53157,#53158,#53159,#53160,#53161,#53162,
#53163,#53164,#53165,#53166,#53167,#53168,#53169,#53170,#53171,#53172,#53173,
#53174,#53175,#53176,#53177,#53178,#53179,#53180),.UNSPECIFIED.,.F.,.F.)
B_SPLINE_CURVE_WITH_KNOTS((6,1,1,1,1,1,1,1,1,1,1,1,1,1,1,1,1,1,1,1,1,6),
(0.428061295609925,0.428571428571429,0.457142857142857,0.485714285714286,
0.514285714285714,0.542857142857143,0.571428571428572,0.6,0.628571428571429,
0.657142857142857,0.685714285714286,0.714285714285714,0.742857142857143,
0.771428571428572,0.8,0.828571428571429,0.857142857142857,0.885714285714286,
0.914285714285714,0.942857142857143,0.971428571428572,1.),.UNSPECIFIED.)
CURVE()
GEOMETRIC_REPRESENTATION_ITEM()
RATIONAL_B_SPLINE_CURVE((1.,1.,1.,1.,1.,1.,1.,1.,1.,1.,1.,1.,1.,1.,1.,1.,
1.,1.,1.,1.,1.,1.,1.,1.,1.,1.))
REPRESENTATION_ITEM('')
);
#788=(
BOUNDED_CURVE()
B_SPLINE_CURVE(5,(#53184,#53185,#53186,#53187,#53188,#53189,#53190,#53191,
#53192,#53193,#53194,#53195,#53196,#53197,#53198,#53199,#53200,#53201,#53202,
#53203,#53204,#53205,#53206,#53207,#53208,#53209,#53210,#53211,#53212),
 .UNSPECIFIED.,.F.,.F.)
B_SPLINE_CURVE_WITH_KNOTS((6,1,1,1,1,1,1,1,1,1,1,1,1,1,1,1,1,1,1,1,1,1,
1,1,6),(0.,0.0285714285714286,0.0571428571428571,0.0857142857142857,0.114285714285714,
0.142857142857143,0.171428571428571,0.2,0.228571428571429,0.257142857142857,
0.285714285714286,0.314285714285714,0.342857142857143,0.371428571428571,
0.4,0.428571428571429,0.457142857142857,0.485714285714286,0.514285714285714,
0.542857142857143,0.571428571428572,0.6,0.628571428571429,0.657142857142857,
0.670627588953113),.UNSPECIFIED.)
CURVE()
GEOMETRIC_REPRESENTATION_ITEM()
RATIONAL_B_SPLINE_CURVE((1.,1.,1.,1.,1.,1.,1.,1.,1.,1.,1.,1.,1.,1.,1.,1.,
1.,1.,1.,1.,1.,1.,1.,1.,1.,1.,1.,1.,1.))
REPRESENTATION_ITEM('')
);
#789=(
BOUNDED_CURVE()
B_SPLINE_CURVE(5,(#53216,#53217,#53218,#53219,#53220,#53221,#53222,#53223,
#53224,#53225,#53226,#53227,#53228,#53229,#53230,#53231,#53232,#53233,#53234,
#53235,#53236,#53237,#53238,#53239,#53240,#53241),.UNSPECIFIED.,.F.,.F.)
B_SPLINE_CURVE_WITH_KNOTS((6,1,1,1,1,1,1,1,1,1,1,1,1,1,1,1,1,1,1,1,1,6),
(0.428061295609926,0.428571428571429,0.457142857142857,0.485714285714286,
0.514285714285714,0.542857142857143,0.571428571428572,0.6,0.628571428571429,
0.657142857142857,0.685714285714286,0.714285714285714,0.742857142857143,
0.771428571428572,0.8,0.828571428571429,0.857142857142857,0.885714285714286,
0.914285714285714,0.942857142857143,0.971428571428572,1.),.UNSPECIFIED.)
CURVE()
GEOMETRIC_REPRESENTATION_ITEM()
RATIONAL_B_SPLINE_CURVE((1.,1.,1.,1.,1.,1.,1.,1.,1.,1.,1.,1.,1.,1.,1.,1.,
1.,1.,1.,1.,1.,1.,1.,1.,1.,1.))
REPRESENTATION_ITEM('')
);
#790=(
BOUNDED_CURVE()
B_SPLINE_CURVE(5,(#53245,#53246,#53247,#53248,#53249,#53250,#53251,#53252,
#53253,#53254,#53255,#53256,#53257,#53258,#53259,#53260,#53261,#53262,#53263,
#53264,#53265,#53266,#53267,#53268,#53269,#53270,#53271,#53272,#53273),
 .UNSPECIFIED.,.F.,.F.)
B_SPLINE_CURVE_WITH_KNOTS((6,1,1,1,1,1,1,1,1,1,1,1,1,1,1,1,1,1,1,1,1,1,
1,1,6),(0.,0.0285714285714286,0.0571428571428571,0.0857142857142857,0.114285714285714,
0.142857142857143,0.171428571428571,0.2,0.228571428571429,0.257142857142857,
0.285714285714286,0.314285714285714,0.342857142857143,0.371428571428571,
0.4,0.428571428571429,0.457142857142857,0.485714285714286,0.514285714285714,
0.542857142857143,0.571428571428572,0.6,0.628571428571429,0.657142857142857,
0.670627588953113),.UNSPECIFIED.)
CURVE()
GEOMETRIC_REPRESENTATION_ITEM()
RATIONAL_B_SPLINE_CURVE((1.,1.,1.,1.,1.,1.,1.,1.,1.,1.,1.,1.,1.,1.,1.,1.,
1.,1.,1.,1.,1.,1.,1.,1.,1.,1.,1.,1.,1.))
REPRESENTATION_ITEM('')
);
#791=(
BOUNDED_CURVE()
B_SPLINE_CURVE(5,(#53277,#53278,#53279,#53280,#53281,#53282,#53283,#53284,
#53285,#53286,#53287,#53288,#53289,#53290,#53291,#53292,#53293,#53294,#53295,
#53296,#53297,#53298,#53299,#53300,#53301,#53302),.UNSPECIFIED.,.F.,.F.)
B_SPLINE_CURVE_WITH_KNOTS((6,1,1,1,1,1,1,1,1,1,1,1,1,1,1,1,1,1,1,1,1,6),
(0.428061295609925,0.428571428571429,0.457142857142857,0.485714285714286,
0.514285714285714,0.542857142857143,0.571428571428572,0.6,0.628571428571429,
0.657142857142857,0.685714285714286,0.714285714285714,0.742857142857143,
0.771428571428572,0.8,0.828571428571429,0.857142857142857,0.885714285714286,
0.914285714285714,0.942857142857143,0.971428571428572,1.),.UNSPECIFIED.)
CURVE()
GEOMETRIC_REPRESENTATION_ITEM()
RATIONAL_B_SPLINE_CURVE((1.,1.,1.,1.,1.,1.,1.,1.,1.,1.,1.,1.,1.,1.,1.,1.,
1.,1.,1.,1.,1.,1.,1.,1.,1.,1.))
REPRESENTATION_ITEM('')
);
#792=(
BOUNDED_CURVE()
B_SPLINE_CURVE(5,(#53306,#53307,#53308,#53309,#53310,#53311,#53312,#53313,
#53314,#53315,#53316,#53317,#53318,#53319,#53320,#53321,#53322,#53323,#53324,
#53325,#53326,#53327,#53328,#53329,#53330,#53331,#53332,#53333,#53334),
 .UNSPECIFIED.,.F.,.F.)
B_SPLINE_CURVE_WITH_KNOTS((6,1,1,1,1,1,1,1,1,1,1,1,1,1,1,1,1,1,1,1,1,1,
1,1,6),(0.,0.0285714285714286,0.0571428571428571,0.0857142857142857,0.114285714285714,
0.142857142857143,0.171428571428571,0.2,0.228571428571429,0.257142857142857,
0.285714285714286,0.314285714285714,0.342857142857143,0.371428571428571,
0.4,0.428571428571429,0.457142857142857,0.485714285714286,0.514285714285714,
0.542857142857143,0.571428571428572,0.6,0.628571428571429,0.657142857142857,
0.670627588953112),.UNSPECIFIED.)
CURVE()
GEOMETRIC_REPRESENTATION_ITEM()
RATIONAL_B_SPLINE_CURVE((1.,1.,1.,1.,1.,1.,1.,1.,1.,1.,1.,1.,1.,1.,1.,1.,
1.,1.,1.,1.,1.,1.,1.,1.,1.,1.,1.,1.,1.))
REPRESENTATION_ITEM('')
);
#793=(
BOUNDED_CURVE()
B_SPLINE_CURVE(5,(#53338,#53339,#53340,#53341,#53342,#53343,#53344,#53345,
#53346,#53347,#53348,#53349,#53350,#53351,#53352,#53353,#53354,#53355,#53356,
#53357,#53358,#53359,#53360,#53361,#53362,#53363),.UNSPECIFIED.,.F.,.F.)
B_SPLINE_CURVE_WITH_KNOTS((6,1,1,1,1,1,1,1,1,1,1,1,1,1,1,1,1,1,1,1,1,6),
(0.428061295609925,0.428571428571429,0.457142857142857,0.485714285714286,
0.514285714285714,0.542857142857143,0.571428571428572,0.6,0.628571428571429,
0.657142857142857,0.685714285714286,0.714285714285714,0.742857142857143,
0.771428571428572,0.8,0.828571428571429,0.857142857142857,0.885714285714286,
0.914285714285714,0.942857142857143,0.971428571428572,1.),.UNSPECIFIED.)
CURVE()
GEOMETRIC_REPRESENTATION_ITEM()
RATIONAL_B_SPLINE_CURVE((1.,1.,1.,1.,1.,1.,1.,1.,1.,1.,1.,1.,1.,1.,1.,1.,
1.,1.,1.,1.,1.,1.,1.,1.,1.,1.))
REPRESENTATION_ITEM('')
);
#794=(
BOUNDED_CURVE()
B_SPLINE_CURVE(5,(#53367,#53368,#53369,#53370,#53371,#53372,#53373,#53374,
#53375,#53376,#53377,#53378,#53379,#53380,#53381,#53382,#53383,#53384,#53385,
#53386,#53387,#53388,#53389,#53390,#53391,#53392,#53393,#53394,#53395),
 .UNSPECIFIED.,.F.,.F.)
B_SPLINE_CURVE_WITH_KNOTS((6,1,1,1,1,1,1,1,1,1,1,1,1,1,1,1,1,1,1,1,1,1,
1,1,6),(0.,0.0285714285714286,0.0571428571428571,0.0857142857142857,0.114285714285714,
0.142857142857143,0.171428571428571,0.2,0.228571428571429,0.257142857142857,
0.285714285714286,0.314285714285714,0.342857142857143,0.371428571428571,
0.4,0.428571428571429,0.457142857142857,0.485714285714286,0.514285714285714,
0.542857142857143,0.571428571428572,0.6,0.628571428571429,0.657142857142857,
0.670627588953112),.UNSPECIFIED.)
CURVE()
GEOMETRIC_REPRESENTATION_ITEM()
RATIONAL_B_SPLINE_CURVE((1.,1.,1.,1.,1.,1.,1.,1.,1.,1.,1.,1.,1.,1.,1.,1.,
1.,1.,1.,1.,1.,1.,1.,1.,1.,1.,1.,1.,1.))
REPRESENTATION_ITEM('')
);
#795=(
BOUNDED_CURVE()
B_SPLINE_CURVE(5,(#53399,#53400,#53401,#53402,#53403,#53404,#53405,#53406,
#53407,#53408,#53409,#53410,#53411,#53412,#53413,#53414,#53415,#53416,#53417,
#53418,#53419,#53420,#53421,#53422,#53423,#53424),.UNSPECIFIED.,.F.,.F.)
B_SPLINE_CURVE_WITH_KNOTS((6,1,1,1,1,1,1,1,1,1,1,1,1,1,1,1,1,1,1,1,1,6),
(0.428061295609926,0.428571428571429,0.457142857142857,0.485714285714286,
0.514285714285714,0.542857142857143,0.571428571428572,0.6,0.628571428571429,
0.657142857142857,0.685714285714286,0.714285714285714,0.742857142857143,
0.771428571428572,0.8,0.828571428571429,0.857142857142857,0.885714285714286,
0.914285714285714,0.942857142857143,0.971428571428572,1.),.UNSPECIFIED.)
CURVE()
GEOMETRIC_REPRESENTATION_ITEM()
RATIONAL_B_SPLINE_CURVE((1.,1.,1.,1.,1.,1.,1.,1.,1.,1.,1.,1.,1.,1.,1.,1.,
1.,1.,1.,1.,1.,1.,1.,1.,1.,1.))
REPRESENTATION_ITEM('')
);
#796=(
BOUNDED_CURVE()
B_SPLINE_CURVE(5,(#53428,#53429,#53430,#53431,#53432,#53433,#53434,#53435,
#53436,#53437,#53438,#53439,#53440,#53441,#53442,#53443,#53444,#53445,#53446,
#53447,#53448,#53449,#53450,#53451,#53452,#53453,#53454,#53455,#53456),
 .UNSPECIFIED.,.F.,.F.)
B_SPLINE_CURVE_WITH_KNOTS((6,1,1,1,1,1,1,1,1,1,1,1,1,1,1,1,1,1,1,1,1,1,
1,1,6),(0.,0.0285714285714286,0.0571428571428571,0.0857142857142857,0.114285714285714,
0.142857142857143,0.171428571428571,0.2,0.228571428571429,0.257142857142857,
0.285714285714286,0.314285714285714,0.342857142857143,0.371428571428571,
0.4,0.428571428571429,0.457142857142857,0.485714285714286,0.514285714285714,
0.542857142857143,0.571428571428572,0.6,0.628571428571429,0.657142857142857,
0.670627588953112),.UNSPECIFIED.)
CURVE()
GEOMETRIC_REPRESENTATION_ITEM()
RATIONAL_B_SPLINE_CURVE((1.,1.,1.,1.,1.,1.,1.,1.,1.,1.,1.,1.,1.,1.,1.,1.,
1.,1.,1.,1.,1.,1.,1.,1.,1.,1.,1.,1.,1.))
REPRESENTATION_ITEM('')
);
#797=(
BOUNDED_CURVE()
B_SPLINE_CURVE(5,(#53460,#53461,#53462,#53463,#53464,#53465,#53466,#53467,
#53468,#53469,#53470,#53471,#53472,#53473,#53474,#53475,#53476,#53477,#53478,
#53479,#53480,#53481,#53482,#53483,#53484,#53485),.UNSPECIFIED.,.F.,.F.)
B_SPLINE_CURVE_WITH_KNOTS((6,1,1,1,1,1,1,1,1,1,1,1,1,1,1,1,1,1,1,1,1,6),
(0.428061295609926,0.428571428571429,0.457142857142857,0.485714285714286,
0.514285714285714,0.542857142857143,0.571428571428572,0.6,0.628571428571429,
0.657142857142857,0.685714285714286,0.714285714285714,0.742857142857143,
0.771428571428572,0.8,0.828571428571429,0.857142857142857,0.885714285714286,
0.914285714285714,0.942857142857143,0.971428571428572,1.),.UNSPECIFIED.)
CURVE()
GEOMETRIC_REPRESENTATION_ITEM()
RATIONAL_B_SPLINE_CURVE((1.,1.,1.,1.,1.,1.,1.,1.,1.,1.,1.,1.,1.,1.,1.,1.,
1.,1.,1.,1.,1.,1.,1.,1.,1.,1.))
REPRESENTATION_ITEM('')
);
#798=(
BOUNDED_CURVE()
B_SPLINE_CURVE(5,(#53489,#53490,#53491,#53492,#53493,#53494,#53495,#53496,
#53497,#53498,#53499,#53500,#53501,#53502,#53503,#53504,#53505,#53506,#53507,
#53508,#53509,#53510,#53511,#53512,#53513,#53514,#53515,#53516,#53517),
 .UNSPECIFIED.,.F.,.F.)
B_SPLINE_CURVE_WITH_KNOTS((6,1,1,1,1,1,1,1,1,1,1,1,1,1,1,1,1,1,1,1,1,1,
1,1,6),(0.,0.0285714285714286,0.0571428571428571,0.0857142857142857,0.114285714285714,
0.142857142857143,0.171428571428571,0.2,0.228571428571429,0.257142857142857,
0.285714285714286,0.314285714285714,0.342857142857143,0.371428571428571,
0.4,0.428571428571429,0.457142857142857,0.485714285714286,0.514285714285714,
0.542857142857143,0.571428571428572,0.6,0.628571428571429,0.657142857142857,
0.670627588953113),.UNSPECIFIED.)
CURVE()
GEOMETRIC_REPRESENTATION_ITEM()
RATIONAL_B_SPLINE_CURVE((1.,1.,1.,1.,1.,1.,1.,1.,1.,1.,1.,1.,1.,1.,1.,1.,
1.,1.,1.,1.,1.,1.,1.,1.,1.,1.,1.,1.,1.))
REPRESENTATION_ITEM('')
);
#799=(
BOUNDED_CURVE()
B_SPLINE_CURVE(5,(#53521,#53522,#53523,#53524,#53525,#53526,#53527,#53528,
#53529,#53530,#53531,#53532,#53533,#53534,#53535,#53536,#53537,#53538,#53539,
#53540,#53541,#53542,#53543,#53544,#53545,#53546),.UNSPECIFIED.,.F.,.F.)
B_SPLINE_CURVE_WITH_KNOTS((6,1,1,1,1,1,1,1,1,1,1,1,1,1,1,1,1,1,1,1,1,6),
(0.428061295609925,0.428571428571429,0.457142857142857,0.485714285714286,
0.514285714285714,0.542857142857143,0.571428571428572,0.6,0.628571428571429,
0.657142857142857,0.685714285714286,0.714285714285714,0.742857142857143,
0.771428571428572,0.8,0.828571428571429,0.857142857142857,0.885714285714286,
0.914285714285714,0.942857142857143,0.971428571428572,1.),.UNSPECIFIED.)
CURVE()
GEOMETRIC_REPRESENTATION_ITEM()
RATIONAL_B_SPLINE_CURVE((1.,1.,1.,1.,1.,1.,1.,1.,1.,1.,1.,1.,1.,1.,1.,1.,
1.,1.,1.,1.,1.,1.,1.,1.,1.,1.))
REPRESENTATION_ITEM('')
);
#800=(
BOUNDED_CURVE()
B_SPLINE_CURVE(5,(#53550,#53551,#53552,#53553,#53554,#53555,#53556,#53557,
#53558,#53559,#53560,#53561,#53562,#53563,#53564,#53565,#53566,#53567,#53568,
#53569,#53570,#53571,#53572,#53573,#53574,#53575,#53576,#53577,#53578),
 .UNSPECIFIED.,.F.,.F.)
B_SPLINE_CURVE_WITH_KNOTS((6,1,1,1,1,1,1,1,1,1,1,1,1,1,1,1,1,1,1,1,1,1,
1,1,6),(0.,0.0285714285714286,0.0571428571428571,0.0857142857142857,0.114285714285714,
0.142857142857143,0.171428571428571,0.2,0.228571428571429,0.257142857142857,
0.285714285714286,0.314285714285714,0.342857142857143,0.371428571428571,
0.4,0.428571428571429,0.457142857142857,0.485714285714286,0.514285714285714,
0.542857142857143,0.571428571428572,0.6,0.628571428571429,0.657142857142857,
0.670627588953112),.UNSPECIFIED.)
CURVE()
GEOMETRIC_REPRESENTATION_ITEM()
RATIONAL_B_SPLINE_CURVE((1.,1.,1.,1.,1.,1.,1.,1.,1.,1.,1.,1.,1.,1.,1.,1.,
1.,1.,1.,1.,1.,1.,1.,1.,1.,1.,1.,1.,1.))
REPRESENTATION_ITEM('')
);
#801=(
BOUNDED_CURVE()
B_SPLINE_CURVE(5,(#53582,#53583,#53584,#53585,#53586,#53587,#53588,#53589,
#53590,#53591,#53592,#53593,#53594,#53595,#53596,#53597,#53598,#53599,#53600,
#53601,#53602,#53603,#53604,#53605,#53606,#53607),.UNSPECIFIED.,.F.,.F.)
B_SPLINE_CURVE_WITH_KNOTS((6,1,1,1,1,1,1,1,1,1,1,1,1,1,1,1,1,1,1,1,1,6),
(0.428061295609926,0.428571428571429,0.457142857142857,0.485714285714286,
0.514285714285714,0.542857142857143,0.571428571428572,0.6,0.628571428571429,
0.657142857142857,0.685714285714286,0.714285714285714,0.742857142857143,
0.771428571428572,0.8,0.828571428571429,0.857142857142857,0.885714285714286,
0.914285714285714,0.942857142857143,0.971428571428572,1.),.UNSPECIFIED.)
CURVE()
GEOMETRIC_REPRESENTATION_ITEM()
RATIONAL_B_SPLINE_CURVE((1.,1.,1.,1.,1.,1.,1.,1.,1.,1.,1.,1.,1.,1.,1.,1.,
1.,1.,1.,1.,1.,1.,1.,1.,1.,1.))
REPRESENTATION_ITEM('')
);
#802=(
BOUNDED_CURVE()
B_SPLINE_CURVE(5,(#53611,#53612,#53613,#53614,#53615,#53616,#53617,#53618,
#53619,#53620,#53621,#53622,#53623,#53624,#53625,#53626,#53627,#53628,#53629,
#53630,#53631,#53632,#53633,#53634,#53635,#53636,#53637,#53638,#53639),
 .UNSPECIFIED.,.F.,.F.)
B_SPLINE_CURVE_WITH_KNOTS((6,1,1,1,1,1,1,1,1,1,1,1,1,1,1,1,1,1,1,1,1,1,
1,1,6),(0.,0.0285714285714286,0.0571428571428571,0.0857142857142857,0.114285714285714,
0.142857142857143,0.171428571428571,0.2,0.228571428571429,0.257142857142857,
0.285714285714286,0.314285714285714,0.342857142857143,0.371428571428571,
0.4,0.428571428571429,0.457142857142857,0.485714285714286,0.514285714285714,
0.542857142857143,0.571428571428572,0.6,0.628571428571429,0.657142857142857,
0.670627588953112),.UNSPECIFIED.)
CURVE()
GEOMETRIC_REPRESENTATION_ITEM()
RATIONAL_B_SPLINE_CURVE((1.,1.,1.,1.,1.,1.,1.,1.,1.,1.,1.,1.,1.,1.,1.,1.,
1.,1.,1.,1.,1.,1.,1.,1.,1.,1.,1.,1.,1.))
REPRESENTATION_ITEM('')
);
#803=(
BOUNDED_CURVE()
B_SPLINE_CURVE(5,(#53643,#53644,#53645,#53646,#53647,#53648,#53649,#53650,
#53651,#53652,#53653,#53654,#53655,#53656,#53657,#53658,#53659,#53660,#53661,
#53662,#53663,#53664,#53665,#53666,#53667,#53668),.UNSPECIFIED.,.F.,.F.)
B_SPLINE_CURVE_WITH_KNOTS((6,1,1,1,1,1,1,1,1,1,1,1,1,1,1,1,1,1,1,1,1,6),
(0.428061295609926,0.428571428571429,0.457142857142857,0.485714285714286,
0.514285714285714,0.542857142857143,0.571428571428572,0.6,0.628571428571429,
0.657142857142857,0.685714285714286,0.714285714285714,0.742857142857143,
0.771428571428572,0.8,0.828571428571429,0.857142857142857,0.885714285714286,
0.914285714285714,0.942857142857143,0.971428571428572,1.),.UNSPECIFIED.)
CURVE()
GEOMETRIC_REPRESENTATION_ITEM()
RATIONAL_B_SPLINE_CURVE((1.,1.,1.,1.,1.,1.,1.,1.,1.,1.,1.,1.,1.,1.,1.,1.,
1.,1.,1.,1.,1.,1.,1.,1.,1.,1.))
REPRESENTATION_ITEM('')
);
#804=(
BOUNDED_CURVE()
B_SPLINE_CURVE(5,(#53674,#53675,#53676,#53677,#53678,#53679,#53680,#53681,
#53682,#53683,#53684,#53685,#53686,#53687,#53688,#53689,#53690,#53691,#53692,
#53693,#53694,#53695,#53696,#53697,#53698,#53699,#53700,#53701,#53702,#53703,
#53704,#53705,#53706,#53707),.UNSPECIFIED.,.F.,.F.)
B_SPLINE_CURVE_WITH_KNOTS((6,1,1,1,1,1,1,1,1,1,1,1,1,1,1,1,1,1,1,1,1,1,
1,1,1,1,1,1,1,6),(0.,0.0285714285714286,0.0571428571428571,0.0857142857142857,
0.114285714285714,0.142857142857143,0.171428571428571,0.2,0.228571428571429,
0.257142857142857,0.285714285714286,0.314285714285714,0.342857142857143,
0.371428571428571,0.4,0.428571428571429,0.457142857142857,0.485714285714286,
0.514285714285714,0.542857142857143,0.571428571428572,0.6,0.628571428571429,
0.657142857142857,0.685714285714286,0.714285714285714,0.742857142857143,
0.771428571428572,0.8,0.816564825616131),.UNSPECIFIED.)
CURVE()
GEOMETRIC_REPRESENTATION_ITEM()
RATIONAL_B_SPLINE_CURVE((1.,1.,1.,1.,1.,1.,1.,1.,1.,1.,1.,1.,1.,1.,1.,1.,
1.,1.,1.,1.,1.,1.,1.,1.,1.,1.,1.,1.,1.,1.,1.,1.,1.,1.))
REPRESENTATION_ITEM('')
);
#805=(
BOUNDED_CURVE()
B_SPLINE_CURVE(5,(#53711,#53712,#53713,#53714,#53715,#53716,#53717,#53718,
#53719,#53720,#53721,#53722,#53723,#53724,#53725,#53726,#53727,#53728,#53729,
#53730,#53731,#53732,#53733,#53734,#53735,#53736,#53737,#53738,#53739),
 .UNSPECIFIED.,.F.,.F.)
B_SPLINE_CURVE_WITH_KNOTS((6,1,1,1,1,1,1,1,1,1,1,1,1,1,1,1,1,1,1,1,1,1,
1,1,6),(0.315728291775709,0.342857142857143,0.371428571428571,0.4,0.428571428571429,
0.457142857142857,0.485714285714286,0.514285714285714,0.542857142857143,
0.571428571428572,0.6,0.628571428571429,0.657142857142857,0.685714285714286,
0.714285714285714,0.742857142857143,0.771428571428572,0.8,0.828571428571429,
0.857142857142857,0.885714285714286,0.914285714285714,0.942857142857143,
0.971428571428572,1.),.UNSPECIFIED.)
CURVE()
GEOMETRIC_REPRESENTATION_ITEM()
RATIONAL_B_SPLINE_CURVE((1.,1.,1.,1.,1.,1.,1.,1.,1.,1.,1.,1.,1.,1.,1.,1.,
1.,1.,1.,1.,1.,1.,1.,1.,1.,1.,1.,1.,1.))
REPRESENTATION_ITEM('')
);
#806=(
BOUNDED_CURVE()
B_SPLINE_CURVE(5,(#53743,#53744,#53745,#53746,#53747,#53748,#53749,#53750,
#53751,#53752,#53753,#53754,#53755,#53756,#53757,#53758,#53759,#53760,#53761,
#53762,#53763,#53764,#53765,#53766,#53767,#53768,#53769,#53770,#53771,#53772,
#53773,#53774,#53775,#53776),.UNSPECIFIED.,.F.,.F.)
B_SPLINE_CURVE_WITH_KNOTS((6,1,1,1,1,1,1,1,1,1,1,1,1,1,1,1,1,1,1,1,1,1,
1,1,1,1,1,1,1,6),(0.,0.0285714285714286,0.0571428571428571,0.0857142857142857,
0.114285714285714,0.142857142857143,0.171428571428571,0.2,0.228571428571429,
0.257142857142857,0.285714285714286,0.314285714285714,0.342857142857143,
0.371428571428571,0.4,0.428571428571429,0.457142857142857,0.485714285714286,
0.514285714285714,0.542857142857143,0.571428571428572,0.6,0.628571428571429,
0.657142857142857,0.685714285714286,0.714285714285714,0.742857142857143,
0.771428571428572,0.8,0.816564825616034),.UNSPECIFIED.)
CURVE()
GEOMETRIC_REPRESENTATION_ITEM()
RATIONAL_B_SPLINE_CURVE((1.,1.,1.,1.,1.,1.,1.,1.,1.,1.,1.,1.,1.,1.,1.,1.,
1.,1.,1.,1.,1.,1.,1.,1.,1.,1.,1.,1.,1.,1.,1.,1.,1.,1.))
REPRESENTATION_ITEM('')
);
#807=(
BOUNDED_CURVE()
B_SPLINE_CURVE(5,(#53780,#53781,#53782,#53783,#53784,#53785,#53786,#53787,
#53788,#53789,#53790,#53791,#53792,#53793,#53794,#53795,#53796,#53797,#53798,
#53799,#53800,#53801,#53802,#53803,#53804,#53805,#53806,#53807,#53808),
 .UNSPECIFIED.,.F.,.F.)
B_SPLINE_CURVE_WITH_KNOTS((6,1,1,1,1,1,1,1,1,1,1,1,1,1,1,1,1,1,1,1,1,1,
1,1,6),(0.31572829177571,0.342857142857143,0.371428571428571,0.4,0.428571428571429,
0.457142857142857,0.485714285714286,0.514285714285714,0.542857142857143,
0.571428571428572,0.6,0.628571428571429,0.657142857142857,0.685714285714286,
0.714285714285714,0.742857142857143,0.771428571428572,0.8,0.828571428571429,
0.857142857142857,0.885714285714286,0.914285714285714,0.942857142857143,
0.971428571428572,1.),.UNSPECIFIED.)
CURVE()
GEOMETRIC_REPRESENTATION_ITEM()
RATIONAL_B_SPLINE_CURVE((1.,1.,1.,1.,1.,1.,1.,1.,1.,1.,1.,1.,1.,1.,1.,1.,
1.,1.,1.,1.,1.,1.,1.,1.,1.,1.,1.,1.,1.))
REPRESENTATION_ITEM('')
);
#808=(
BOUNDED_CURVE()
B_SPLINE_CURVE(5,(#53812,#53813,#53814,#53815,#53816,#53817,#53818,#53819,
#53820,#53821,#53822,#53823,#53824,#53825,#53826,#53827,#53828,#53829,#53830,
#53831,#53832,#53833,#53834,#53835,#53836,#53837,#53838,#53839,#53840,#53841,
#53842,#53843,#53844,#53845),.UNSPECIFIED.,.F.,.F.)
B_SPLINE_CURVE_WITH_KNOTS((6,1,1,1,1,1,1,1,1,1,1,1,1,1,1,1,1,1,1,1,1,1,
1,1,1,1,1,1,1,6),(0.,0.0285714285714286,0.0571428571428571,0.0857142857142857,
0.114285714285714,0.142857142857143,0.171428571428571,0.2,0.228571428571429,
0.257142857142857,0.285714285714286,0.314285714285714,0.342857142857143,
0.371428571428571,0.4,0.428571428571429,0.457142857142857,0.485714285714286,
0.514285714285714,0.542857142857143,0.571428571428572,0.6,0.628571428571429,
0.657142857142857,0.685714285714286,0.714285714285714,0.742857142857143,
0.771428571428572,0.8,0.816564825616131),.UNSPECIFIED.)
CURVE()
GEOMETRIC_REPRESENTATION_ITEM()
RATIONAL_B_SPLINE_CURVE((1.,1.,1.,1.,1.,1.,1.,1.,1.,1.,1.,1.,1.,1.,1.,1.,
1.,1.,1.,1.,1.,1.,1.,1.,1.,1.,1.,1.,1.,1.,1.,1.,1.,1.))
REPRESENTATION_ITEM('')
);
#809=(
BOUNDED_CURVE()
B_SPLINE_CURVE(5,(#53849,#53850,#53851,#53852,#53853,#53854,#53855,#53856,
#53857,#53858,#53859,#53860,#53861,#53862,#53863,#53864,#53865,#53866,#53867,
#53868,#53869,#53870,#53871,#53872,#53873,#53874,#53875,#53876,#53877),
 .UNSPECIFIED.,.F.,.F.)
B_SPLINE_CURVE_WITH_KNOTS((6,1,1,1,1,1,1,1,1,1,1,1,1,1,1,1,1,1,1,1,1,1,
1,1,6),(0.315728291775709,0.342857142857143,0.371428571428571,0.4,0.428571428571429,
0.457142857142857,0.485714285714286,0.514285714285714,0.542857142857143,
0.571428571428572,0.6,0.628571428571429,0.657142857142857,0.685714285714286,
0.714285714285714,0.742857142857143,0.771428571428572,0.8,0.828571428571429,
0.857142857142857,0.885714285714286,0.914285714285714,0.942857142857143,
0.971428571428572,1.),.UNSPECIFIED.)
CURVE()
GEOMETRIC_REPRESENTATION_ITEM()
RATIONAL_B_SPLINE_CURVE((1.,1.,1.,1.,1.,1.,1.,1.,1.,1.,1.,1.,1.,1.,1.,1.,
1.,1.,1.,1.,1.,1.,1.,1.,1.,1.,1.,1.,1.))
REPRESENTATION_ITEM('')
);
#810=(
BOUNDED_CURVE()
B_SPLINE_CURVE(5,(#53881,#53882,#53883,#53884,#53885,#53886,#53887,#53888,
#53889,#53890,#53891,#53892,#53893,#53894,#53895,#53896,#53897,#53898,#53899,
#53900,#53901,#53902,#53903,#53904,#53905,#53906,#53907,#53908,#53909,#53910,
#53911,#53912,#53913,#53914),.UNSPECIFIED.,.F.,.F.)
B_SPLINE_CURVE_WITH_KNOTS((6,1,1,1,1,1,1,1,1,1,1,1,1,1,1,1,1,1,1,1,1,1,
1,1,1,1,1,1,1,6),(0.,0.0285714285714286,0.0571428571428571,0.0857142857142857,
0.114285714285714,0.142857142857143,0.171428571428571,0.2,0.228571428571429,
0.257142857142857,0.285714285714286,0.314285714285714,0.342857142857143,
0.371428571428571,0.4,0.428571428571429,0.457142857142857,0.485714285714286,
0.514285714285714,0.542857142857143,0.571428571428572,0.6,0.628571428571429,
0.657142857142857,0.685714285714286,0.714285714285714,0.742857142857143,
0.771428571428572,0.8,0.816564825616034),.UNSPECIFIED.)
CURVE()
GEOMETRIC_REPRESENTATION_ITEM()
RATIONAL_B_SPLINE_CURVE((1.,1.,1.,1.,1.,1.,1.,1.,1.,1.,1.,1.,1.,1.,1.,1.,
1.,1.,1.,1.,1.,1.,1.,1.,1.,1.,1.,1.,1.,1.,1.,1.,1.,1.))
REPRESENTATION_ITEM('')
);
#811=(
BOUNDED_CURVE()
B_SPLINE_CURVE(5,(#53918,#53919,#53920,#53921,#53922,#53923,#53924,#53925,
#53926,#53927,#53928,#53929,#53930,#53931,#53932,#53933,#53934,#53935,#53936,
#53937,#53938,#53939,#53940,#53941,#53942,#53943,#53944,#53945,#53946),
 .UNSPECIFIED.,.F.,.F.)
B_SPLINE_CURVE_WITH_KNOTS((6,1,1,1,1,1,1,1,1,1,1,1,1,1,1,1,1,1,1,1,1,1,
1,1,6),(0.315728291775709,0.342857142857143,0.371428571428571,0.4,0.428571428571429,
0.457142857142857,0.485714285714286,0.514285714285714,0.542857142857143,
0.571428571428572,0.6,0.628571428571429,0.657142857142857,0.685714285714286,
0.714285714285714,0.742857142857143,0.771428571428572,0.8,0.828571428571429,
0.857142857142857,0.885714285714286,0.914285714285714,0.942857142857143,
0.971428571428572,1.),.UNSPECIFIED.)
CURVE()
GEOMETRIC_REPRESENTATION_ITEM()
RATIONAL_B_SPLINE_CURVE((1.,1.,1.,1.,1.,1.,1.,1.,1.,1.,1.,1.,1.,1.,1.,1.,
1.,1.,1.,1.,1.,1.,1.,1.,1.,1.,1.,1.,1.))
REPRESENTATION_ITEM('')
);
#812=(
BOUNDED_CURVE()
B_SPLINE_CURVE(5,(#53950,#53951,#53952,#53953,#53954,#53955,#53956,#53957,
#53958,#53959,#53960,#53961,#53962,#53963,#53964,#53965,#53966,#53967,#53968,
#53969,#53970,#53971,#53972,#53973,#53974,#53975,#53976,#53977,#53978,#53979,
#53980,#53981,#53982,#53983),.UNSPECIFIED.,.F.,.F.)
B_SPLINE_CURVE_WITH_KNOTS((6,1,1,1,1,1,1,1,1,1,1,1,1,1,1,1,1,1,1,1,1,1,
1,1,1,1,1,1,1,6),(0.,0.0285714285714286,0.0571428571428571,0.0857142857142857,
0.114285714285714,0.142857142857143,0.171428571428571,0.2,0.228571428571429,
0.257142857142857,0.285714285714286,0.314285714285714,0.342857142857143,
0.371428571428571,0.4,0.428571428571429,0.457142857142857,0.485714285714286,
0.514285714285714,0.542857142857143,0.571428571428572,0.6,0.628571428571429,
0.657142857142857,0.685714285714286,0.714285714285714,0.742857142857143,
0.771428571428572,0.8,0.816564825616131),.UNSPECIFIED.)
CURVE()
GEOMETRIC_REPRESENTATION_ITEM()
RATIONAL_B_SPLINE_CURVE((1.,1.,1.,1.,1.,1.,1.,1.,1.,1.,1.,1.,1.,1.,1.,1.,
1.,1.,1.,1.,1.,1.,1.,1.,1.,1.,1.,1.,1.,1.,1.,1.,1.,1.))
REPRESENTATION_ITEM('')
);
#813=(
BOUNDED_CURVE()
B_SPLINE_CURVE(5,(#53987,#53988,#53989,#53990,#53991,#53992,#53993,#53994,
#53995,#53996,#53997,#53998,#53999,#54000,#54001,#54002,#54003,#54004,#54005,
#54006,#54007,#54008,#54009,#54010,#54011,#54012,#54013,#54014,#54015),
 .UNSPECIFIED.,.F.,.F.)
B_SPLINE_CURVE_WITH_KNOTS((6,1,1,1,1,1,1,1,1,1,1,1,1,1,1,1,1,1,1,1,1,1,
1,1,6),(0.315728291775709,0.342857142857143,0.371428571428571,0.4,0.428571428571429,
0.457142857142857,0.485714285714286,0.514285714285714,0.542857142857143,
0.571428571428572,0.6,0.628571428571429,0.657142857142857,0.685714285714286,
0.714285714285714,0.742857142857143,0.771428571428572,0.8,0.828571428571429,
0.857142857142857,0.885714285714286,0.914285714285714,0.942857142857143,
0.971428571428572,1.),.UNSPECIFIED.)
CURVE()
GEOMETRIC_REPRESENTATION_ITEM()
RATIONAL_B_SPLINE_CURVE((1.,1.,1.,1.,1.,1.,1.,1.,1.,1.,1.,1.,1.,1.,1.,1.,
1.,1.,1.,1.,1.,1.,1.,1.,1.,1.,1.,1.,1.))
REPRESENTATION_ITEM('')
);
#814=(
BOUNDED_CURVE()
B_SPLINE_CURVE(5,(#54019,#54020,#54021,#54022,#54023,#54024,#54025,#54026,
#54027,#54028,#54029,#54030,#54031,#54032,#54033,#54034,#54035,#54036,#54037,
#54038,#54039,#54040,#54041,#54042,#54043,#54044,#54045,#54046,#54047,#54048,
#54049,#54050,#54051,#54052),.UNSPECIFIED.,.F.,.F.)
B_SPLINE_CURVE_WITH_KNOTS((6,1,1,1,1,1,1,1,1,1,1,1,1,1,1,1,1,1,1,1,1,1,
1,1,1,1,1,1,1,6),(0.,0.0285714285714286,0.0571428571428571,0.0857142857142857,
0.114285714285714,0.142857142857143,0.171428571428571,0.2,0.228571428571429,
0.257142857142857,0.285714285714286,0.314285714285714,0.342857142857143,
0.371428571428571,0.4,0.428571428571429,0.457142857142857,0.485714285714286,
0.514285714285714,0.542857142857143,0.571428571428572,0.6,0.628571428571429,
0.657142857142857,0.685714285714286,0.714285714285714,0.742857142857143,
0.771428571428572,0.8,0.816564825616033),.UNSPECIFIED.)
CURVE()
GEOMETRIC_REPRESENTATION_ITEM()
RATIONAL_B_SPLINE_CURVE((1.,1.,1.,1.,1.,1.,1.,1.,1.,1.,1.,1.,1.,1.,1.,1.,
1.,1.,1.,1.,1.,1.,1.,1.,1.,1.,1.,1.,1.,1.,1.,1.,1.,1.))
REPRESENTATION_ITEM('')
);
#815=(
BOUNDED_CURVE()
B_SPLINE_CURVE(5,(#54056,#54057,#54058,#54059,#54060,#54061,#54062,#54063,
#54064,#54065,#54066,#54067,#54068,#54069,#54070,#54071,#54072,#54073,#54074,
#54075,#54076,#54077,#54078,#54079,#54080,#54081,#54082,#54083,#54084),
 .UNSPECIFIED.,.F.,.F.)
B_SPLINE_CURVE_WITH_KNOTS((6,1,1,1,1,1,1,1,1,1,1,1,1,1,1,1,1,1,1,1,1,1,
1,1,6),(0.31572829177571,0.342857142857143,0.371428571428571,0.4,0.428571428571429,
0.457142857142857,0.485714285714286,0.514285714285714,0.542857142857143,
0.571428571428572,0.6,0.628571428571429,0.657142857142857,0.685714285714286,
0.714285714285714,0.742857142857143,0.771428571428572,0.8,0.828571428571429,
0.857142857142857,0.885714285714286,0.914285714285714,0.942857142857143,
0.971428571428572,1.),.UNSPECIFIED.)
CURVE()
GEOMETRIC_REPRESENTATION_ITEM()
RATIONAL_B_SPLINE_CURVE((1.,1.,1.,1.,1.,1.,1.,1.,1.,1.,1.,1.,1.,1.,1.,1.,
1.,1.,1.,1.,1.,1.,1.,1.,1.,1.,1.,1.,1.))
REPRESENTATION_ITEM('')
);
#816=(
BOUNDED_CURVE()
B_SPLINE_CURVE(5,(#54088,#54089,#54090,#54091,#54092,#54093,#54094,#54095,
#54096,#54097,#54098,#54099,#54100,#54101,#54102,#54103,#54104,#54105,#54106,
#54107,#54108,#54109,#54110,#54111,#54112,#54113,#54114,#54115,#54116,#54117,
#54118,#54119,#54120,#54121),.UNSPECIFIED.,.F.,.F.)
B_SPLINE_CURVE_WITH_KNOTS((6,1,1,1,1,1,1,1,1,1,1,1,1,1,1,1,1,1,1,1,1,1,
1,1,1,1,1,1,1,6),(0.,0.0285714285714286,0.0571428571428571,0.0857142857142857,
0.114285714285714,0.142857142857143,0.171428571428571,0.2,0.228571428571429,
0.257142857142857,0.285714285714286,0.314285714285714,0.342857142857143,
0.371428571428571,0.4,0.428571428571429,0.457142857142857,0.485714285714286,
0.514285714285714,0.542857142857143,0.571428571428572,0.6,0.628571428571429,
0.657142857142857,0.685714285714286,0.714285714285714,0.742857142857143,
0.771428571428572,0.8,0.816564825616131),.UNSPECIFIED.)
CURVE()
GEOMETRIC_REPRESENTATION_ITEM()
RATIONAL_B_SPLINE_CURVE((1.,1.,1.,1.,1.,1.,1.,1.,1.,1.,1.,1.,1.,1.,1.,1.,
1.,1.,1.,1.,1.,1.,1.,1.,1.,1.,1.,1.,1.,1.,1.,1.,1.,1.))
REPRESENTATION_ITEM('')
);
#817=(
BOUNDED_CURVE()
B_SPLINE_CURVE(5,(#54125,#54126,#54127,#54128,#54129,#54130,#54131,#54132,
#54133,#54134,#54135,#54136,#54137,#54138,#54139,#54140,#54141,#54142,#54143,
#54144,#54145,#54146,#54147,#54148,#54149,#54150,#54151,#54152,#54153),
 .UNSPECIFIED.,.F.,.F.)
B_SPLINE_CURVE_WITH_KNOTS((6,1,1,1,1,1,1,1,1,1,1,1,1,1,1,1,1,1,1,1,1,1,
1,1,6),(0.315728291775709,0.342857142857143,0.371428571428571,0.4,0.428571428571429,
0.457142857142857,0.485714285714286,0.514285714285714,0.542857142857143,
0.571428571428572,0.6,0.628571428571429,0.657142857142857,0.685714285714286,
0.714285714285714,0.742857142857143,0.771428571428572,0.8,0.828571428571429,
0.857142857142857,0.885714285714286,0.914285714285714,0.942857142857143,
0.971428571428572,1.),.UNSPECIFIED.)
CURVE()
GEOMETRIC_REPRESENTATION_ITEM()
RATIONAL_B_SPLINE_CURVE((1.,1.,1.,1.,1.,1.,1.,1.,1.,1.,1.,1.,1.,1.,1.,1.,
1.,1.,1.,1.,1.,1.,1.,1.,1.,1.,1.,1.,1.))
REPRESENTATION_ITEM('')
);
#818=(
BOUNDED_CURVE()
B_SPLINE_CURVE(5,(#54157,#54158,#54159,#54160,#54161,#54162,#54163,#54164,
#54165,#54166,#54167,#54168,#54169,#54170,#54171,#54172,#54173,#54174,#54175,
#54176,#54177,#54178,#54179,#54180,#54181,#54182,#54183,#54184,#54185,#54186,
#54187,#54188,#54189,#54190),.UNSPECIFIED.,.F.,.F.)
B_SPLINE_CURVE_WITH_KNOTS((6,1,1,1,1,1,1,1,1,1,1,1,1,1,1,1,1,1,1,1,1,1,
1,1,1,1,1,1,1,6),(0.,0.0285714285714286,0.0571428571428571,0.0857142857142857,
0.114285714285714,0.142857142857143,0.171428571428571,0.2,0.228571428571429,
0.257142857142857,0.285714285714286,0.314285714285714,0.342857142857143,
0.371428571428571,0.4,0.428571428571429,0.457142857142857,0.485714285714286,
0.514285714285714,0.542857142857143,0.571428571428572,0.6,0.628571428571429,
0.657142857142857,0.685714285714286,0.714285714285714,0.742857142857143,
0.771428571428572,0.8,0.816564825616034),.UNSPECIFIED.)
CURVE()
GEOMETRIC_REPRESENTATION_ITEM()
RATIONAL_B_SPLINE_CURVE((1.,1.,1.,1.,1.,1.,1.,1.,1.,1.,1.,1.,1.,1.,1.,1.,
1.,1.,1.,1.,1.,1.,1.,1.,1.,1.,1.,1.,1.,1.,1.,1.,1.,1.))
REPRESENTATION_ITEM('')
);
#819=(
BOUNDED_CURVE()
B_SPLINE_CURVE(5,(#54194,#54195,#54196,#54197,#54198,#54199,#54200,#54201,
#54202,#54203,#54204,#54205,#54206,#54207,#54208,#54209,#54210,#54211,#54212,
#54213,#54214,#54215,#54216,#54217,#54218,#54219,#54220,#54221,#54222),
 .UNSPECIFIED.,.F.,.F.)
B_SPLINE_CURVE_WITH_KNOTS((6,1,1,1,1,1,1,1,1,1,1,1,1,1,1,1,1,1,1,1,1,1,
1,1,6),(0.315728291775709,0.342857142857143,0.371428571428571,0.4,0.428571428571429,
0.457142857142857,0.485714285714286,0.514285714285714,0.542857142857143,
0.571428571428572,0.6,0.628571428571429,0.657142857142857,0.685714285714286,
0.714285714285714,0.742857142857143,0.771428571428572,0.8,0.828571428571429,
0.857142857142857,0.885714285714286,0.914285714285714,0.942857142857143,
0.971428571428572,1.),.UNSPECIFIED.)
CURVE()
GEOMETRIC_REPRESENTATION_ITEM()
RATIONAL_B_SPLINE_CURVE((1.,1.,1.,1.,1.,1.,1.,1.,1.,1.,1.,1.,1.,1.,1.,1.,
1.,1.,1.,1.,1.,1.,1.,1.,1.,1.,1.,1.,1.))
REPRESENTATION_ITEM('')
);
#820=(
BOUNDED_CURVE()
B_SPLINE_CURVE(5,(#54226,#54227,#54228,#54229,#54230,#54231,#54232,#54233,
#54234,#54235,#54236,#54237,#54238,#54239,#54240,#54241,#54242,#54243,#54244,
#54245,#54246,#54247,#54248,#54249,#54250,#54251,#54252,#54253,#54254,#54255,
#54256,#54257,#54258,#54259),.UNSPECIFIED.,.F.,.F.)
B_SPLINE_CURVE_WITH_KNOTS((6,1,1,1,1,1,1,1,1,1,1,1,1,1,1,1,1,1,1,1,1,1,
1,1,1,1,1,1,1,6),(0.,0.0285714285714286,0.0571428571428571,0.0857142857142857,
0.114285714285714,0.142857142857143,0.171428571428571,0.2,0.228571428571429,
0.257142857142857,0.285714285714286,0.314285714285714,0.342857142857143,
0.371428571428571,0.4,0.428571428571429,0.457142857142857,0.485714285714286,
0.514285714285714,0.542857142857143,0.571428571428572,0.6,0.628571428571429,
0.657142857142857,0.685714285714286,0.714285714285714,0.742857142857143,
0.771428571428572,0.8,0.816564825616131),.UNSPECIFIED.)
CURVE()
GEOMETRIC_REPRESENTATION_ITEM()
RATIONAL_B_SPLINE_CURVE((1.,1.,1.,1.,1.,1.,1.,1.,1.,1.,1.,1.,1.,1.,1.,1.,
1.,1.,1.,1.,1.,1.,1.,1.,1.,1.,1.,1.,1.,1.,1.,1.,1.,1.))
REPRESENTATION_ITEM('')
);
#821=(
BOUNDED_CURVE()
B_SPLINE_CURVE(5,(#54263,#54264,#54265,#54266,#54267,#54268,#54269,#54270,
#54271,#54272,#54273,#54274,#54275,#54276,#54277,#54278,#54279,#54280,#54281,
#54282,#54283,#54284,#54285,#54286,#54287,#54288,#54289,#54290,#54291),
 .UNSPECIFIED.,.F.,.F.)
B_SPLINE_CURVE_WITH_KNOTS((6,1,1,1,1,1,1,1,1,1,1,1,1,1,1,1,1,1,1,1,1,1,
1,1,6),(0.31572829177571,0.342857142857143,0.371428571428571,0.4,0.428571428571429,
0.457142857142857,0.485714285714286,0.514285714285714,0.542857142857143,
0.571428571428572,0.6,0.628571428571429,0.657142857142857,0.685714285714286,
0.714285714285714,0.742857142857143,0.771428571428572,0.8,0.828571428571429,
0.857142857142857,0.885714285714286,0.914285714285714,0.942857142857143,
0.971428571428572,1.),.UNSPECIFIED.)
CURVE()
GEOMETRIC_REPRESENTATION_ITEM()
RATIONAL_B_SPLINE_CURVE((1.,1.,1.,1.,1.,1.,1.,1.,1.,1.,1.,1.,1.,1.,1.,1.,
1.,1.,1.,1.,1.,1.,1.,1.,1.,1.,1.,1.,1.))
REPRESENTATION_ITEM('')
);
#822=(
BOUNDED_CURVE()
B_SPLINE_CURVE(5,(#54295,#54296,#54297,#54298,#54299,#54300,#54301,#54302,
#54303,#54304,#54305,#54306,#54307,#54308,#54309,#54310,#54311,#54312,#54313,
#54314,#54315,#54316,#54317,#54318,#54319,#54320,#54321,#54322,#54323,#54324,
#54325,#54326,#54327,#54328),.UNSPECIFIED.,.F.,.F.)
B_SPLINE_CURVE_WITH_KNOTS((6,1,1,1,1,1,1,1,1,1,1,1,1,1,1,1,1,1,1,1,1,1,
1,1,1,1,1,1,1,6),(0.,0.0285714285714286,0.0571428571428571,0.0857142857142857,
0.114285714285714,0.142857142857143,0.171428571428571,0.2,0.228571428571429,
0.257142857142857,0.285714285714286,0.314285714285714,0.342857142857143,
0.371428571428571,0.4,0.428571428571429,0.457142857142857,0.485714285714286,
0.514285714285714,0.542857142857143,0.571428571428572,0.6,0.628571428571429,
0.657142857142857,0.685714285714286,0.714285714285714,0.742857142857143,
0.771428571428572,0.8,0.816564825616034),.UNSPECIFIED.)
CURVE()
GEOMETRIC_REPRESENTATION_ITEM()
RATIONAL_B_SPLINE_CURVE((1.,1.,1.,1.,1.,1.,1.,1.,1.,1.,1.,1.,1.,1.,1.,1.,
1.,1.,1.,1.,1.,1.,1.,1.,1.,1.,1.,1.,1.,1.,1.,1.,1.,1.))
REPRESENTATION_ITEM('')
);
#823=(
BOUNDED_CURVE()
B_SPLINE_CURVE(5,(#54332,#54333,#54334,#54335,#54336,#54337,#54338,#54339,
#54340,#54341,#54342,#54343,#54344,#54345,#54346,#54347,#54348,#54349,#54350,
#54351,#54352,#54353,#54354,#54355,#54356,#54357,#54358,#54359,#54360),
 .UNSPECIFIED.,.F.,.F.)
B_SPLINE_CURVE_WITH_KNOTS((6,1,1,1,1,1,1,1,1,1,1,1,1,1,1,1,1,1,1,1,1,1,
1,1,6),(0.31572829177571,0.342857142857143,0.371428571428571,0.4,0.428571428571429,
0.457142857142857,0.485714285714286,0.514285714285714,0.542857142857143,
0.571428571428572,0.6,0.628571428571429,0.657142857142857,0.685714285714286,
0.714285714285714,0.742857142857143,0.771428571428572,0.8,0.828571428571429,
0.857142857142857,0.885714285714286,0.914285714285714,0.942857142857143,
0.971428571428572,1.),.UNSPECIFIED.)
CURVE()
GEOMETRIC_REPRESENTATION_ITEM()
RATIONAL_B_SPLINE_CURVE((1.,1.,1.,1.,1.,1.,1.,1.,1.,1.,1.,1.,1.,1.,1.,1.,
1.,1.,1.,1.,1.,1.,1.,1.,1.,1.,1.,1.,1.))
REPRESENTATION_ITEM('')
);
#824=(
BOUNDED_CURVE()
B_SPLINE_CURVE(5,(#54364,#54365,#54366,#54367,#54368,#54369,#54370,#54371,
#54372,#54373,#54374,#54375,#54376,#54377,#54378,#54379,#54380,#54381,#54382,
#54383,#54384,#54385,#54386,#54387,#54388,#54389,#54390,#54391,#54392,#54393,
#54394,#54395,#54396,#54397),.UNSPECIFIED.,.F.,.F.)
B_SPLINE_CURVE_WITH_KNOTS((6,1,1,1,1,1,1,1,1,1,1,1,1,1,1,1,1,1,1,1,1,1,
1,1,1,1,1,1,1,6),(0.,0.0285714285714286,0.0571428571428571,0.0857142857142857,
0.114285714285714,0.142857142857143,0.171428571428571,0.2,0.228571428571429,
0.257142857142857,0.285714285714286,0.314285714285714,0.342857142857143,
0.371428571428571,0.4,0.428571428571429,0.457142857142857,0.485714285714286,
0.514285714285714,0.542857142857143,0.571428571428572,0.6,0.628571428571429,
0.657142857142857,0.685714285714286,0.714285714285714,0.742857142857143,
0.771428571428572,0.8,0.816564825616131),.UNSPECIFIED.)
CURVE()
GEOMETRIC_REPRESENTATION_ITEM()
RATIONAL_B_SPLINE_CURVE((1.,1.,1.,1.,1.,1.,1.,1.,1.,1.,1.,1.,1.,1.,1.,1.,
1.,1.,1.,1.,1.,1.,1.,1.,1.,1.,1.,1.,1.,1.,1.,1.,1.,1.))
REPRESENTATION_ITEM('')
);
#825=(
BOUNDED_CURVE()
B_SPLINE_CURVE(5,(#54401,#54402,#54403,#54404,#54405,#54406,#54407,#54408,
#54409,#54410,#54411,#54412,#54413,#54414,#54415,#54416,#54417,#54418,#54419,
#54420,#54421,#54422,#54423,#54424,#54425,#54426,#54427,#54428,#54429),
 .UNSPECIFIED.,.F.,.F.)
B_SPLINE_CURVE_WITH_KNOTS((6,1,1,1,1,1,1,1,1,1,1,1,1,1,1,1,1,1,1,1,1,1,
1,1,6),(0.315728291775709,0.342857142857143,0.371428571428571,0.4,0.428571428571429,
0.457142857142857,0.485714285714286,0.514285714285714,0.542857142857143,
0.571428571428572,0.6,0.628571428571429,0.657142857142857,0.685714285714286,
0.714285714285714,0.742857142857143,0.771428571428572,0.8,0.828571428571429,
0.857142857142857,0.885714285714286,0.914285714285714,0.942857142857143,
0.971428571428572,1.),.UNSPECIFIED.)
CURVE()
GEOMETRIC_REPRESENTATION_ITEM()
RATIONAL_B_SPLINE_CURVE((1.,1.,1.,1.,1.,1.,1.,1.,1.,1.,1.,1.,1.,1.,1.,1.,
1.,1.,1.,1.,1.,1.,1.,1.,1.,1.,1.,1.,1.))
REPRESENTATION_ITEM('')
);
#826=(
BOUNDED_CURVE()
B_SPLINE_CURVE(5,(#54433,#54434,#54435,#54436,#54437,#54438,#54439,#54440,
#54441,#54442,#54443,#54444,#54445,#54446,#54447,#54448,#54449,#54450,#54451,
#54452,#54453,#54454,#54455,#54456,#54457,#54458,#54459,#54460,#54461,#54462,
#54463,#54464,#54465,#54466),.UNSPECIFIED.,.F.,.F.)
B_SPLINE_CURVE_WITH_KNOTS((6,1,1,1,1,1,1,1,1,1,1,1,1,1,1,1,1,1,1,1,1,1,
1,1,1,1,1,1,1,6),(0.,0.0285714285714286,0.0571428571428571,0.0857142857142857,
0.114285714285714,0.142857142857143,0.171428571428571,0.2,0.228571428571429,
0.257142857142857,0.285714285714286,0.314285714285714,0.342857142857143,
0.371428571428571,0.4,0.428571428571429,0.457142857142857,0.485714285714286,
0.514285714285714,0.542857142857143,0.571428571428572,0.6,0.628571428571429,
0.657142857142857,0.685714285714286,0.714285714285714,0.742857142857143,
0.771428571428572,0.8,0.816564825616131),.UNSPECIFIED.)
CURVE()
GEOMETRIC_REPRESENTATION_ITEM()
RATIONAL_B_SPLINE_CURVE((1.,1.,1.,1.,1.,1.,1.,1.,1.,1.,1.,1.,1.,1.,1.,1.,
1.,1.,1.,1.,1.,1.,1.,1.,1.,1.,1.,1.,1.,1.,1.,1.,1.,1.))
REPRESENTATION_ITEM('')
);
#827=(
BOUNDED_CURVE()
B_SPLINE_CURVE(5,(#54469,#54470,#54471,#54472,#54473,#54474,#54475,#54476,
#54477,#54478,#54479,#54480,#54481,#54482,#54483,#54484,#54485,#54486,#54487,
#54488,#54489,#54490,#54491,#54492,#54493,#54494,#54495,#54496,#54497),
 .UNSPECIFIED.,.F.,.F.)
B_SPLINE_CURVE_WITH_KNOTS((6,1,1,1,1,1,1,1,1,1,1,1,1,1,1,1,1,1,1,1,1,1,
1,1,6),(0.315728291775709,0.342857142857143,0.371428571428571,0.4,0.428571428571429,
0.457142857142857,0.485714285714286,0.514285714285714,0.542857142857143,
0.571428571428572,0.6,0.628571428571429,0.657142857142857,0.685714285714286,
0.714285714285714,0.742857142857143,0.771428571428572,0.8,0.828571428571429,
0.857142857142857,0.885714285714286,0.914285714285714,0.942857142857143,
0.971428571428572,1.),.UNSPECIFIED.)
CURVE()
GEOMETRIC_REPRESENTATION_ITEM()
RATIONAL_B_SPLINE_CURVE((1.,1.,1.,1.,1.,1.,1.,1.,1.,1.,1.,1.,1.,1.,1.,1.,
1.,1.,1.,1.,1.,1.,1.,1.,1.,1.,1.,1.,1.))
REPRESENTATION_ITEM('')
);
#971=PLANE('',#21306);
#972=PLANE('',#21337);
#973=PLANE('',#21396);
#1115=FACE_BOUND('',#2974,.T.);
#1116=FACE_BOUND('',#2977,.T.);
#1117=FACE_BOUND('',#2987,.T.);
#1752=FACE_OUTER_BOUND('',#2971,.T.);
#1753=FACE_OUTER_BOUND('',#2972,.T.);
#1754=FACE_OUTER_BOUND('',#2973,.T.);
#1755=FACE_OUTER_BOUND('',#2975,.T.);
#1756=FACE_OUTER_BOUND('',#2976,.T.);
#1757=FACE_OUTER_BOUND('',#2978,.T.);
#1758=FACE_OUTER_BOUND('',#2979,.T.);
#1759=FACE_OUTER_BOUND('',#2980,.T.);
#1760=FACE_OUTER_BOUND('',#2981,.T.);
#1761=FACE_OUTER_BOUND('',#2982,.T.);
#1762=FACE_OUTER_BOUND('',#2983,.T.);
#1763=FACE_OUTER_BOUND('',#2984,.T.);
#1764=FACE_OUTER_BOUND('',#2985,.T.);
#1765=FACE_OUTER_BOUND('',#2986,.T.);
#1766=FACE_OUTER_BOUND('',#2988,.T.);
#1767=FACE_OUTER_BOUND('',#2989,.T.);
#1768=FACE_OUTER_BOUND('',#2990,.T.);
#1769=FACE_OUTER_BOUND('',#2991,.T.);
#1770=FACE_OUTER_BOUND('',#2992,.T.);
#1771=FACE_OUTER_BOUND('',#2993,.T.);
#1772=FACE_OUTER_BOUND('',#2994,.T.);
#1773=FACE_OUTER_BOUND('',#2995,.T.);
#1774=FACE_OUTER_BOUND('',#2996,.T.);
#1775=FACE_OUTER_BOUND('',#2997,.T.);
#1776=FACE_OUTER_BOUND('',#2998,.T.);
#1777=FACE_OUTER_BOUND('',#2999,.T.);
#1778=FACE_OUTER_BOUND('',#3000,.T.);
#1779=FACE_OUTER_BOUND('',#3001,.T.);
#1780=FACE_OUTER_BOUND('',#3002,.T.);
#1781=FACE_OUTER_BOUND('',#3003,.T.);
#1782=FACE_OUTER_BOUND('',#3004,.T.);
#1783=FACE_OUTER_BOUND('',#3005,.T.);
#1784=FACE_OUTER_BOUND('',#3006,.T.);
#1785=FACE_OUTER_BOUND('',#3007,.T.);
#1786=FACE_OUTER_BOUND('',#3008,.T.);
#1787=FACE_OUTER_BOUND('',#3009,.T.);
#1788=FACE_OUTER_BOUND('',#3010,.T.);
#1789=FACE_OUTER_BOUND('',#3011,.T.);
#1790=FACE_OUTER_BOUND('',#3012,.T.);
#1791=FACE_OUTER_BOUND('',#3013,.T.);
#1792=FACE_OUTER_BOUND('',#3014,.T.);
#1793=FACE_OUTER_BOUND('',#3015,.T.);
#1794=FACE_OUTER_BOUND('',#3016,.T.);
#1795=FACE_OUTER_BOUND('',#3017,.T.);
#1796=FACE_OUTER_BOUND('',#3018,.T.);
#1797=FACE_OUTER_BOUND('',#3019,.T.);
#1798=FACE_OUTER_BOUND('',#3020,.T.);
#1799=FACE_OUTER_BOUND('',#3021,.T.);
#1800=FACE_OUTER_BOUND('',#3022,.T.);
#1801=FACE_OUTER_BOUND('',#3023,.T.);
#1802=FACE_OUTER_BOUND('',#3024,.T.);
#1803=FACE_OUTER_BOUND('',#3025,.T.);
#1804=FACE_OUTER_BOUND('',#3026,.T.);
#1805=FACE_OUTER_BOUND('',#3027,.T.);
#1806=FACE_OUTER_BOUND('',#3028,.T.);
#1807=FACE_OUTER_BOUND('',#3029,.T.);
#1808=FACE_OUTER_BOUND('',#3030,.T.);
#1809=FACE_OUTER_BOUND('',#3031,.T.);
#1810=FACE_OUTER_BOUND('',#3032,.T.);
#1811=FACE_OUTER_BOUND('',#3033,.T.);
#1812=FACE_OUTER_BOUND('',#3034,.T.);
#1813=FACE_OUTER_BOUND('',#3035,.T.);
#1814=FACE_OUTER_BOUND('',#3036,.T.);
#1815=FACE_OUTER_BOUND('',#3037,.T.);
#1816=FACE_OUTER_BOUND('',#3038,.T.);
#1817=FACE_OUTER_BOUND('',#3039,.T.);
#1818=FACE_OUTER_BOUND('',#3040,.T.);
#1819=FACE_OUTER_BOUND('',#3041,.T.);
#1820=FACE_OUTER_BOUND('',#3042,.T.);
#1821=FACE_OUTER_BOUND('',#3043,.T.);
#1822=FACE_OUTER_BOUND('',#3044,.T.);
#1823=FACE_OUTER_BOUND('',#3045,.T.);
#1824=FACE_OUTER_BOUND('',#3046,.T.);
#1825=FACE_OUTER_BOUND('',#3047,.T.);
#1826=FACE_OUTER_BOUND('',#3048,.T.);
#1827=FACE_OUTER_BOUND('',#3049,.T.);
#1828=FACE_OUTER_BOUND('',#3050,.T.);
#1829=FACE_OUTER_BOUND('',#3051,.T.);
#1830=FACE_OUTER_BOUND('',#3052,.T.);
#1831=FACE_OUTER_BOUND('',#3053,.T.);
#1832=FACE_OUTER_BOUND('',#3054,.T.);
#1833=FACE_OUTER_BOUND('',#3055,.T.);
#1834=FACE_OUTER_BOUND('',#3056,.T.);
#1835=FACE_OUTER_BOUND('',#3057,.T.);
#1836=FACE_OUTER_BOUND('',#3058,.T.);
#1837=FACE_OUTER_BOUND('',#3059,.T.);
#1838=FACE_OUTER_BOUND('',#3060,.T.);
#1839=FACE_OUTER_BOUND('',#3061,.T.);
#1840=FACE_OUTER_BOUND('',#3062,.T.);
#1841=FACE_OUTER_BOUND('',#3063,.T.);
#1842=FACE_OUTER_BOUND('',#3064,.T.);
#1843=FACE_OUTER_BOUND('',#3065,.T.);
#1844=FACE_OUTER_BOUND('',#3066,.T.);
#1845=FACE_OUTER_BOUND('',#3067,.T.);
#1846=FACE_OUTER_BOUND('',#3068,.T.);
#1847=FACE_OUTER_BOUND('',#3069,.T.);
#1848=FACE_OUTER_BOUND('',#3070,.T.);
#1849=FACE_OUTER_BOUND('',#3071,.T.);
#1850=FACE_OUTER_BOUND('',#3072,.T.);
#1851=FACE_OUTER_BOUND('',#3073,.T.);
#1852=FACE_OUTER_BOUND('',#3074,.T.);
#1853=FACE_OUTER_BOUND('',#3075,.T.);
#1854=FACE_OUTER_BOUND('',#3076,.T.);
#1855=FACE_OUTER_BOUND('',#3077,.T.);
#1856=FACE_OUTER_BOUND('',#3078,.T.);
#1857=FACE_OUTER_BOUND('',#3079,.T.);
#1858=FACE_OUTER_BOUND('',#3080,.T.);
#1859=FACE_OUTER_BOUND('',#3081,.T.);
#1860=FACE_OUTER_BOUND('',#3082,.T.);
#1861=FACE_OUTER_BOUND('',#3083,.T.);
#1862=FACE_OUTER_BOUND('',#3084,.T.);
#1863=FACE_OUTER_BOUND('',#3085,.T.);
#1864=FACE_OUTER_BOUND('',#3086,.T.);
#1865=FACE_OUTER_BOUND('',#3087,.T.);
#1866=FACE_OUTER_BOUND('',#3088,.T.);
#1867=FACE_OUTER_BOUND('',#3089,.T.);
#1868=FACE_OUTER_BOUND('',#3090,.T.);
#1869=FACE_OUTER_BOUND('',#3091,.T.);
#1870=FACE_OUTER_BOUND('',#3092,.T.);
#1871=FACE_OUTER_BOUND('',#3093,.T.);
#1872=FACE_OUTER_BOUND('',#3094,.T.);
#1873=FACE_OUTER_BOUND('',#3095,.T.);
#1874=FACE_OUTER_BOUND('',#3096,.T.);
#1875=FACE_OUTER_BOUND('',#3097,.T.);
#1876=FACE_OUTER_BOUND('',#3098,.T.);
#1877=FACE_OUTER_BOUND('',#3099,.T.);
#1878=FACE_OUTER_BOUND('',#3100,.T.);
#1879=FACE_OUTER_BOUND('',#3101,.T.);
#1880=FACE_OUTER_BOUND('',#3102,.T.);
#1881=FACE_OUTER_BOUND('',#3103,.T.);
#1882=FACE_OUTER_BOUND('',#3104,.T.);
#1883=FACE_OUTER_BOUND('',#3105,.T.);
#1884=FACE_OUTER_BOUND('',#3106,.T.);
#1885=FACE_OUTER_BOUND('',#3107,.T.);
#1886=FACE_OUTER_BOUND('',#3108,.T.);
#1887=FACE_OUTER_BOUND('',#3109,.T.);
#1888=FACE_OUTER_BOUND('',#3110,.T.);
#1889=FACE_OUTER_BOUND('',#3111,.T.);
#1890=FACE_OUTER_BOUND('',#3112,.T.);
#1891=FACE_OUTER_BOUND('',#3113,.T.);
#1892=FACE_OUTER_BOUND('',#3114,.T.);
#1893=FACE_OUTER_BOUND('',#3115,.T.);
#1894=FACE_OUTER_BOUND('',#3116,.T.);
#1895=FACE_OUTER_BOUND('',#3117,.T.);
#1896=FACE_OUTER_BOUND('',#3118,.T.);
#1897=FACE_OUTER_BOUND('',#3119,.T.);
#1898=FACE_OUTER_BOUND('',#3120,.T.);
#1899=FACE_OUTER_BOUND('',#3121,.T.);
#1900=FACE_OUTER_BOUND('',#3122,.T.);
#1901=FACE_OUTER_BOUND('',#3123,.T.);
#1902=FACE_OUTER_BOUND('',#3124,.T.);
#1903=FACE_OUTER_BOUND('',#3125,.T.);
#1904=FACE_OUTER_BOUND('',#3126,.T.);
#1905=FACE_OUTER_BOUND('',#3127,.T.);
#1906=FACE_OUTER_BOUND('',#3128,.T.);
#1907=FACE_OUTER_BOUND('',#3129,.T.);
#1908=FACE_OUTER_BOUND('',#3130,.T.);
#1909=FACE_OUTER_BOUND('',#3131,.T.);
#1910=FACE_OUTER_BOUND('',#3132,.T.);
#1911=FACE_OUTER_BOUND('',#3133,.T.);
#1912=FACE_OUTER_BOUND('',#3134,.T.);
#1913=FACE_OUTER_BOUND('',#3135,.T.);
#1914=FACE_OUTER_BOUND('',#3136,.T.);
#1915=FACE_OUTER_BOUND('',#3137,.T.);
#1916=FACE_OUTER_BOUND('',#3138,.T.);
#1917=FACE_OUTER_BOUND('',#3139,.T.);
#1918=FACE_OUTER_BOUND('',#3140,.T.);
#1919=FACE_OUTER_BOUND('',#3141,.T.);
#1920=FACE_OUTER_BOUND('',#3142,.T.);
#1921=FACE_OUTER_BOUND('',#3143,.T.);
#1922=FACE_OUTER_BOUND('',#3144,.T.);
#1923=FACE_OUTER_BOUND('',#3145,.T.);
#1924=FACE_OUTER_BOUND('',#3146,.T.);
#1925=FACE_OUTER_BOUND('',#3147,.T.);
#1926=FACE_OUTER_BOUND('',#3148,.T.);
#1927=FACE_OUTER_BOUND('',#3149,.T.);
#1928=FACE_OUTER_BOUND('',#3150,.T.);
#1929=FACE_OUTER_BOUND('',#3151,.T.);
#1930=FACE_OUTER_BOUND('',#3152,.T.);
#1931=FACE_OUTER_BOUND('',#3153,.T.);
#1932=FACE_OUTER_BOUND('',#3154,.T.);
#1933=FACE_OUTER_BOUND('',#3155,.T.);
#1934=FACE_OUTER_BOUND('',#3156,.T.);
#1935=FACE_OUTER_BOUND('',#3157,.T.);
#1936=FACE_OUTER_BOUND('',#3158,.T.);
#1937=FACE_OUTER_BOUND('',#3159,.T.);
#1938=FACE_OUTER_BOUND('',#3160,.T.);
#1939=FACE_OUTER_BOUND('',#3161,.T.);
#1940=FACE_OUTER_BOUND('',#3162,.T.);
#1941=FACE_OUTER_BOUND('',#3163,.T.);
#1942=FACE_OUTER_BOUND('',#3164,.T.);
#1943=FACE_OUTER_BOUND('',#3165,.T.);
#1944=FACE_OUTER_BOUND('',#3166,.T.);
#1945=FACE_OUTER_BOUND('',#3167,.T.);
#1946=FACE_OUTER_BOUND('',#3168,.T.);
#1947=FACE_OUTER_BOUND('',#3169,.T.);
#1948=FACE_OUTER_BOUND('',#3170,.T.);
#1949=FACE_OUTER_BOUND('',#3171,.T.);
#1950=FACE_OUTER_BOUND('',#3172,.T.);
#1951=FACE_OUTER_BOUND('',#3173,.T.);
#1952=FACE_OUTER_BOUND('',#3174,.T.);
#1953=FACE_OUTER_BOUND('',#3175,.T.);
#1954=FACE_OUTER_BOUND('',#3176,.T.);
#1955=FACE_OUTER_BOUND('',#3177,.T.);
#1956=FACE_OUTER_BOUND('',#3178,.T.);
#1957=FACE_OUTER_BOUND('',#3179,.T.);
#1958=FACE_OUTER_BOUND('',#3180,.T.);
#1959=FACE_OUTER_BOUND('',#3181,.T.);
#1960=FACE_OUTER_BOUND('',#3182,.T.);
#1961=FACE_OUTER_BOUND('',#3183,.T.);
#1962=FACE_OUTER_BOUND('',#3184,.T.);
#1963=FACE_OUTER_BOUND('',#3185,.T.);
#1964=FACE_OUTER_BOUND('',#3186,.T.);
#1965=FACE_OUTER_BOUND('',#3187,.T.);
#1966=FACE_OUTER_BOUND('',#3188,.T.);
#1967=FACE_OUTER_BOUND('',#3189,.T.);
#1968=FACE_OUTER_BOUND('',#3190,.T.);
#1969=FACE_OUTER_BOUND('',#3191,.T.);
#1970=FACE_OUTER_BOUND('',#3192,.T.);
#1971=FACE_OUTER_BOUND('',#3193,.T.);
#1972=FACE_OUTER_BOUND('',#3194,.T.);
#1973=FACE_OUTER_BOUND('',#3195,.T.);
#1974=FACE_OUTER_BOUND('',#3196,.T.);
#1975=FACE_OUTER_BOUND('',#3197,.T.);
#1976=FACE_OUTER_BOUND('',#3198,.T.);
#1977=FACE_OUTER_BOUND('',#3199,.T.);
#2971=EDGE_LOOP('',(#15364,#15365,#15366,#15367,#15368));
#2972=EDGE_LOOP('',(#15369,#15370,#15371,#15372,#15373,#15374));
#2973=EDGE_LOOP('',(#15375,#15376,#15377,#15378,#15379,#15380,#15381,#15382,
#15383,#15384,#15385,#15386,#15387,#15388,#15389,#15390,#15391,#15392,#15393,
#15394,#15395,#15396,#15397,#15398,#15399,#15400,#15401,#15402,#15403,#15404,
#15405,#15406,#15407,#15408,#15409,#15410,#15411,#15412,#15413,#15414,#15415,
#15416,#15417,#15418,#15419,#15420,#15421,#15422,#15423,#15424,#15425,#15426,
#15427,#15428,#15429,#15430));
#2974=EDGE_LOOP('',(#15431));
#2975=EDGE_LOOP('',(#15432,#15433,#15434,#15435,#15436));
#2976=EDGE_LOOP('',(#15437,#15438,#15439,#15440,#15441,#15442,#15443,#15444,
#15445,#15446,#15447,#15448,#15449,#15450,#15451,#15452,#15453,#15454,#15455,
#15456,#15457,#15458,#15459,#15460,#15461,#15462,#15463,#15464,#15465,#15466,
#15467,#15468,#15469,#15470,#15471,#15472,#15473,#15474,#15475,#15476,#15477,
#15478,#15479,#15480,#15481,#15482,#15483,#15484,#15485,#15486,#15487,#15488,
#15489,#15490,#15491,#15492,#15493,#15494,#15495,#15496,#15497,#15498,#15499,
#15500,#15501,#15502,#15503,#15504,#15505,#15506,#15507,#15508,#15509,#15510,
#15511,#15512,#15513,#15514,#15515,#15516,#15517,#15518,#15519,#15520,#15521,
#15522,#15523,#15524,#15525,#15526,#15527,#15528,#15529,#15530,#15531,#15532,
#15533,#15534,#15535,#15536));
#2977=EDGE_LOOP('',(#15537));
#2978=EDGE_LOOP('',(#15538,#15539,#15540,#15541,#15542));
#2979=EDGE_LOOP('',(#15543,#15544,#15545,#15546));
#2980=EDGE_LOOP('',(#15547,#15548,#15549,#15550,#15551));
#2981=EDGE_LOOP('',(#15552,#15553,#15554,#15555));
#2982=EDGE_LOOP('',(#15556,#15557,#15558,#15559));
#2983=EDGE_LOOP('',(#15560,#15561,#15562,#15563,#15564));
#2984=EDGE_LOOP('',(#15565,#15566,#15567,#15568));
#2985=EDGE_LOOP('',(#15569,#15570,#15571,#15572,#15573));
#2986=EDGE_LOOP('',(#15574,#15575,#15576,#15577,#15578,#15579,#15580,#15581,
#15582,#15583,#15584,#15585,#15586,#15587,#15588,#15589,#15590,#15591,#15592,
#15593,#15594,#15595,#15596,#15597,#15598,#15599,#15600,#15601,#15602,#15603,
#15604,#15605,#15606,#15607,#15608,#15609,#15610,#15611,#15612,#15613,#15614,
#15615,#15616,#15617,#15618,#15619,#15620,#15621,#15622,#15623,#15624,#15625,
#15626,#15627,#15628,#15629,#15630,#15631,#15632,#15633,#15634,#15635,#15636,
#15637,#15638,#15639,#15640,#15641,#15642,#15643,#15644,#15645,#15646,#15647,
#15648,#15649,#15650,#15651,#15652,#15653,#15654,#15655,#15656,#15657,#15658,
#15659,#15660,#15661,#15662,#15663,#15664,#15665,#15666,#15667,#15668,#15669,
#15670,#15671,#15672,#15673));
#2987=EDGE_LOOP('',(#15674,#15675,#15676,#15677,#15678,#15679,#15680,#15681,
#15682,#15683,#15684,#15685,#15686,#15687,#15688,#15689,#15690,#15691,#15692,
#15693,#15694,#15695,#15696,#15697,#15698,#15699,#15700,#15701,#15702,#15703,
#15704,#15705,#15706,#15707,#15708,#15709,#15710,#15711,#15712,#15713,#15714,
#15715,#15716,#15717,#15718,#15719,#15720,#15721,#15722,#15723,#15724,#15725,
#15726,#15727,#15728,#15729));
#2988=EDGE_LOOP('',(#15730,#15731,#15732,#15733));
#2989=EDGE_LOOP('',(#15734,#15735,#15736,#15737));
#2990=EDGE_LOOP('',(#15738,#15739,#15740,#15741,#15742));
#2991=EDGE_LOOP('',(#15743,#15744,#15745,#15746));
#2992=EDGE_LOOP('',(#15747,#15748,#15749,#15750,#15751));
#2993=EDGE_LOOP('',(#15752,#15753,#15754,#15755));
#2994=EDGE_LOOP('',(#15756,#15757,#15758,#15759));
#2995=EDGE_LOOP('',(#15760,#15761,#15762,#15763,#15764));
#2996=EDGE_LOOP('',(#15765,#15766,#15767,#15768));
#2997=EDGE_LOOP('',(#15769,#15770,#15771,#15772,#15773));
#2998=EDGE_LOOP('',(#15774,#15775,#15776,#15777));
#2999=EDGE_LOOP('',(#15778,#15779,#15780,#15781));
#3000=EDGE_LOOP('',(#15782,#15783,#15784,#15785,#15786));
#3001=EDGE_LOOP('',(#15787,#15788,#15789,#15790));
#3002=EDGE_LOOP('',(#15791,#15792,#15793,#15794,#15795));
#3003=EDGE_LOOP('',(#15796,#15797,#15798,#15799));
#3004=EDGE_LOOP('',(#15800,#15801,#15802,#15803));
#3005=EDGE_LOOP('',(#15804,#15805,#15806,#15807,#15808));
#3006=EDGE_LOOP('',(#15809,#15810,#15811,#15812));
#3007=EDGE_LOOP('',(#15813,#15814,#15815,#15816,#15817));
#3008=EDGE_LOOP('',(#15818,#15819,#15820,#15821));
#3009=EDGE_LOOP('',(#15822,#15823,#15824,#15825));
#3010=EDGE_LOOP('',(#15826,#15827,#15828,#15829,#15830));
#3011=EDGE_LOOP('',(#15831,#15832,#15833,#15834));
#3012=EDGE_LOOP('',(#15835,#15836,#15837,#15838,#15839));
#3013=EDGE_LOOP('',(#15840,#15841,#15842,#15843));
#3014=EDGE_LOOP('',(#15844,#15845,#15846,#15847));
#3015=EDGE_LOOP('',(#15848,#15849,#15850,#15851,#15852));
#3016=EDGE_LOOP('',(#15853,#15854,#15855,#15856));
#3017=EDGE_LOOP('',(#15857,#15858,#15859,#15860,#15861));
#3018=EDGE_LOOP('',(#15862,#15863,#15864,#15865));
#3019=EDGE_LOOP('',(#15866,#15867,#15868,#15869));
#3020=EDGE_LOOP('',(#15870,#15871,#15872,#15873,#15874));
#3021=EDGE_LOOP('',(#15875,#15876,#15877,#15878));
#3022=EDGE_LOOP('',(#15879,#15880,#15881,#15882,#15883));
#3023=EDGE_LOOP('',(#15884,#15885,#15886,#15887));
#3024=EDGE_LOOP('',(#15888,#15889,#15890,#15891));
#3025=EDGE_LOOP('',(#15892,#15893,#15894,#15895,#15896));
#3026=EDGE_LOOP('',(#15897,#15898,#15899,#15900));
#3027=EDGE_LOOP('',(#15901,#15902,#15903,#15904,#15905));
#3028=EDGE_LOOP('',(#15906,#15907,#15908,#15909));
#3029=EDGE_LOOP('',(#15910,#15911,#15912,#15913));
#3030=EDGE_LOOP('',(#15914,#15915,#15916,#15917,#15918));
#3031=EDGE_LOOP('',(#15919,#15920,#15921,#15922));
#3032=EDGE_LOOP('',(#15923,#15924,#15925,#15926,#15927));
#3033=EDGE_LOOP('',(#15928,#15929,#15930,#15931));
#3034=EDGE_LOOP('',(#15932,#15933,#15934,#15935));
#3035=EDGE_LOOP('',(#15936,#15937,#15938,#15939,#15940));
#3036=EDGE_LOOP('',(#15941,#15942,#15943,#15944));
#3037=EDGE_LOOP('',(#15945,#15946,#15947,#15948,#15949));
#3038=EDGE_LOOP('',(#15950,#15951,#15952,#15953));
#3039=EDGE_LOOP('',(#15954,#15955,#15956,#15957));
#3040=EDGE_LOOP('',(#15958,#15959,#15960,#15961,#15962));
#3041=EDGE_LOOP('',(#15963,#15964,#15965,#15966));
#3042=EDGE_LOOP('',(#15967,#15968,#15969,#15970,#15971));
#3043=EDGE_LOOP('',(#15972,#15973,#15974,#15975));
#3044=EDGE_LOOP('',(#15976,#15977,#15978,#15979));
#3045=EDGE_LOOP('',(#15980,#15981,#15982,#15983,#15984));
#3046=EDGE_LOOP('',(#15985,#15986,#15987,#15988));
#3047=EDGE_LOOP('',(#15989,#15990,#15991,#15992,#15993));
#3048=EDGE_LOOP('',(#15994,#15995,#15996,#15997,#15998,#15999));
#3049=EDGE_LOOP('',(#16000,#16001,#16002,#16003));
#3050=EDGE_LOOP('',(#16004,#16005,#16006,#16007,#16008,#16009));
#3051=EDGE_LOOP('',(#16010,#16011,#16012,#16013));
#3052=EDGE_LOOP('',(#16014,#16015,#16016,#16017));
#3053=EDGE_LOOP('',(#16018,#16019,#16020,#16021));
#3054=EDGE_LOOP('',(#16022,#16023,#16024,#16025,#16026,#16027));
#3055=EDGE_LOOP('',(#16028,#16029,#16030,#16031));
#3056=EDGE_LOOP('',(#16032,#16033,#16034,#16035,#16036,#16037));
#3057=EDGE_LOOP('',(#16038,#16039,#16040,#16041));
#3058=EDGE_LOOP('',(#16042,#16043,#16044,#16045));
#3059=EDGE_LOOP('',(#16046,#16047,#16048,#16049));
#3060=EDGE_LOOP('',(#16050,#16051,#16052,#16053,#16054,#16055));
#3061=EDGE_LOOP('',(#16056,#16057,#16058,#16059));
#3062=EDGE_LOOP('',(#16060,#16061,#16062,#16063,#16064,#16065));
#3063=EDGE_LOOP('',(#16066,#16067,#16068,#16069));
#3064=EDGE_LOOP('',(#16070,#16071,#16072,#16073));
#3065=EDGE_LOOP('',(#16074,#16075,#16076,#16077));
#3066=EDGE_LOOP('',(#16078,#16079,#16080,#16081,#16082,#16083));
#3067=EDGE_LOOP('',(#16084,#16085,#16086,#16087));
#3068=EDGE_LOOP('',(#16088,#16089,#16090,#16091,#16092,#16093));
#3069=EDGE_LOOP('',(#16094,#16095,#16096,#16097));
#3070=EDGE_LOOP('',(#16098,#16099,#16100,#16101));
#3071=EDGE_LOOP('',(#16102,#16103,#16104,#16105));
#3072=EDGE_LOOP('',(#16106,#16107,#16108,#16109,#16110,#16111));
#3073=EDGE_LOOP('',(#16112,#16113,#16114,#16115));
#3074=EDGE_LOOP('',(#16116,#16117,#16118,#16119,#16120,#16121));
#3075=EDGE_LOOP('',(#16122,#16123,#16124,#16125));
#3076=EDGE_LOOP('',(#16126,#16127,#16128,#16129));
#3077=EDGE_LOOP('',(#16130,#16131,#16132,#16133));
#3078=EDGE_LOOP('',(#16134,#16135,#16136,#16137,#16138,#16139));
#3079=EDGE_LOOP('',(#16140,#16141,#16142,#16143));
#3080=EDGE_LOOP('',(#16144,#16145,#16146,#16147,#16148,#16149));
#3081=EDGE_LOOP('',(#16150,#16151,#16152,#16153));
#3082=EDGE_LOOP('',(#16154,#16155,#16156,#16157));
#3083=EDGE_LOOP('',(#16158,#16159,#16160,#16161));
#3084=EDGE_LOOP('',(#16162,#16163,#16164,#16165,#16166,#16167));
#3085=EDGE_LOOP('',(#16168,#16169,#16170,#16171));
#3086=EDGE_LOOP('',(#16172,#16173,#16174,#16175,#16176,#16177));
#3087=EDGE_LOOP('',(#16178,#16179,#16180,#16181));
#3088=EDGE_LOOP('',(#16182,#16183,#16184,#16185));
#3089=EDGE_LOOP('',(#16186,#16187,#16188,#16189));
#3090=EDGE_LOOP('',(#16190,#16191,#16192,#16193,#16194,#16195));
#3091=EDGE_LOOP('',(#16196,#16197,#16198,#16199));
#3092=EDGE_LOOP('',(#16200,#16201,#16202,#16203,#16204,#16205));
#3093=EDGE_LOOP('',(#16206,#16207,#16208,#16209));
#3094=EDGE_LOOP('',(#16210,#16211,#16212,#16213));
#3095=EDGE_LOOP('',(#16214,#16215,#16216,#16217));
#3096=EDGE_LOOP('',(#16218,#16219,#16220,#16221,#16222,#16223));
#3097=EDGE_LOOP('',(#16224,#16225,#16226,#16227));
#3098=EDGE_LOOP('',(#16228,#16229,#16230,#16231,#16232,#16233));
#3099=EDGE_LOOP('',(#16234,#16235,#16236,#16237));
#3100=EDGE_LOOP('',(#16238,#16239,#16240,#16241));
#3101=EDGE_LOOP('',(#16242,#16243,#16244,#16245));
#3102=EDGE_LOOP('',(#16246,#16247,#16248,#16249,#16250,#16251));
#3103=EDGE_LOOP('',(#16252,#16253,#16254,#16255));
#3104=EDGE_LOOP('',(#16256,#16257,#16258,#16259,#16260,#16261));
#3105=EDGE_LOOP('',(#16262,#16263,#16264,#16265));
#3106=EDGE_LOOP('',(#16266,#16267,#16268,#16269));
#3107=EDGE_LOOP('',(#16270,#16271,#16272,#16273));
#3108=EDGE_LOOP('',(#16274,#16275,#16276,#16277,#16278,#16279));
#3109=EDGE_LOOP('',(#16280,#16281,#16282,#16283));
#3110=EDGE_LOOP('',(#16284,#16285,#16286,#16287,#16288,#16289));
#3111=EDGE_LOOP('',(#16290,#16291,#16292,#16293));
#3112=EDGE_LOOP('',(#16294,#16295,#16296,#16297));
#3113=EDGE_LOOP('',(#16298,#16299,#16300,#16301));
#3114=EDGE_LOOP('',(#16302,#16303,#16304,#16305,#16306,#16307));
#3115=EDGE_LOOP('',(#16308,#16309,#16310,#16311));
#3116=EDGE_LOOP('',(#16312,#16313,#16314,#16315,#16316,#16317));
#3117=EDGE_LOOP('',(#16318,#16319,#16320,#16321));
#3118=EDGE_LOOP('',(#16322,#16323,#16324,#16325));
#3119=EDGE_LOOP('',(#16326,#16327,#16328,#16329));
#3120=EDGE_LOOP('',(#16330,#16331,#16332,#16333,#16334,#16335));
#3121=EDGE_LOOP('',(#16336,#16337,#16338,#16339));
#3122=EDGE_LOOP('',(#16340,#16341,#16342,#16343,#16344,#16345));
#3123=EDGE_LOOP('',(#16346,#16347,#16348,#16349));
#3124=EDGE_LOOP('',(#16350,#16351,#16352,#16353));
#3125=EDGE_LOOP('',(#16354,#16355,#16356,#16357));
#3126=EDGE_LOOP('',(#16358,#16359,#16360,#16361,#16362,#16363));
#3127=EDGE_LOOP('',(#16364,#16365,#16366,#16367));
#3128=EDGE_LOOP('',(#16368,#16369,#16370,#16371,#16372,#16373));
#3129=EDGE_LOOP('',(#16374,#16375,#16376,#16377));
#3130=EDGE_LOOP('',(#16378,#16379,#16380,#16381));
#3131=EDGE_LOOP('',(#16382,#16383,#16384,#16385));
#3132=EDGE_LOOP('',(#16386,#16387,#16388,#16389,#16390,#16391));
#3133=EDGE_LOOP('',(#16392,#16393,#16394,#16395));
#3134=EDGE_LOOP('',(#16396,#16397,#16398,#16399,#16400,#16401));
#3135=EDGE_LOOP('',(#16402,#16403,#16404,#16405));
#3136=EDGE_LOOP('',(#16406,#16407,#16408,#16409));
#3137=EDGE_LOOP('',(#16410,#16411,#16412,#16413));
#3138=EDGE_LOOP('',(#16414,#16415,#16416,#16417,#16418,#16419));
#3139=EDGE_LOOP('',(#16420,#16421,#16422,#16423));
#3140=EDGE_LOOP('',(#16424,#16425,#16426,#16427,#16428,#16429));
#3141=EDGE_LOOP('',(#16430,#16431,#16432,#16433));
#3142=EDGE_LOOP('',(#16434,#16435,#16436,#16437));
#3143=EDGE_LOOP('',(#16438,#16439,#16440,#16441));
#3144=EDGE_LOOP('',(#16442,#16443,#16444,#16445,#16446,#16447));
#3145=EDGE_LOOP('',(#16448,#16449,#16450,#16451));
#3146=EDGE_LOOP('',(#16452,#16453,#16454,#16455,#16456,#16457));
#3147=EDGE_LOOP('',(#16458,#16459,#16460,#16461));
#3148=EDGE_LOOP('',(#16462,#16463,#16464,#16465));
#3149=EDGE_LOOP('',(#16466,#16467,#16468,#16469));
#3150=EDGE_LOOP('',(#16470,#16471,#16472,#16473,#16474,#16475));
#3151=EDGE_LOOP('',(#16476,#16477,#16478,#16479));
#3152=EDGE_LOOP('',(#16480,#16481,#16482,#16483,#16484,#16485));
#3153=EDGE_LOOP('',(#16486,#16487,#16488,#16489));
#3154=EDGE_LOOP('',(#16490,#16491,#16492,#16493));
#3155=EDGE_LOOP('',(#16494,#16495,#16496,#16497));
#3156=EDGE_LOOP('',(#16498,#16499,#16500,#16501,#16502,#16503));
#3157=EDGE_LOOP('',(#16504,#16505,#16506,#16507));
#3158=EDGE_LOOP('',(#16508,#16509,#16510,#16511,#16512,#16513));
#3159=EDGE_LOOP('',(#16514,#16515,#16516,#16517));
#3160=EDGE_LOOP('',(#16518,#16519,#16520,#16521));
#3161=EDGE_LOOP('',(#16522,#16523,#16524,#16525));
#3162=EDGE_LOOP('',(#16526,#16527,#16528,#16529,#16530,#16531));
#3163=EDGE_LOOP('',(#16532,#16533,#16534,#16535));
#3164=EDGE_LOOP('',(#16536,#16537,#16538,#16539,#16540,#16541));
#3165=EDGE_LOOP('',(#16542,#16543,#16544,#16545));
#3166=EDGE_LOOP('',(#16546,#16547,#16548,#16549));
#3167=EDGE_LOOP('',(#16550,#16551,#16552,#16553));
#3168=EDGE_LOOP('',(#16554,#16555,#16556,#16557,#16558,#16559));
#3169=EDGE_LOOP('',(#16560,#16561,#16562,#16563));
#3170=EDGE_LOOP('',(#16564,#16565,#16566,#16567,#16568,#16569));
#3171=EDGE_LOOP('',(#16570,#16571,#16572,#16573));
#3172=EDGE_LOOP('',(#16574,#16575,#16576,#16577));
#3173=EDGE_LOOP('',(#16578,#16579,#16580,#16581));
#3174=EDGE_LOOP('',(#16582,#16583,#16584,#16585,#16586,#16587));
#3175=EDGE_LOOP('',(#16588,#16589,#16590,#16591));
#3176=EDGE_LOOP('',(#16592,#16593,#16594,#16595,#16596,#16597));
#3177=EDGE_LOOP('',(#16598,#16599,#16600,#16601));
#3178=EDGE_LOOP('',(#16602,#16603,#16604,#16605));
#3179=EDGE_LOOP('',(#16606,#16607,#16608,#16609));
#3180=EDGE_LOOP('',(#16610,#16611,#16612,#16613,#16614,#16615));
#3181=EDGE_LOOP('',(#16616,#16617,#16618,#16619));
#3182=EDGE_LOOP('',(#16620,#16621,#16622,#16623,#16624,#16625));
#3183=EDGE_LOOP('',(#16626,#16627,#16628,#16629));
#3184=EDGE_LOOP('',(#16630,#16631,#16632,#16633));
#3185=EDGE_LOOP('',(#16634,#16635,#16636,#16637));
#3186=EDGE_LOOP('',(#16638,#16639,#16640,#16641,#16642,#16643));
#3187=EDGE_LOOP('',(#16644,#16645,#16646,#16647));
#3188=EDGE_LOOP('',(#16648,#16649,#16650,#16651,#16652,#16653));
#3189=EDGE_LOOP('',(#16654,#16655,#16656,#16657));
#3190=EDGE_LOOP('',(#16658,#16659,#16660,#16661));
#3191=EDGE_LOOP('',(#16662,#16663,#16664,#16665));
#3192=EDGE_LOOP('',(#16666,#16667,#16668,#16669,#16670,#16671));
#3193=EDGE_LOOP('',(#16672,#16673,#16674,#16675));
#3194=EDGE_LOOP('',(#16676,#16677,#16678,#16679,#16680,#16681));
#3195=EDGE_LOOP('',(#16682,#16683,#16684,#16685));
#3196=EDGE_LOOP('',(#16686,#16687,#16688,#16689));
#3197=EDGE_LOOP('',(#16690,#16691,#16692,#16693));
#3198=EDGE_LOOP('',(#16694,#16695,#16696,#16697));
#3199=EDGE_LOOP('',(#16698,#16699,#16700,#16701));
#4076=CIRCLE('',#21300,3.03);
#4077=CIRCLE('',#21301,3.03);
#4078=CIRCLE('',#21302,3.33);
#4079=CIRCLE('',#21304,3.03);
#4080=CIRCLE('',#21305,3.03);
#4081=CIRCLE('',#21307,7.1875);
#4082=CIRCLE('',#21308,9.5);
#4083=CIRCLE('',#21309,7.1875);
#4084=CIRCLE('',#21310,9.5);
#4085=CIRCLE('',#21311,7.1875);
#4086=CIRCLE('',#21312,9.5);
#4087=CIRCLE('',#21313,7.1875);
#4088=CIRCLE('',#21314,9.5);
#4089=CIRCLE('',#21315,7.1875);
#4090=CIRCLE('',#21316,9.5);
#4091=CIRCLE('',#21317,7.1875);
#4092=CIRCLE('',#21318,9.5);
#4093=CIRCLE('',#21319,7.1875);
#4094=CIRCLE('',#21320,9.5);
#4095=CIRCLE('',#21321,7.1875);
#4096=CIRCLE('',#21322,9.5);
#4097=CIRCLE('',#21323,7.1875);
#4098=CIRCLE('',#21324,9.5);
#4099=CIRCLE('',#21325,7.1875);
#4100=CIRCLE('',#21326,9.5);
#4101=CIRCLE('',#21327,7.1875);
#4102=CIRCLE('',#21328,9.5);
#4103=CIRCLE('',#21329,7.1875);
#4104=CIRCLE('',#21330,9.5);
#4105=CIRCLE('',#21331,7.1875);
#4106=CIRCLE('',#21332,9.5);
#4107=CIRCLE('',#21333,7.1875);
#4108=CIRCLE('',#21334,9.5);
#4109=CIRCLE('',#21336,3.33);
#4110=CIRCLE('',#21338,14.0625);
#4111=CIRCLE('',#21339,16.375);
#4112=CIRCLE('',#21340,14.0625);
#4113=CIRCLE('',#21341,16.375);
#4114=CIRCLE('',#21342,14.0625);
#4115=CIRCLE('',#21343,16.375);
#4116=CIRCLE('',#21344,14.0625);
#4117=CIRCLE('',#21345,16.375);
#4118=CIRCLE('',#21346,14.0625);
#4119=CIRCLE('',#21347,16.375);
#4120=CIRCLE('',#21348,14.0625);
#4121=CIRCLE('',#21349,16.375);
#4122=CIRCLE('',#21350,14.0625);
#4123=CIRCLE('',#21351,16.375);
#4124=CIRCLE('',#21352,14.0625);
#4125=CIRCLE('',#21353,16.375);
#4126=CIRCLE('',#21354,14.0625);
#4127=CIRCLE('',#21355,16.375);
#4128=CIRCLE('',#21356,14.0625);
#4129=CIRCLE('',#21357,16.375);
#4130=CIRCLE('',#21358,14.0625);
#4131=CIRCLE('',#21359,16.375);
#4132=CIRCLE('',#21360,14.0625);
#4133=CIRCLE('',#21361,16.375);
#4134=CIRCLE('',#21362,14.0625);
#4135=CIRCLE('',#21363,16.375);
#4136=CIRCLE('',#21364,14.0625);
#4137=CIRCLE('',#21365,16.375);
#4138=CIRCLE('',#21366,14.0625);
#4139=CIRCLE('',#21367,16.375);
#4140=CIRCLE('',#21368,14.0625);
#4141=CIRCLE('',#21369,16.375);
#4142=CIRCLE('',#21370,14.0625);
#4143=CIRCLE('',#21371,16.375);
#4144=CIRCLE('',#21372,14.0625);
#4145=CIRCLE('',#21373,16.375);
#4146=CIRCLE('',#21374,14.0625);
#4147=CIRCLE('',#21375,16.375);
#4148=CIRCLE('',#21376,14.0625);
#4149=CIRCLE('',#21377,16.375);
#4150=CIRCLE('',#21378,14.0625);
#4151=CIRCLE('',#21379,16.375);
#4152=CIRCLE('',#21380,14.0625);
#4153=CIRCLE('',#21381,16.375);
#4154=CIRCLE('',#21382,14.0625);
#4155=CIRCLE('',#21383,16.375);
#4156=CIRCLE('',#21384,14.0625);
#4157=CIRCLE('',#21385,16.375);
#4158=CIRCLE('',#21386,14.0625);
#4159=CIRCLE('',#21387,16.375);
#4160=CIRCLE('',#21389,7.1875);
#4161=CIRCLE('',#21391,10.);
#4162=CIRCLE('',#21393,10.);
#4163=CIRCLE('',#21395,7.1875);
#4164=CIRCLE('',#21397,16.375);
#4165=CIRCLE('',#21398,14.0625);
#4166=CIRCLE('',#21399,16.375);
#4167=CIRCLE('',#21400,14.0625);
#4168=CIRCLE('',#21401,16.375);
#4169=CIRCLE('',#21402,14.0625);
#4170=CIRCLE('',#21403,16.375);
#4171=CIRCLE('',#21404,14.0625);
#4172=CIRCLE('',#21405,16.375);
#4173=CIRCLE('',#21406,14.0625);
#4174=CIRCLE('',#21407,16.375);
#4175=CIRCLE('',#21408,14.0625);
#4176=CIRCLE('',#21409,16.375);
#4177=CIRCLE('',#21410,14.0625);
#4178=CIRCLE('',#21411,16.375);
#4179=CIRCLE('',#21412,14.0625);
#4180=CIRCLE('',#21413,16.375);
#4181=CIRCLE('',#21414,14.0625);
#4182=CIRCLE('',#21415,16.375);
#4183=CIRCLE('',#21416,14.0625);
#4184=CIRCLE('',#21417,16.375);
#4185=CIRCLE('',#21418,14.0625);
#4186=CIRCLE('',#21419,16.375);
#4187=CIRCLE('',#21420,14.0625);
#4188=CIRCLE('',#21421,16.375);
#4189=CIRCLE('',#21422,14.0625);
#4190=CIRCLE('',#21423,16.375);
#4191=CIRCLE('',#21424,14.0625);
#4192=CIRCLE('',#21425,16.375);
#4193=CIRCLE('',#21426,14.0625);
#4194=CIRCLE('',#21427,16.375);
#4195=CIRCLE('',#21428,14.0625);
#4196=CIRCLE('',#21429,16.375);
#4197=CIRCLE('',#21430,14.0625);
#4198=CIRCLE('',#21431,16.375);
#4199=CIRCLE('',#21432,14.0625);
#4200=CIRCLE('',#21433,16.375);
#4201=CIRCLE('',#21434,14.0625);
#4202=CIRCLE('',#21435,16.375);
#4203=CIRCLE('',#21436,14.0625);
#4204=CIRCLE('',#21437,16.375);
#4205=CIRCLE('',#21438,14.0625);
#4206=CIRCLE('',#21439,16.375);
#4207=CIRCLE('',#21440,14.0625);
#4208=CIRCLE('',#21441,16.375);
#4209=CIRCLE('',#21442,14.0625);
#4210=CIRCLE('',#21443,16.375);
#4211=CIRCLE('',#21444,14.0625);
#4212=CIRCLE('',#21445,16.375);
#4213=CIRCLE('',#21446,14.0625);
#4214=CIRCLE('',#21447,10.);
#4215=CIRCLE('',#21448,10.);
#4216=CIRCLE('',#21449,7.1875);
#4217=CIRCLE('',#21450,10.);
#4218=CIRCLE('',#21451,7.1875);
#4219=CIRCLE('',#21452,10.);
#4220=CIRCLE('',#21453,7.1875);
#4221=CIRCLE('',#21454,10.);
#4222=CIRCLE('',#21455,7.1875);
#4223=CIRCLE('',#21456,10.);
#4224=CIRCLE('',#21457,7.1875);
#4225=CIRCLE('',#21458,10.);
#4226=CIRCLE('',#21459,7.1875);
#4227=CIRCLE('',#21460,10.);
#4228=CIRCLE('',#21461,7.1875);
#4229=CIRCLE('',#21462,10.);
#4230=CIRCLE('',#21463,7.1875);
#4231=CIRCLE('',#21464,10.);
#4232=CIRCLE('',#21465,7.1875);
#4233=CIRCLE('',#21466,10.);
#4234=CIRCLE('',#21467,7.1875);
#4235=CIRCLE('',#21468,10.);
#4236=CIRCLE('',#21469,7.1875);
#4237=CIRCLE('',#21470,10.);
#4238=CIRCLE('',#21471,7.1875);
#4239=CIRCLE('',#21473,10.);
#4240=CIRCLE('',#21477,10.);
#4241=CIRCLE('',#21481,10.);
#4242=CIRCLE('',#21485,10.);
#4243=CIRCLE('',#21489,10.);
#4244=CIRCLE('',#21493,10.);
#4245=CIRCLE('',#21497,10.);
#4246=CIRCLE('',#21501,10.);
#4247=CIRCLE('',#21505,10.);
#4248=CIRCLE('',#21509,10.);
#4249=CIRCLE('',#21513,10.);
#4250=CIRCLE('',#21517,10.);
#4251=CIRCLE('',#21522,16.875);
#4252=CIRCLE('',#21524,16.875);
#4253=CIRCLE('',#21528,16.875);
#4254=CIRCLE('',#21530,16.875);
#4255=CIRCLE('',#21534,16.875);
#4256=CIRCLE('',#21536,16.875);
#4257=CIRCLE('',#21540,16.875);
#4258=CIRCLE('',#21542,16.875);
#4259=CIRCLE('',#21546,16.875);
#4260=CIRCLE('',#21548,16.875);
#4261=CIRCLE('',#21552,16.875);
#4262=CIRCLE('',#21554,16.875);
#4263=CIRCLE('',#21558,16.875);
#4264=CIRCLE('',#21560,16.875);
#4265=CIRCLE('',#21564,16.875);
#4266=CIRCLE('',#21566,16.875);
#4267=CIRCLE('',#21570,16.875);
#4268=CIRCLE('',#21572,16.875);
#4269=CIRCLE('',#21576,16.875);
#4270=CIRCLE('',#21578,16.875);
#4271=CIRCLE('',#21582,16.875);
#4272=CIRCLE('',#21584,16.875);
#4273=CIRCLE('',#21588,16.875);
#4274=CIRCLE('',#21590,16.875);
#4275=CIRCLE('',#21594,16.875);
#4276=CIRCLE('',#21596,16.875);
#4277=CIRCLE('',#21600,16.875);
#4278=CIRCLE('',#21602,16.875);
#4279=CIRCLE('',#21606,16.875);
#4280=CIRCLE('',#21608,16.875);
#4281=CIRCLE('',#21612,16.875);
#4282=CIRCLE('',#21614,16.875);
#4283=CIRCLE('',#21618,16.875);
#4284=CIRCLE('',#21620,16.875);
#4285=CIRCLE('',#21624,16.875);
#4286=CIRCLE('',#21626,16.875);
#4287=CIRCLE('',#21630,16.875);
#4288=CIRCLE('',#21632,16.875);
#4289=CIRCLE('',#21636,16.875);
#4290=CIRCLE('',#21638,16.875);
#4291=CIRCLE('',#21642,16.875);
#4292=CIRCLE('',#21644,16.875);
#4293=CIRCLE('',#21648,16.875);
#4294=CIRCLE('',#21650,16.875);
#4295=CIRCLE('',#21654,16.875);
#4296=CIRCLE('',#21656,16.875);
#4297=CIRCLE('',#21660,16.875);
#4298=CIRCLE('',#21662,16.875);
#4299=CIRCLE('',#21666,16.875);
#4300=CIRCLE('',#21668,16.875);
#4301=CIRCLE('',#21671,10.);
#5142=B_SPLINE_CURVE_WITH_KNOTS('',3,(#51694,#51695,#51696,#51697,#51698,
#51699,#51700),.UNSPECIFIED.,.F.,.F.,(4,3,4),(0.,0.0297140756221973,0.0782401718747037),
 .UNSPECIFIED.);
#5143=B_SPLINE_CURVE_WITH_KNOTS('',3,(#51738,#51739,#51740,#51741,#51742,
#51743),.UNSPECIFIED.,.F.,.F.,(4,2,4),(0.,1.45,2.85),.UNSPECIFIED.);
#5144=B_SPLINE_CURVE_WITH_KNOTS('',3,(#51829,#51830,#51831,#51832,#51833,
#51834),.UNSPECIFIED.,.F.,.F.,(4,2,4),(0.924746809899207,0.981018841216537,
1.21342818548362),.UNSPECIFIED.);
#5145=B_SPLINE_CURVE_WITH_KNOTS('',3,(#51836,#51837,#51838,#51839,#51840,
#51841),.UNSPECIFIED.,.F.,.F.,(4,2,4),(0.,1.45,2.85),.UNSPECIFIED.);
#5146=B_SPLINE_CURVE_WITH_KNOTS('',3,(#51874,#51875,#51876,#51877,#51878,
#51879),.UNSPECIFIED.,.F.,.F.,(4,2,4),(0.924746809879486,0.981018841193929,
1.21342818544405),.UNSPECIFIED.);
#5147=B_SPLINE_CURVE_WITH_KNOTS('',3,(#51883,#51884,#51885,#51886,#51887,
#51888),.UNSPECIFIED.,.F.,.F.,(4,2,4),(0.,1.45,2.85),.UNSPECIFIED.);
#5148=B_SPLINE_CURVE_WITH_KNOTS('',3,(#51971,#51972,#51973,#51974,#51975,
#51976),.UNSPECIFIED.,.F.,.F.,(4,2,4),(0.,1.45,2.85),.UNSPECIFIED.);
#5149=B_SPLINE_CURVE_WITH_KNOTS('',3,(#52008,#52009,#52010,#52011,#52012,
#52013),.UNSPECIFIED.,.F.,.F.,(4,2,4),(0.924746809888898,0.981018841204197,
1.21342818545661),.UNSPECIFIED.);
#5150=B_SPLINE_CURVE_WITH_KNOTS('',3,(#52100,#52101,#52102,#52103,#52104,
#52105),.UNSPECIFIED.,.F.,.F.,(4,2,4),(0.,1.45,2.85),.UNSPECIFIED.);
#5151=B_SPLINE_CURVE_WITH_KNOTS('',3,(#52106,#52107,#52108,#52109),
 .UNSPECIFIED.,.F.,.F.,(4,4),(0.,0.0536817275864003),.UNSPECIFIED.);
#5152=B_SPLINE_CURVE_WITH_KNOTS('',3,(#54501,#54502,#54503,#54504,#54505,
#54506),.UNSPECIFIED.,.F.,.F.,(4,2,4),(0.,1.45,2.85),.UNSPECIFIED.);
#5153=B_SPLINE_CURVE_WITH_KNOTS('',3,(#54508,#54509,#54510,#54511),
 .UNSPECIFIED.,.F.,.F.,(4,4),(0.,0.0536817275781464),.UNSPECIFIED.);
#5154=B_SPLINE_CURVE_WITH_KNOTS('',3,(#54676,#54677,#54678,#54679,#54680,
#54681),.UNSPECIFIED.,.F.,.F.,(4,2,4),(0.924746809879285,0.981018841193106,
1.21342818543858),.UNSPECIFIED.);
#5155=B_SPLINE_CURVE_WITH_KNOTS('',3,(#54682,#54683,#54684,#54685,#54686,
#54687),.UNSPECIFIED.,.F.,.F.,(4,2,4),(0.,1.45,2.85),.UNSPECIFIED.);
#5156=B_SPLINE_CURVE_WITH_KNOTS('',3,(#54772,#54773,#54774,#54775,#54776,
#54777),.UNSPECIFIED.,.F.,.F.,(4,2,4),(0.,1.45,2.85),.UNSPECIFIED.);
#5157=B_SPLINE_CURVE_WITH_KNOTS('',3,(#54779,#54780,#54781,#54782,#54783,
#54784),.UNSPECIFIED.,.F.,.F.,(4,2,4),(0.0895985967037025,0.107791487575302,
0.178841206013496),.UNSPECIFIED.);
#5158=B_SPLINE_CURVE_WITH_KNOTS('',3,(#54868,#54869,#54870,#54871,#54872,
#54873),.UNSPECIFIED.,.F.,.F.,(4,2,4),(0.,1.45,2.85),.UNSPECIFIED.);
#5159=B_SPLINE_CURVE_WITH_KNOTS('',3,(#54874,#54875,#54876,#54877),
 .UNSPECIFIED.,.F.,.F.,(4,4),(0.,0.0782778812827931),.UNSPECIFIED.);
#5160=B_SPLINE_CURVE_WITH_KNOTS('',3,(#54881,#54882,#54883,#54884,#54885,
#54886),.UNSPECIFIED.,.F.,.F.,(4,2,4),(0.,1.45,2.85),.UNSPECIFIED.);
#5161=B_SPLINE_CURVE_WITH_KNOTS('',3,(#54888,#54889,#54890,#54891,#54892,
#54893,#54894,#54895,#54896,#54897),.UNSPECIFIED.,.F.,.F.,(4,3,3,4),(0.,
0.0272825353841119,0.0540089361834485,0.0724627707915405),.UNSPECIFIED.);
#5162=B_SPLINE_CURVE_WITH_KNOTS('',3,(#55062,#55063,#55064,#55065,#55066,
#55067),.UNSPECIFIED.,.F.,.F.,(4,2,4),(0.791208984971947,0.837333988005476,
1.0275823715977),.UNSPECIFIED.);
#5163=B_SPLINE_CURVE_WITH_KNOTS('',3,(#55068,#55069,#55070,#55071,#55072,
#55073),.UNSPECIFIED.,.F.,.F.,(4,2,4),(0.,1.45,2.85),.UNSPECIFIED.);
#5164=B_SPLINE_CURVE_WITH_KNOTS('',3,(#55158,#55159,#55160,#55161,#55162,
#55163),.UNSPECIFIED.,.F.,.F.,(4,2,4),(0.,1.45,2.85),.UNSPECIFIED.);
#5165=B_SPLINE_CURVE_WITH_KNOTS('',3,(#55165,#55166,#55167,#55168,#55169,
#55170),.UNSPECIFIED.,.F.,.F.,(4,2,4),(0.924746809891892,0.981018841208115,
1.21342818547153),.UNSPECIFIED.);
#5166=B_SPLINE_CURVE_WITH_KNOTS('',3,(#55254,#55255,#55256,#55257,#55258,
#55259),.UNSPECIFIED.,.F.,.F.,(4,2,4),(0.,1.45,2.85),.UNSPECIFIED.);
#5167=B_SPLINE_CURVE_WITH_KNOTS('',3,(#55260,#55261,#55262,#55263),
 .UNSPECIFIED.,.F.,.F.,(4,4),(0.,0.0536817275837366),.UNSPECIFIED.);
#5168=B_SPLINE_CURVE_WITH_KNOTS('',3,(#55267,#55268,#55269,#55270,#55271,
#55272),.UNSPECIFIED.,.F.,.F.,(4,2,4),(0.,1.45,2.85),.UNSPECIFIED.);
#5169=B_SPLINE_CURVE_WITH_KNOTS('',3,(#55274,#55275,#55276,#55277),
 .UNSPECIFIED.,.F.,.F.,(4,4),(0.,0.0536817275826949),.UNSPECIFIED.);
#5170=B_SPLINE_CURVE_WITH_KNOTS('',3,(#55442,#55443,#55444,#55445,#55446,
#55447),.UNSPECIFIED.,.F.,.F.,(4,2,4),(0.924746809881685,0.981018841196878,
1.2134281854522),.UNSPECIFIED.);
#5171=B_SPLINE_CURVE_WITH_KNOTS('',3,(#55448,#55449,#55450,#55451,#55452,
#55453),.UNSPECIFIED.,.F.,.F.,(4,2,4),(0.,1.45,2.85),.UNSPECIFIED.);
#5172=B_SPLINE_CURVE_WITH_KNOTS('',3,(#55538,#55539,#55540,#55541,#55542,
#55543),.UNSPECIFIED.,.F.,.F.,(4,2,4),(0.,1.45,2.85),.UNSPECIFIED.);
#5173=B_SPLINE_CURVE_WITH_KNOTS('',3,(#55545,#55546,#55547,#55548,#55549,
#55550),.UNSPECIFIED.,.F.,.F.,(4,2,4),(0.92474680987975,0.981018841194028,
1.21342818544147),.UNSPECIFIED.);
#5174=B_SPLINE_CURVE_WITH_KNOTS('',3,(#55634,#55635,#55636,#55637,#55638,
#55639),.UNSPECIFIED.,.F.,.F.,(4,2,4),(0.,1.45,2.85),.UNSPECIFIED.);
#5175=B_SPLINE_CURVE_WITH_KNOTS('',3,(#55640,#55641,#55642,#55643,#55644,
#55645,#55646),.UNSPECIFIED.,.F.,.F.,(4,3,4),(0.,0.0297140756203395,0.0782401718741553),
 .UNSPECIFIED.);
#5176=B_SPLINE_CURVE_WITH_KNOTS('',3,(#55650,#55651,#55652,#55653,#55654,
#55655),.UNSPECIFIED.,.F.,.F.,(4,2,4),(0.,1.45,2.85),.UNSPECIFIED.);
#5177=B_SPLINE_CURVE_WITH_KNOTS('',3,(#55657,#55658,#55659,#55660),
 .UNSPECIFIED.,.F.,.F.,(4,4),(0.,0.0536817275848442),.UNSPECIFIED.);
#5178=B_SPLINE_CURVE_WITH_KNOTS('',3,(#55825,#55826,#55827,#55828,#55829,
#55830),.UNSPECIFIED.,.F.,.F.,(4,2,4),(0.924746809894682,0.981018841211385,
1.21342818547561),.UNSPECIFIED.);
#5179=B_SPLINE_CURVE_WITH_KNOTS('',3,(#55831,#55832,#55833,#55834,#55835,
#55836),.UNSPECIFIED.,.F.,.F.,(4,2,4),(0.,1.45,2.85),.UNSPECIFIED.);
#5180=B_SPLINE_CURVE_WITH_KNOTS('',3,(#55921,#55922,#55923,#55924,#55925,
#55926),.UNSPECIFIED.,.F.,.F.,(4,2,4),(0.,1.45,2.85),.UNSPECIFIED.);
#5181=B_SPLINE_CURVE_WITH_KNOTS('',3,(#55928,#55929,#55930,#55931,#55932,
#55933),.UNSPECIFIED.,.F.,.F.,(4,2,4),(0.924746809888962,0.98101884120512,
1.21342818546788),.UNSPECIFIED.);
#5182=B_SPLINE_CURVE_WITH_KNOTS('',3,(#56017,#56018,#56019,#56020,#56021,
#56022),.UNSPECIFIED.,.F.,.F.,(4,2,4),(0.,1.45,2.85),.UNSPECIFIED.);
#5183=B_SPLINE_CURVE_WITH_KNOTS('',3,(#56023,#56024,#56025,#56026),
 .UNSPECIFIED.,.F.,.F.,(4,4),(0.,0.0536817275789145),.UNSPECIFIED.);
#5184=B_SPLINE_CURVE_WITH_KNOTS('',3,(#56030,#56031,#56032,#56033,#56034,
#56035),.UNSPECIFIED.,.F.,.F.,(4,2,4),(0.,1.45,2.85),.UNSPECIFIED.);
#5185=B_SPLINE_CURVE_WITH_KNOTS('',3,(#56037,#56038,#56039,#56040),
 .UNSPECIFIED.,.F.,.F.,(4,4),(0.,0.0782778812825522),.UNSPECIFIED.);
#5186=B_SPLINE_CURVE_WITH_KNOTS('',3,(#56205,#56206,#56207,#56208,#56209,
#56210),.UNSPECIFIED.,.F.,.F.,(4,2,4),(0.0895985966900729,0.107791487558596,
0.178841205983874),.UNSPECIFIED.);
#5187=B_SPLINE_CURVE_WITH_KNOTS('',3,(#56211,#56212,#56213,#56214,#56215,
#56216),.UNSPECIFIED.,.F.,.F.,(4,2,4),(0.,1.45,2.85),.UNSPECIFIED.);
#5188=B_SPLINE_CURVE_WITH_KNOTS('',3,(#56301,#56302,#56303,#56304,#56305,
#56306),.UNSPECIFIED.,.F.,.F.,(4,2,4),(0.,1.45,2.85),.UNSPECIFIED.);
#5189=B_SPLINE_CURVE_WITH_KNOTS('',3,(#56308,#56309,#56310,#56311,#56312,
#56313),.UNSPECIFIED.,.F.,.F.,(4,2,4),(0.791208985000826,0.837333988039583,
1.0275823716573),.UNSPECIFIED.);
#5190=B_SPLINE_CURVE_WITH_KNOTS('',3,(#56397,#56398,#56399,#56400,#56401,
#56402),.UNSPECIFIED.,.F.,.F.,(4,2,4),(0.,1.45,2.85),.UNSPECIFIED.);
#5191=B_SPLINE_CURVE_WITH_KNOTS('',3,(#56403,#56404,#56405,#56406,#56407,
#56408,#56409,#56410,#56411,#56412),.UNSPECIFIED.,.F.,.F.,(4,3,3,4),(0.,
0.0272825353828734,0.0540089361863412,0.0724627707912745),.UNSPECIFIED.);
#5192=B_SPLINE_CURVE_WITH_KNOTS('',3,(#56416,#56417,#56418,#56419,#56420,
#56421),.UNSPECIFIED.,.F.,.F.,(4,2,4),(0.,1.45,2.85),.UNSPECIFIED.);
#5193=B_SPLINE_CURVE_WITH_KNOTS('',3,(#56423,#56424,#56425,#56426),
 .UNSPECIFIED.,.F.,.F.,(4,4),(0.,0.0536817275846425),.UNSPECIFIED.);
#5194=B_SPLINE_CURVE_WITH_KNOTS('',3,(#56591,#56592,#56593,#56594,#56595,
#56596),.UNSPECIFIED.,.F.,.F.,(4,2,4),(0.924746809884044,0.981018841198511,
1.21342818544902),.UNSPECIFIED.);
#5195=B_SPLINE_CURVE_WITH_KNOTS('',3,(#56597,#56598,#56599,#56600,#56601,
#56602),.UNSPECIFIED.,.F.,.F.,(4,2,4),(0.,1.45,2.85),.UNSPECIFIED.);
#5196=B_SPLINE_CURVE_WITH_KNOTS('',3,(#56687,#56688,#56689,#56690),
 .UNSPECIFIED.,.F.,.F.,(4,4),(0.,0.053681727571403),.UNSPECIFIED.);
#5197=B_SPLINE_CURVE_WITH_KNOTS('',3,(#56692,#56693,#56694,#56695,#56696,
#56697),.UNSPECIFIED.,.F.,.F.,(4,2,4),(0.,1.45,2.85),.UNSPECIFIED.);
#5198=B_SPLINE_CURVE_WITH_KNOTS('',3,(#56861,#56862,#56863,#56864),
 .UNSPECIFIED.,.F.,.F.,(4,4),(0.,0.0942418390735999),.UNSPECIFIED.);
#5199=B_SPLINE_CURVE_WITH_KNOTS('',3,(#56867,#56868,#56869,#56870,#56871,
#56872),.UNSPECIFIED.,.F.,.F.,(4,2,4),(0.336411782332586,0.341442004890514,
0.473061015913503),.UNSPECIFIED.);
#5200=B_SPLINE_CURVE_WITH_KNOTS('',3,(#56873,#56874,#56875,#56876),
 .UNSPECIFIED.,.F.,.F.,(4,4),(0.,1.5),.UNSPECIFIED.);
#5201=B_SPLINE_CURVE_WITH_KNOTS('',3,(#56960,#56961,#56962,#56963,#56964,
#56965,#56966,#56967,#56968,#56969),.UNSPECIFIED.,.F.,.F.,(4,3,3,4),(0.00555547746779166,
0.0431313379163893,0.0740617625597658,0.080707198364987),.UNSPECIFIED.);
#5202=B_SPLINE_CURVE_WITH_KNOTS('',3,(#56971,#56972,#56973,#56974),
 .UNSPECIFIED.,.F.,.F.,(4,4),(0.,1.5),.UNSPECIFIED.);
#5203=B_SPLINE_CURVE_WITH_KNOTS('',3,(#56975,#56976,#56977,#56978,#56979,
#56980,#56981,#56982,#56983,#56984),.UNSPECIFIED.,.F.,.F.,(4,3,3,4),(0.,
0.0325402337502392,0.0706876468156212,0.074495117381235),.UNSPECIFIED.);
#5204=B_SPLINE_CURVE_WITH_KNOTS('',3,(#56988,#56989,#56990,#56991),
 .UNSPECIFIED.,.F.,.F.,(4,4),(0.100001236859483,0.210043570655993),
 .UNSPECIFIED.);
#5205=B_SPLINE_CURVE_WITH_KNOTS('',3,(#56995,#56996,#56997,#56998),
 .UNSPECIFIED.,.F.,.F.,(4,4),(0.,1.5),.UNSPECIFIED.);
#5206=B_SPLINE_CURVE_WITH_KNOTS('',3,(#57000,#57001,#57002,#57003),
 .UNSPECIFIED.,.F.,.F.,(4,4),(0.,0.0623435089195132),.UNSPECIFIED.);
#5207=B_SPLINE_CURVE_WITH_KNOTS('',3,(#57085,#57086,#57087,#57088),
 .UNSPECIFIED.,.F.,.F.,(4,4),(0.,0.0942418390734902),.UNSPECIFIED.);
#5208=B_SPLINE_CURVE_WITH_KNOTS('',3,(#57091,#57092,#57093,#57094,#57095,
#57096),.UNSPECIFIED.,.F.,.F.,(4,2,4),(0.811792901815019,0.910057458243994,
1.10441658254866),.UNSPECIFIED.);
#5209=B_SPLINE_CURVE_WITH_KNOTS('',3,(#57097,#57098,#57099,#57100),
 .UNSPECIFIED.,.F.,.F.,(4,4),(0.,1.5),.UNSPECIFIED.);
#5210=B_SPLINE_CURVE_WITH_KNOTS('',3,(#57186,#57187,#57188,#57189),
 .UNSPECIFIED.,.F.,.F.,(4,4),(0.102444446506542,0.212752916833154),
 .UNSPECIFIED.);
#5211=B_SPLINE_CURVE_WITH_KNOTS('',3,(#57193,#57194,#57195,#57196),
 .UNSPECIFIED.,.F.,.F.,(4,4),(0.,1.5),.UNSPECIFIED.);
#5212=B_SPLINE_CURVE_WITH_KNOTS('',3,(#57198,#57199,#57200,#57201),
 .UNSPECIFIED.,.F.,.F.,(4,4),(0.,0.0624333513906016),.UNSPECIFIED.);
#5213=B_SPLINE_CURVE_WITH_KNOTS('',3,(#57283,#57284,#57285,#57286),
 .UNSPECIFIED.,.F.,.F.,(4,4),(0.,0.0942418390735364),.UNSPECIFIED.);
#5214=B_SPLINE_CURVE_WITH_KNOTS('',3,(#57289,#57290,#57291,#57292,#57293,
#57294),.UNSPECIFIED.,.F.,.F.,(4,2,4),(0.813847978397809,0.909406578862909,
1.10554196286624),.UNSPECIFIED.);
#5215=B_SPLINE_CURVE_WITH_KNOTS('',3,(#57295,#57296,#57297,#57298),
 .UNSPECIFIED.,.F.,.F.,(4,4),(0.,1.5),.UNSPECIFIED.);
#5216=B_SPLINE_CURVE_WITH_KNOTS('',3,(#57384,#57385,#57386,#57387),
 .UNSPECIFIED.,.F.,.F.,(4,4),(0.102444446504211,0.212752916831367),
 .UNSPECIFIED.);
#5217=B_SPLINE_CURVE_WITH_KNOTS('',3,(#57391,#57392,#57393,#57394),
 .UNSPECIFIED.,.F.,.F.,(4,4),(0.,1.5),.UNSPECIFIED.);
#5218=B_SPLINE_CURVE_WITH_KNOTS('',3,(#57396,#57397,#57398,#57399),
 .UNSPECIFIED.,.F.,.F.,(4,4),(0.,0.0624333513927156),.UNSPECIFIED.);
#5219=B_SPLINE_CURVE_WITH_KNOTS('',3,(#57481,#57482,#57483,#57484),
 .UNSPECIFIED.,.F.,.F.,(4,4),(0.,0.0942418390735309),.UNSPECIFIED.);
#5220=B_SPLINE_CURVE_WITH_KNOTS('',3,(#57487,#57488,#57489,#57490,#57491,
#57492),.UNSPECIFIED.,.F.,.F.,(4,2,4),(0.813847978500005,0.909406579009422,
1.10554196310352),.UNSPECIFIED.);
#5221=B_SPLINE_CURVE_WITH_KNOTS('',3,(#57493,#57494,#57495,#57496),
 .UNSPECIFIED.,.F.,.F.,(4,4),(0.,1.5),.UNSPECIFIED.);
#5222=B_SPLINE_CURVE_WITH_KNOTS('',3,(#57582,#57583,#57584,#57585),
 .UNSPECIFIED.,.F.,.F.,(4,4),(0.102444446507355,0.212752916840295),
 .UNSPECIFIED.);
#5223=B_SPLINE_CURVE_WITH_KNOTS('',3,(#57589,#57590,#57591,#57592),
 .UNSPECIFIED.,.F.,.F.,(4,4),(0.,1.5),.UNSPECIFIED.);
#5224=B_SPLINE_CURVE_WITH_KNOTS('',3,(#57594,#57595,#57596,#57597),
 .UNSPECIFIED.,.F.,.F.,(4,4),(0.,0.0624333513891726),.UNSPECIFIED.);
#5225=B_SPLINE_CURVE_WITH_KNOTS('',3,(#57679,#57680,#57681,#57682),
 .UNSPECIFIED.,.F.,.F.,(4,4),(0.,0.094241839073544),.UNSPECIFIED.);
#5226=B_SPLINE_CURVE_WITH_KNOTS('',3,(#57685,#57686,#57687,#57688,#57689,
#57690),.UNSPECIFIED.,.F.,.F.,(4,2,4),(0.813847978462672,0.909406578962002,
1.10554196303347),.UNSPECIFIED.);
#5227=B_SPLINE_CURVE_WITH_KNOTS('',3,(#57691,#57692,#57693,#57694),
 .UNSPECIFIED.,.F.,.F.,(4,4),(0.,1.5),.UNSPECIFIED.);
#5228=B_SPLINE_CURVE_WITH_KNOTS('',3,(#57780,#57781,#57782,#57783),
 .UNSPECIFIED.,.F.,.F.,(4,4),(0.102444446505091,0.212752916823378),
 .UNSPECIFIED.);
#5229=B_SPLINE_CURVE_WITH_KNOTS('',3,(#57787,#57788,#57789,#57790),
 .UNSPECIFIED.,.F.,.F.,(4,4),(0.,1.5),.UNSPECIFIED.);
#5230=B_SPLINE_CURVE_WITH_KNOTS('',3,(#57792,#57793,#57794,#57795),
 .UNSPECIFIED.,.F.,.F.,(4,4),(0.,0.0624333513861405),.UNSPECIFIED.);
#5231=B_SPLINE_CURVE_WITH_KNOTS('',3,(#57877,#57878,#57879,#57880),
 .UNSPECIFIED.,.F.,.F.,(4,4),(0.,0.0942418390734816),.UNSPECIFIED.);
#5232=B_SPLINE_CURVE_WITH_KNOTS('',3,(#57883,#57884,#57885,#57886,#57887,
#57888),.UNSPECIFIED.,.F.,.F.,(4,2,4),(0.813847978451045,0.909406578940421,
1.10554196299329),.UNSPECIFIED.);
#5233=B_SPLINE_CURVE_WITH_KNOTS('',3,(#57889,#57890,#57891,#57892),
 .UNSPECIFIED.,.F.,.F.,(4,4),(0.,1.5),.UNSPECIFIED.);
#5234=B_SPLINE_CURVE_WITH_KNOTS('',3,(#57978,#57979,#57980,#57981,#57982,
#57983,#57984,#57985,#57986,#57987),.UNSPECIFIED.,.F.,.F.,(4,3,3,4),(0.00477610030196731,
0.0423460197867061,0.0734754921810407,0.079915939271445),.UNSPECIFIED.);
#5235=B_SPLINE_CURVE_WITH_KNOTS('',3,(#57991,#57992,#57993,#57994),
 .UNSPECIFIED.,.F.,.F.,(4,4),(0.,1.5),.UNSPECIFIED.);
#5236=B_SPLINE_CURVE_WITH_KNOTS('',3,(#57996,#57997,#57998,#57999,#58000,
#58001,#58002,#58003,#58004,#58005),.UNSPECIFIED.,.F.,.F.,(4,3,3,4),(0.,
0.0327390254020849,0.0706978041544828,0.0745133058834629),.UNSPECIFIED.);
#5237=B_SPLINE_CURVE_WITH_KNOTS('',3,(#58087,#58088,#58089,#58090,#58091,
#58092),.UNSPECIFIED.,.F.,.F.,(4,2,4),(0.,0.0726060447861878,0.0941220646064719),
 .UNSPECIFIED.);
#5238=B_SPLINE_CURVE_WITH_KNOTS('',3,(#58095,#58096,#58097,#58098,#58099,
#58100,#58101,#58102,#58103,#58104,#58105,#58106,#58107,#58108,#58109,#58110,
#58111,#58112,#58113),.UNSPECIFIED.,.F.,.F.,(4,3,3,3,3,3,4),(0.0359490020947758,
0.0514463139246939,0.0621647509937864,0.0701407164412387,0.0817621854071257,
0.0922147861198435,0.0991326682752126),.UNSPECIFIED.);
#5239=B_SPLINE_CURVE_WITH_KNOTS('',3,(#58114,#58115,#58116,#58117),
 .UNSPECIFIED.,.F.,.F.,(4,4),(0.,1.5),.UNSPECIFIED.);
#5240=B_SPLINE_CURVE_WITH_KNOTS('',3,(#58203,#58204,#58205,#58206),
 .UNSPECIFIED.,.F.,.F.,(4,4),(0.0684253031638949,0.146459794934132),
 .UNSPECIFIED.);
#5241=B_SPLINE_CURVE_WITH_KNOTS('',3,(#58210,#58211,#58212,#58213),
 .UNSPECIFIED.,.F.,.F.,(4,4),(0.,1.5),.UNSPECIFIED.);
#5242=B_SPLINE_CURVE_WITH_KNOTS('',3,(#58215,#58216,#58217,#58218),
 .UNSPECIFIED.,.F.,.F.,(4,4),(0.,0.0743296555811839),.UNSPECIFIED.);
#5243=B_SPLINE_CURVE_WITH_KNOTS('',3,(#58300,#58301,#58302,#58303),
 .UNSPECIFIED.,.F.,.F.,(4,4),(0.,0.0942418390734843),.UNSPECIFIED.);
#5244=B_SPLINE_CURVE_WITH_KNOTS('',3,(#58306,#58307,#58308,#58309,#58310,
#58311),.UNSPECIFIED.,.F.,.F.,(4,2,4),(0.780516546471215,0.880889879619728,
1.03952845678898),.UNSPECIFIED.);
#5245=B_SPLINE_CURVE_WITH_KNOTS('',3,(#58312,#58313,#58314,#58315),
 .UNSPECIFIED.,.F.,.F.,(4,4),(0.,1.5),.UNSPECIFIED.);
#5246=B_SPLINE_CURVE_WITH_KNOTS('',3,(#58401,#58402,#58403,#58404),
 .UNSPECIFIED.,.F.,.F.,(4,4),(0.102444446506539,0.212752916832809),
 .UNSPECIFIED.);
#5247=B_SPLINE_CURVE_WITH_KNOTS('',3,(#58408,#58409,#58410,#58411),
 .UNSPECIFIED.,.F.,.F.,(4,4),(0.,1.5),.UNSPECIFIED.);
#5248=B_SPLINE_CURVE_WITH_KNOTS('',3,(#58413,#58414,#58415,#58416),
 .UNSPECIFIED.,.F.,.F.,(4,4),(0.,0.0624333513889912),.UNSPECIFIED.);
#5249=B_SPLINE_CURVE_WITH_KNOTS('',3,(#58498,#58499,#58500,#58501),
 .UNSPECIFIED.,.F.,.F.,(4,4),(0.,0.0942418390729746),.UNSPECIFIED.);
#5250=B_SPLINE_CURVE_WITH_KNOTS('',3,(#58504,#58505,#58506,#58507,#58508,
#58509),.UNSPECIFIED.,.F.,.F.,(4,2,4),(0.813847978400163,0.909406578867221,
1.10554196287215),.UNSPECIFIED.);
#5251=B_SPLINE_CURVE_WITH_KNOTS('',3,(#58510,#58511,#58512,#58513),
 .UNSPECIFIED.,.F.,.F.,(4,4),(0.,1.5),.UNSPECIFIED.);
#5252=B_SPLINE_CURVE_WITH_KNOTS('',3,(#58599,#58600,#58601,#58602),
 .UNSPECIFIED.,.F.,.F.,(4,4),(0.102444446511599,0.212752916841184),
 .UNSPECIFIED.);
#5253=B_SPLINE_CURVE_WITH_KNOTS('',3,(#58606,#58607,#58608,#58609),
 .UNSPECIFIED.,.F.,.F.,(4,4),(0.,1.5),.UNSPECIFIED.);
#5254=B_SPLINE_CURVE_WITH_KNOTS('',3,(#58611,#58612,#58613,#58614),
 .UNSPECIFIED.,.F.,.F.,(4,4),(0.,0.0624333513921405),.UNSPECIFIED.);
#5255=B_SPLINE_CURVE_WITH_KNOTS('',3,(#58696,#58697,#58698,#58699),
 .UNSPECIFIED.,.F.,.F.,(4,4),(0.,0.0942418390729232),.UNSPECIFIED.);
#5256=B_SPLINE_CURVE_WITH_KNOTS('',3,(#58702,#58703,#58704,#58705,#58706,
#58707),.UNSPECIFIED.,.F.,.F.,(4,2,4),(0.813847978447724,0.909406578934804,
1.10554196297989),.UNSPECIFIED.);
#5257=B_SPLINE_CURVE_WITH_KNOTS('',3,(#58708,#58709,#58710,#58711),
 .UNSPECIFIED.,.F.,.F.,(4,4),(0.,1.5),.UNSPECIFIED.);
#5258=B_SPLINE_CURVE_WITH_KNOTS('',3,(#58797,#58798,#58799,#58800),
 .UNSPECIFIED.,.F.,.F.,(4,4),(0.102444446506069,0.212752916828345),
 .UNSPECIFIED.);
#5259=B_SPLINE_CURVE_WITH_KNOTS('',3,(#58804,#58805,#58806,#58807),
 .UNSPECIFIED.,.F.,.F.,(4,4),(0.,1.5),.UNSPECIFIED.);
#5260=B_SPLINE_CURVE_WITH_KNOTS('',3,(#58809,#58810,#58811,#58812),
 .UNSPECIFIED.,.F.,.F.,(4,4),(0.,0.0624333513925485),.UNSPECIFIED.);
#5261=B_SPLINE_CURVE_WITH_KNOTS('',3,(#58894,#58895,#58896,#58897),
 .UNSPECIFIED.,.F.,.F.,(4,4),(0.,0.0942418390736248),.UNSPECIFIED.);
#5262=B_SPLINE_CURVE_WITH_KNOTS('',3,(#58900,#58901,#58902,#58903,#58904,
#58905),.UNSPECIFIED.,.F.,.F.,(4,2,4),(0.813847978393684,0.909406578861889,
1.10554196287168),.UNSPECIFIED.);
#5263=B_SPLINE_CURVE_WITH_KNOTS('',3,(#58906,#58907,#58908,#58909),
 .UNSPECIFIED.,.F.,.F.,(4,4),(0.,1.5),.UNSPECIFIED.);
#5264=B_SPLINE_CURVE_WITH_KNOTS('',3,(#58995,#58996,#58997,#58998),
 .UNSPECIFIED.,.F.,.F.,(4,4),(0.102444446506724,0.212752916833258),
 .UNSPECIFIED.);
#5265=B_SPLINE_CURVE_WITH_KNOTS('',3,(#59002,#59003,#59004,#59005),
 .UNSPECIFIED.,.F.,.F.,(4,4),(0.,1.5),.UNSPECIFIED.);
#5266=B_SPLINE_CURVE_WITH_KNOTS('',3,(#59007,#59008,#59009,#59010),
 .UNSPECIFIED.,.F.,.F.,(4,4),(0.,0.0624333513889975),.UNSPECIFIED.);
#5267=B_SPLINE_CURVE_WITH_KNOTS('',3,(#59092,#59093,#59094,#59095),
 .UNSPECIFIED.,.F.,.F.,(4,4),(0.,0.0942418390734104),.UNSPECIFIED.);
#5268=B_SPLINE_CURVE_WITH_KNOTS('',3,(#59098,#59099,#59100,#59101,#59102,
#59103),.UNSPECIFIED.,.F.,.F.,(4,2,4),(0.813847978443022,0.909406578934323,
1.10554196299104),.UNSPECIFIED.);
#5269=B_SPLINE_CURVE_WITH_KNOTS('',3,(#59104,#59105,#59106,#59107),
 .UNSPECIFIED.,.F.,.F.,(4,4),(0.,1.5),.UNSPECIFIED.);
#5270=B_SPLINE_CURVE_WITH_KNOTS('',3,(#59193,#59194,#59195,#59196,#59197,
#59198,#59199,#59200,#59201,#59202),.UNSPECIFIED.,.F.,.F.,(4,3,3,4),(0.0202435582116424,
0.0580416628844639,0.0862802856669505,0.0958397675572854),.UNSPECIFIED.);
#5271=B_SPLINE_CURVE_WITH_KNOTS('',3,(#59206,#59207,#59208,#59209),
 .UNSPECIFIED.,.F.,.F.,(4,4),(0.,1.5),.UNSPECIFIED.);
#5272=B_SPLINE_CURVE_WITH_KNOTS('',3,(#59211,#59212,#59213,#59214,#59215,
#59216,#59217,#59218,#59219,#59220),.UNSPECIFIED.,.F.,.F.,(4,3,3,4),(0.,
0.0294422535083819,0.0624658169425315,0.0742491588861056),.UNSPECIFIED.);
#5273=B_SPLINE_CURVE_WITH_KNOTS('',3,(#59302,#59303,#59304,#59305,#59306,
#59307,#59308,#59309),.UNSPECIFIED.,.F.,.F.,(4,2,2,4),(0.,0.0579167605929198,
0.0898095080041945,0.0921865044561621),.UNSPECIFIED.);
#5274=B_SPLINE_CURVE_WITH_KNOTS('',3,(#59312,#59313,#59314,#59315,#59316,
#59317),.UNSPECIFIED.,.F.,.F.,(4,2,4),(0.0188457662145042,0.0323539946370597,
0.0791558368865173),.UNSPECIFIED.);
#5275=B_SPLINE_CURVE_WITH_KNOTS('',3,(#59318,#59319,#59320,#59321),
 .UNSPECIFIED.,.F.,.F.,(4,4),(0.,1.5),.UNSPECIFIED.);
#5276=B_SPLINE_CURVE_WITH_KNOTS('',3,(#59407,#59408,#59409,#59410,#59411,
#59412,#59413,#59414,#59415,#59416),.UNSPECIFIED.,.F.,.F.,(4,3,3,4),(0.0395084943485573,
0.0733345045630657,0.101123500261748,0.116125323696474),.UNSPECIFIED.);
#5277=B_SPLINE_CURVE_WITH_KNOTS('',3,(#59420,#59421,#59422,#59423),
 .UNSPECIFIED.,.F.,.F.,(4,4),(0.,1.5),.UNSPECIFIED.);
#5278=B_SPLINE_CURVE_WITH_KNOTS('',3,(#59425,#59426,#59427,#59428,#59429,
#59430,#59431,#59432,#59433,#59434),.UNSPECIFIED.,.F.,.F.,(4,3,3,4),(0.,
0.0270437474794931,0.0553924043849417,0.0741757654504447),.UNSPECIFIED.);
#5279=B_SPLINE_CURVE_WITH_KNOTS('',3,(#59516,#59517,#59518,#59519),
 .UNSPECIFIED.,.F.,.F.,(4,4),(0.,0.0942418390732598),.UNSPECIFIED.);
#5280=B_SPLINE_CURVE_WITH_KNOTS('',3,(#59522,#59523,#59524,#59525,#59526,
#59527),.UNSPECIFIED.,.F.,.F.,(4,2,4),(0.779548576793953,0.882208032727733,
1.03977959949153),.UNSPECIFIED.);
#5281=B_SPLINE_CURVE_WITH_KNOTS('',3,(#59528,#59529,#59530,#59531),
 .UNSPECIFIED.,.F.,.F.,(4,4),(0.,1.5),.UNSPECIFIED.);
#5282=B_SPLINE_CURVE_WITH_KNOTS('',3,(#59617,#59618,#59619,#59620),
 .UNSPECIFIED.,.F.,.F.,(4,4),(0.102444446506346,0.212752916828858),
 .UNSPECIFIED.);
#5283=B_SPLINE_CURVE_WITH_KNOTS('',3,(#59624,#59625,#59626,#59627),
 .UNSPECIFIED.,.F.,.F.,(4,4),(0.,1.5),.UNSPECIFIED.);
#5284=B_SPLINE_CURVE_WITH_KNOTS('',3,(#59629,#59630,#59631,#59632),
 .UNSPECIFIED.,.F.,.F.,(4,4),(0.,0.0624333513912447),.UNSPECIFIED.);
#5285=B_SPLINE_CURVE_WITH_KNOTS('',3,(#59714,#59715,#59716,#59717),
 .UNSPECIFIED.,.F.,.F.,(4,4),(0.,0.0942418390735563),.UNSPECIFIED.);
#5286=B_SPLINE_CURVE_WITH_KNOTS('',3,(#59720,#59721,#59722,#59723,#59724,
#59725),.UNSPECIFIED.,.F.,.F.,(4,2,4),(0.813847978426091,0.909406578908649,
1.10554196294765),.UNSPECIFIED.);
#5287=B_SPLINE_CURVE_WITH_KNOTS('',3,(#59726,#59727,#59728,#59729),
 .UNSPECIFIED.,.F.,.F.,(4,4),(0.,1.5),.UNSPECIFIED.);
#5288=B_SPLINE_CURVE_WITH_KNOTS('',3,(#59815,#59816,#59817,#59818),
 .UNSPECIFIED.,.F.,.F.,(4,4),(0.10244444650535,0.212752916825456),
 .UNSPECIFIED.);
#5289=B_SPLINE_CURVE_WITH_KNOTS('',3,(#59822,#59823,#59824,#59825),
 .UNSPECIFIED.,.F.,.F.,(4,4),(0.,1.5),.UNSPECIFIED.);
#5290=B_SPLINE_CURVE_WITH_KNOTS('',3,(#59827,#59828,#59829,#59830),
 .UNSPECIFIED.,.F.,.F.,(4,4),(0.,0.0624333513928975),.UNSPECIFIED.);
#5291=B_SPLINE_CURVE_WITH_KNOTS('',3,(#59912,#59913,#59914,#59915),
 .UNSPECIFIED.,.F.,.F.,(4,4),(0.,0.0942418390733905),.UNSPECIFIED.);
#5292=B_SPLINE_CURVE_WITH_KNOTS('',3,(#59918,#59919,#59920,#59921,#59922,
#59923),.UNSPECIFIED.,.F.,.F.,(4,2,4),(0.81384797842961,0.90940657891296,
1.1055419629536),.UNSPECIFIED.);
#5293=B_SPLINE_CURVE_WITH_KNOTS('',3,(#59924,#59925,#59926,#59927),
 .UNSPECIFIED.,.F.,.F.,(4,4),(0.,1.5),.UNSPECIFIED.);
#5294=B_SPLINE_CURVE_WITH_KNOTS('',3,(#60013,#60014,#60015,#60016),
 .UNSPECIFIED.,.F.,.F.,(4,4),(0.102444446506175,0.21275291682957),
 .UNSPECIFIED.);
#5295=B_SPLINE_CURVE_WITH_KNOTS('',3,(#60020,#60021,#60022,#60023),
 .UNSPECIFIED.,.F.,.F.,(4,4),(0.,1.5),.UNSPECIFIED.);
#5296=B_SPLINE_CURVE_WITH_KNOTS('',3,(#60025,#60026,#60027,#60028),
 .UNSPECIFIED.,.F.,.F.,(4,4),(0.,0.0624333513924381),.UNSPECIFIED.);
#5297=B_SPLINE_CURVE_WITH_KNOTS('',3,(#60110,#60111,#60112,#60113),
 .UNSPECIFIED.,.F.,.F.,(4,4),(0.,0.0942418390734806),.UNSPECIFIED.);
#5298=B_SPLINE_CURVE_WITH_KNOTS('',3,(#60116,#60117,#60118,#60119,#60120,
#60121),.UNSPECIFIED.,.F.,.F.,(4,2,4),(0.813847978432191,0.909406578917468,
1.10554196296299),.UNSPECIFIED.);
#5299=B_SPLINE_CURVE_WITH_KNOTS('',3,(#60122,#60123,#60124,#60125),
 .UNSPECIFIED.,.F.,.F.,(4,4),(0.,1.5),.UNSPECIFIED.);
#5300=B_SPLINE_CURVE_WITH_KNOTS('',3,(#60211,#60212,#60213,#60214),
 .UNSPECIFIED.,.F.,.F.,(4,4),(0.10244444650664,0.212752916829421),
 .UNSPECIFIED.);
#5301=B_SPLINE_CURVE_WITH_KNOTS('',3,(#60218,#60219,#60220,#60221),
 .UNSPECIFIED.,.F.,.F.,(4,4),(0.,1.5),.UNSPECIFIED.);
#5302=B_SPLINE_CURVE_WITH_KNOTS('',3,(#60223,#60224,#60225,#60226),
 .UNSPECIFIED.,.F.,.F.,(4,4),(0.,0.0624333513894458),.UNSPECIFIED.);
#5303=B_SPLINE_CURVE_WITH_KNOTS('',3,(#60308,#60309,#60310,#60311),
 .UNSPECIFIED.,.F.,.F.,(4,4),(0.,0.0942418390733715),.UNSPECIFIED.);
#5304=B_SPLINE_CURVE_WITH_KNOTS('',3,(#60314,#60315,#60316,#60317,#60318,
#60319),.UNSPECIFIED.,.F.,.F.,(4,2,4),(0.81384797850735,0.909406579018074,
1.10554196311433),.UNSPECIFIED.);
#5305=B_SPLINE_CURVE_WITH_KNOTS('',3,(#60320,#60321,#60322,#60323),
 .UNSPECIFIED.,.F.,.F.,(4,4),(0.,1.5),.UNSPECIFIED.);
#5306=B_SPLINE_CURVE_WITH_KNOTS('',3,(#60409,#60410,#60411,#60412,#60413,
#60414,#60415,#60416,#60417,#60418),.UNSPECIFIED.,.F.,.F.,(4,3,3,4),(0.0463594297612979,
0.0792638205058534,0.106678138460634,0.123352993578161),.UNSPECIFIED.);
#5307=B_SPLINE_CURVE_WITH_KNOTS('',3,(#60422,#60423,#60424,#60425),
 .UNSPECIFIED.,.F.,.F.,(4,4),(0.,1.5),.UNSPECIFIED.);
#5308=B_SPLINE_CURVE_WITH_KNOTS('',3,(#60427,#60428,#60429,#60430,#60431,
#60432,#60433,#60434,#60435,#60436),.UNSPECIFIED.,.F.,.F.,(4,3,3,4),(0.,
0.0265473416310855,0.0541632094422211,0.0741956218732892),.UNSPECIFIED.);
#5309=B_SPLINE_CURVE_WITH_KNOTS('',3,(#60518,#60519,#60520,#60521,#60522,
#60523),.UNSPECIFIED.,.F.,.F.,(4,2,4),(0.,0.0841859688066849,0.0944738106033242),
 .UNSPECIFIED.);
#5310=B_SPLINE_CURVE_WITH_KNOTS('',3,(#60526,#60527,#60528,#60529,#60530,
#60531),.UNSPECIFIED.,.F.,.F.,(4,2,4),(0.0591715987737748,0.0874825086625098,
0.130961342687466),.UNSPECIFIED.);
#5311=B_SPLINE_CURVE_WITH_KNOTS('',3,(#60532,#60533,#60534,#60535),
 .UNSPECIFIED.,.F.,.F.,(4,4),(0.,1.5),.UNSPECIFIED.);
#5312=B_SPLINE_CURVE_WITH_KNOTS('',3,(#60621,#60622,#60623,#60624,#60625,
#60626,#60627,#60628,#60629,#60630),.UNSPECIFIED.,.F.,.F.,(4,3,3,4),(0.0186187815726518,
0.05638216058415,0.0848432631253004,0.0941455395956483),.UNSPECIFIED.);
#5313=B_SPLINE_CURVE_WITH_KNOTS('',3,(#60634,#60635,#60636,#60637),
 .UNSPECIFIED.,.F.,.F.,(4,4),(0.,1.5),.UNSPECIFIED.);
#5314=B_SPLINE_CURVE_WITH_KNOTS('',3,(#60639,#60640,#60641,#60642,#60643,
#60644,#60645,#60646,#60647,#60648),.UNSPECIFIED.,.F.,.F.,(4,3,3,4),(0.,
0.029729407461831,0.0634621728237244,0.0742674437057334),.UNSPECIFIED.);
#5315=B_SPLINE_CURVE_WITH_KNOTS('',3,(#60730,#60731,#60732,#60733),
 .UNSPECIFIED.,.F.,.F.,(4,4),(0.,0.0942418390732922),.UNSPECIFIED.);
#5316=B_SPLINE_CURVE_WITH_KNOTS('',3,(#60736,#60737,#60738,#60739,#60740,
#60741),.UNSPECIFIED.,.F.,.F.,(4,2,4),(0.78291638968198,0.879991065903176,
1.0497516190461),.UNSPECIFIED.);
#5317=B_SPLINE_CURVE_WITH_KNOTS('',3,(#60742,#60743,#60744,#60745),
 .UNSPECIFIED.,.F.,.F.,(4,4),(0.,1.5),.UNSPECIFIED.);
#5318=B_SPLINE_CURVE_WITH_KNOTS('',3,(#60831,#60832,#60833,#60834),
 .UNSPECIFIED.,.F.,.F.,(4,4),(0.102444446507287,0.212752916834514),
 .UNSPECIFIED.);
#5319=B_SPLINE_CURVE_WITH_KNOTS('',3,(#60838,#60839,#60840,#60841),
 .UNSPECIFIED.,.F.,.F.,(4,4),(0.,1.5),.UNSPECIFIED.);
#5320=B_SPLINE_CURVE_WITH_KNOTS('',3,(#60843,#60844,#60845,#60846),
 .UNSPECIFIED.,.F.,.F.,(4,4),(0.,0.0624333513900251),.UNSPECIFIED.);
#5321=B_SPLINE_CURVE_WITH_KNOTS('',3,(#60928,#60929,#60930,#60931),
 .UNSPECIFIED.,.F.,.F.,(4,4),(0.,0.0942418390732355),.UNSPECIFIED.);
#5322=B_SPLINE_CURVE_WITH_KNOTS('',3,(#60934,#60935,#60936,#60937,#60938,
#60939),.UNSPECIFIED.,.F.,.F.,(4,2,4),(0.813847978423661,0.909406578902529,
1.10554196293435),.UNSPECIFIED.);
#5323=B_SPLINE_CURVE_WITH_KNOTS('',3,(#60940,#60941,#60942,#60943),
 .UNSPECIFIED.,.F.,.F.,(4,4),(0.,1.5),.UNSPECIFIED.);
#5324=B_SPLINE_CURVE_WITH_KNOTS('',3,(#61029,#61030,#61031,#61032),
 .UNSPECIFIED.,.F.,.F.,(4,4),(0.102444446507506,0.212752916837424),
 .UNSPECIFIED.);
#5325=B_SPLINE_CURVE_WITH_KNOTS('',3,(#61036,#61037,#61038,#61039),
 .UNSPECIFIED.,.F.,.F.,(4,4),(0.,1.5),.UNSPECIFIED.);
#5326=B_SPLINE_CURVE_WITH_KNOTS('',3,(#61041,#61042,#61043,#61044),
 .UNSPECIFIED.,.F.,.F.,(4,4),(0.,0.0624333513922893),.UNSPECIFIED.);
#5327=B_SPLINE_CURVE_WITH_KNOTS('',3,(#61126,#61127,#61128,#61129),
 .UNSPECIFIED.,.F.,.F.,(4,4),(0.,0.0942418390731036),.UNSPECIFIED.);
#5328=B_SPLINE_CURVE_WITH_KNOTS('',3,(#61132,#61133,#61134,#61135,#61136,
#61137),.UNSPECIFIED.,.F.,.F.,(4,2,4),(0.813847978416476,0.909406578891062,
1.10554196291473),.UNSPECIFIED.);
#5329=B_SPLINE_CURVE_WITH_KNOTS('',3,(#61138,#61139,#61140,#61141),
 .UNSPECIFIED.,.F.,.F.,(4,4),(0.,1.5),.UNSPECIFIED.);
#5330=B_SPLINE_CURVE_WITH_KNOTS('',3,(#61227,#61228,#61229,#61230),
 .UNSPECIFIED.,.F.,.F.,(4,4),(0.102444446497694,0.212752916802265),
 .UNSPECIFIED.);
#5331=B_SPLINE_CURVE_WITH_KNOTS('',3,(#61234,#61235,#61236,#61237),
 .UNSPECIFIED.,.F.,.F.,(4,4),(0.,1.5),.UNSPECIFIED.);
#5332=B_SPLINE_CURVE_WITH_KNOTS('',3,(#61239,#61240,#61241,#61242),
 .UNSPECIFIED.,.F.,.F.,(4,4),(0.,0.0624333513878915),.UNSPECIFIED.);
#5333=B_SPLINE_CURVE_WITH_KNOTS('',3,(#61324,#61325,#61326,#61327),
 .UNSPECIFIED.,.F.,.F.,(4,4),(0.,0.0942418390734442),.UNSPECIFIED.);
#5334=B_SPLINE_CURVE_WITH_KNOTS('',3,(#61330,#61331,#61332,#61333,#61334,
#61335),.UNSPECIFIED.,.F.,.F.,(4,2,4),(0.813847978408599,0.909406578879065,
1.10554196289057),.UNSPECIFIED.);
#5335=B_SPLINE_CURVE_WITH_KNOTS('',3,(#61336,#61337,#61338,#61339),
 .UNSPECIFIED.,.F.,.F.,(4,4),(0.,1.5),.UNSPECIFIED.);
#5336=B_SPLINE_CURVE_WITH_KNOTS('',3,(#61425,#61426,#61427,#61428),
 .UNSPECIFIED.,.F.,.F.,(4,4),(0.102444446506644,0.212752916832659),
 .UNSPECIFIED.);
#5337=B_SPLINE_CURVE_WITH_KNOTS('',3,(#61432,#61433,#61434,#61435),
 .UNSPECIFIED.,.F.,.F.,(4,4),(0.,1.5),.UNSPECIFIED.);
#5338=B_SPLINE_CURVE_WITH_KNOTS('',3,(#61437,#61438,#61439,#61440),
 .UNSPECIFIED.,.F.,.F.,(4,4),(0.,0.0624333513938403),.UNSPECIFIED.);
#5339=B_SPLINE_CURVE_WITH_KNOTS('',3,(#61522,#61523,#61524,#61525),
 .UNSPECIFIED.,.F.,.F.,(4,4),(0.,0.0942418390734082),.UNSPECIFIED.);
#5340=B_SPLINE_CURVE_WITH_KNOTS('',3,(#61528,#61529,#61530,#61531,#61532,
#61533),.UNSPECIFIED.,.F.,.F.,(4,2,4),(0.813847978438528,0.909406578924881,
1.10554196297139),.UNSPECIFIED.);
#5341=B_SPLINE_CURVE_WITH_KNOTS('',3,(#61534,#61535,#61536,#61537),
 .UNSPECIFIED.,.F.,.F.,(4,4),(0.,1.5),.UNSPECIFIED.);
#5342=B_SPLINE_CURVE_WITH_KNOTS('',3,(#61623,#61624,#61625,#61626),
 .UNSPECIFIED.,.F.,.F.,(4,4),(0.0904405428983144,0.199382706551901),
 .UNSPECIFIED.);
#5343=B_SPLINE_CURVE_WITH_KNOTS('',3,(#61630,#61631,#61632,#61633),
 .UNSPECIFIED.,.F.,.F.,(4,4),(0.,1.5),.UNSPECIFIED.);
#5344=B_SPLINE_CURVE_WITH_KNOTS('',3,(#61635,#61636,#61637,#61638),
 .UNSPECIFIED.,.F.,.F.,(4,4),(0.,0.0619557939569426),.UNSPECIFIED.);
#5345=B_SPLINE_CURVE_WITH_KNOTS('',3,(#61720,#61721,#61722,#61723),
 .UNSPECIFIED.,.F.,.F.,(4,4),(0.,0.0942418390734305),.UNSPECIFIED.);
#5346=B_SPLINE_CURVE_WITH_KNOTS('',3,(#61726,#61727,#61728,#61729,#61730,
#61731),.UNSPECIFIED.,.F.,.F.,(4,2,4),(0.604749643384554,0.619109901140346,
0.773617109883765),.UNSPECIFIED.);
#5347=B_SPLINE_CURVE_WITH_KNOTS('',3,(#61732,#61733,#61734,#61735),
 .UNSPECIFIED.,.F.,.F.,(4,4),(0.,1.5),.UNSPECIFIED.);
#5926=LINE('',#49234,#6818);
#5927=LINE('',#49238,#6819);
#5928=LINE('',#50086,#6820);
#5929=LINE('',#51702,#6821);
#5930=LINE('',#51747,#6822);
#5931=LINE('',#52007,#6823);
#5932=LINE('',#52017,#6824);
#5933=LINE('',#54592,#6825);
#5934=LINE('',#54594,#6826);
#5935=LINE('',#54778,#6827);
#5936=LINE('',#54786,#6828);
#5937=LINE('',#54978,#6829);
#5938=LINE('',#54980,#6830);
#5939=LINE('',#55164,#6831);
#5940=LINE('',#55172,#6832);
#5941=LINE('',#55358,#6833);
#5942=LINE('',#55360,#6834);
#5943=LINE('',#55544,#6835);
#5944=LINE('',#55552,#6836);
#5945=LINE('',#55741,#6837);
#5946=LINE('',#55743,#6838);
#5947=LINE('',#55927,#6839);
#5948=LINE('',#55935,#6840);
#5949=LINE('',#56121,#6841);
#5950=LINE('',#56123,#6842);
#5951=LINE('',#56307,#6843);
#5952=LINE('',#56315,#6844);
#5953=LINE('',#56507,#6845);
#5954=LINE('',#56509,#6846);
#5955=LINE('',#56691,#6847);
#5956=LINE('',#56699,#6848);
#5957=LINE('',#56865,#6849);
#5958=LINE('',#56878,#6850);
#5959=LINE('',#57089,#6851);
#5960=LINE('',#57102,#6852);
#5961=LINE('',#57287,#6853);
#5962=LINE('',#57300,#6854);
#5963=LINE('',#57485,#6855);
#5964=LINE('',#57498,#6856);
#5965=LINE('',#57683,#6857);
#5966=LINE('',#57696,#6858);
#5967=LINE('',#57881,#6859);
#5968=LINE('',#57894,#6860);
#5969=LINE('',#58093,#6861);
#5970=LINE('',#58119,#6862);
#5971=LINE('',#58304,#6863);
#5972=LINE('',#58317,#6864);
#5973=LINE('',#58502,#6865);
#5974=LINE('',#58515,#6866);
#5975=LINE('',#58700,#6867);
#5976=LINE('',#58713,#6868);
#5977=LINE('',#58898,#6869);
#5978=LINE('',#58911,#6870);
#5979=LINE('',#59096,#6871);
#5980=LINE('',#59109,#6872);
#5981=LINE('',#59310,#6873);
#5982=LINE('',#59323,#6874);
#5983=LINE('',#59520,#6875);
#5984=LINE('',#59533,#6876);
#5985=LINE('',#59718,#6877);
#5986=LINE('',#59731,#6878);
#5987=LINE('',#59916,#6879);
#5988=LINE('',#59929,#6880);
#5989=LINE('',#60114,#6881);
#5990=LINE('',#60127,#6882);
#5991=LINE('',#60312,#6883);
#5992=LINE('',#60325,#6884);
#5993=LINE('',#60524,#6885);
#5994=LINE('',#60537,#6886);
#5995=LINE('',#60734,#6887);
#5996=LINE('',#60747,#6888);
#5997=LINE('',#60932,#6889);
#5998=LINE('',#60945,#6890);
#5999=LINE('',#61130,#6891);
#6000=LINE('',#61143,#6892);
#6001=LINE('',#61328,#6893);
#6002=LINE('',#61341,#6894);
#6003=LINE('',#61526,#6895);
#6004=LINE('',#61539,#6896);
#6005=LINE('',#61724,#6897);
#6006=LINE('',#61737,#6898);
#6818=VECTOR('',#25209,3.18);
#6819=VECTOR('',#25214,3.03);
#6820=VECTOR('',#25281,3.18);
#6821=VECTOR('',#25384,10.);
#6822=VECTOR('',#25389,10.);
#6823=VECTOR('',#25398,10.);
#6824=VECTOR('',#25403,10.);
#6825=VECTOR('',#25562,10.);
#6826=VECTOR('',#25565,10.);
#6827=VECTOR('',#25572,10.);
#6828=VECTOR('',#25575,10.);
#6829=VECTOR('',#25582,10.);
#6830=VECTOR('',#25585,10.);
#6831=VECTOR('',#25592,10.);
#6832=VECTOR('',#25595,10.);
#6833=VECTOR('',#25602,10.);
#6834=VECTOR('',#25605,10.);
#6835=VECTOR('',#25612,10.);
#6836=VECTOR('',#25615,10.);
#6837=VECTOR('',#25622,10.);
#6838=VECTOR('',#25625,10.);
#6839=VECTOR('',#25632,10.);
#6840=VECTOR('',#25635,10.);
#6841=VECTOR('',#25642,10.);
#6842=VECTOR('',#25645,10.);
#6843=VECTOR('',#25652,10.);
#6844=VECTOR('',#25655,10.);
#6845=VECTOR('',#25662,10.);
#6846=VECTOR('',#25665,10.);
#6847=VECTOR('',#25672,10.);
#6848=VECTOR('',#25675,10.);
#6849=VECTOR('',#25676,10.);
#6850=VECTOR('',#25679,10.);
#6851=VECTOR('',#25690,10.);
#6852=VECTOR('',#25693,10.);
#6853=VECTOR('',#25704,10.);
#6854=VECTOR('',#25707,10.);
#6855=VECTOR('',#25718,10.);
#6856=VECTOR('',#25721,10.);
#6857=VECTOR('',#25732,10.);
#6858=VECTOR('',#25735,10.);
#6859=VECTOR('',#25746,10.);
#6860=VECTOR('',#25749,10.);
#6861=VECTOR('',#25760,10.);
#6862=VECTOR('',#25763,10.);
#6863=VECTOR('',#25774,10.);
#6864=VECTOR('',#25777,10.);
#6865=VECTOR('',#25788,10.);
#6866=VECTOR('',#25791,10.);
#6867=VECTOR('',#25802,10.);
#6868=VECTOR('',#25805,10.);
#6869=VECTOR('',#25816,10.);
#6870=VECTOR('',#25819,10.);
#6871=VECTOR('',#25830,10.);
#6872=VECTOR('',#25833,10.);
#6873=VECTOR('',#25844,10.);
#6874=VECTOR('',#25847,10.);
#6875=VECTOR('',#25858,10.);
#6876=VECTOR('',#25861,10.);
#6877=VECTOR('',#25872,10.);
#6878=VECTOR('',#25875,10.);
#6879=VECTOR('',#25886,10.);
#6880=VECTOR('',#25889,10.);
#6881=VECTOR('',#25900,10.);
#6882=VECTOR('',#25903,10.);
#6883=VECTOR('',#25914,10.);
#6884=VECTOR('',#25917,10.);
#6885=VECTOR('',#25928,10.);
#6886=VECTOR('',#25931,10.);
#6887=VECTOR('',#25942,10.);
#6888=VECTOR('',#25945,10.);
#6889=VECTOR('',#25956,10.);
#6890=VECTOR('',#25959,10.);
#6891=VECTOR('',#25970,10.);
#6892=VECTOR('',#25973,10.);
#6893=VECTOR('',#25984,10.);
#6894=VECTOR('',#25987,10.);
#6895=VECTOR('',#25998,10.);
#6896=VECTOR('',#26001,10.);
#6897=VECTOR('',#26012,10.);
#6898=VECTOR('',#26015,10.);
#8201=VERTEX_POINT('',#49229);
#8202=VERTEX_POINT('',#49230);
#8203=VERTEX_POINT('',#49233);
#8204=VERTEX_POINT('',#49237);
#8205=VERTEX_POINT('',#49239);
#8206=VERTEX_POINT('',#49243);
#8207=VERTEX_POINT('',#49244);
#8208=VERTEX_POINT('',#49270);
#8209=VERTEX_POINT('',#49272);
#8210=VERTEX_POINT('',#49302);
#8211=VERTEX_POINT('',#49304);
#8212=VERTEX_POINT('',#49330);
#8213=VERTEX_POINT('',#49332);
#8214=VERTEX_POINT('',#49362);
#8215=VERTEX_POINT('',#49364);
#8216=VERTEX_POINT('',#49390);
#8217=VERTEX_POINT('',#49392);
#8218=VERTEX_POINT('',#49422);
#8219=VERTEX_POINT('',#49424);
#8220=VERTEX_POINT('',#49450);
#8221=VERTEX_POINT('',#49452);
#8222=VERTEX_POINT('',#49482);
#8223=VERTEX_POINT('',#49484);
#8224=VERTEX_POINT('',#49510);
#8225=VERTEX_POINT('',#49512);
#8226=VERTEX_POINT('',#49542);
#8227=VERTEX_POINT('',#49544);
#8228=VERTEX_POINT('',#49570);
#8229=VERTEX_POINT('',#49572);
#8230=VERTEX_POINT('',#49602);
#8231=VERTEX_POINT('',#49604);
#8232=VERTEX_POINT('',#49630);
#8233=VERTEX_POINT('',#49632);
#8234=VERTEX_POINT('',#49662);
#8235=VERTEX_POINT('',#49664);
#8236=VERTEX_POINT('',#49690);
#8237=VERTEX_POINT('',#49692);
#8238=VERTEX_POINT('',#49722);
#8239=VERTEX_POINT('',#49724);
#8240=VERTEX_POINT('',#49750);
#8241=VERTEX_POINT('',#49752);
#8242=VERTEX_POINT('',#49782);
#8243=VERTEX_POINT('',#49784);
#8244=VERTEX_POINT('',#49810);
#8245=VERTEX_POINT('',#49812);
#8246=VERTEX_POINT('',#49842);
#8247=VERTEX_POINT('',#49844);
#8248=VERTEX_POINT('',#49870);
#8249=VERTEX_POINT('',#49872);
#8250=VERTEX_POINT('',#49902);
#8251=VERTEX_POINT('',#49904);
#8252=VERTEX_POINT('',#49930);
#8253=VERTEX_POINT('',#49932);
#8254=VERTEX_POINT('',#49962);
#8255=VERTEX_POINT('',#49964);
#8256=VERTEX_POINT('',#49990);
#8257=VERTEX_POINT('',#49992);
#8258=VERTEX_POINT('',#50022);
#8259=VERTEX_POINT('',#50024);
#8260=VERTEX_POINT('',#50050);
#8261=VERTEX_POINT('',#50052);
#8262=VERTEX_POINT('',#50084);
#8263=VERTEX_POINT('',#50088);
#8264=VERTEX_POINT('',#50089);
#8265=VERTEX_POINT('',#50119);
#8266=VERTEX_POINT('',#50121);
#8267=VERTEX_POINT('',#50148);
#8268=VERTEX_POINT('',#50150);
#8269=VERTEX_POINT('',#50180);
#8270=VERTEX_POINT('',#50182);
#8271=VERTEX_POINT('',#50209);
#8272=VERTEX_POINT('',#50211);
#8273=VERTEX_POINT('',#50241);
#8274=VERTEX_POINT('',#50243);
#8275=VERTEX_POINT('',#50270);
#8276=VERTEX_POINT('',#50272);
#8277=VERTEX_POINT('',#50302);
#8278=VERTEX_POINT('',#50304);
#8279=VERTEX_POINT('',#50331);
#8280=VERTEX_POINT('',#50333);
#8281=VERTEX_POINT('',#50363);
#8282=VERTEX_POINT('',#50365);
#8283=VERTEX_POINT('',#50392);
#8284=VERTEX_POINT('',#50394);
#8285=VERTEX_POINT('',#50424);
#8286=VERTEX_POINT('',#50426);
#8287=VERTEX_POINT('',#50453);
#8288=VERTEX_POINT('',#50455);
#8289=VERTEX_POINT('',#50485);
#8290=VERTEX_POINT('',#50487);
#8291=VERTEX_POINT('',#50514);
#8292=VERTEX_POINT('',#50516);
#8293=VERTEX_POINT('',#50546);
#8294=VERTEX_POINT('',#50548);
#8295=VERTEX_POINT('',#50575);
#8296=VERTEX_POINT('',#50577);
#8297=VERTEX_POINT('',#50607);
#8298=VERTEX_POINT('',#50609);
#8299=VERTEX_POINT('',#50636);
#8300=VERTEX_POINT('',#50638);
#8301=VERTEX_POINT('',#50668);
#8302=VERTEX_POINT('',#50670);
#8303=VERTEX_POINT('',#50697);
#8304=VERTEX_POINT('',#50699);
#8305=VERTEX_POINT('',#50729);
#8306=VERTEX_POINT('',#50731);
#8307=VERTEX_POINT('',#50758);
#8308=VERTEX_POINT('',#50760);
#8309=VERTEX_POINT('',#50790);
#8310=VERTEX_POINT('',#50792);
#8311=VERTEX_POINT('',#50819);
#8312=VERTEX_POINT('',#50821);
#8313=VERTEX_POINT('',#50851);
#8314=VERTEX_POINT('',#50853);
#8315=VERTEX_POINT('',#50880);
#8316=VERTEX_POINT('',#50882);
#8317=VERTEX_POINT('',#50912);
#8318=VERTEX_POINT('',#50914);
#8319=VERTEX_POINT('',#50941);
#8320=VERTEX_POINT('',#50943);
#8321=VERTEX_POINT('',#50973);
#8322=VERTEX_POINT('',#50975);
#8323=VERTEX_POINT('',#51002);
#8324=VERTEX_POINT('',#51004);
#8325=VERTEX_POINT('',#51034);
#8326=VERTEX_POINT('',#51036);
#8327=VERTEX_POINT('',#51063);
#8328=VERTEX_POINT('',#51065);
#8329=VERTEX_POINT('',#51095);
#8330=VERTEX_POINT('',#51097);
#8331=VERTEX_POINT('',#51124);
#8332=VERTEX_POINT('',#51126);
#8333=VERTEX_POINT('',#51156);
#8334=VERTEX_POINT('',#51158);
#8335=VERTEX_POINT('',#51185);
#8336=VERTEX_POINT('',#51187);
#8337=VERTEX_POINT('',#51217);
#8338=VERTEX_POINT('',#51219);
#8339=VERTEX_POINT('',#51246);
#8340=VERTEX_POINT('',#51248);
#8341=VERTEX_POINT('',#51278);
#8342=VERTEX_POINT('',#51280);
#8343=VERTEX_POINT('',#51307);
#8344=VERTEX_POINT('',#51309);
#8345=VERTEX_POINT('',#51339);
#8346=VERTEX_POINT('',#51341);
#8347=VERTEX_POINT('',#51368);
#8348=VERTEX_POINT('',#51370);
#8349=VERTEX_POINT('',#51400);
#8350=VERTEX_POINT('',#51402);
#8351=VERTEX_POINT('',#51429);
#8352=VERTEX_POINT('',#51431);
#8353=VERTEX_POINT('',#51461);
#8354=VERTEX_POINT('',#51463);
#8355=VERTEX_POINT('',#51490);
#8356=VERTEX_POINT('',#51492);
#8357=VERTEX_POINT('',#51522);
#8358=VERTEX_POINT('',#51524);
#8359=VERTEX_POINT('',#51551);
#8360=VERTEX_POINT('',#51553);
#8361=VERTEX_POINT('',#51583);
#8362=VERTEX_POINT('',#51585);
#8363=VERTEX_POINT('',#51693);
#8364=VERTEX_POINT('',#51701);
#8365=VERTEX_POINT('',#51703);
#8366=VERTEX_POINT('',#51745);
#8367=VERTEX_POINT('',#51828);
#8368=VERTEX_POINT('',#51835);
#8369=VERTEX_POINT('',#51872);
#8370=VERTEX_POINT('',#51881);
#8371=VERTEX_POINT('',#51969);
#8372=VERTEX_POINT('',#51970);
#8373=VERTEX_POINT('',#51977);
#8374=VERTEX_POINT('',#52015);
#8375=VERTEX_POINT('',#52098);
#8376=VERTEX_POINT('',#52099);
#8377=VERTEX_POINT('',#52145);
#8378=VERTEX_POINT('',#52146);
#8379=VERTEX_POINT('',#52176);
#8380=VERTEX_POINT('',#52178);
#8381=VERTEX_POINT('',#52205);
#8382=VERTEX_POINT('',#52207);
#8383=VERTEX_POINT('',#52237);
#8384=VERTEX_POINT('',#52239);
#8385=VERTEX_POINT('',#52266);
#8386=VERTEX_POINT('',#52268);
#8387=VERTEX_POINT('',#52298);
#8388=VERTEX_POINT('',#52300);
#8389=VERTEX_POINT('',#52327);
#8390=VERTEX_POINT('',#52329);
#8391=VERTEX_POINT('',#52359);
#8392=VERTEX_POINT('',#52361);
#8393=VERTEX_POINT('',#52388);
#8394=VERTEX_POINT('',#52390);
#8395=VERTEX_POINT('',#52420);
#8396=VERTEX_POINT('',#52422);
#8397=VERTEX_POINT('',#52449);
#8398=VERTEX_POINT('',#52451);
#8399=VERTEX_POINT('',#52481);
#8400=VERTEX_POINT('',#52483);
#8401=VERTEX_POINT('',#52510);
#8402=VERTEX_POINT('',#52512);
#8403=VERTEX_POINT('',#52542);
#8404=VERTEX_POINT('',#52544);
#8405=VERTEX_POINT('',#52571);
#8406=VERTEX_POINT('',#52573);
#8407=VERTEX_POINT('',#52603);
#8408=VERTEX_POINT('',#52605);
#8409=VERTEX_POINT('',#52632);
#8410=VERTEX_POINT('',#52634);
#8411=VERTEX_POINT('',#52664);
#8412=VERTEX_POINT('',#52666);
#8413=VERTEX_POINT('',#52693);
#8414=VERTEX_POINT('',#52695);
#8415=VERTEX_POINT('',#52725);
#8416=VERTEX_POINT('',#52727);
#8417=VERTEX_POINT('',#52754);
#8418=VERTEX_POINT('',#52756);
#8419=VERTEX_POINT('',#52786);
#8420=VERTEX_POINT('',#52788);
#8421=VERTEX_POINT('',#52815);
#8422=VERTEX_POINT('',#52817);
#8423=VERTEX_POINT('',#52847);
#8424=VERTEX_POINT('',#52849);
#8425=VERTEX_POINT('',#52876);
#8426=VERTEX_POINT('',#52878);
#8427=VERTEX_POINT('',#52908);
#8428=VERTEX_POINT('',#52910);
#8429=VERTEX_POINT('',#52937);
#8430=VERTEX_POINT('',#52939);
#8431=VERTEX_POINT('',#52969);
#8432=VERTEX_POINT('',#52971);
#8433=VERTEX_POINT('',#52998);
#8434=VERTEX_POINT('',#53000);
#8435=VERTEX_POINT('',#53030);
#8436=VERTEX_POINT('',#53032);
#8437=VERTEX_POINT('',#53059);
#8438=VERTEX_POINT('',#53061);
#8439=VERTEX_POINT('',#53091);
#8440=VERTEX_POINT('',#53093);
#8441=VERTEX_POINT('',#53120);
#8442=VERTEX_POINT('',#53122);
#8443=VERTEX_POINT('',#53152);
#8444=VERTEX_POINT('',#53154);
#8445=VERTEX_POINT('',#53181);
#8446=VERTEX_POINT('',#53183);
#8447=VERTEX_POINT('',#53213);
#8448=VERTEX_POINT('',#53215);
#8449=VERTEX_POINT('',#53242);
#8450=VERTEX_POINT('',#53244);
#8451=VERTEX_POINT('',#53274);
#8452=VERTEX_POINT('',#53276);
#8453=VERTEX_POINT('',#53303);
#8454=VERTEX_POINT('',#53305);
#8455=VERTEX_POINT('',#53335);
#8456=VERTEX_POINT('',#53337);
#8457=VERTEX_POINT('',#53364);
#8458=VERTEX_POINT('',#53366);
#8459=VERTEX_POINT('',#53396);
#8460=VERTEX_POINT('',#53398);
#8461=VERTEX_POINT('',#53425);
#8462=VERTEX_POINT('',#53427);
#8463=VERTEX_POINT('',#53457);
#8464=VERTEX_POINT('',#53459);
#8465=VERTEX_POINT('',#53486);
#8466=VERTEX_POINT('',#53488);
#8467=VERTEX_POINT('',#53518);
#8468=VERTEX_POINT('',#53520);
#8469=VERTEX_POINT('',#53547);
#8470=VERTEX_POINT('',#53549);
#8471=VERTEX_POINT('',#53579);
#8472=VERTEX_POINT('',#53581);
#8473=VERTEX_POINT('',#53608);
#8474=VERTEX_POINT('',#53610);
#8475=VERTEX_POINT('',#53640);
#8476=VERTEX_POINT('',#53642);
#8477=VERTEX_POINT('',#53671);
#8478=VERTEX_POINT('',#53673);
#8479=VERTEX_POINT('',#53708);
#8480=VERTEX_POINT('',#53710);
#8481=VERTEX_POINT('',#53740);
#8482=VERTEX_POINT('',#53742);
#8483=VERTEX_POINT('',#53777);
#8484=VERTEX_POINT('',#53779);
#8485=VERTEX_POINT('',#53809);
#8486=VERTEX_POINT('',#53811);
#8487=VERTEX_POINT('',#53846);
#8488=VERTEX_POINT('',#53848);
#8489=VERTEX_POINT('',#53878);
#8490=VERTEX_POINT('',#53880);
#8491=VERTEX_POINT('',#53915);
#8492=VERTEX_POINT('',#53917);
#8493=VERTEX_POINT('',#53947);
#8494=VERTEX_POINT('',#53949);
#8495=VERTEX_POINT('',#53984);
#8496=VERTEX_POINT('',#53986);
#8497=VERTEX_POINT('',#54016);
#8498=VERTEX_POINT('',#54018);
#8499=VERTEX_POINT('',#54053);
#8500=VERTEX_POINT('',#54055);
#8501=VERTEX_POINT('',#54085);
#8502=VERTEX_POINT('',#54087);
#8503=VERTEX_POINT('',#54122);
#8504=VERTEX_POINT('',#54124);
#8505=VERTEX_POINT('',#54154);
#8506=VERTEX_POINT('',#54156);
#8507=VERTEX_POINT('',#54191);
#8508=VERTEX_POINT('',#54193);
#8509=VERTEX_POINT('',#54223);
#8510=VERTEX_POINT('',#54225);
#8511=VERTEX_POINT('',#54260);
#8512=VERTEX_POINT('',#54262);
#8513=VERTEX_POINT('',#54292);
#8514=VERTEX_POINT('',#54294);
#8515=VERTEX_POINT('',#54329);
#8516=VERTEX_POINT('',#54331);
#8517=VERTEX_POINT('',#54361);
#8518=VERTEX_POINT('',#54363);
#8519=VERTEX_POINT('',#54398);
#8520=VERTEX_POINT('',#54400);
#8521=VERTEX_POINT('',#54430);
#8522=VERTEX_POINT('',#54432);
#8523=VERTEX_POINT('',#54467);
#8524=VERTEX_POINT('',#54499);
#8525=VERTEX_POINT('',#54675);
#8526=VERTEX_POINT('',#54771);
#8527=VERTEX_POINT('',#54867);
#8528=VERTEX_POINT('',#54879);
#8529=VERTEX_POINT('',#55061);
#8530=VERTEX_POINT('',#55157);
#8531=VERTEX_POINT('',#55253);
#8532=VERTEX_POINT('',#55265);
#8533=VERTEX_POINT('',#55441);
#8534=VERTEX_POINT('',#55537);
#8535=VERTEX_POINT('',#55633);
#8536=VERTEX_POINT('',#55648);
#8537=VERTEX_POINT('',#55824);
#8538=VERTEX_POINT('',#55920);
#8539=VERTEX_POINT('',#56016);
#8540=VERTEX_POINT('',#56028);
#8541=VERTEX_POINT('',#56204);
#8542=VERTEX_POINT('',#56300);
#8543=VERTEX_POINT('',#56396);
#8544=VERTEX_POINT('',#56414);
#8545=VERTEX_POINT('',#56590);
#8546=VERTEX_POINT('',#56686);
#8547=VERTEX_POINT('',#56860);
#8548=VERTEX_POINT('',#56866);
#8549=VERTEX_POINT('',#56959);
#8550=VERTEX_POINT('',#56970);
#8551=VERTEX_POINT('',#56986);
#8552=VERTEX_POINT('',#56993);
#8553=VERTEX_POINT('',#57084);
#8554=VERTEX_POINT('',#57090);
#8555=VERTEX_POINT('',#57184);
#8556=VERTEX_POINT('',#57191);
#8557=VERTEX_POINT('',#57282);
#8558=VERTEX_POINT('',#57288);
#8559=VERTEX_POINT('',#57382);
#8560=VERTEX_POINT('',#57389);
#8561=VERTEX_POINT('',#57480);
#8562=VERTEX_POINT('',#57486);
#8563=VERTEX_POINT('',#57580);
#8564=VERTEX_POINT('',#57587);
#8565=VERTEX_POINT('',#57678);
#8566=VERTEX_POINT('',#57684);
#8567=VERTEX_POINT('',#57778);
#8568=VERTEX_POINT('',#57785);
#8569=VERTEX_POINT('',#57876);
#8570=VERTEX_POINT('',#57882);
#8571=VERTEX_POINT('',#57976);
#8572=VERTEX_POINT('',#57989);
#8573=VERTEX_POINT('',#58086);
#8574=VERTEX_POINT('',#58094);
#8575=VERTEX_POINT('',#58201);
#8576=VERTEX_POINT('',#58208);
#8577=VERTEX_POINT('',#58299);
#8578=VERTEX_POINT('',#58305);
#8579=VERTEX_POINT('',#58399);
#8580=VERTEX_POINT('',#58406);
#8581=VERTEX_POINT('',#58497);
#8582=VERTEX_POINT('',#58503);
#8583=VERTEX_POINT('',#58597);
#8584=VERTEX_POINT('',#58604);
#8585=VERTEX_POINT('',#58695);
#8586=VERTEX_POINT('',#58701);
#8587=VERTEX_POINT('',#58795);
#8588=VERTEX_POINT('',#58802);
#8589=VERTEX_POINT('',#58893);
#8590=VERTEX_POINT('',#58899);
#8591=VERTEX_POINT('',#58993);
#8592=VERTEX_POINT('',#59000);
#8593=VERTEX_POINT('',#59091);
#8594=VERTEX_POINT('',#59097);
#8595=VERTEX_POINT('',#59191);
#8596=VERTEX_POINT('',#59204);
#8597=VERTEX_POINT('',#59301);
#8598=VERTEX_POINT('',#59311);
#8599=VERTEX_POINT('',#59405);
#8600=VERTEX_POINT('',#59418);
#8601=VERTEX_POINT('',#59515);
#8602=VERTEX_POINT('',#59521);
#8603=VERTEX_POINT('',#59615);
#8604=VERTEX_POINT('',#59622);
#8605=VERTEX_POINT('',#59713);
#8606=VERTEX_POINT('',#59719);
#8607=VERTEX_POINT('',#59813);
#8608=VERTEX_POINT('',#59820);
#8609=VERTEX_POINT('',#59911);
#8610=VERTEX_POINT('',#59917);
#8611=VERTEX_POINT('',#60011);
#8612=VERTEX_POINT('',#60018);
#8613=VERTEX_POINT('',#60109);
#8614=VERTEX_POINT('',#60115);
#8615=VERTEX_POINT('',#60209);
#8616=VERTEX_POINT('',#60216);
#8617=VERTEX_POINT('',#60307);
#8618=VERTEX_POINT('',#60313);
#8619=VERTEX_POINT('',#60407);
#8620=VERTEX_POINT('',#60420);
#8621=VERTEX_POINT('',#60517);
#8622=VERTEX_POINT('',#60525);
#8623=VERTEX_POINT('',#60619);
#8624=VERTEX_POINT('',#60632);
#8625=VERTEX_POINT('',#60729);
#8626=VERTEX_POINT('',#60735);
#8627=VERTEX_POINT('',#60829);
#8628=VERTEX_POINT('',#60836);
#8629=VERTEX_POINT('',#60927);
#8630=VERTEX_POINT('',#60933);
#8631=VERTEX_POINT('',#61027);
#8632=VERTEX_POINT('',#61034);
#8633=VERTEX_POINT('',#61125);
#8634=VERTEX_POINT('',#61131);
#8635=VERTEX_POINT('',#61225);
#8636=VERTEX_POINT('',#61232);
#8637=VERTEX_POINT('',#61323);
#8638=VERTEX_POINT('',#61329);
#8639=VERTEX_POINT('',#61423);
#8640=VERTEX_POINT('',#61430);
#8641=VERTEX_POINT('',#61521);
#8642=VERTEX_POINT('',#61527);
#8643=VERTEX_POINT('',#61621);
#8644=VERTEX_POINT('',#61628);
#8645=VERTEX_POINT('',#61719);
#8646=VERTEX_POINT('',#61725);
#10715=EDGE_CURVE('',#8201,#8202,#4076,.T.);
#10716=EDGE_CURVE('',#8202,#8201,#4077,.T.);
#10717=EDGE_CURVE('',#8201,#8203,#5926,.T.);
#10718=EDGE_CURVE('',#8203,#8203,#4078,.T.);
#10719=EDGE_CURVE('',#8202,#8204,#5927,.T.);
#10720=EDGE_CURVE('',#8205,#8204,#4079,.T.);
#10721=EDGE_CURVE('',#8204,#8205,#4080,.T.);
#10722=EDGE_CURVE('',#8206,#8207,#672,.T.);
#10723=EDGE_CURVE('',#8207,#8208,#4081,.T.);
#10724=EDGE_CURVE('',#8208,#8209,#673,.T.);
#10725=EDGE_CURVE('',#8209,#8210,#4082,.T.);
#10726=EDGE_CURVE('',#8210,#8211,#674,.T.);
#10727=EDGE_CURVE('',#8211,#8212,#4083,.T.);
#10728=EDGE_CURVE('',#8212,#8213,#675,.T.);
#10729=EDGE_CURVE('',#8213,#8214,#4084,.T.);
#10730=EDGE_CURVE('',#8214,#8215,#676,.T.);
#10731=EDGE_CURVE('',#8215,#8216,#4085,.T.);
#10732=EDGE_CURVE('',#8216,#8217,#677,.T.);
#10733=EDGE_CURVE('',#8217,#8218,#4086,.T.);
#10734=EDGE_CURVE('',#8218,#8219,#678,.T.);
#10735=EDGE_CURVE('',#8219,#8220,#4087,.T.);
#10736=EDGE_CURVE('',#8220,#8221,#679,.T.);
#10737=EDGE_CURVE('',#8221,#8222,#4088,.T.);
#10738=EDGE_CURVE('',#8222,#8223,#680,.T.);
#10739=EDGE_CURVE('',#8223,#8224,#4089,.T.);
#10740=EDGE_CURVE('',#8224,#8225,#681,.T.);
#10741=EDGE_CURVE('',#8225,#8226,#4090,.T.);
#10742=EDGE_CURVE('',#8226,#8227,#682,.T.);
#10743=EDGE_CURVE('',#8227,#8228,#4091,.T.);
#10744=EDGE_CURVE('',#8228,#8229,#683,.T.);
#10745=EDGE_CURVE('',#8229,#8230,#4092,.T.);
#10746=EDGE_CURVE('',#8230,#8231,#684,.T.);
#10747=EDGE_CURVE('',#8231,#8232,#4093,.T.);
#10748=EDGE_CURVE('',#8232,#8233,#685,.T.);
#10749=EDGE_CURVE('',#8233,#8234,#4094,.T.);
#10750=EDGE_CURVE('',#8234,#8235,#686,.T.);
#10751=EDGE_CURVE('',#8235,#8236,#4095,.T.);
#10752=EDGE_CURVE('',#8236,#8237,#687,.T.);
#10753=EDGE_CURVE('',#8237,#8238,#4096,.T.);
#10754=EDGE_CURVE('',#8238,#8239,#688,.T.);
#10755=EDGE_CURVE('',#8239,#8240,#4097,.T.);
#10756=EDGE_CURVE('',#8240,#8241,#689,.T.);
#10757=EDGE_CURVE('',#8241,#8242,#4098,.T.);
#10758=EDGE_CURVE('',#8242,#8243,#690,.T.);
#10759=EDGE_CURVE('',#8243,#8244,#4099,.T.);
#10760=EDGE_CURVE('',#8244,#8245,#691,.T.);
#10761=EDGE_CURVE('',#8245,#8246,#4100,.T.);
#10762=EDGE_CURVE('',#8246,#8247,#692,.T.);
#10763=EDGE_CURVE('',#8247,#8248,#4101,.T.);
#10764=EDGE_CURVE('',#8248,#8249,#693,.T.);
#10765=EDGE_CURVE('',#8249,#8250,#4102,.T.);
#10766=EDGE_CURVE('',#8250,#8251,#694,.T.);
#10767=EDGE_CURVE('',#8251,#8252,#4103,.T.);
#10768=EDGE_CURVE('',#8252,#8253,#695,.T.);
#10769=EDGE_CURVE('',#8253,#8254,#4104,.T.);
#10770=EDGE_CURVE('',#8254,#8255,#696,.T.);
#10771=EDGE_CURVE('',#8255,#8256,#4105,.T.);
#10772=EDGE_CURVE('',#8256,#8257,#697,.T.);
#10773=EDGE_CURVE('',#8257,#8258,#4106,.T.);
#10774=EDGE_CURVE('',#8258,#8259,#698,.T.);
#10775=EDGE_CURVE('',#8259,#8260,#4107,.T.);
#10776=EDGE_CURVE('',#8260,#8261,#699,.T.);
#10777=EDGE_CURVE('',#8261,#8206,#4108,.T.);
#10778=EDGE_CURVE('',#8262,#8262,#4109,.T.);
#10779=EDGE_CURVE('',#8262,#8205,#5928,.T.);
#10780=EDGE_CURVE('',#8263,#8264,#700,.T.);
#10781=EDGE_CURVE('',#8264,#8265,#4110,.T.);
#10782=EDGE_CURVE('',#8265,#8266,#701,.T.);
#10783=EDGE_CURVE('',#8267,#8266,#4111,.T.);
#10784=EDGE_CURVE('',#8267,#8268,#702,.T.);
#10785=EDGE_CURVE('',#8268,#8269,#4112,.T.);
#10786=EDGE_CURVE('',#8269,#8270,#703,.T.);
#10787=EDGE_CURVE('',#8271,#8270,#4113,.T.);
#10788=EDGE_CURVE('',#8271,#8272,#704,.T.);
#10789=EDGE_CURVE('',#8272,#8273,#4114,.T.);
#10790=EDGE_CURVE('',#8273,#8274,#705,.T.);
#10791=EDGE_CURVE('',#8275,#8274,#4115,.T.);
#10792=EDGE_CURVE('',#8275,#8276,#706,.T.);
#10793=EDGE_CURVE('',#8276,#8277,#4116,.T.);
#10794=EDGE_CURVE('',#8277,#8278,#707,.T.);
#10795=EDGE_CURVE('',#8279,#8278,#4117,.T.);
#10796=EDGE_CURVE('',#8279,#8280,#708,.T.);
#10797=EDGE_CURVE('',#8280,#8281,#4118,.T.);
#10798=EDGE_CURVE('',#8281,#8282,#709,.T.);
#10799=EDGE_CURVE('',#8283,#8282,#4119,.T.);
#10800=EDGE_CURVE('',#8283,#8284,#710,.T.);
#10801=EDGE_CURVE('',#8284,#8285,#4120,.T.);
#10802=EDGE_CURVE('',#8285,#8286,#711,.T.);
#10803=EDGE_CURVE('',#8287,#8286,#4121,.T.);
#10804=EDGE_CURVE('',#8287,#8288,#712,.T.);
#10805=EDGE_CURVE('',#8288,#8289,#4122,.T.);
#10806=EDGE_CURVE('',#8289,#8290,#713,.T.);
#10807=EDGE_CURVE('',#8291,#8290,#4123,.T.);
#10808=EDGE_CURVE('',#8291,#8292,#714,.T.);
#10809=EDGE_CURVE('',#8292,#8293,#4124,.T.);
#10810=EDGE_CURVE('',#8293,#8294,#715,.T.);
#10811=EDGE_CURVE('',#8295,#8294,#4125,.T.);
#10812=EDGE_CURVE('',#8295,#8296,#716,.T.);
#10813=EDGE_CURVE('',#8296,#8297,#4126,.T.);
#10814=EDGE_CURVE('',#8297,#8298,#717,.T.);
#10815=EDGE_CURVE('',#8299,#8298,#4127,.T.);
#10816=EDGE_CURVE('',#8299,#8300,#718,.T.);
#10817=EDGE_CURVE('',#8300,#8301,#4128,.T.);
#10818=EDGE_CURVE('',#8301,#8302,#719,.T.);
#10819=EDGE_CURVE('',#8303,#8302,#4129,.T.);
#10820=EDGE_CURVE('',#8303,#8304,#720,.T.);
#10821=EDGE_CURVE('',#8304,#8305,#4130,.T.);
#10822=EDGE_CURVE('',#8305,#8306,#721,.T.);
#10823=EDGE_CURVE('',#8307,#8306,#4131,.T.);
#10824=EDGE_CURVE('',#8307,#8308,#722,.T.);
#10825=EDGE_CURVE('',#8308,#8309,#4132,.T.);
#10826=EDGE_CURVE('',#8309,#8310,#723,.T.);
#10827=EDGE_CURVE('',#8311,#8310,#4133,.T.);
#10828=EDGE_CURVE('',#8311,#8312,#724,.T.);
#10829=EDGE_CURVE('',#8312,#8313,#4134,.T.);
#10830=EDGE_CURVE('',#8313,#8314,#725,.T.);
#10831=EDGE_CURVE('',#8315,#8314,#4135,.T.);
#10832=EDGE_CURVE('',#8315,#8316,#726,.T.);
#10833=EDGE_CURVE('',#8316,#8317,#4136,.T.);
#10834=EDGE_CURVE('',#8317,#8318,#727,.T.);
#10835=EDGE_CURVE('',#8319,#8318,#4137,.T.);
#10836=EDGE_CURVE('',#8319,#8320,#728,.T.);
#10837=EDGE_CURVE('',#8320,#8321,#4138,.T.);
#10838=EDGE_CURVE('',#8321,#8322,#729,.T.);
#10839=EDGE_CURVE('',#8323,#8322,#4139,.T.);
#10840=EDGE_CURVE('',#8323,#8324,#730,.T.);
#10841=EDGE_CURVE('',#8324,#8325,#4140,.T.);
#10842=EDGE_CURVE('',#8325,#8326,#731,.T.);
#10843=EDGE_CURVE('',#8327,#8326,#4141,.T.);
#10844=EDGE_CURVE('',#8327,#8328,#732,.T.);
#10845=EDGE_CURVE('',#8328,#8329,#4142,.T.);
#10846=EDGE_CURVE('',#8329,#8330,#733,.T.);
#10847=EDGE_CURVE('',#8331,#8330,#4143,.T.);
#10848=EDGE_CURVE('',#8331,#8332,#734,.T.);
#10849=EDGE_CURVE('',#8332,#8333,#4144,.T.);
#10850=EDGE_CURVE('',#8333,#8334,#735,.T.);
#10851=EDGE_CURVE('',#8335,#8334,#4145,.T.);
#10852=EDGE_CURVE('',#8335,#8336,#736,.T.);
#10853=EDGE_CURVE('',#8336,#8337,#4146,.T.);
#10854=EDGE_CURVE('',#8337,#8338,#737,.T.);
#10855=EDGE_CURVE('',#8339,#8338,#4147,.T.);
#10856=EDGE_CURVE('',#8339,#8340,#738,.T.);
#10857=EDGE_CURVE('',#8340,#8341,#4148,.T.);
#10858=EDGE_CURVE('',#8341,#8342,#739,.T.);
#10859=EDGE_CURVE('',#8343,#8342,#4149,.T.);
#10860=EDGE_CURVE('',#8343,#8344,#740,.T.);
#10861=EDGE_CURVE('',#8344,#8345,#4150,.T.);
#10862=EDGE_CURVE('',#8345,#8346,#741,.T.);
#10863=EDGE_CURVE('',#8347,#8346,#4151,.T.);
#10864=EDGE_CURVE('',#8347,#8348,#742,.T.);
#10865=EDGE_CURVE('',#8348,#8349,#4152,.T.);
#10866=EDGE_CURVE('',#8349,#8350,#743,.T.);
#10867=EDGE_CURVE('',#8351,#8350,#4153,.T.);
#10868=EDGE_CURVE('',#8351,#8352,#744,.T.);
#10869=EDGE_CURVE('',#8352,#8353,#4154,.T.);
#10870=EDGE_CURVE('',#8353,#8354,#745,.T.);
#10871=EDGE_CURVE('',#8355,#8354,#4155,.T.);
#10872=EDGE_CURVE('',#8355,#8356,#746,.T.);
#10873=EDGE_CURVE('',#8356,#8357,#4156,.T.);
#10874=EDGE_CURVE('',#8357,#8358,#747,.T.);
#10875=EDGE_CURVE('',#8359,#8358,#4157,.T.);
#10876=EDGE_CURVE('',#8359,#8360,#748,.T.);
#10877=EDGE_CURVE('',#8360,#8361,#4158,.T.);
#10878=EDGE_CURVE('',#8361,#8362,#749,.T.);
#10879=EDGE_CURVE('',#8263,#8362,#4159,.T.);
#10880=EDGE_CURVE('',#8209,#8363,#5142,.T.);
#10881=EDGE_CURVE('',#8364,#8208,#5929,.T.);
#10882=EDGE_CURVE('',#8364,#8365,#750,.T.);
#10883=EDGE_CURVE('',#8363,#8365,#5143,.T.);
#10884=EDGE_CURVE('',#8366,#8364,#4160,.T.);
#10885=EDGE_CURVE('',#8366,#8207,#5930,.T.);
#10886=EDGE_CURVE('',#8367,#8206,#5144,.T.);
#10887=EDGE_CURVE('',#8368,#8367,#5145,.T.);
#10888=EDGE_CURVE('',#8368,#8366,#751,.T.);
#10889=EDGE_CURVE('',#8363,#8369,#4161,.T.);
#10890=EDGE_CURVE('',#8369,#8210,#5146,.T.);
#10891=EDGE_CURVE('',#8365,#8370,#4162,.T.);
#10892=EDGE_CURVE('',#8370,#8369,#5147,.T.);
#10893=EDGE_CURVE('',#8371,#8372,#5148,.T.);
#10894=EDGE_CURVE('',#8371,#8373,#752,.T.);
#10895=EDGE_CURVE('',#8373,#8259,#5931,.T.);
#10896=EDGE_CURVE('',#8372,#8258,#5149,.T.);
#10897=EDGE_CURVE('',#8373,#8374,#4163,.T.);
#10898=EDGE_CURVE('',#8374,#8260,#5932,.T.);
#10899=EDGE_CURVE('',#8375,#8376,#5150,.T.);
#10900=EDGE_CURVE('',#8261,#8375,#5151,.T.);
#10901=EDGE_CURVE('',#8374,#8376,#753,.T.);
#10902=EDGE_CURVE('',#8377,#8378,#754,.T.);
#10903=EDGE_CURVE('',#8378,#8379,#4164,.T.);
#10904=EDGE_CURVE('',#8379,#8380,#755,.T.);
#10905=EDGE_CURVE('',#8380,#8381,#4165,.T.);
#10906=EDGE_CURVE('',#8381,#8382,#756,.T.);
#10907=EDGE_CURVE('',#8382,#8383,#4166,.T.);
#10908=EDGE_CURVE('',#8383,#8384,#757,.T.);
#10909=EDGE_CURVE('',#8384,#8385,#4167,.T.);
#10910=EDGE_CURVE('',#8385,#8386,#758,.T.);
#10911=EDGE_CURVE('',#8386,#8387,#4168,.T.);
#10912=EDGE_CURVE('',#8387,#8388,#759,.T.);
#10913=EDGE_CURVE('',#8388,#8389,#4169,.T.);
#10914=EDGE_CURVE('',#8389,#8390,#760,.T.);
#10915=EDGE_CURVE('',#8390,#8391,#4170,.T.);
#10916=EDGE_CURVE('',#8391,#8392,#761,.T.);
#10917=EDGE_CURVE('',#8392,#8393,#4171,.T.);
#10918=EDGE_CURVE('',#8393,#8394,#762,.T.);
#10919=EDGE_CURVE('',#8394,#8395,#4172,.T.);
#10920=EDGE_CURVE('',#8395,#8396,#763,.T.);
#10921=EDGE_CURVE('',#8396,#8397,#4173,.T.);
#10922=EDGE_CURVE('',#8397,#8398,#764,.T.);
#10923=EDGE_CURVE('',#8398,#8399,#4174,.T.);
#10924=EDGE_CURVE('',#8399,#8400,#765,.T.);
#10925=EDGE_CURVE('',#8400,#8401,#4175,.T.);
#10926=EDGE_CURVE('',#8401,#8402,#766,.T.);
#10927=EDGE_CURVE('',#8402,#8403,#4176,.T.);
#10928=EDGE_CURVE('',#8403,#8404,#767,.T.);
#10929=EDGE_CURVE('',#8404,#8405,#4177,.T.);
#10930=EDGE_CURVE('',#8405,#8406,#768,.T.);
#10931=EDGE_CURVE('',#8406,#8407,#4178,.T.);
#10932=EDGE_CURVE('',#8407,#8408,#769,.T.);
#10933=EDGE_CURVE('',#8408,#8409,#4179,.T.);
#10934=EDGE_CURVE('',#8409,#8410,#770,.T.);
#10935=EDGE_CURVE('',#8410,#8411,#4180,.T.);
#10936=EDGE_CURVE('',#8411,#8412,#771,.T.);
#10937=EDGE_CURVE('',#8412,#8413,#4181,.T.);
#10938=EDGE_CURVE('',#8413,#8414,#772,.T.);
#10939=EDGE_CURVE('',#8414,#8415,#4182,.T.);
#10940=EDGE_CURVE('',#8415,#8416,#773,.T.);
#10941=EDGE_CURVE('',#8416,#8417,#4183,.T.);
#10942=EDGE_CURVE('',#8417,#8418,#774,.T.);
#10943=EDGE_CURVE('',#8418,#8419,#4184,.T.);
#10944=EDGE_CURVE('',#8419,#8420,#775,.T.);
#10945=EDGE_CURVE('',#8420,#8421,#4185,.T.);
#10946=EDGE_CURVE('',#8421,#8422,#776,.T.);
#10947=EDGE_CURVE('',#8422,#8423,#4186,.T.);
#10948=EDGE_CURVE('',#8423,#8424,#777,.T.);
#10949=EDGE_CURVE('',#8424,#8425,#4187,.T.);
#10950=EDGE_CURVE('',#8425,#8426,#778,.T.);
#10951=EDGE_CURVE('',#8426,#8427,#4188,.T.);
#10952=EDGE_CURVE('',#8427,#8428,#779,.T.);
#10953=EDGE_CURVE('',#8428,#8429,#4189,.T.);
#10954=EDGE_CURVE('',#8429,#8430,#780,.T.);
#10955=EDGE_CURVE('',#8430,#8431,#4190,.T.);
#10956=EDGE_CURVE('',#8431,#8432,#781,.T.);
#10957=EDGE_CURVE('',#8432,#8433,#4191,.T.);
#10958=EDGE_CURVE('',#8433,#8434,#782,.T.);
#10959=EDGE_CURVE('',#8434,#8435,#4192,.T.);
#10960=EDGE_CURVE('',#8435,#8436,#783,.T.);
#10961=EDGE_CURVE('',#8436,#8437,#4193,.T.);
#10962=EDGE_CURVE('',#8437,#8438,#784,.T.);
#10963=EDGE_CURVE('',#8438,#8439,#4194,.T.);
#10964=EDGE_CURVE('',#8439,#8440,#785,.T.);
#10965=EDGE_CURVE('',#8440,#8441,#4195,.T.);
#10966=EDGE_CURVE('',#8441,#8442,#786,.T.);
#10967=EDGE_CURVE('',#8442,#8443,#4196,.T.);
#10968=EDGE_CURVE('',#8443,#8444,#787,.T.);
#10969=EDGE_CURVE('',#8444,#8445,#4197,.T.);
#10970=EDGE_CURVE('',#8445,#8446,#788,.T.);
#10971=EDGE_CURVE('',#8446,#8447,#4198,.T.);
#10972=EDGE_CURVE('',#8447,#8448,#789,.T.);
#10973=EDGE_CURVE('',#8448,#8449,#4199,.T.);
#10974=EDGE_CURVE('',#8449,#8450,#790,.T.);
#10975=EDGE_CURVE('',#8450,#8451,#4200,.T.);
#10976=EDGE_CURVE('',#8451,#8452,#791,.T.);
#10977=EDGE_CURVE('',#8452,#8453,#4201,.T.);
#10978=EDGE_CURVE('',#8453,#8454,#792,.T.);
#10979=EDGE_CURVE('',#8454,#8455,#4202,.T.);
#10980=EDGE_CURVE('',#8455,#8456,#793,.T.);
#10981=EDGE_CURVE('',#8456,#8457,#4203,.T.);
#10982=EDGE_CURVE('',#8457,#8458,#794,.T.);
#10983=EDGE_CURVE('',#8458,#8459,#4204,.T.);
#10984=EDGE_CURVE('',#8459,#8460,#795,.T.);
#10985=EDGE_CURVE('',#8460,#8461,#4205,.T.);
#10986=EDGE_CURVE('',#8461,#8462,#796,.T.);
#10987=EDGE_CURVE('',#8462,#8463,#4206,.T.);
#10988=EDGE_CURVE('',#8463,#8464,#797,.T.);
#10989=EDGE_CURVE('',#8464,#8465,#4207,.T.);
#10990=EDGE_CURVE('',#8465,#8466,#798,.T.);
#10991=EDGE_CURVE('',#8466,#8467,#4208,.T.);
#10992=EDGE_CURVE('',#8467,#8468,#799,.T.);
#10993=EDGE_CURVE('',#8468,#8469,#4209,.T.);
#10994=EDGE_CURVE('',#8469,#8470,#800,.T.);
#10995=EDGE_CURVE('',#8470,#8471,#4210,.T.);
#10996=EDGE_CURVE('',#8471,#8472,#801,.T.);
#10997=EDGE_CURVE('',#8472,#8473,#4211,.T.);
#10998=EDGE_CURVE('',#8473,#8474,#802,.T.);
#10999=EDGE_CURVE('',#8474,#8475,#4212,.T.);
#11000=EDGE_CURVE('',#8475,#8476,#803,.T.);
#11001=EDGE_CURVE('',#8476,#8377,#4213,.T.);
#11002=EDGE_CURVE('',#8376,#8368,#4214,.T.);
#11003=EDGE_CURVE('',#8477,#8371,#4215,.T.);
#11004=EDGE_CURVE('',#8478,#8477,#804,.T.);
#11005=EDGE_CURVE('',#8479,#8478,#4216,.T.);
#11006=EDGE_CURVE('',#8480,#8479,#805,.T.);
#11007=EDGE_CURVE('',#8481,#8480,#4217,.T.);
#11008=EDGE_CURVE('',#8482,#8481,#806,.T.);
#11009=EDGE_CURVE('',#8483,#8482,#4218,.T.);
#11010=EDGE_CURVE('',#8484,#8483,#807,.T.);
#11011=EDGE_CURVE('',#8485,#8484,#4219,.T.);
#11012=EDGE_CURVE('',#8486,#8485,#808,.T.);
#11013=EDGE_CURVE('',#8487,#8486,#4220,.T.);
#11014=EDGE_CURVE('',#8488,#8487,#809,.T.);
#11015=EDGE_CURVE('',#8489,#8488,#4221,.T.);
#11016=EDGE_CURVE('',#8490,#8489,#810,.T.);
#11017=EDGE_CURVE('',#8491,#8490,#4222,.T.);
#11018=EDGE_CURVE('',#8492,#8491,#811,.T.);
#11019=EDGE_CURVE('',#8493,#8492,#4223,.T.);
#11020=EDGE_CURVE('',#8494,#8493,#812,.T.);
#11021=EDGE_CURVE('',#8495,#8494,#4224,.T.);
#11022=EDGE_CURVE('',#8496,#8495,#813,.T.);
#11023=EDGE_CURVE('',#8497,#8496,#4225,.T.);
#11024=EDGE_CURVE('',#8498,#8497,#814,.T.);
#11025=EDGE_CURVE('',#8499,#8498,#4226,.T.);
#11026=EDGE_CURVE('',#8500,#8499,#815,.T.);
#11027=EDGE_CURVE('',#8501,#8500,#4227,.T.);
#11028=EDGE_CURVE('',#8502,#8501,#816,.T.);
#11029=EDGE_CURVE('',#8503,#8502,#4228,.T.);
#11030=EDGE_CURVE('',#8504,#8503,#817,.T.);
#11031=EDGE_CURVE('',#8505,#8504,#4229,.T.);
#11032=EDGE_CURVE('',#8506,#8505,#818,.T.);
#11033=EDGE_CURVE('',#8507,#8506,#4230,.T.);
#11034=EDGE_CURVE('',#8508,#8507,#819,.T.);
#11035=EDGE_CURVE('',#8509,#8508,#4231,.T.);
#11036=EDGE_CURVE('',#8510,#8509,#820,.T.);
#11037=EDGE_CURVE('',#8511,#8510,#4232,.T.);
#11038=EDGE_CURVE('',#8512,#8511,#821,.T.);
#11039=EDGE_CURVE('',#8513,#8512,#4233,.T.);
#11040=EDGE_CURVE('',#8514,#8513,#822,.T.);
#11041=EDGE_CURVE('',#8515,#8514,#4234,.T.);
#11042=EDGE_CURVE('',#8516,#8515,#823,.T.);
#11043=EDGE_CURVE('',#8517,#8516,#4235,.T.);
#11044=EDGE_CURVE('',#8518,#8517,#824,.T.);
#11045=EDGE_CURVE('',#8519,#8518,#4236,.T.);
#11046=EDGE_CURVE('',#8520,#8519,#825,.T.);
#11047=EDGE_CURVE('',#8521,#8520,#4237,.T.);
#11048=EDGE_CURVE('',#8522,#8521,#826,.T.);
#11049=EDGE_CURVE('',#8523,#8522,#4238,.T.);
#11050=EDGE_CURVE('',#8370,#8523,#827,.T.);
#11051=EDGE_CURVE('',#8524,#8372,#4239,.T.);
#11052=EDGE_CURVE('',#8524,#8477,#5152,.T.);
#11053=EDGE_CURVE('',#8257,#8524,#5153,.T.);
#11054=EDGE_CURVE('',#8478,#8256,#5933,.T.);
#11055=EDGE_CURVE('',#8479,#8255,#5934,.T.);
#11056=EDGE_CURVE('',#8525,#8254,#5154,.T.);
#11057=EDGE_CURVE('',#8480,#8525,#5155,.T.);
#11058=EDGE_CURVE('',#8375,#8367,#4240,.T.);
#11059=EDGE_CURVE('',#8484,#8526,#5156,.T.);
#11060=EDGE_CURVE('',#8483,#8251,#5935,.T.);
#11061=EDGE_CURVE('',#8526,#8250,#5157,.T.);
#11062=EDGE_CURVE('',#8482,#8252,#5936,.T.);
#11063=EDGE_CURVE('',#8527,#8481,#5158,.T.);
#11064=EDGE_CURVE('',#8253,#8527,#5159,.T.);
#11065=EDGE_CURVE('',#8528,#8526,#4241,.T.);
#11066=EDGE_CURVE('',#8528,#8485,#5160,.T.);
#11067=EDGE_CURVE('',#8249,#8528,#5161,.T.);
#11068=EDGE_CURVE('',#8486,#8248,#5937,.T.);
#11069=EDGE_CURVE('',#8487,#8247,#5938,.T.);
#11070=EDGE_CURVE('',#8529,#8246,#5162,.T.);
#11071=EDGE_CURVE('',#8488,#8529,#5163,.T.);
#11072=EDGE_CURVE('',#8527,#8525,#4242,.T.);
#11073=EDGE_CURVE('',#8492,#8530,#5164,.T.);
#11074=EDGE_CURVE('',#8491,#8243,#5939,.T.);
#11075=EDGE_CURVE('',#8530,#8242,#5165,.T.);
#11076=EDGE_CURVE('',#8490,#8244,#5940,.T.);
#11077=EDGE_CURVE('',#8531,#8489,#5166,.T.);
#11078=EDGE_CURVE('',#8245,#8531,#5167,.T.);
#11079=EDGE_CURVE('',#8532,#8530,#4243,.T.);
#11080=EDGE_CURVE('',#8532,#8493,#5168,.T.);
#11081=EDGE_CURVE('',#8241,#8532,#5169,.T.);
#11082=EDGE_CURVE('',#8494,#8240,#5941,.T.);
#11083=EDGE_CURVE('',#8495,#8239,#5942,.T.);
#11084=EDGE_CURVE('',#8533,#8238,#5170,.T.);
#11085=EDGE_CURVE('',#8496,#8533,#5171,.T.);
#11086=EDGE_CURVE('',#8531,#8529,#4244,.T.);
#11087=EDGE_CURVE('',#8500,#8534,#5172,.T.);
#11088=EDGE_CURVE('',#8499,#8235,#5943,.T.);
#11089=EDGE_CURVE('',#8534,#8234,#5173,.T.);
#11090=EDGE_CURVE('',#8498,#8236,#5944,.T.);
#11091=EDGE_CURVE('',#8535,#8497,#5174,.T.);
#11092=EDGE_CURVE('',#8237,#8535,#5175,.T.);
#11093=EDGE_CURVE('',#8536,#8534,#4245,.T.);
#11094=EDGE_CURVE('',#8536,#8501,#5176,.T.);
#11095=EDGE_CURVE('',#8233,#8536,#5177,.T.);
#11096=EDGE_CURVE('',#8502,#8232,#5945,.T.);
#11097=EDGE_CURVE('',#8503,#8231,#5946,.T.);
#11098=EDGE_CURVE('',#8537,#8230,#5178,.T.);
#11099=EDGE_CURVE('',#8504,#8537,#5179,.T.);
#11100=EDGE_CURVE('',#8535,#8533,#4246,.T.);
#11101=EDGE_CURVE('',#8508,#8538,#5180,.T.);
#11102=EDGE_CURVE('',#8507,#8227,#5947,.T.);
#11103=EDGE_CURVE('',#8538,#8226,#5181,.T.);
#11104=EDGE_CURVE('',#8506,#8228,#5948,.T.);
#11105=EDGE_CURVE('',#8539,#8505,#5182,.T.);
#11106=EDGE_CURVE('',#8229,#8539,#5183,.T.);
#11107=EDGE_CURVE('',#8540,#8538,#4247,.T.);
#11108=EDGE_CURVE('',#8540,#8509,#5184,.T.);
#11109=EDGE_CURVE('',#8225,#8540,#5185,.T.);
#11110=EDGE_CURVE('',#8510,#8224,#5949,.T.);
#11111=EDGE_CURVE('',#8511,#8223,#5950,.T.);
#11112=EDGE_CURVE('',#8541,#8222,#5186,.T.);
#11113=EDGE_CURVE('',#8512,#8541,#5187,.T.);
#11114=EDGE_CURVE('',#8539,#8537,#4248,.T.);
#11115=EDGE_CURVE('',#8516,#8542,#5188,.T.);
#11116=EDGE_CURVE('',#8515,#8219,#5951,.T.);
#11117=EDGE_CURVE('',#8542,#8218,#5189,.T.);
#11118=EDGE_CURVE('',#8514,#8220,#5952,.T.);
#11119=EDGE_CURVE('',#8543,#8513,#5190,.T.);
#11120=EDGE_CURVE('',#8221,#8543,#5191,.T.);
#11121=EDGE_CURVE('',#8544,#8542,#4249,.T.);
#11122=EDGE_CURVE('',#8544,#8517,#5192,.T.);
#11123=EDGE_CURVE('',#8217,#8544,#5193,.T.);
#11124=EDGE_CURVE('',#8518,#8216,#5953,.T.);
#11125=EDGE_CURVE('',#8519,#8215,#5954,.T.);
#11126=EDGE_CURVE('',#8545,#8214,#5194,.T.);
#11127=EDGE_CURVE('',#8520,#8545,#5195,.T.);
#11128=EDGE_CURVE('',#8543,#8541,#4250,.T.);
#11129=EDGE_CURVE('',#8213,#8546,#5196,.T.);
#11130=EDGE_CURVE('',#8522,#8212,#5955,.T.);
#11131=EDGE_CURVE('',#8546,#8521,#5197,.T.);
#11132=EDGE_CURVE('',#8523,#8211,#5956,.T.);
#11133=EDGE_CURVE('',#8266,#8547,#5198,.T.);
#11134=EDGE_CURVE('',#8265,#8476,#5957,.T.);
#11135=EDGE_CURVE('',#8548,#8475,#5199,.T.);
#11136=EDGE_CURVE('',#8547,#8548,#5200,.T.);
#11137=EDGE_CURVE('',#8264,#8377,#5958,.T.);
#11138=EDGE_CURVE('',#8549,#8263,#5201,.T.);
#11139=EDGE_CURVE('',#8550,#8549,#5202,.T.);
#11140=EDGE_CURVE('',#8378,#8550,#5203,.T.);
#11141=EDGE_CURVE('',#8551,#8547,#4251,.T.);
#11142=EDGE_CURVE('',#8551,#8267,#5204,.T.);
#11143=EDGE_CURVE('',#8552,#8548,#4252,.T.);
#11144=EDGE_CURVE('',#8552,#8551,#5205,.T.);
#11145=EDGE_CURVE('',#8474,#8552,#5206,.T.);
#11146=EDGE_CURVE('',#8270,#8553,#5207,.T.);
#11147=EDGE_CURVE('',#8269,#8472,#5959,.T.);
#11148=EDGE_CURVE('',#8554,#8471,#5208,.T.);
#11149=EDGE_CURVE('',#8553,#8554,#5209,.T.);
#11150=EDGE_CURVE('',#8268,#8473,#5960,.T.);
#11151=EDGE_CURVE('',#8555,#8553,#4253,.T.);
#11152=EDGE_CURVE('',#8555,#8271,#5210,.T.);
#11153=EDGE_CURVE('',#8556,#8554,#4254,.T.);
#11154=EDGE_CURVE('',#8556,#8555,#5211,.T.);
#11155=EDGE_CURVE('',#8470,#8556,#5212,.T.);
#11156=EDGE_CURVE('',#8274,#8557,#5213,.T.);
#11157=EDGE_CURVE('',#8273,#8468,#5961,.T.);
#11158=EDGE_CURVE('',#8558,#8467,#5214,.T.);
#11159=EDGE_CURVE('',#8557,#8558,#5215,.T.);
#11160=EDGE_CURVE('',#8272,#8469,#5962,.T.);
#11161=EDGE_CURVE('',#8559,#8557,#4255,.T.);
#11162=EDGE_CURVE('',#8559,#8275,#5216,.T.);
#11163=EDGE_CURVE('',#8560,#8558,#4256,.T.);
#11164=EDGE_CURVE('',#8560,#8559,#5217,.T.);
#11165=EDGE_CURVE('',#8466,#8560,#5218,.T.);
#11166=EDGE_CURVE('',#8278,#8561,#5219,.T.);
#11167=EDGE_CURVE('',#8277,#8464,#5963,.T.);
#11168=EDGE_CURVE('',#8562,#8463,#5220,.T.);
#11169=EDGE_CURVE('',#8561,#8562,#5221,.T.);
#11170=EDGE_CURVE('',#8276,#8465,#5964,.T.);
#11171=EDGE_CURVE('',#8563,#8561,#4257,.T.);
#11172=EDGE_CURVE('',#8563,#8279,#5222,.T.);
#11173=EDGE_CURVE('',#8564,#8562,#4258,.T.);
#11174=EDGE_CURVE('',#8564,#8563,#5223,.T.);
#11175=EDGE_CURVE('',#8462,#8564,#5224,.T.);
#11176=EDGE_CURVE('',#8282,#8565,#5225,.T.);
#11177=EDGE_CURVE('',#8281,#8460,#5965,.T.);
#11178=EDGE_CURVE('',#8566,#8459,#5226,.T.);
#11179=EDGE_CURVE('',#8565,#8566,#5227,.T.);
#11180=EDGE_CURVE('',#8280,#8461,#5966,.T.);
#11181=EDGE_CURVE('',#8567,#8565,#4259,.T.);
#11182=EDGE_CURVE('',#8567,#8283,#5228,.T.);
#11183=EDGE_CURVE('',#8568,#8566,#4260,.T.);
#11184=EDGE_CURVE('',#8568,#8567,#5229,.T.);
#11185=EDGE_CURVE('',#8458,#8568,#5230,.T.);
#11186=EDGE_CURVE('',#8286,#8569,#5231,.T.);
#11187=EDGE_CURVE('',#8285,#8456,#5967,.T.);
#11188=EDGE_CURVE('',#8570,#8455,#5232,.T.);
#11189=EDGE_CURVE('',#8569,#8570,#5233,.T.);
#11190=EDGE_CURVE('',#8284,#8457,#5968,.T.);
#11191=EDGE_CURVE('',#8571,#8569,#4261,.T.);
#11192=EDGE_CURVE('',#8571,#8287,#5234,.T.);
#11193=EDGE_CURVE('',#8572,#8570,#4262,.T.);
#11194=EDGE_CURVE('',#8572,#8571,#5235,.T.);
#11195=EDGE_CURVE('',#8454,#8572,#5236,.T.);
#11196=EDGE_CURVE('',#8290,#8573,#5237,.T.);
#11197=EDGE_CURVE('',#8289,#8452,#5969,.T.);
#11198=EDGE_CURVE('',#8574,#8451,#5238,.T.);
#11199=EDGE_CURVE('',#8573,#8574,#5239,.T.);
#11200=EDGE_CURVE('',#8288,#8453,#5970,.T.);
#11201=EDGE_CURVE('',#8575,#8573,#4263,.T.);
#11202=EDGE_CURVE('',#8575,#8291,#5240,.T.);
#11203=EDGE_CURVE('',#8576,#8574,#4264,.T.);
#11204=EDGE_CURVE('',#8576,#8575,#5241,.T.);
#11205=EDGE_CURVE('',#8450,#8576,#5242,.T.);
#11206=EDGE_CURVE('',#8294,#8577,#5243,.T.);
#11207=EDGE_CURVE('',#8293,#8448,#5971,.T.);
#11208=EDGE_CURVE('',#8578,#8447,#5244,.T.);
#11209=EDGE_CURVE('',#8577,#8578,#5245,.T.);
#11210=EDGE_CURVE('',#8292,#8449,#5972,.T.);
#11211=EDGE_CURVE('',#8579,#8577,#4265,.T.);
#11212=EDGE_CURVE('',#8579,#8295,#5246,.T.);
#11213=EDGE_CURVE('',#8580,#8578,#4266,.T.);
#11214=EDGE_CURVE('',#8580,#8579,#5247,.T.);
#11215=EDGE_CURVE('',#8446,#8580,#5248,.T.);
#11216=EDGE_CURVE('',#8298,#8581,#5249,.T.);
#11217=EDGE_CURVE('',#8297,#8444,#5973,.T.);
#11218=EDGE_CURVE('',#8582,#8443,#5250,.T.);
#11219=EDGE_CURVE('',#8581,#8582,#5251,.T.);
#11220=EDGE_CURVE('',#8296,#8445,#5974,.T.);
#11221=EDGE_CURVE('',#8583,#8581,#4267,.T.);
#11222=EDGE_CURVE('',#8583,#8299,#5252,.T.);
#11223=EDGE_CURVE('',#8584,#8582,#4268,.T.);
#11224=EDGE_CURVE('',#8584,#8583,#5253,.T.);
#11225=EDGE_CURVE('',#8442,#8584,#5254,.T.);
#11226=EDGE_CURVE('',#8302,#8585,#5255,.T.);
#11227=EDGE_CURVE('',#8301,#8440,#5975,.T.);
#11228=EDGE_CURVE('',#8586,#8439,#5256,.T.);
#11229=EDGE_CURVE('',#8585,#8586,#5257,.T.);
#11230=EDGE_CURVE('',#8300,#8441,#5976,.T.);
#11231=EDGE_CURVE('',#8587,#8585,#4269,.T.);
#11232=EDGE_CURVE('',#8587,#8303,#5258,.T.);
#11233=EDGE_CURVE('',#8588,#8586,#4270,.T.);
#11234=EDGE_CURVE('',#8588,#8587,#5259,.T.);
#11235=EDGE_CURVE('',#8438,#8588,#5260,.T.);
#11236=EDGE_CURVE('',#8306,#8589,#5261,.T.);
#11237=EDGE_CURVE('',#8305,#8436,#5977,.T.);
#11238=EDGE_CURVE('',#8590,#8435,#5262,.T.);
#11239=EDGE_CURVE('',#8589,#8590,#5263,.T.);
#11240=EDGE_CURVE('',#8304,#8437,#5978,.T.);
#11241=EDGE_CURVE('',#8591,#8589,#4271,.T.);
#11242=EDGE_CURVE('',#8591,#8307,#5264,.T.);
#11243=EDGE_CURVE('',#8592,#8590,#4272,.T.);
#11244=EDGE_CURVE('',#8592,#8591,#5265,.T.);
#11245=EDGE_CURVE('',#8434,#8592,#5266,.T.);
#11246=EDGE_CURVE('',#8310,#8593,#5267,.T.);
#11247=EDGE_CURVE('',#8309,#8432,#5979,.T.);
#11248=EDGE_CURVE('',#8594,#8431,#5268,.T.);
#11249=EDGE_CURVE('',#8593,#8594,#5269,.T.);
#11250=EDGE_CURVE('',#8308,#8433,#5980,.T.);
#11251=EDGE_CURVE('',#8595,#8593,#4273,.T.);
#11252=EDGE_CURVE('',#8595,#8311,#5270,.T.);
#11253=EDGE_CURVE('',#8596,#8594,#4274,.T.);
#11254=EDGE_CURVE('',#8596,#8595,#5271,.T.);
#11255=EDGE_CURVE('',#8430,#8596,#5272,.T.);
#11256=EDGE_CURVE('',#8314,#8597,#5273,.T.);
#11257=EDGE_CURVE('',#8313,#8428,#5981,.T.);
#11258=EDGE_CURVE('',#8598,#8427,#5274,.T.);
#11259=EDGE_CURVE('',#8597,#8598,#5275,.T.);
#11260=EDGE_CURVE('',#8312,#8429,#5982,.T.);
#11261=EDGE_CURVE('',#8599,#8597,#4275,.T.);
#11262=EDGE_CURVE('',#8599,#8315,#5276,.T.);
#11263=EDGE_CURVE('',#8600,#8598,#4276,.T.);
#11264=EDGE_CURVE('',#8600,#8599,#5277,.T.);
#11265=EDGE_CURVE('',#8426,#8600,#5278,.T.);
#11266=EDGE_CURVE('',#8318,#8601,#5279,.T.);
#11267=EDGE_CURVE('',#8317,#8424,#5983,.T.);
#11268=EDGE_CURVE('',#8602,#8423,#5280,.T.);
#11269=EDGE_CURVE('',#8601,#8602,#5281,.T.);
#11270=EDGE_CURVE('',#8316,#8425,#5984,.T.);
#11271=EDGE_CURVE('',#8603,#8601,#4277,.T.);
#11272=EDGE_CURVE('',#8603,#8319,#5282,.T.);
#11273=EDGE_CURVE('',#8604,#8602,#4278,.T.);
#11274=EDGE_CURVE('',#8604,#8603,#5283,.T.);
#11275=EDGE_CURVE('',#8422,#8604,#5284,.T.);
#11276=EDGE_CURVE('',#8322,#8605,#5285,.T.);
#11277=EDGE_CURVE('',#8321,#8420,#5985,.T.);
#11278=EDGE_CURVE('',#8606,#8419,#5286,.T.);
#11279=EDGE_CURVE('',#8605,#8606,#5287,.T.);
#11280=EDGE_CURVE('',#8320,#8421,#5986,.T.);
#11281=EDGE_CURVE('',#8607,#8605,#4279,.T.);
#11282=EDGE_CURVE('',#8607,#8323,#5288,.T.);
#11283=EDGE_CURVE('',#8608,#8606,#4280,.T.);
#11284=EDGE_CURVE('',#8608,#8607,#5289,.T.);
#11285=EDGE_CURVE('',#8418,#8608,#5290,.T.);
#11286=EDGE_CURVE('',#8326,#8609,#5291,.T.);
#11287=EDGE_CURVE('',#8325,#8416,#5987,.T.);
#11288=EDGE_CURVE('',#8610,#8415,#5292,.T.);
#11289=EDGE_CURVE('',#8609,#8610,#5293,.T.);
#11290=EDGE_CURVE('',#8324,#8417,#5988,.T.);
#11291=EDGE_CURVE('',#8611,#8609,#4281,.T.);
#11292=EDGE_CURVE('',#8611,#8327,#5294,.T.);
#11293=EDGE_CURVE('',#8612,#8610,#4282,.T.);
#11294=EDGE_CURVE('',#8612,#8611,#5295,.T.);
#11295=EDGE_CURVE('',#8414,#8612,#5296,.T.);
#11296=EDGE_CURVE('',#8330,#8613,#5297,.T.);
#11297=EDGE_CURVE('',#8329,#8412,#5989,.T.);
#11298=EDGE_CURVE('',#8614,#8411,#5298,.T.);
#11299=EDGE_CURVE('',#8613,#8614,#5299,.T.);
#11300=EDGE_CURVE('',#8328,#8413,#5990,.T.);
#11301=EDGE_CURVE('',#8615,#8613,#4283,.T.);
#11302=EDGE_CURVE('',#8615,#8331,#5300,.T.);
#11303=EDGE_CURVE('',#8616,#8614,#4284,.T.);
#11304=EDGE_CURVE('',#8616,#8615,#5301,.T.);
#11305=EDGE_CURVE('',#8410,#8616,#5302,.T.);
#11306=EDGE_CURVE('',#8334,#8617,#5303,.T.);
#11307=EDGE_CURVE('',#8333,#8408,#5991,.T.);
#11308=EDGE_CURVE('',#8618,#8407,#5304,.T.);
#11309=EDGE_CURVE('',#8617,#8618,#5305,.T.);
#11310=EDGE_CURVE('',#8332,#8409,#5992,.T.);
#11311=EDGE_CURVE('',#8619,#8617,#4285,.T.);
#11312=EDGE_CURVE('',#8619,#8335,#5306,.T.);
#11313=EDGE_CURVE('',#8620,#8618,#4286,.T.);
#11314=EDGE_CURVE('',#8620,#8619,#5307,.T.);
#11315=EDGE_CURVE('',#8406,#8620,#5308,.T.);
#11316=EDGE_CURVE('',#8338,#8621,#5309,.T.);
#11317=EDGE_CURVE('',#8337,#8404,#5993,.T.);
#11318=EDGE_CURVE('',#8622,#8403,#5310,.T.);
#11319=EDGE_CURVE('',#8621,#8622,#5311,.T.);
#11320=EDGE_CURVE('',#8336,#8405,#5994,.T.);
#11321=EDGE_CURVE('',#8623,#8621,#4287,.T.);
#11322=EDGE_CURVE('',#8623,#8339,#5312,.T.);
#11323=EDGE_CURVE('',#8624,#8622,#4288,.T.);
#11324=EDGE_CURVE('',#8624,#8623,#5313,.T.);
#11325=EDGE_CURVE('',#8402,#8624,#5314,.T.);
#11326=EDGE_CURVE('',#8342,#8625,#5315,.T.);
#11327=EDGE_CURVE('',#8341,#8400,#5995,.T.);
#11328=EDGE_CURVE('',#8626,#8399,#5316,.T.);
#11329=EDGE_CURVE('',#8625,#8626,#5317,.T.);
#11330=EDGE_CURVE('',#8340,#8401,#5996,.T.);
#11331=EDGE_CURVE('',#8627,#8625,#4289,.T.);
#11332=EDGE_CURVE('',#8627,#8343,#5318,.T.);
#11333=EDGE_CURVE('',#8628,#8626,#4290,.T.);
#11334=EDGE_CURVE('',#8628,#8627,#5319,.T.);
#11335=EDGE_CURVE('',#8398,#8628,#5320,.T.);
#11336=EDGE_CURVE('',#8346,#8629,#5321,.T.);
#11337=EDGE_CURVE('',#8345,#8396,#5997,.T.);
#11338=EDGE_CURVE('',#8630,#8395,#5322,.T.);
#11339=EDGE_CURVE('',#8629,#8630,#5323,.T.);
#11340=EDGE_CURVE('',#8344,#8397,#5998,.T.);
#11341=EDGE_CURVE('',#8631,#8629,#4291,.T.);
#11342=EDGE_CURVE('',#8631,#8347,#5324,.T.);
#11343=EDGE_CURVE('',#8632,#8630,#4292,.T.);
#11344=EDGE_CURVE('',#8632,#8631,#5325,.T.);
#11345=EDGE_CURVE('',#8394,#8632,#5326,.T.);
#11346=EDGE_CURVE('',#8350,#8633,#5327,.T.);
#11347=EDGE_CURVE('',#8349,#8392,#5999,.T.);
#11348=EDGE_CURVE('',#8634,#8391,#5328,.T.);
#11349=EDGE_CURVE('',#8633,#8634,#5329,.T.);
#11350=EDGE_CURVE('',#8348,#8393,#6000,.T.);
#11351=EDGE_CURVE('',#8635,#8633,#4293,.T.);
#11352=EDGE_CURVE('',#8635,#8351,#5330,.T.);
#11353=EDGE_CURVE('',#8636,#8634,#4294,.T.);
#11354=EDGE_CURVE('',#8636,#8635,#5331,.T.);
#11355=EDGE_CURVE('',#8390,#8636,#5332,.T.);
#11356=EDGE_CURVE('',#8354,#8637,#5333,.T.);
#11357=EDGE_CURVE('',#8353,#8388,#6001,.T.);
#11358=EDGE_CURVE('',#8638,#8387,#5334,.T.);
#11359=EDGE_CURVE('',#8637,#8638,#5335,.T.);
#11360=EDGE_CURVE('',#8352,#8389,#6002,.T.);
#11361=EDGE_CURVE('',#8639,#8637,#4295,.T.);
#11362=EDGE_CURVE('',#8639,#8355,#5336,.T.);
#11363=EDGE_CURVE('',#8640,#8638,#4296,.T.);
#11364=EDGE_CURVE('',#8640,#8639,#5337,.T.);
#11365=EDGE_CURVE('',#8386,#8640,#5338,.T.);
#11366=EDGE_CURVE('',#8358,#8641,#5339,.T.);
#11367=EDGE_CURVE('',#8357,#8384,#6003,.T.);
#11368=EDGE_CURVE('',#8642,#8383,#5340,.T.);
#11369=EDGE_CURVE('',#8641,#8642,#5341,.T.);
#11370=EDGE_CURVE('',#8356,#8385,#6004,.T.);
#11371=EDGE_CURVE('',#8643,#8641,#4297,.T.);
#11372=EDGE_CURVE('',#8643,#8359,#5342,.T.);
#11373=EDGE_CURVE('',#8644,#8642,#4298,.T.);
#11374=EDGE_CURVE('',#8644,#8643,#5343,.T.);
#11375=EDGE_CURVE('',#8382,#8644,#5344,.T.);
#11376=EDGE_CURVE('',#8362,#8645,#5345,.T.);
#11377=EDGE_CURVE('',#8361,#8380,#6005,.T.);
#11378=EDGE_CURVE('',#8646,#8379,#5346,.T.);
#11379=EDGE_CURVE('',#8645,#8646,#5347,.T.);
#11380=EDGE_CURVE('',#8360,#8381,#6006,.T.);
#11381=EDGE_CURVE('',#8549,#8645,#4299,.T.);
#11382=EDGE_CURVE('',#8550,#8646,#4300,.T.);
#11383=EDGE_CURVE('',#8546,#8545,#4301,.T.);
#15364=ORIENTED_EDGE('',*,*,#10715,.T.);
#15365=ORIENTED_EDGE('',*,*,#10716,.T.);
#15366=ORIENTED_EDGE('',*,*,#10717,.T.);
#15367=ORIENTED_EDGE('',*,*,#10718,.T.);
#15368=ORIENTED_EDGE('',*,*,#10717,.F.);
#15369=ORIENTED_EDGE('',*,*,#10715,.F.);
#15370=ORIENTED_EDGE('',*,*,#10716,.F.);
#15371=ORIENTED_EDGE('',*,*,#10719,.T.);
#15372=ORIENTED_EDGE('',*,*,#10720,.F.);
#15373=ORIENTED_EDGE('',*,*,#10721,.F.);
#15374=ORIENTED_EDGE('',*,*,#10719,.F.);
#15375=ORIENTED_EDGE('',*,*,#10722,.T.);
#15376=ORIENTED_EDGE('',*,*,#10723,.T.);
#15377=ORIENTED_EDGE('',*,*,#10724,.T.);
#15378=ORIENTED_EDGE('',*,*,#10725,.T.);
#15379=ORIENTED_EDGE('',*,*,#10726,.T.);
#15380=ORIENTED_EDGE('',*,*,#10727,.T.);
#15381=ORIENTED_EDGE('',*,*,#10728,.T.);
#15382=ORIENTED_EDGE('',*,*,#10729,.T.);
#15383=ORIENTED_EDGE('',*,*,#10730,.T.);
#15384=ORIENTED_EDGE('',*,*,#10731,.T.);
#15385=ORIENTED_EDGE('',*,*,#10732,.T.);
#15386=ORIENTED_EDGE('',*,*,#10733,.T.);
#15387=ORIENTED_EDGE('',*,*,#10734,.T.);
#15388=ORIENTED_EDGE('',*,*,#10735,.T.);
#15389=ORIENTED_EDGE('',*,*,#10736,.T.);
#15390=ORIENTED_EDGE('',*,*,#10737,.T.);
#15391=ORIENTED_EDGE('',*,*,#10738,.T.);
#15392=ORIENTED_EDGE('',*,*,#10739,.T.);
#15393=ORIENTED_EDGE('',*,*,#10740,.T.);
#15394=ORIENTED_EDGE('',*,*,#10741,.T.);
#15395=ORIENTED_EDGE('',*,*,#10742,.T.);
#15396=ORIENTED_EDGE('',*,*,#10743,.T.);
#15397=ORIENTED_EDGE('',*,*,#10744,.T.);
#15398=ORIENTED_EDGE('',*,*,#10745,.T.);
#15399=ORIENTED_EDGE('',*,*,#10746,.T.);
#15400=ORIENTED_EDGE('',*,*,#10747,.T.);
#15401=ORIENTED_EDGE('',*,*,#10748,.T.);
#15402=ORIENTED_EDGE('',*,*,#10749,.T.);
#15403=ORIENTED_EDGE('',*,*,#10750,.T.);
#15404=ORIENTED_EDGE('',*,*,#10751,.T.);
#15405=ORIENTED_EDGE('',*,*,#10752,.T.);
#15406=ORIENTED_EDGE('',*,*,#10753,.T.);
#15407=ORIENTED_EDGE('',*,*,#10754,.T.);
#15408=ORIENTED_EDGE('',*,*,#10755,.T.);
#15409=ORIENTED_EDGE('',*,*,#10756,.T.);
#15410=ORIENTED_EDGE('',*,*,#10757,.T.);
#15411=ORIENTED_EDGE('',*,*,#10758,.T.);
#15412=ORIENTED_EDGE('',*,*,#10759,.T.);
#15413=ORIENTED_EDGE('',*,*,#10760,.T.);
#15414=ORIENTED_EDGE('',*,*,#10761,.T.);
#15415=ORIENTED_EDGE('',*,*,#10762,.T.);
#15416=ORIENTED_EDGE('',*,*,#10763,.T.);
#15417=ORIENTED_EDGE('',*,*,#10764,.T.);
#15418=ORIENTED_EDGE('',*,*,#10765,.T.);
#15419=ORIENTED_EDGE('',*,*,#10766,.T.);
#15420=ORIENTED_EDGE('',*,*,#10767,.T.);
#15421=ORIENTED_EDGE('',*,*,#10768,.T.);
#15422=ORIENTED_EDGE('',*,*,#10769,.T.);
#15423=ORIENTED_EDGE('',*,*,#10770,.T.);
#15424=ORIENTED_EDGE('',*,*,#10771,.T.);
#15425=ORIENTED_EDGE('',*,*,#10772,.T.);
#15426=ORIENTED_EDGE('',*,*,#10773,.T.);
#15427=ORIENTED_EDGE('',*,*,#10774,.T.);
#15428=ORIENTED_EDGE('',*,*,#10775,.T.);
#15429=ORIENTED_EDGE('',*,*,#10776,.T.);
#15430=ORIENTED_EDGE('',*,*,#10777,.T.);
#15431=ORIENTED_EDGE('',*,*,#10718,.F.);
#15432=ORIENTED_EDGE('',*,*,#10778,.T.);
#15433=ORIENTED_EDGE('',*,*,#10779,.T.);
#15434=ORIENTED_EDGE('',*,*,#10720,.T.);
#15435=ORIENTED_EDGE('',*,*,#10721,.T.);
#15436=ORIENTED_EDGE('',*,*,#10779,.F.);
#15437=ORIENTED_EDGE('',*,*,#10780,.T.);
#15438=ORIENTED_EDGE('',*,*,#10781,.T.);
#15439=ORIENTED_EDGE('',*,*,#10782,.T.);
#15440=ORIENTED_EDGE('',*,*,#10783,.F.);
#15441=ORIENTED_EDGE('',*,*,#10784,.T.);
#15442=ORIENTED_EDGE('',*,*,#10785,.T.);
#15443=ORIENTED_EDGE('',*,*,#10786,.T.);
#15444=ORIENTED_EDGE('',*,*,#10787,.F.);
#15445=ORIENTED_EDGE('',*,*,#10788,.T.);
#15446=ORIENTED_EDGE('',*,*,#10789,.T.);
#15447=ORIENTED_EDGE('',*,*,#10790,.T.);
#15448=ORIENTED_EDGE('',*,*,#10791,.F.);
#15449=ORIENTED_EDGE('',*,*,#10792,.T.);
#15450=ORIENTED_EDGE('',*,*,#10793,.T.);
#15451=ORIENTED_EDGE('',*,*,#10794,.T.);
#15452=ORIENTED_EDGE('',*,*,#10795,.F.);
#15453=ORIENTED_EDGE('',*,*,#10796,.T.);
#15454=ORIENTED_EDGE('',*,*,#10797,.T.);
#15455=ORIENTED_EDGE('',*,*,#10798,.T.);
#15456=ORIENTED_EDGE('',*,*,#10799,.F.);
#15457=ORIENTED_EDGE('',*,*,#10800,.T.);
#15458=ORIENTED_EDGE('',*,*,#10801,.T.);
#15459=ORIENTED_EDGE('',*,*,#10802,.T.);
#15460=ORIENTED_EDGE('',*,*,#10803,.F.);
#15461=ORIENTED_EDGE('',*,*,#10804,.T.);
#15462=ORIENTED_EDGE('',*,*,#10805,.T.);
#15463=ORIENTED_EDGE('',*,*,#10806,.T.);
#15464=ORIENTED_EDGE('',*,*,#10807,.F.);
#15465=ORIENTED_EDGE('',*,*,#10808,.T.);
#15466=ORIENTED_EDGE('',*,*,#10809,.T.);
#15467=ORIENTED_EDGE('',*,*,#10810,.T.);
#15468=ORIENTED_EDGE('',*,*,#10811,.F.);
#15469=ORIENTED_EDGE('',*,*,#10812,.T.);
#15470=ORIENTED_EDGE('',*,*,#10813,.T.);
#15471=ORIENTED_EDGE('',*,*,#10814,.T.);
#15472=ORIENTED_EDGE('',*,*,#10815,.F.);
#15473=ORIENTED_EDGE('',*,*,#10816,.T.);
#15474=ORIENTED_EDGE('',*,*,#10817,.T.);
#15475=ORIENTED_EDGE('',*,*,#10818,.T.);
#15476=ORIENTED_EDGE('',*,*,#10819,.F.);
#15477=ORIENTED_EDGE('',*,*,#10820,.T.);
#15478=ORIENTED_EDGE('',*,*,#10821,.T.);
#15479=ORIENTED_EDGE('',*,*,#10822,.T.);
#15480=ORIENTED_EDGE('',*,*,#10823,.F.);
#15481=ORIENTED_EDGE('',*,*,#10824,.T.);
#15482=ORIENTED_EDGE('',*,*,#10825,.T.);
#15483=ORIENTED_EDGE('',*,*,#10826,.T.);
#15484=ORIENTED_EDGE('',*,*,#10827,.F.);
#15485=ORIENTED_EDGE('',*,*,#10828,.T.);
#15486=ORIENTED_EDGE('',*,*,#10829,.T.);
#15487=ORIENTED_EDGE('',*,*,#10830,.T.);
#15488=ORIENTED_EDGE('',*,*,#10831,.F.);
#15489=ORIENTED_EDGE('',*,*,#10832,.T.);
#15490=ORIENTED_EDGE('',*,*,#10833,.T.);
#15491=ORIENTED_EDGE('',*,*,#10834,.T.);
#15492=ORIENTED_EDGE('',*,*,#10835,.F.);
#15493=ORIENTED_EDGE('',*,*,#10836,.T.);
#15494=ORIENTED_EDGE('',*,*,#10837,.T.);
#15495=ORIENTED_EDGE('',*,*,#10838,.T.);
#15496=ORIENTED_EDGE('',*,*,#10839,.F.);
#15497=ORIENTED_EDGE('',*,*,#10840,.T.);
#15498=ORIENTED_EDGE('',*,*,#10841,.T.);
#15499=ORIENTED_EDGE('',*,*,#10842,.T.);
#15500=ORIENTED_EDGE('',*,*,#10843,.F.);
#15501=ORIENTED_EDGE('',*,*,#10844,.T.);
#15502=ORIENTED_EDGE('',*,*,#10845,.T.);
#15503=ORIENTED_EDGE('',*,*,#10846,.T.);
#15504=ORIENTED_EDGE('',*,*,#10847,.F.);
#15505=ORIENTED_EDGE('',*,*,#10848,.T.);
#15506=ORIENTED_EDGE('',*,*,#10849,.T.);
#15507=ORIENTED_EDGE('',*,*,#10850,.T.);
#15508=ORIENTED_EDGE('',*,*,#10851,.F.);
#15509=ORIENTED_EDGE('',*,*,#10852,.T.);
#15510=ORIENTED_EDGE('',*,*,#10853,.T.);
#15511=ORIENTED_EDGE('',*,*,#10854,.T.);
#15512=ORIENTED_EDGE('',*,*,#10855,.F.);
#15513=ORIENTED_EDGE('',*,*,#10856,.T.);
#15514=ORIENTED_EDGE('',*,*,#10857,.T.);
#15515=ORIENTED_EDGE('',*,*,#10858,.T.);
#15516=ORIENTED_EDGE('',*,*,#10859,.F.);
#15517=ORIENTED_EDGE('',*,*,#10860,.T.);
#15518=ORIENTED_EDGE('',*,*,#10861,.T.);
#15519=ORIENTED_EDGE('',*,*,#10862,.T.);
#15520=ORIENTED_EDGE('',*,*,#10863,.F.);
#15521=ORIENTED_EDGE('',*,*,#10864,.T.);
#15522=ORIENTED_EDGE('',*,*,#10865,.T.);
#15523=ORIENTED_EDGE('',*,*,#10866,.T.);
#15524=ORIENTED_EDGE('',*,*,#10867,.F.);
#15525=ORIENTED_EDGE('',*,*,#10868,.T.);
#15526=ORIENTED_EDGE('',*,*,#10869,.T.);
#15527=ORIENTED_EDGE('',*,*,#10870,.T.);
#15528=ORIENTED_EDGE('',*,*,#10871,.F.);
#15529=ORIENTED_EDGE('',*,*,#10872,.T.);
#15530=ORIENTED_EDGE('',*,*,#10873,.T.);
#15531=ORIENTED_EDGE('',*,*,#10874,.T.);
#15532=ORIENTED_EDGE('',*,*,#10875,.F.);
#15533=ORIENTED_EDGE('',*,*,#10876,.T.);
#15534=ORIENTED_EDGE('',*,*,#10877,.T.);
#15535=ORIENTED_EDGE('',*,*,#10878,.T.);
#15536=ORIENTED_EDGE('',*,*,#10879,.F.);
#15537=ORIENTED_EDGE('',*,*,#10778,.F.);
#15538=ORIENTED_EDGE('',*,*,#10880,.F.);
#15539=ORIENTED_EDGE('',*,*,#10724,.F.);
#15540=ORIENTED_EDGE('',*,*,#10881,.F.);
#15541=ORIENTED_EDGE('',*,*,#10882,.T.);
#15542=ORIENTED_EDGE('',*,*,#10883,.F.);
#15543=ORIENTED_EDGE('',*,*,#10884,.T.);
#15544=ORIENTED_EDGE('',*,*,#10881,.T.);
#15545=ORIENTED_EDGE('',*,*,#10723,.F.);
#15546=ORIENTED_EDGE('',*,*,#10885,.F.);
#15547=ORIENTED_EDGE('',*,*,#10886,.F.);
#15548=ORIENTED_EDGE('',*,*,#10887,.F.);
#15549=ORIENTED_EDGE('',*,*,#10888,.T.);
#15550=ORIENTED_EDGE('',*,*,#10885,.T.);
#15551=ORIENTED_EDGE('',*,*,#10722,.F.);
#15552=ORIENTED_EDGE('',*,*,#10880,.T.);
#15553=ORIENTED_EDGE('',*,*,#10889,.T.);
#15554=ORIENTED_EDGE('',*,*,#10890,.T.);
#15555=ORIENTED_EDGE('',*,*,#10725,.F.);
#15556=ORIENTED_EDGE('',*,*,#10883,.T.);
#15557=ORIENTED_EDGE('',*,*,#10891,.T.);
#15558=ORIENTED_EDGE('',*,*,#10892,.T.);
#15559=ORIENTED_EDGE('',*,*,#10889,.F.);
#15560=ORIENTED_EDGE('',*,*,#10893,.F.);
#15561=ORIENTED_EDGE('',*,*,#10894,.T.);
#15562=ORIENTED_EDGE('',*,*,#10895,.T.);
#15563=ORIENTED_EDGE('',*,*,#10774,.F.);
#15564=ORIENTED_EDGE('',*,*,#10896,.F.);
#15565=ORIENTED_EDGE('',*,*,#10897,.T.);
#15566=ORIENTED_EDGE('',*,*,#10898,.T.);
#15567=ORIENTED_EDGE('',*,*,#10775,.F.);
#15568=ORIENTED_EDGE('',*,*,#10895,.F.);
#15569=ORIENTED_EDGE('',*,*,#10899,.F.);
#15570=ORIENTED_EDGE('',*,*,#10900,.F.);
#15571=ORIENTED_EDGE('',*,*,#10776,.F.);
#15572=ORIENTED_EDGE('',*,*,#10898,.F.);
#15573=ORIENTED_EDGE('',*,*,#10901,.T.);
#15574=ORIENTED_EDGE('',*,*,#10902,.T.);
#15575=ORIENTED_EDGE('',*,*,#10903,.T.);
#15576=ORIENTED_EDGE('',*,*,#10904,.T.);
#15577=ORIENTED_EDGE('',*,*,#10905,.T.);
#15578=ORIENTED_EDGE('',*,*,#10906,.T.);
#15579=ORIENTED_EDGE('',*,*,#10907,.T.);
#15580=ORIENTED_EDGE('',*,*,#10908,.T.);
#15581=ORIENTED_EDGE('',*,*,#10909,.T.);
#15582=ORIENTED_EDGE('',*,*,#10910,.T.);
#15583=ORIENTED_EDGE('',*,*,#10911,.T.);
#15584=ORIENTED_EDGE('',*,*,#10912,.T.);
#15585=ORIENTED_EDGE('',*,*,#10913,.T.);
#15586=ORIENTED_EDGE('',*,*,#10914,.T.);
#15587=ORIENTED_EDGE('',*,*,#10915,.T.);
#15588=ORIENTED_EDGE('',*,*,#10916,.T.);
#15589=ORIENTED_EDGE('',*,*,#10917,.T.);
#15590=ORIENTED_EDGE('',*,*,#10918,.T.);
#15591=ORIENTED_EDGE('',*,*,#10919,.T.);
#15592=ORIENTED_EDGE('',*,*,#10920,.T.);
#15593=ORIENTED_EDGE('',*,*,#10921,.T.);
#15594=ORIENTED_EDGE('',*,*,#10922,.T.);
#15595=ORIENTED_EDGE('',*,*,#10923,.T.);
#15596=ORIENTED_EDGE('',*,*,#10924,.T.);
#15597=ORIENTED_EDGE('',*,*,#10925,.T.);
#15598=ORIENTED_EDGE('',*,*,#10926,.T.);
#15599=ORIENTED_EDGE('',*,*,#10927,.T.);
#15600=ORIENTED_EDGE('',*,*,#10928,.T.);
#15601=ORIENTED_EDGE('',*,*,#10929,.T.);
#15602=ORIENTED_EDGE('',*,*,#10930,.T.);
#15603=ORIENTED_EDGE('',*,*,#10931,.T.);
#15604=ORIENTED_EDGE('',*,*,#10932,.T.);
#15605=ORIENTED_EDGE('',*,*,#10933,.T.);
#15606=ORIENTED_EDGE('',*,*,#10934,.T.);
#15607=ORIENTED_EDGE('',*,*,#10935,.T.);
#15608=ORIENTED_EDGE('',*,*,#10936,.T.);
#15609=ORIENTED_EDGE('',*,*,#10937,.T.);
#15610=ORIENTED_EDGE('',*,*,#10938,.T.);
#15611=ORIENTED_EDGE('',*,*,#10939,.T.);
#15612=ORIENTED_EDGE('',*,*,#10940,.T.);
#15613=ORIENTED_EDGE('',*,*,#10941,.T.);
#15614=ORIENTED_EDGE('',*,*,#10942,.T.);
#15615=ORIENTED_EDGE('',*,*,#10943,.T.);
#15616=ORIENTED_EDGE('',*,*,#10944,.T.);
#15617=ORIENTED_EDGE('',*,*,#10945,.T.);
#15618=ORIENTED_EDGE('',*,*,#10946,.T.);
#15619=ORIENTED_EDGE('',*,*,#10947,.T.);
#15620=ORIENTED_EDGE('',*,*,#10948,.T.);
#15621=ORIENTED_EDGE('',*,*,#10949,.T.);
#15622=ORIENTED_EDGE('',*,*,#10950,.T.);
#15623=ORIENTED_EDGE('',*,*,#10951,.T.);
#15624=ORIENTED_EDGE('',*,*,#10952,.T.);
#15625=ORIENTED_EDGE('',*,*,#10953,.T.);
#15626=ORIENTED_EDGE('',*,*,#10954,.T.);
#15627=ORIENTED_EDGE('',*,*,#10955,.T.);
#15628=ORIENTED_EDGE('',*,*,#10956,.T.);
#15629=ORIENTED_EDGE('',*,*,#10957,.T.);
#15630=ORIENTED_EDGE('',*,*,#10958,.T.);
#15631=ORIENTED_EDGE('',*,*,#10959,.T.);
#15632=ORIENTED_EDGE('',*,*,#10960,.T.);
#15633=ORIENTED_EDGE('',*,*,#10961,.T.);
#15634=ORIENTED_EDGE('',*,*,#10962,.T.);
#15635=ORIENTED_EDGE('',*,*,#10963,.T.);
#15636=ORIENTED_EDGE('',*,*,#10964,.T.);
#15637=ORIENTED_EDGE('',*,*,#10965,.T.);
#15638=ORIENTED_EDGE('',*,*,#10966,.T.);
#15639=ORIENTED_EDGE('',*,*,#10967,.T.);
#15640=ORIENTED_EDGE('',*,*,#10968,.T.);
#15641=ORIENTED_EDGE('',*,*,#10969,.T.);
#15642=ORIENTED_EDGE('',*,*,#10970,.T.);
#15643=ORIENTED_EDGE('',*,*,#10971,.T.);
#15644=ORIENTED_EDGE('',*,*,#10972,.T.);
#15645=ORIENTED_EDGE('',*,*,#10973,.T.);
#15646=ORIENTED_EDGE('',*,*,#10974,.T.);
#15647=ORIENTED_EDGE('',*,*,#10975,.T.);
#15648=ORIENTED_EDGE('',*,*,#10976,.T.);
#15649=ORIENTED_EDGE('',*,*,#10977,.T.);
#15650=ORIENTED_EDGE('',*,*,#10978,.T.);
#15651=ORIENTED_EDGE('',*,*,#10979,.T.);
#15652=ORIENTED_EDGE('',*,*,#10980,.T.);
#15653=ORIENTED_EDGE('',*,*,#10981,.T.);
#15654=ORIENTED_EDGE('',*,*,#10982,.T.);
#15655=ORIENTED_EDGE('',*,*,#10983,.T.);
#15656=ORIENTED_EDGE('',*,*,#10984,.T.);
#15657=ORIENTED_EDGE('',*,*,#10985,.T.);
#15658=ORIENTED_EDGE('',*,*,#10986,.T.);
#15659=ORIENTED_EDGE('',*,*,#10987,.T.);
#15660=ORIENTED_EDGE('',*,*,#10988,.T.);
#15661=ORIENTED_EDGE('',*,*,#10989,.T.);
#15662=ORIENTED_EDGE('',*,*,#10990,.T.);
#15663=ORIENTED_EDGE('',*,*,#10991,.T.);
#15664=ORIENTED_EDGE('',*,*,#10992,.T.);
#15665=ORIENTED_EDGE('',*,*,#10993,.T.);
#15666=ORIENTED_EDGE('',*,*,#10994,.T.);
#15667=ORIENTED_EDGE('',*,*,#10995,.T.);
#15668=ORIENTED_EDGE('',*,*,#10996,.T.);
#15669=ORIENTED_EDGE('',*,*,#10997,.T.);
#15670=ORIENTED_EDGE('',*,*,#10998,.T.);
#15671=ORIENTED_EDGE('',*,*,#10999,.T.);
#15672=ORIENTED_EDGE('',*,*,#11000,.T.);
#15673=ORIENTED_EDGE('',*,*,#11001,.T.);
#15674=ORIENTED_EDGE('',*,*,#11002,.F.);
#15675=ORIENTED_EDGE('',*,*,#10901,.F.);
#15676=ORIENTED_EDGE('',*,*,#10897,.F.);
#15677=ORIENTED_EDGE('',*,*,#10894,.F.);
#15678=ORIENTED_EDGE('',*,*,#11003,.F.);
#15679=ORIENTED_EDGE('',*,*,#11004,.F.);
#15680=ORIENTED_EDGE('',*,*,#11005,.F.);
#15681=ORIENTED_EDGE('',*,*,#11006,.F.);
#15682=ORIENTED_EDGE('',*,*,#11007,.F.);
#15683=ORIENTED_EDGE('',*,*,#11008,.F.);
#15684=ORIENTED_EDGE('',*,*,#11009,.F.);
#15685=ORIENTED_EDGE('',*,*,#11010,.F.);
#15686=ORIENTED_EDGE('',*,*,#11011,.F.);
#15687=ORIENTED_EDGE('',*,*,#11012,.F.);
#15688=ORIENTED_EDGE('',*,*,#11013,.F.);
#15689=ORIENTED_EDGE('',*,*,#11014,.F.);
#15690=ORIENTED_EDGE('',*,*,#11015,.F.);
#15691=ORIENTED_EDGE('',*,*,#11016,.F.);
#15692=ORIENTED_EDGE('',*,*,#11017,.F.);
#15693=ORIENTED_EDGE('',*,*,#11018,.F.);
#15694=ORIENTED_EDGE('',*,*,#11019,.F.);
#15695=ORIENTED_EDGE('',*,*,#11020,.F.);
#15696=ORIENTED_EDGE('',*,*,#11021,.F.);
#15697=ORIENTED_EDGE('',*,*,#11022,.F.);
#15698=ORIENTED_EDGE('',*,*,#11023,.F.);
#15699=ORIENTED_EDGE('',*,*,#11024,.F.);
#15700=ORIENTED_EDGE('',*,*,#11025,.F.);
#15701=ORIENTED_EDGE('',*,*,#11026,.F.);
#15702=ORIENTED_EDGE('',*,*,#11027,.F.);
#15703=ORIENTED_EDGE('',*,*,#11028,.F.);
#15704=ORIENTED_EDGE('',*,*,#11029,.F.);
#15705=ORIENTED_EDGE('',*,*,#11030,.F.);
#15706=ORIENTED_EDGE('',*,*,#11031,.F.);
#15707=ORIENTED_EDGE('',*,*,#11032,.F.);
#15708=ORIENTED_EDGE('',*,*,#11033,.F.);
#15709=ORIENTED_EDGE('',*,*,#11034,.F.);
#15710=ORIENTED_EDGE('',*,*,#11035,.F.);
#15711=ORIENTED_EDGE('',*,*,#11036,.F.);
#15712=ORIENTED_EDGE('',*,*,#11037,.F.);
#15713=ORIENTED_EDGE('',*,*,#11038,.F.);
#15714=ORIENTED_EDGE('',*,*,#11039,.F.);
#15715=ORIENTED_EDGE('',*,*,#11040,.F.);
#15716=ORIENTED_EDGE('',*,*,#11041,.F.);
#15717=ORIENTED_EDGE('',*,*,#11042,.F.);
#15718=ORIENTED_EDGE('',*,*,#11043,.F.);
#15719=ORIENTED_EDGE('',*,*,#11044,.F.);
#15720=ORIENTED_EDGE('',*,*,#11045,.F.);
#15721=ORIENTED_EDGE('',*,*,#11046,.F.);
#15722=ORIENTED_EDGE('',*,*,#11047,.F.);
#15723=ORIENTED_EDGE('',*,*,#11048,.F.);
#15724=ORIENTED_EDGE('',*,*,#11049,.F.);
#15725=ORIENTED_EDGE('',*,*,#11050,.F.);
#15726=ORIENTED_EDGE('',*,*,#10891,.F.);
#15727=ORIENTED_EDGE('',*,*,#10882,.F.);
#15728=ORIENTED_EDGE('',*,*,#10884,.F.);
#15729=ORIENTED_EDGE('',*,*,#10888,.F.);
#15730=ORIENTED_EDGE('',*,*,#10893,.T.);
#15731=ORIENTED_EDGE('',*,*,#11051,.F.);
#15732=ORIENTED_EDGE('',*,*,#11052,.T.);
#15733=ORIENTED_EDGE('',*,*,#11003,.T.);
#15734=ORIENTED_EDGE('',*,*,#10896,.T.);
#15735=ORIENTED_EDGE('',*,*,#10773,.F.);
#15736=ORIENTED_EDGE('',*,*,#11053,.T.);
#15737=ORIENTED_EDGE('',*,*,#11051,.T.);
#15738=ORIENTED_EDGE('',*,*,#11053,.F.);
#15739=ORIENTED_EDGE('',*,*,#10772,.F.);
#15740=ORIENTED_EDGE('',*,*,#11054,.F.);
#15741=ORIENTED_EDGE('',*,*,#11004,.T.);
#15742=ORIENTED_EDGE('',*,*,#11052,.F.);
#15743=ORIENTED_EDGE('',*,*,#11005,.T.);
#15744=ORIENTED_EDGE('',*,*,#11054,.T.);
#15745=ORIENTED_EDGE('',*,*,#10771,.F.);
#15746=ORIENTED_EDGE('',*,*,#11055,.F.);
#15747=ORIENTED_EDGE('',*,*,#11056,.F.);
#15748=ORIENTED_EDGE('',*,*,#11057,.F.);
#15749=ORIENTED_EDGE('',*,*,#11006,.T.);
#15750=ORIENTED_EDGE('',*,*,#11055,.T.);
#15751=ORIENTED_EDGE('',*,*,#10770,.F.);
#15752=ORIENTED_EDGE('',*,*,#10886,.T.);
#15753=ORIENTED_EDGE('',*,*,#10777,.F.);
#15754=ORIENTED_EDGE('',*,*,#10900,.T.);
#15755=ORIENTED_EDGE('',*,*,#11058,.T.);
#15756=ORIENTED_EDGE('',*,*,#10887,.T.);
#15757=ORIENTED_EDGE('',*,*,#11058,.F.);
#15758=ORIENTED_EDGE('',*,*,#10899,.T.);
#15759=ORIENTED_EDGE('',*,*,#11002,.T.);
#15760=ORIENTED_EDGE('',*,*,#11059,.F.);
#15761=ORIENTED_EDGE('',*,*,#11010,.T.);
#15762=ORIENTED_EDGE('',*,*,#11060,.T.);
#15763=ORIENTED_EDGE('',*,*,#10766,.F.);
#15764=ORIENTED_EDGE('',*,*,#11061,.F.);
#15765=ORIENTED_EDGE('',*,*,#11009,.T.);
#15766=ORIENTED_EDGE('',*,*,#11062,.T.);
#15767=ORIENTED_EDGE('',*,*,#10767,.F.);
#15768=ORIENTED_EDGE('',*,*,#11060,.F.);
#15769=ORIENTED_EDGE('',*,*,#11063,.F.);
#15770=ORIENTED_EDGE('',*,*,#11064,.F.);
#15771=ORIENTED_EDGE('',*,*,#10768,.F.);
#15772=ORIENTED_EDGE('',*,*,#11062,.F.);
#15773=ORIENTED_EDGE('',*,*,#11008,.T.);
#15774=ORIENTED_EDGE('',*,*,#11059,.T.);
#15775=ORIENTED_EDGE('',*,*,#11065,.F.);
#15776=ORIENTED_EDGE('',*,*,#11066,.T.);
#15777=ORIENTED_EDGE('',*,*,#11011,.T.);
#15778=ORIENTED_EDGE('',*,*,#11061,.T.);
#15779=ORIENTED_EDGE('',*,*,#10765,.F.);
#15780=ORIENTED_EDGE('',*,*,#11067,.T.);
#15781=ORIENTED_EDGE('',*,*,#11065,.T.);
#15782=ORIENTED_EDGE('',*,*,#11067,.F.);
#15783=ORIENTED_EDGE('',*,*,#10764,.F.);
#15784=ORIENTED_EDGE('',*,*,#11068,.F.);
#15785=ORIENTED_EDGE('',*,*,#11012,.T.);
#15786=ORIENTED_EDGE('',*,*,#11066,.F.);
#15787=ORIENTED_EDGE('',*,*,#11013,.T.);
#15788=ORIENTED_EDGE('',*,*,#11068,.T.);
#15789=ORIENTED_EDGE('',*,*,#10763,.F.);
#15790=ORIENTED_EDGE('',*,*,#11069,.F.);
#15791=ORIENTED_EDGE('',*,*,#11070,.F.);
#15792=ORIENTED_EDGE('',*,*,#11071,.F.);
#15793=ORIENTED_EDGE('',*,*,#11014,.T.);
#15794=ORIENTED_EDGE('',*,*,#11069,.T.);
#15795=ORIENTED_EDGE('',*,*,#10762,.F.);
#15796=ORIENTED_EDGE('',*,*,#11056,.T.);
#15797=ORIENTED_EDGE('',*,*,#10769,.F.);
#15798=ORIENTED_EDGE('',*,*,#11064,.T.);
#15799=ORIENTED_EDGE('',*,*,#11072,.T.);
#15800=ORIENTED_EDGE('',*,*,#11057,.T.);
#15801=ORIENTED_EDGE('',*,*,#11072,.F.);
#15802=ORIENTED_EDGE('',*,*,#11063,.T.);
#15803=ORIENTED_EDGE('',*,*,#11007,.T.);
#15804=ORIENTED_EDGE('',*,*,#11073,.F.);
#15805=ORIENTED_EDGE('',*,*,#11018,.T.);
#15806=ORIENTED_EDGE('',*,*,#11074,.T.);
#15807=ORIENTED_EDGE('',*,*,#10758,.F.);
#15808=ORIENTED_EDGE('',*,*,#11075,.F.);
#15809=ORIENTED_EDGE('',*,*,#11017,.T.);
#15810=ORIENTED_EDGE('',*,*,#11076,.T.);
#15811=ORIENTED_EDGE('',*,*,#10759,.F.);
#15812=ORIENTED_EDGE('',*,*,#11074,.F.);
#15813=ORIENTED_EDGE('',*,*,#11077,.F.);
#15814=ORIENTED_EDGE('',*,*,#11078,.F.);
#15815=ORIENTED_EDGE('',*,*,#10760,.F.);
#15816=ORIENTED_EDGE('',*,*,#11076,.F.);
#15817=ORIENTED_EDGE('',*,*,#11016,.T.);
#15818=ORIENTED_EDGE('',*,*,#11073,.T.);
#15819=ORIENTED_EDGE('',*,*,#11079,.F.);
#15820=ORIENTED_EDGE('',*,*,#11080,.T.);
#15821=ORIENTED_EDGE('',*,*,#11019,.T.);
#15822=ORIENTED_EDGE('',*,*,#11075,.T.);
#15823=ORIENTED_EDGE('',*,*,#10757,.F.);
#15824=ORIENTED_EDGE('',*,*,#11081,.T.);
#15825=ORIENTED_EDGE('',*,*,#11079,.T.);
#15826=ORIENTED_EDGE('',*,*,#11081,.F.);
#15827=ORIENTED_EDGE('',*,*,#10756,.F.);
#15828=ORIENTED_EDGE('',*,*,#11082,.F.);
#15829=ORIENTED_EDGE('',*,*,#11020,.T.);
#15830=ORIENTED_EDGE('',*,*,#11080,.F.);
#15831=ORIENTED_EDGE('',*,*,#11021,.T.);
#15832=ORIENTED_EDGE('',*,*,#11082,.T.);
#15833=ORIENTED_EDGE('',*,*,#10755,.F.);
#15834=ORIENTED_EDGE('',*,*,#11083,.F.);
#15835=ORIENTED_EDGE('',*,*,#11084,.F.);
#15836=ORIENTED_EDGE('',*,*,#11085,.F.);
#15837=ORIENTED_EDGE('',*,*,#11022,.T.);
#15838=ORIENTED_EDGE('',*,*,#11083,.T.);
#15839=ORIENTED_EDGE('',*,*,#10754,.F.);
#15840=ORIENTED_EDGE('',*,*,#11070,.T.);
#15841=ORIENTED_EDGE('',*,*,#10761,.F.);
#15842=ORIENTED_EDGE('',*,*,#11078,.T.);
#15843=ORIENTED_EDGE('',*,*,#11086,.T.);
#15844=ORIENTED_EDGE('',*,*,#11071,.T.);
#15845=ORIENTED_EDGE('',*,*,#11086,.F.);
#15846=ORIENTED_EDGE('',*,*,#11077,.T.);
#15847=ORIENTED_EDGE('',*,*,#11015,.T.);
#15848=ORIENTED_EDGE('',*,*,#11087,.F.);
#15849=ORIENTED_EDGE('',*,*,#11026,.T.);
#15850=ORIENTED_EDGE('',*,*,#11088,.T.);
#15851=ORIENTED_EDGE('',*,*,#10750,.F.);
#15852=ORIENTED_EDGE('',*,*,#11089,.F.);
#15853=ORIENTED_EDGE('',*,*,#11025,.T.);
#15854=ORIENTED_EDGE('',*,*,#11090,.T.);
#15855=ORIENTED_EDGE('',*,*,#10751,.F.);
#15856=ORIENTED_EDGE('',*,*,#11088,.F.);
#15857=ORIENTED_EDGE('',*,*,#11091,.F.);
#15858=ORIENTED_EDGE('',*,*,#11092,.F.);
#15859=ORIENTED_EDGE('',*,*,#10752,.F.);
#15860=ORIENTED_EDGE('',*,*,#11090,.F.);
#15861=ORIENTED_EDGE('',*,*,#11024,.T.);
#15862=ORIENTED_EDGE('',*,*,#11087,.T.);
#15863=ORIENTED_EDGE('',*,*,#11093,.F.);
#15864=ORIENTED_EDGE('',*,*,#11094,.T.);
#15865=ORIENTED_EDGE('',*,*,#11027,.T.);
#15866=ORIENTED_EDGE('',*,*,#11089,.T.);
#15867=ORIENTED_EDGE('',*,*,#10749,.F.);
#15868=ORIENTED_EDGE('',*,*,#11095,.T.);
#15869=ORIENTED_EDGE('',*,*,#11093,.T.);
#15870=ORIENTED_EDGE('',*,*,#11095,.F.);
#15871=ORIENTED_EDGE('',*,*,#10748,.F.);
#15872=ORIENTED_EDGE('',*,*,#11096,.F.);
#15873=ORIENTED_EDGE('',*,*,#11028,.T.);
#15874=ORIENTED_EDGE('',*,*,#11094,.F.);
#15875=ORIENTED_EDGE('',*,*,#11029,.T.);
#15876=ORIENTED_EDGE('',*,*,#11096,.T.);
#15877=ORIENTED_EDGE('',*,*,#10747,.F.);
#15878=ORIENTED_EDGE('',*,*,#11097,.F.);
#15879=ORIENTED_EDGE('',*,*,#11098,.F.);
#15880=ORIENTED_EDGE('',*,*,#11099,.F.);
#15881=ORIENTED_EDGE('',*,*,#11030,.T.);
#15882=ORIENTED_EDGE('',*,*,#11097,.T.);
#15883=ORIENTED_EDGE('',*,*,#10746,.F.);
#15884=ORIENTED_EDGE('',*,*,#11084,.T.);
#15885=ORIENTED_EDGE('',*,*,#10753,.F.);
#15886=ORIENTED_EDGE('',*,*,#11092,.T.);
#15887=ORIENTED_EDGE('',*,*,#11100,.T.);
#15888=ORIENTED_EDGE('',*,*,#11085,.T.);
#15889=ORIENTED_EDGE('',*,*,#11100,.F.);
#15890=ORIENTED_EDGE('',*,*,#11091,.T.);
#15891=ORIENTED_EDGE('',*,*,#11023,.T.);
#15892=ORIENTED_EDGE('',*,*,#11101,.F.);
#15893=ORIENTED_EDGE('',*,*,#11034,.T.);
#15894=ORIENTED_EDGE('',*,*,#11102,.T.);
#15895=ORIENTED_EDGE('',*,*,#10742,.F.);
#15896=ORIENTED_EDGE('',*,*,#11103,.F.);
#15897=ORIENTED_EDGE('',*,*,#11033,.T.);
#15898=ORIENTED_EDGE('',*,*,#11104,.T.);
#15899=ORIENTED_EDGE('',*,*,#10743,.F.);
#15900=ORIENTED_EDGE('',*,*,#11102,.F.);
#15901=ORIENTED_EDGE('',*,*,#11105,.F.);
#15902=ORIENTED_EDGE('',*,*,#11106,.F.);
#15903=ORIENTED_EDGE('',*,*,#10744,.F.);
#15904=ORIENTED_EDGE('',*,*,#11104,.F.);
#15905=ORIENTED_EDGE('',*,*,#11032,.T.);
#15906=ORIENTED_EDGE('',*,*,#11101,.T.);
#15907=ORIENTED_EDGE('',*,*,#11107,.F.);
#15908=ORIENTED_EDGE('',*,*,#11108,.T.);
#15909=ORIENTED_EDGE('',*,*,#11035,.T.);
#15910=ORIENTED_EDGE('',*,*,#11103,.T.);
#15911=ORIENTED_EDGE('',*,*,#10741,.F.);
#15912=ORIENTED_EDGE('',*,*,#11109,.T.);
#15913=ORIENTED_EDGE('',*,*,#11107,.T.);
#15914=ORIENTED_EDGE('',*,*,#11109,.F.);
#15915=ORIENTED_EDGE('',*,*,#10740,.F.);
#15916=ORIENTED_EDGE('',*,*,#11110,.F.);
#15917=ORIENTED_EDGE('',*,*,#11036,.T.);
#15918=ORIENTED_EDGE('',*,*,#11108,.F.);
#15919=ORIENTED_EDGE('',*,*,#11037,.T.);
#15920=ORIENTED_EDGE('',*,*,#11110,.T.);
#15921=ORIENTED_EDGE('',*,*,#10739,.F.);
#15922=ORIENTED_EDGE('',*,*,#11111,.F.);
#15923=ORIENTED_EDGE('',*,*,#11112,.F.);
#15924=ORIENTED_EDGE('',*,*,#11113,.F.);
#15925=ORIENTED_EDGE('',*,*,#11038,.T.);
#15926=ORIENTED_EDGE('',*,*,#11111,.T.);
#15927=ORIENTED_EDGE('',*,*,#10738,.F.);
#15928=ORIENTED_EDGE('',*,*,#11098,.T.);
#15929=ORIENTED_EDGE('',*,*,#10745,.F.);
#15930=ORIENTED_EDGE('',*,*,#11106,.T.);
#15931=ORIENTED_EDGE('',*,*,#11114,.T.);
#15932=ORIENTED_EDGE('',*,*,#11099,.T.);
#15933=ORIENTED_EDGE('',*,*,#11114,.F.);
#15934=ORIENTED_EDGE('',*,*,#11105,.T.);
#15935=ORIENTED_EDGE('',*,*,#11031,.T.);
#15936=ORIENTED_EDGE('',*,*,#11115,.F.);
#15937=ORIENTED_EDGE('',*,*,#11042,.T.);
#15938=ORIENTED_EDGE('',*,*,#11116,.T.);
#15939=ORIENTED_EDGE('',*,*,#10734,.F.);
#15940=ORIENTED_EDGE('',*,*,#11117,.F.);
#15941=ORIENTED_EDGE('',*,*,#11041,.T.);
#15942=ORIENTED_EDGE('',*,*,#11118,.T.);
#15943=ORIENTED_EDGE('',*,*,#10735,.F.);
#15944=ORIENTED_EDGE('',*,*,#11116,.F.);
#15945=ORIENTED_EDGE('',*,*,#11119,.F.);
#15946=ORIENTED_EDGE('',*,*,#11120,.F.);
#15947=ORIENTED_EDGE('',*,*,#10736,.F.);
#15948=ORIENTED_EDGE('',*,*,#11118,.F.);
#15949=ORIENTED_EDGE('',*,*,#11040,.T.);
#15950=ORIENTED_EDGE('',*,*,#11115,.T.);
#15951=ORIENTED_EDGE('',*,*,#11121,.F.);
#15952=ORIENTED_EDGE('',*,*,#11122,.T.);
#15953=ORIENTED_EDGE('',*,*,#11043,.T.);
#15954=ORIENTED_EDGE('',*,*,#11117,.T.);
#15955=ORIENTED_EDGE('',*,*,#10733,.F.);
#15956=ORIENTED_EDGE('',*,*,#11123,.T.);
#15957=ORIENTED_EDGE('',*,*,#11121,.T.);
#15958=ORIENTED_EDGE('',*,*,#11123,.F.);
#15959=ORIENTED_EDGE('',*,*,#10732,.F.);
#15960=ORIENTED_EDGE('',*,*,#11124,.F.);
#15961=ORIENTED_EDGE('',*,*,#11044,.T.);
#15962=ORIENTED_EDGE('',*,*,#11122,.F.);
#15963=ORIENTED_EDGE('',*,*,#11045,.T.);
#15964=ORIENTED_EDGE('',*,*,#11124,.T.);
#15965=ORIENTED_EDGE('',*,*,#10731,.F.);
#15966=ORIENTED_EDGE('',*,*,#11125,.F.);
#15967=ORIENTED_EDGE('',*,*,#11126,.F.);
#15968=ORIENTED_EDGE('',*,*,#11127,.F.);
#15969=ORIENTED_EDGE('',*,*,#11046,.T.);
#15970=ORIENTED_EDGE('',*,*,#11125,.T.);
#15971=ORIENTED_EDGE('',*,*,#10730,.F.);
#15972=ORIENTED_EDGE('',*,*,#11112,.T.);
#15973=ORIENTED_EDGE('',*,*,#10737,.F.);
#15974=ORIENTED_EDGE('',*,*,#11120,.T.);
#15975=ORIENTED_EDGE('',*,*,#11128,.T.);
#15976=ORIENTED_EDGE('',*,*,#11113,.T.);
#15977=ORIENTED_EDGE('',*,*,#11128,.F.);
#15978=ORIENTED_EDGE('',*,*,#11119,.T.);
#15979=ORIENTED_EDGE('',*,*,#11039,.T.);
#15980=ORIENTED_EDGE('',*,*,#11129,.F.);
#15981=ORIENTED_EDGE('',*,*,#10728,.F.);
#15982=ORIENTED_EDGE('',*,*,#11130,.F.);
#15983=ORIENTED_EDGE('',*,*,#11048,.T.);
#15984=ORIENTED_EDGE('',*,*,#11131,.F.);
#15985=ORIENTED_EDGE('',*,*,#11049,.T.);
#15986=ORIENTED_EDGE('',*,*,#11130,.T.);
#15987=ORIENTED_EDGE('',*,*,#10727,.F.);
#15988=ORIENTED_EDGE('',*,*,#11132,.F.);
#15989=ORIENTED_EDGE('',*,*,#10890,.F.);
#15990=ORIENTED_EDGE('',*,*,#10892,.F.);
#15991=ORIENTED_EDGE('',*,*,#11050,.T.);
#15992=ORIENTED_EDGE('',*,*,#11132,.T.);
#15993=ORIENTED_EDGE('',*,*,#10726,.F.);
#15994=ORIENTED_EDGE('',*,*,#11133,.F.);
#15995=ORIENTED_EDGE('',*,*,#10782,.F.);
#15996=ORIENTED_EDGE('',*,*,#11134,.T.);
#15997=ORIENTED_EDGE('',*,*,#11000,.F.);
#15998=ORIENTED_EDGE('',*,*,#11135,.F.);
#15999=ORIENTED_EDGE('',*,*,#11136,.F.);
#16000=ORIENTED_EDGE('',*,*,#10781,.F.);
#16001=ORIENTED_EDGE('',*,*,#11137,.T.);
#16002=ORIENTED_EDGE('',*,*,#11001,.F.);
#16003=ORIENTED_EDGE('',*,*,#11134,.F.);
#16004=ORIENTED_EDGE('',*,*,#11138,.F.);
#16005=ORIENTED_EDGE('',*,*,#11139,.F.);
#16006=ORIENTED_EDGE('',*,*,#11140,.F.);
#16007=ORIENTED_EDGE('',*,*,#10902,.F.);
#16008=ORIENTED_EDGE('',*,*,#11137,.F.);
#16009=ORIENTED_EDGE('',*,*,#10780,.F.);
#16010=ORIENTED_EDGE('',*,*,#11133,.T.);
#16011=ORIENTED_EDGE('',*,*,#11141,.F.);
#16012=ORIENTED_EDGE('',*,*,#11142,.T.);
#16013=ORIENTED_EDGE('',*,*,#10783,.T.);
#16014=ORIENTED_EDGE('',*,*,#11136,.T.);
#16015=ORIENTED_EDGE('',*,*,#11143,.F.);
#16016=ORIENTED_EDGE('',*,*,#11144,.T.);
#16017=ORIENTED_EDGE('',*,*,#11141,.T.);
#16018=ORIENTED_EDGE('',*,*,#11135,.T.);
#16019=ORIENTED_EDGE('',*,*,#10999,.F.);
#16020=ORIENTED_EDGE('',*,*,#11145,.T.);
#16021=ORIENTED_EDGE('',*,*,#11143,.T.);
#16022=ORIENTED_EDGE('',*,*,#11146,.F.);
#16023=ORIENTED_EDGE('',*,*,#10786,.F.);
#16024=ORIENTED_EDGE('',*,*,#11147,.T.);
#16025=ORIENTED_EDGE('',*,*,#10996,.F.);
#16026=ORIENTED_EDGE('',*,*,#11148,.F.);
#16027=ORIENTED_EDGE('',*,*,#11149,.F.);
#16028=ORIENTED_EDGE('',*,*,#10785,.F.);
#16029=ORIENTED_EDGE('',*,*,#11150,.T.);
#16030=ORIENTED_EDGE('',*,*,#10997,.F.);
#16031=ORIENTED_EDGE('',*,*,#11147,.F.);
#16032=ORIENTED_EDGE('',*,*,#11142,.F.);
#16033=ORIENTED_EDGE('',*,*,#11144,.F.);
#16034=ORIENTED_EDGE('',*,*,#11145,.F.);
#16035=ORIENTED_EDGE('',*,*,#10998,.F.);
#16036=ORIENTED_EDGE('',*,*,#11150,.F.);
#16037=ORIENTED_EDGE('',*,*,#10784,.F.);
#16038=ORIENTED_EDGE('',*,*,#11146,.T.);
#16039=ORIENTED_EDGE('',*,*,#11151,.F.);
#16040=ORIENTED_EDGE('',*,*,#11152,.T.);
#16041=ORIENTED_EDGE('',*,*,#10787,.T.);
#16042=ORIENTED_EDGE('',*,*,#11149,.T.);
#16043=ORIENTED_EDGE('',*,*,#11153,.F.);
#16044=ORIENTED_EDGE('',*,*,#11154,.T.);
#16045=ORIENTED_EDGE('',*,*,#11151,.T.);
#16046=ORIENTED_EDGE('',*,*,#11148,.T.);
#16047=ORIENTED_EDGE('',*,*,#10995,.F.);
#16048=ORIENTED_EDGE('',*,*,#11155,.T.);
#16049=ORIENTED_EDGE('',*,*,#11153,.T.);
#16050=ORIENTED_EDGE('',*,*,#11156,.F.);
#16051=ORIENTED_EDGE('',*,*,#10790,.F.);
#16052=ORIENTED_EDGE('',*,*,#11157,.T.);
#16053=ORIENTED_EDGE('',*,*,#10992,.F.);
#16054=ORIENTED_EDGE('',*,*,#11158,.F.);
#16055=ORIENTED_EDGE('',*,*,#11159,.F.);
#16056=ORIENTED_EDGE('',*,*,#10789,.F.);
#16057=ORIENTED_EDGE('',*,*,#11160,.T.);
#16058=ORIENTED_EDGE('',*,*,#10993,.F.);
#16059=ORIENTED_EDGE('',*,*,#11157,.F.);
#16060=ORIENTED_EDGE('',*,*,#11152,.F.);
#16061=ORIENTED_EDGE('',*,*,#11154,.F.);
#16062=ORIENTED_EDGE('',*,*,#11155,.F.);
#16063=ORIENTED_EDGE('',*,*,#10994,.F.);
#16064=ORIENTED_EDGE('',*,*,#11160,.F.);
#16065=ORIENTED_EDGE('',*,*,#10788,.F.);
#16066=ORIENTED_EDGE('',*,*,#11156,.T.);
#16067=ORIENTED_EDGE('',*,*,#11161,.F.);
#16068=ORIENTED_EDGE('',*,*,#11162,.T.);
#16069=ORIENTED_EDGE('',*,*,#10791,.T.);
#16070=ORIENTED_EDGE('',*,*,#11159,.T.);
#16071=ORIENTED_EDGE('',*,*,#11163,.F.);
#16072=ORIENTED_EDGE('',*,*,#11164,.T.);
#16073=ORIENTED_EDGE('',*,*,#11161,.T.);
#16074=ORIENTED_EDGE('',*,*,#11158,.T.);
#16075=ORIENTED_EDGE('',*,*,#10991,.F.);
#16076=ORIENTED_EDGE('',*,*,#11165,.T.);
#16077=ORIENTED_EDGE('',*,*,#11163,.T.);
#16078=ORIENTED_EDGE('',*,*,#11166,.F.);
#16079=ORIENTED_EDGE('',*,*,#10794,.F.);
#16080=ORIENTED_EDGE('',*,*,#11167,.T.);
#16081=ORIENTED_EDGE('',*,*,#10988,.F.);
#16082=ORIENTED_EDGE('',*,*,#11168,.F.);
#16083=ORIENTED_EDGE('',*,*,#11169,.F.);
#16084=ORIENTED_EDGE('',*,*,#10793,.F.);
#16085=ORIENTED_EDGE('',*,*,#11170,.T.);
#16086=ORIENTED_EDGE('',*,*,#10989,.F.);
#16087=ORIENTED_EDGE('',*,*,#11167,.F.);
#16088=ORIENTED_EDGE('',*,*,#11162,.F.);
#16089=ORIENTED_EDGE('',*,*,#11164,.F.);
#16090=ORIENTED_EDGE('',*,*,#11165,.F.);
#16091=ORIENTED_EDGE('',*,*,#10990,.F.);
#16092=ORIENTED_EDGE('',*,*,#11170,.F.);
#16093=ORIENTED_EDGE('',*,*,#10792,.F.);
#16094=ORIENTED_EDGE('',*,*,#11166,.T.);
#16095=ORIENTED_EDGE('',*,*,#11171,.F.);
#16096=ORIENTED_EDGE('',*,*,#11172,.T.);
#16097=ORIENTED_EDGE('',*,*,#10795,.T.);
#16098=ORIENTED_EDGE('',*,*,#11169,.T.);
#16099=ORIENTED_EDGE('',*,*,#11173,.F.);
#16100=ORIENTED_EDGE('',*,*,#11174,.T.);
#16101=ORIENTED_EDGE('',*,*,#11171,.T.);
#16102=ORIENTED_EDGE('',*,*,#11168,.T.);
#16103=ORIENTED_EDGE('',*,*,#10987,.F.);
#16104=ORIENTED_EDGE('',*,*,#11175,.T.);
#16105=ORIENTED_EDGE('',*,*,#11173,.T.);
#16106=ORIENTED_EDGE('',*,*,#11176,.F.);
#16107=ORIENTED_EDGE('',*,*,#10798,.F.);
#16108=ORIENTED_EDGE('',*,*,#11177,.T.);
#16109=ORIENTED_EDGE('',*,*,#10984,.F.);
#16110=ORIENTED_EDGE('',*,*,#11178,.F.);
#16111=ORIENTED_EDGE('',*,*,#11179,.F.);
#16112=ORIENTED_EDGE('',*,*,#10797,.F.);
#16113=ORIENTED_EDGE('',*,*,#11180,.T.);
#16114=ORIENTED_EDGE('',*,*,#10985,.F.);
#16115=ORIENTED_EDGE('',*,*,#11177,.F.);
#16116=ORIENTED_EDGE('',*,*,#11172,.F.);
#16117=ORIENTED_EDGE('',*,*,#11174,.F.);
#16118=ORIENTED_EDGE('',*,*,#11175,.F.);
#16119=ORIENTED_EDGE('',*,*,#10986,.F.);
#16120=ORIENTED_EDGE('',*,*,#11180,.F.);
#16121=ORIENTED_EDGE('',*,*,#10796,.F.);
#16122=ORIENTED_EDGE('',*,*,#11176,.T.);
#16123=ORIENTED_EDGE('',*,*,#11181,.F.);
#16124=ORIENTED_EDGE('',*,*,#11182,.T.);
#16125=ORIENTED_EDGE('',*,*,#10799,.T.);
#16126=ORIENTED_EDGE('',*,*,#11179,.T.);
#16127=ORIENTED_EDGE('',*,*,#11183,.F.);
#16128=ORIENTED_EDGE('',*,*,#11184,.T.);
#16129=ORIENTED_EDGE('',*,*,#11181,.T.);
#16130=ORIENTED_EDGE('',*,*,#11178,.T.);
#16131=ORIENTED_EDGE('',*,*,#10983,.F.);
#16132=ORIENTED_EDGE('',*,*,#11185,.T.);
#16133=ORIENTED_EDGE('',*,*,#11183,.T.);
#16134=ORIENTED_EDGE('',*,*,#11186,.F.);
#16135=ORIENTED_EDGE('',*,*,#10802,.F.);
#16136=ORIENTED_EDGE('',*,*,#11187,.T.);
#16137=ORIENTED_EDGE('',*,*,#10980,.F.);
#16138=ORIENTED_EDGE('',*,*,#11188,.F.);
#16139=ORIENTED_EDGE('',*,*,#11189,.F.);
#16140=ORIENTED_EDGE('',*,*,#10801,.F.);
#16141=ORIENTED_EDGE('',*,*,#11190,.T.);
#16142=ORIENTED_EDGE('',*,*,#10981,.F.);
#16143=ORIENTED_EDGE('',*,*,#11187,.F.);
#16144=ORIENTED_EDGE('',*,*,#11182,.F.);
#16145=ORIENTED_EDGE('',*,*,#11184,.F.);
#16146=ORIENTED_EDGE('',*,*,#11185,.F.);
#16147=ORIENTED_EDGE('',*,*,#10982,.F.);
#16148=ORIENTED_EDGE('',*,*,#11190,.F.);
#16149=ORIENTED_EDGE('',*,*,#10800,.F.);
#16150=ORIENTED_EDGE('',*,*,#11186,.T.);
#16151=ORIENTED_EDGE('',*,*,#11191,.F.);
#16152=ORIENTED_EDGE('',*,*,#11192,.T.);
#16153=ORIENTED_EDGE('',*,*,#10803,.T.);
#16154=ORIENTED_EDGE('',*,*,#11189,.T.);
#16155=ORIENTED_EDGE('',*,*,#11193,.F.);
#16156=ORIENTED_EDGE('',*,*,#11194,.T.);
#16157=ORIENTED_EDGE('',*,*,#11191,.T.);
#16158=ORIENTED_EDGE('',*,*,#11188,.T.);
#16159=ORIENTED_EDGE('',*,*,#10979,.F.);
#16160=ORIENTED_EDGE('',*,*,#11195,.T.);
#16161=ORIENTED_EDGE('',*,*,#11193,.T.);
#16162=ORIENTED_EDGE('',*,*,#11196,.F.);
#16163=ORIENTED_EDGE('',*,*,#10806,.F.);
#16164=ORIENTED_EDGE('',*,*,#11197,.T.);
#16165=ORIENTED_EDGE('',*,*,#10976,.F.);
#16166=ORIENTED_EDGE('',*,*,#11198,.F.);
#16167=ORIENTED_EDGE('',*,*,#11199,.F.);
#16168=ORIENTED_EDGE('',*,*,#10805,.F.);
#16169=ORIENTED_EDGE('',*,*,#11200,.T.);
#16170=ORIENTED_EDGE('',*,*,#10977,.F.);
#16171=ORIENTED_EDGE('',*,*,#11197,.F.);
#16172=ORIENTED_EDGE('',*,*,#11192,.F.);
#16173=ORIENTED_EDGE('',*,*,#11194,.F.);
#16174=ORIENTED_EDGE('',*,*,#11195,.F.);
#16175=ORIENTED_EDGE('',*,*,#10978,.F.);
#16176=ORIENTED_EDGE('',*,*,#11200,.F.);
#16177=ORIENTED_EDGE('',*,*,#10804,.F.);
#16178=ORIENTED_EDGE('',*,*,#11196,.T.);
#16179=ORIENTED_EDGE('',*,*,#11201,.F.);
#16180=ORIENTED_EDGE('',*,*,#11202,.T.);
#16181=ORIENTED_EDGE('',*,*,#10807,.T.);
#16182=ORIENTED_EDGE('',*,*,#11199,.T.);
#16183=ORIENTED_EDGE('',*,*,#11203,.F.);
#16184=ORIENTED_EDGE('',*,*,#11204,.T.);
#16185=ORIENTED_EDGE('',*,*,#11201,.T.);
#16186=ORIENTED_EDGE('',*,*,#11198,.T.);
#16187=ORIENTED_EDGE('',*,*,#10975,.F.);
#16188=ORIENTED_EDGE('',*,*,#11205,.T.);
#16189=ORIENTED_EDGE('',*,*,#11203,.T.);
#16190=ORIENTED_EDGE('',*,*,#11206,.F.);
#16191=ORIENTED_EDGE('',*,*,#10810,.F.);
#16192=ORIENTED_EDGE('',*,*,#11207,.T.);
#16193=ORIENTED_EDGE('',*,*,#10972,.F.);
#16194=ORIENTED_EDGE('',*,*,#11208,.F.);
#16195=ORIENTED_EDGE('',*,*,#11209,.F.);
#16196=ORIENTED_EDGE('',*,*,#10809,.F.);
#16197=ORIENTED_EDGE('',*,*,#11210,.T.);
#16198=ORIENTED_EDGE('',*,*,#10973,.F.);
#16199=ORIENTED_EDGE('',*,*,#11207,.F.);
#16200=ORIENTED_EDGE('',*,*,#11202,.F.);
#16201=ORIENTED_EDGE('',*,*,#11204,.F.);
#16202=ORIENTED_EDGE('',*,*,#11205,.F.);
#16203=ORIENTED_EDGE('',*,*,#10974,.F.);
#16204=ORIENTED_EDGE('',*,*,#11210,.F.);
#16205=ORIENTED_EDGE('',*,*,#10808,.F.);
#16206=ORIENTED_EDGE('',*,*,#11206,.T.);
#16207=ORIENTED_EDGE('',*,*,#11211,.F.);
#16208=ORIENTED_EDGE('',*,*,#11212,.T.);
#16209=ORIENTED_EDGE('',*,*,#10811,.T.);
#16210=ORIENTED_EDGE('',*,*,#11209,.T.);
#16211=ORIENTED_EDGE('',*,*,#11213,.F.);
#16212=ORIENTED_EDGE('',*,*,#11214,.T.);
#16213=ORIENTED_EDGE('',*,*,#11211,.T.);
#16214=ORIENTED_EDGE('',*,*,#11208,.T.);
#16215=ORIENTED_EDGE('',*,*,#10971,.F.);
#16216=ORIENTED_EDGE('',*,*,#11215,.T.);
#16217=ORIENTED_EDGE('',*,*,#11213,.T.);
#16218=ORIENTED_EDGE('',*,*,#11216,.F.);
#16219=ORIENTED_EDGE('',*,*,#10814,.F.);
#16220=ORIENTED_EDGE('',*,*,#11217,.T.);
#16221=ORIENTED_EDGE('',*,*,#10968,.F.);
#16222=ORIENTED_EDGE('',*,*,#11218,.F.);
#16223=ORIENTED_EDGE('',*,*,#11219,.F.);
#16224=ORIENTED_EDGE('',*,*,#10813,.F.);
#16225=ORIENTED_EDGE('',*,*,#11220,.T.);
#16226=ORIENTED_EDGE('',*,*,#10969,.F.);
#16227=ORIENTED_EDGE('',*,*,#11217,.F.);
#16228=ORIENTED_EDGE('',*,*,#11212,.F.);
#16229=ORIENTED_EDGE('',*,*,#11214,.F.);
#16230=ORIENTED_EDGE('',*,*,#11215,.F.);
#16231=ORIENTED_EDGE('',*,*,#10970,.F.);
#16232=ORIENTED_EDGE('',*,*,#11220,.F.);
#16233=ORIENTED_EDGE('',*,*,#10812,.F.);
#16234=ORIENTED_EDGE('',*,*,#11216,.T.);
#16235=ORIENTED_EDGE('',*,*,#11221,.F.);
#16236=ORIENTED_EDGE('',*,*,#11222,.T.);
#16237=ORIENTED_EDGE('',*,*,#10815,.T.);
#16238=ORIENTED_EDGE('',*,*,#11219,.T.);
#16239=ORIENTED_EDGE('',*,*,#11223,.F.);
#16240=ORIENTED_EDGE('',*,*,#11224,.T.);
#16241=ORIENTED_EDGE('',*,*,#11221,.T.);
#16242=ORIENTED_EDGE('',*,*,#11218,.T.);
#16243=ORIENTED_EDGE('',*,*,#10967,.F.);
#16244=ORIENTED_EDGE('',*,*,#11225,.T.);
#16245=ORIENTED_EDGE('',*,*,#11223,.T.);
#16246=ORIENTED_EDGE('',*,*,#11226,.F.);
#16247=ORIENTED_EDGE('',*,*,#10818,.F.);
#16248=ORIENTED_EDGE('',*,*,#11227,.T.);
#16249=ORIENTED_EDGE('',*,*,#10964,.F.);
#16250=ORIENTED_EDGE('',*,*,#11228,.F.);
#16251=ORIENTED_EDGE('',*,*,#11229,.F.);
#16252=ORIENTED_EDGE('',*,*,#10817,.F.);
#16253=ORIENTED_EDGE('',*,*,#11230,.T.);
#16254=ORIENTED_EDGE('',*,*,#10965,.F.);
#16255=ORIENTED_EDGE('',*,*,#11227,.F.);
#16256=ORIENTED_EDGE('',*,*,#11222,.F.);
#16257=ORIENTED_EDGE('',*,*,#11224,.F.);
#16258=ORIENTED_EDGE('',*,*,#11225,.F.);
#16259=ORIENTED_EDGE('',*,*,#10966,.F.);
#16260=ORIENTED_EDGE('',*,*,#11230,.F.);
#16261=ORIENTED_EDGE('',*,*,#10816,.F.);
#16262=ORIENTED_EDGE('',*,*,#11226,.T.);
#16263=ORIENTED_EDGE('',*,*,#11231,.F.);
#16264=ORIENTED_EDGE('',*,*,#11232,.T.);
#16265=ORIENTED_EDGE('',*,*,#10819,.T.);
#16266=ORIENTED_EDGE('',*,*,#11229,.T.);
#16267=ORIENTED_EDGE('',*,*,#11233,.F.);
#16268=ORIENTED_EDGE('',*,*,#11234,.T.);
#16269=ORIENTED_EDGE('',*,*,#11231,.T.);
#16270=ORIENTED_EDGE('',*,*,#11228,.T.);
#16271=ORIENTED_EDGE('',*,*,#10963,.F.);
#16272=ORIENTED_EDGE('',*,*,#11235,.T.);
#16273=ORIENTED_EDGE('',*,*,#11233,.T.);
#16274=ORIENTED_EDGE('',*,*,#11236,.F.);
#16275=ORIENTED_EDGE('',*,*,#10822,.F.);
#16276=ORIENTED_EDGE('',*,*,#11237,.T.);
#16277=ORIENTED_EDGE('',*,*,#10960,.F.);
#16278=ORIENTED_EDGE('',*,*,#11238,.F.);
#16279=ORIENTED_EDGE('',*,*,#11239,.F.);
#16280=ORIENTED_EDGE('',*,*,#10821,.F.);
#16281=ORIENTED_EDGE('',*,*,#11240,.T.);
#16282=ORIENTED_EDGE('',*,*,#10961,.F.);
#16283=ORIENTED_EDGE('',*,*,#11237,.F.);
#16284=ORIENTED_EDGE('',*,*,#11232,.F.);
#16285=ORIENTED_EDGE('',*,*,#11234,.F.);
#16286=ORIENTED_EDGE('',*,*,#11235,.F.);
#16287=ORIENTED_EDGE('',*,*,#10962,.F.);
#16288=ORIENTED_EDGE('',*,*,#11240,.F.);
#16289=ORIENTED_EDGE('',*,*,#10820,.F.);
#16290=ORIENTED_EDGE('',*,*,#11236,.T.);
#16291=ORIENTED_EDGE('',*,*,#11241,.F.);
#16292=ORIENTED_EDGE('',*,*,#11242,.T.);
#16293=ORIENTED_EDGE('',*,*,#10823,.T.);
#16294=ORIENTED_EDGE('',*,*,#11239,.T.);
#16295=ORIENTED_EDGE('',*,*,#11243,.F.);
#16296=ORIENTED_EDGE('',*,*,#11244,.T.);
#16297=ORIENTED_EDGE('',*,*,#11241,.T.);
#16298=ORIENTED_EDGE('',*,*,#11238,.T.);
#16299=ORIENTED_EDGE('',*,*,#10959,.F.);
#16300=ORIENTED_EDGE('',*,*,#11245,.T.);
#16301=ORIENTED_EDGE('',*,*,#11243,.T.);
#16302=ORIENTED_EDGE('',*,*,#11246,.F.);
#16303=ORIENTED_EDGE('',*,*,#10826,.F.);
#16304=ORIENTED_EDGE('',*,*,#11247,.T.);
#16305=ORIENTED_EDGE('',*,*,#10956,.F.);
#16306=ORIENTED_EDGE('',*,*,#11248,.F.);
#16307=ORIENTED_EDGE('',*,*,#11249,.F.);
#16308=ORIENTED_EDGE('',*,*,#10825,.F.);
#16309=ORIENTED_EDGE('',*,*,#11250,.T.);
#16310=ORIENTED_EDGE('',*,*,#10957,.F.);
#16311=ORIENTED_EDGE('',*,*,#11247,.F.);
#16312=ORIENTED_EDGE('',*,*,#11242,.F.);
#16313=ORIENTED_EDGE('',*,*,#11244,.F.);
#16314=ORIENTED_EDGE('',*,*,#11245,.F.);
#16315=ORIENTED_EDGE('',*,*,#10958,.F.);
#16316=ORIENTED_EDGE('',*,*,#11250,.F.);
#16317=ORIENTED_EDGE('',*,*,#10824,.F.);
#16318=ORIENTED_EDGE('',*,*,#11246,.T.);
#16319=ORIENTED_EDGE('',*,*,#11251,.F.);
#16320=ORIENTED_EDGE('',*,*,#11252,.T.);
#16321=ORIENTED_EDGE('',*,*,#10827,.T.);
#16322=ORIENTED_EDGE('',*,*,#11249,.T.);
#16323=ORIENTED_EDGE('',*,*,#11253,.F.);
#16324=ORIENTED_EDGE('',*,*,#11254,.T.);
#16325=ORIENTED_EDGE('',*,*,#11251,.T.);
#16326=ORIENTED_EDGE('',*,*,#11248,.T.);
#16327=ORIENTED_EDGE('',*,*,#10955,.F.);
#16328=ORIENTED_EDGE('',*,*,#11255,.T.);
#16329=ORIENTED_EDGE('',*,*,#11253,.T.);
#16330=ORIENTED_EDGE('',*,*,#11256,.F.);
#16331=ORIENTED_EDGE('',*,*,#10830,.F.);
#16332=ORIENTED_EDGE('',*,*,#11257,.T.);
#16333=ORIENTED_EDGE('',*,*,#10952,.F.);
#16334=ORIENTED_EDGE('',*,*,#11258,.F.);
#16335=ORIENTED_EDGE('',*,*,#11259,.F.);
#16336=ORIENTED_EDGE('',*,*,#10829,.F.);
#16337=ORIENTED_EDGE('',*,*,#11260,.T.);
#16338=ORIENTED_EDGE('',*,*,#10953,.F.);
#16339=ORIENTED_EDGE('',*,*,#11257,.F.);
#16340=ORIENTED_EDGE('',*,*,#11252,.F.);
#16341=ORIENTED_EDGE('',*,*,#11254,.F.);
#16342=ORIENTED_EDGE('',*,*,#11255,.F.);
#16343=ORIENTED_EDGE('',*,*,#10954,.F.);
#16344=ORIENTED_EDGE('',*,*,#11260,.F.);
#16345=ORIENTED_EDGE('',*,*,#10828,.F.);
#16346=ORIENTED_EDGE('',*,*,#11256,.T.);
#16347=ORIENTED_EDGE('',*,*,#11261,.F.);
#16348=ORIENTED_EDGE('',*,*,#11262,.T.);
#16349=ORIENTED_EDGE('',*,*,#10831,.T.);
#16350=ORIENTED_EDGE('',*,*,#11259,.T.);
#16351=ORIENTED_EDGE('',*,*,#11263,.F.);
#16352=ORIENTED_EDGE('',*,*,#11264,.T.);
#16353=ORIENTED_EDGE('',*,*,#11261,.T.);
#16354=ORIENTED_EDGE('',*,*,#11258,.T.);
#16355=ORIENTED_EDGE('',*,*,#10951,.F.);
#16356=ORIENTED_EDGE('',*,*,#11265,.T.);
#16357=ORIENTED_EDGE('',*,*,#11263,.T.);
#16358=ORIENTED_EDGE('',*,*,#11266,.F.);
#16359=ORIENTED_EDGE('',*,*,#10834,.F.);
#16360=ORIENTED_EDGE('',*,*,#11267,.T.);
#16361=ORIENTED_EDGE('',*,*,#10948,.F.);
#16362=ORIENTED_EDGE('',*,*,#11268,.F.);
#16363=ORIENTED_EDGE('',*,*,#11269,.F.);
#16364=ORIENTED_EDGE('',*,*,#10833,.F.);
#16365=ORIENTED_EDGE('',*,*,#11270,.T.);
#16366=ORIENTED_EDGE('',*,*,#10949,.F.);
#16367=ORIENTED_EDGE('',*,*,#11267,.F.);
#16368=ORIENTED_EDGE('',*,*,#11262,.F.);
#16369=ORIENTED_EDGE('',*,*,#11264,.F.);
#16370=ORIENTED_EDGE('',*,*,#11265,.F.);
#16371=ORIENTED_EDGE('',*,*,#10950,.F.);
#16372=ORIENTED_EDGE('',*,*,#11270,.F.);
#16373=ORIENTED_EDGE('',*,*,#10832,.F.);
#16374=ORIENTED_EDGE('',*,*,#11266,.T.);
#16375=ORIENTED_EDGE('',*,*,#11271,.F.);
#16376=ORIENTED_EDGE('',*,*,#11272,.T.);
#16377=ORIENTED_EDGE('',*,*,#10835,.T.);
#16378=ORIENTED_EDGE('',*,*,#11269,.T.);
#16379=ORIENTED_EDGE('',*,*,#11273,.F.);
#16380=ORIENTED_EDGE('',*,*,#11274,.T.);
#16381=ORIENTED_EDGE('',*,*,#11271,.T.);
#16382=ORIENTED_EDGE('',*,*,#11268,.T.);
#16383=ORIENTED_EDGE('',*,*,#10947,.F.);
#16384=ORIENTED_EDGE('',*,*,#11275,.T.);
#16385=ORIENTED_EDGE('',*,*,#11273,.T.);
#16386=ORIENTED_EDGE('',*,*,#11276,.F.);
#16387=ORIENTED_EDGE('',*,*,#10838,.F.);
#16388=ORIENTED_EDGE('',*,*,#11277,.T.);
#16389=ORIENTED_EDGE('',*,*,#10944,.F.);
#16390=ORIENTED_EDGE('',*,*,#11278,.F.);
#16391=ORIENTED_EDGE('',*,*,#11279,.F.);
#16392=ORIENTED_EDGE('',*,*,#10837,.F.);
#16393=ORIENTED_EDGE('',*,*,#11280,.T.);
#16394=ORIENTED_EDGE('',*,*,#10945,.F.);
#16395=ORIENTED_EDGE('',*,*,#11277,.F.);
#16396=ORIENTED_EDGE('',*,*,#11272,.F.);
#16397=ORIENTED_EDGE('',*,*,#11274,.F.);
#16398=ORIENTED_EDGE('',*,*,#11275,.F.);
#16399=ORIENTED_EDGE('',*,*,#10946,.F.);
#16400=ORIENTED_EDGE('',*,*,#11280,.F.);
#16401=ORIENTED_EDGE('',*,*,#10836,.F.);
#16402=ORIENTED_EDGE('',*,*,#11276,.T.);
#16403=ORIENTED_EDGE('',*,*,#11281,.F.);
#16404=ORIENTED_EDGE('',*,*,#11282,.T.);
#16405=ORIENTED_EDGE('',*,*,#10839,.T.);
#16406=ORIENTED_EDGE('',*,*,#11279,.T.);
#16407=ORIENTED_EDGE('',*,*,#11283,.F.);
#16408=ORIENTED_EDGE('',*,*,#11284,.T.);
#16409=ORIENTED_EDGE('',*,*,#11281,.T.);
#16410=ORIENTED_EDGE('',*,*,#11278,.T.);
#16411=ORIENTED_EDGE('',*,*,#10943,.F.);
#16412=ORIENTED_EDGE('',*,*,#11285,.T.);
#16413=ORIENTED_EDGE('',*,*,#11283,.T.);
#16414=ORIENTED_EDGE('',*,*,#11286,.F.);
#16415=ORIENTED_EDGE('',*,*,#10842,.F.);
#16416=ORIENTED_EDGE('',*,*,#11287,.T.);
#16417=ORIENTED_EDGE('',*,*,#10940,.F.);
#16418=ORIENTED_EDGE('',*,*,#11288,.F.);
#16419=ORIENTED_EDGE('',*,*,#11289,.F.);
#16420=ORIENTED_EDGE('',*,*,#10841,.F.);
#16421=ORIENTED_EDGE('',*,*,#11290,.T.);
#16422=ORIENTED_EDGE('',*,*,#10941,.F.);
#16423=ORIENTED_EDGE('',*,*,#11287,.F.);
#16424=ORIENTED_EDGE('',*,*,#11282,.F.);
#16425=ORIENTED_EDGE('',*,*,#11284,.F.);
#16426=ORIENTED_EDGE('',*,*,#11285,.F.);
#16427=ORIENTED_EDGE('',*,*,#10942,.F.);
#16428=ORIENTED_EDGE('',*,*,#11290,.F.);
#16429=ORIENTED_EDGE('',*,*,#10840,.F.);
#16430=ORIENTED_EDGE('',*,*,#11286,.T.);
#16431=ORIENTED_EDGE('',*,*,#11291,.F.);
#16432=ORIENTED_EDGE('',*,*,#11292,.T.);
#16433=ORIENTED_EDGE('',*,*,#10843,.T.);
#16434=ORIENTED_EDGE('',*,*,#11289,.T.);
#16435=ORIENTED_EDGE('',*,*,#11293,.F.);
#16436=ORIENTED_EDGE('',*,*,#11294,.T.);
#16437=ORIENTED_EDGE('',*,*,#11291,.T.);
#16438=ORIENTED_EDGE('',*,*,#11288,.T.);
#16439=ORIENTED_EDGE('',*,*,#10939,.F.);
#16440=ORIENTED_EDGE('',*,*,#11295,.T.);
#16441=ORIENTED_EDGE('',*,*,#11293,.T.);
#16442=ORIENTED_EDGE('',*,*,#11296,.F.);
#16443=ORIENTED_EDGE('',*,*,#10846,.F.);
#16444=ORIENTED_EDGE('',*,*,#11297,.T.);
#16445=ORIENTED_EDGE('',*,*,#10936,.F.);
#16446=ORIENTED_EDGE('',*,*,#11298,.F.);
#16447=ORIENTED_EDGE('',*,*,#11299,.F.);
#16448=ORIENTED_EDGE('',*,*,#10845,.F.);
#16449=ORIENTED_EDGE('',*,*,#11300,.T.);
#16450=ORIENTED_EDGE('',*,*,#10937,.F.);
#16451=ORIENTED_EDGE('',*,*,#11297,.F.);
#16452=ORIENTED_EDGE('',*,*,#11292,.F.);
#16453=ORIENTED_EDGE('',*,*,#11294,.F.);
#16454=ORIENTED_EDGE('',*,*,#11295,.F.);
#16455=ORIENTED_EDGE('',*,*,#10938,.F.);
#16456=ORIENTED_EDGE('',*,*,#11300,.F.);
#16457=ORIENTED_EDGE('',*,*,#10844,.F.);
#16458=ORIENTED_EDGE('',*,*,#11296,.T.);
#16459=ORIENTED_EDGE('',*,*,#11301,.F.);
#16460=ORIENTED_EDGE('',*,*,#11302,.T.);
#16461=ORIENTED_EDGE('',*,*,#10847,.T.);
#16462=ORIENTED_EDGE('',*,*,#11299,.T.);
#16463=ORIENTED_EDGE('',*,*,#11303,.F.);
#16464=ORIENTED_EDGE('',*,*,#11304,.T.);
#16465=ORIENTED_EDGE('',*,*,#11301,.T.);
#16466=ORIENTED_EDGE('',*,*,#11298,.T.);
#16467=ORIENTED_EDGE('',*,*,#10935,.F.);
#16468=ORIENTED_EDGE('',*,*,#11305,.T.);
#16469=ORIENTED_EDGE('',*,*,#11303,.T.);
#16470=ORIENTED_EDGE('',*,*,#11306,.F.);
#16471=ORIENTED_EDGE('',*,*,#10850,.F.);
#16472=ORIENTED_EDGE('',*,*,#11307,.T.);
#16473=ORIENTED_EDGE('',*,*,#10932,.F.);
#16474=ORIENTED_EDGE('',*,*,#11308,.F.);
#16475=ORIENTED_EDGE('',*,*,#11309,.F.);
#16476=ORIENTED_EDGE('',*,*,#10849,.F.);
#16477=ORIENTED_EDGE('',*,*,#11310,.T.);
#16478=ORIENTED_EDGE('',*,*,#10933,.F.);
#16479=ORIENTED_EDGE('',*,*,#11307,.F.);
#16480=ORIENTED_EDGE('',*,*,#11302,.F.);
#16481=ORIENTED_EDGE('',*,*,#11304,.F.);
#16482=ORIENTED_EDGE('',*,*,#11305,.F.);
#16483=ORIENTED_EDGE('',*,*,#10934,.F.);
#16484=ORIENTED_EDGE('',*,*,#11310,.F.);
#16485=ORIENTED_EDGE('',*,*,#10848,.F.);
#16486=ORIENTED_EDGE('',*,*,#11306,.T.);
#16487=ORIENTED_EDGE('',*,*,#11311,.F.);
#16488=ORIENTED_EDGE('',*,*,#11312,.T.);
#16489=ORIENTED_EDGE('',*,*,#10851,.T.);
#16490=ORIENTED_EDGE('',*,*,#11309,.T.);
#16491=ORIENTED_EDGE('',*,*,#11313,.F.);
#16492=ORIENTED_EDGE('',*,*,#11314,.T.);
#16493=ORIENTED_EDGE('',*,*,#11311,.T.);
#16494=ORIENTED_EDGE('',*,*,#11308,.T.);
#16495=ORIENTED_EDGE('',*,*,#10931,.F.);
#16496=ORIENTED_EDGE('',*,*,#11315,.T.);
#16497=ORIENTED_EDGE('',*,*,#11313,.T.);
#16498=ORIENTED_EDGE('',*,*,#11316,.F.);
#16499=ORIENTED_EDGE('',*,*,#10854,.F.);
#16500=ORIENTED_EDGE('',*,*,#11317,.T.);
#16501=ORIENTED_EDGE('',*,*,#10928,.F.);
#16502=ORIENTED_EDGE('',*,*,#11318,.F.);
#16503=ORIENTED_EDGE('',*,*,#11319,.F.);
#16504=ORIENTED_EDGE('',*,*,#10853,.F.);
#16505=ORIENTED_EDGE('',*,*,#11320,.T.);
#16506=ORIENTED_EDGE('',*,*,#10929,.F.);
#16507=ORIENTED_EDGE('',*,*,#11317,.F.);
#16508=ORIENTED_EDGE('',*,*,#11312,.F.);
#16509=ORIENTED_EDGE('',*,*,#11314,.F.);
#16510=ORIENTED_EDGE('',*,*,#11315,.F.);
#16511=ORIENTED_EDGE('',*,*,#10930,.F.);
#16512=ORIENTED_EDGE('',*,*,#11320,.F.);
#16513=ORIENTED_EDGE('',*,*,#10852,.F.);
#16514=ORIENTED_EDGE('',*,*,#11316,.T.);
#16515=ORIENTED_EDGE('',*,*,#11321,.F.);
#16516=ORIENTED_EDGE('',*,*,#11322,.T.);
#16517=ORIENTED_EDGE('',*,*,#10855,.T.);
#16518=ORIENTED_EDGE('',*,*,#11319,.T.);
#16519=ORIENTED_EDGE('',*,*,#11323,.F.);
#16520=ORIENTED_EDGE('',*,*,#11324,.T.);
#16521=ORIENTED_EDGE('',*,*,#11321,.T.);
#16522=ORIENTED_EDGE('',*,*,#11318,.T.);
#16523=ORIENTED_EDGE('',*,*,#10927,.F.);
#16524=ORIENTED_EDGE('',*,*,#11325,.T.);
#16525=ORIENTED_EDGE('',*,*,#11323,.T.);
#16526=ORIENTED_EDGE('',*,*,#11326,.F.);
#16527=ORIENTED_EDGE('',*,*,#10858,.F.);
#16528=ORIENTED_EDGE('',*,*,#11327,.T.);
#16529=ORIENTED_EDGE('',*,*,#10924,.F.);
#16530=ORIENTED_EDGE('',*,*,#11328,.F.);
#16531=ORIENTED_EDGE('',*,*,#11329,.F.);
#16532=ORIENTED_EDGE('',*,*,#10857,.F.);
#16533=ORIENTED_EDGE('',*,*,#11330,.T.);
#16534=ORIENTED_EDGE('',*,*,#10925,.F.);
#16535=ORIENTED_EDGE('',*,*,#11327,.F.);
#16536=ORIENTED_EDGE('',*,*,#11322,.F.);
#16537=ORIENTED_EDGE('',*,*,#11324,.F.);
#16538=ORIENTED_EDGE('',*,*,#11325,.F.);
#16539=ORIENTED_EDGE('',*,*,#10926,.F.);
#16540=ORIENTED_EDGE('',*,*,#11330,.F.);
#16541=ORIENTED_EDGE('',*,*,#10856,.F.);
#16542=ORIENTED_EDGE('',*,*,#11326,.T.);
#16543=ORIENTED_EDGE('',*,*,#11331,.F.);
#16544=ORIENTED_EDGE('',*,*,#11332,.T.);
#16545=ORIENTED_EDGE('',*,*,#10859,.T.);
#16546=ORIENTED_EDGE('',*,*,#11329,.T.);
#16547=ORIENTED_EDGE('',*,*,#11333,.F.);
#16548=ORIENTED_EDGE('',*,*,#11334,.T.);
#16549=ORIENTED_EDGE('',*,*,#11331,.T.);
#16550=ORIENTED_EDGE('',*,*,#11328,.T.);
#16551=ORIENTED_EDGE('',*,*,#10923,.F.);
#16552=ORIENTED_EDGE('',*,*,#11335,.T.);
#16553=ORIENTED_EDGE('',*,*,#11333,.T.);
#16554=ORIENTED_EDGE('',*,*,#11336,.F.);
#16555=ORIENTED_EDGE('',*,*,#10862,.F.);
#16556=ORIENTED_EDGE('',*,*,#11337,.T.);
#16557=ORIENTED_EDGE('',*,*,#10920,.F.);
#16558=ORIENTED_EDGE('',*,*,#11338,.F.);
#16559=ORIENTED_EDGE('',*,*,#11339,.F.);
#16560=ORIENTED_EDGE('',*,*,#10861,.F.);
#16561=ORIENTED_EDGE('',*,*,#11340,.T.);
#16562=ORIENTED_EDGE('',*,*,#10921,.F.);
#16563=ORIENTED_EDGE('',*,*,#11337,.F.);
#16564=ORIENTED_EDGE('',*,*,#11332,.F.);
#16565=ORIENTED_EDGE('',*,*,#11334,.F.);
#16566=ORIENTED_EDGE('',*,*,#11335,.F.);
#16567=ORIENTED_EDGE('',*,*,#10922,.F.);
#16568=ORIENTED_EDGE('',*,*,#11340,.F.);
#16569=ORIENTED_EDGE('',*,*,#10860,.F.);
#16570=ORIENTED_EDGE('',*,*,#11336,.T.);
#16571=ORIENTED_EDGE('',*,*,#11341,.F.);
#16572=ORIENTED_EDGE('',*,*,#11342,.T.);
#16573=ORIENTED_EDGE('',*,*,#10863,.T.);
#16574=ORIENTED_EDGE('',*,*,#11339,.T.);
#16575=ORIENTED_EDGE('',*,*,#11343,.F.);
#16576=ORIENTED_EDGE('',*,*,#11344,.T.);
#16577=ORIENTED_EDGE('',*,*,#11341,.T.);
#16578=ORIENTED_EDGE('',*,*,#11338,.T.);
#16579=ORIENTED_EDGE('',*,*,#10919,.F.);
#16580=ORIENTED_EDGE('',*,*,#11345,.T.);
#16581=ORIENTED_EDGE('',*,*,#11343,.T.);
#16582=ORIENTED_EDGE('',*,*,#11346,.F.);
#16583=ORIENTED_EDGE('',*,*,#10866,.F.);
#16584=ORIENTED_EDGE('',*,*,#11347,.T.);
#16585=ORIENTED_EDGE('',*,*,#10916,.F.);
#16586=ORIENTED_EDGE('',*,*,#11348,.F.);
#16587=ORIENTED_EDGE('',*,*,#11349,.F.);
#16588=ORIENTED_EDGE('',*,*,#10865,.F.);
#16589=ORIENTED_EDGE('',*,*,#11350,.T.);
#16590=ORIENTED_EDGE('',*,*,#10917,.F.);
#16591=ORIENTED_EDGE('',*,*,#11347,.F.);
#16592=ORIENTED_EDGE('',*,*,#11342,.F.);
#16593=ORIENTED_EDGE('',*,*,#11344,.F.);
#16594=ORIENTED_EDGE('',*,*,#11345,.F.);
#16595=ORIENTED_EDGE('',*,*,#10918,.F.);
#16596=ORIENTED_EDGE('',*,*,#11350,.F.);
#16597=ORIENTED_EDGE('',*,*,#10864,.F.);
#16598=ORIENTED_EDGE('',*,*,#11346,.T.);
#16599=ORIENTED_EDGE('',*,*,#11351,.F.);
#16600=ORIENTED_EDGE('',*,*,#11352,.T.);
#16601=ORIENTED_EDGE('',*,*,#10867,.T.);
#16602=ORIENTED_EDGE('',*,*,#11349,.T.);
#16603=ORIENTED_EDGE('',*,*,#11353,.F.);
#16604=ORIENTED_EDGE('',*,*,#11354,.T.);
#16605=ORIENTED_EDGE('',*,*,#11351,.T.);
#16606=ORIENTED_EDGE('',*,*,#11348,.T.);
#16607=ORIENTED_EDGE('',*,*,#10915,.F.);
#16608=ORIENTED_EDGE('',*,*,#11355,.T.);
#16609=ORIENTED_EDGE('',*,*,#11353,.T.);
#16610=ORIENTED_EDGE('',*,*,#11356,.F.);
#16611=ORIENTED_EDGE('',*,*,#10870,.F.);
#16612=ORIENTED_EDGE('',*,*,#11357,.T.);
#16613=ORIENTED_EDGE('',*,*,#10912,.F.);
#16614=ORIENTED_EDGE('',*,*,#11358,.F.);
#16615=ORIENTED_EDGE('',*,*,#11359,.F.);
#16616=ORIENTED_EDGE('',*,*,#10869,.F.);
#16617=ORIENTED_EDGE('',*,*,#11360,.T.);
#16618=ORIENTED_EDGE('',*,*,#10913,.F.);
#16619=ORIENTED_EDGE('',*,*,#11357,.F.);
#16620=ORIENTED_EDGE('',*,*,#11352,.F.);
#16621=ORIENTED_EDGE('',*,*,#11354,.F.);
#16622=ORIENTED_EDGE('',*,*,#11355,.F.);
#16623=ORIENTED_EDGE('',*,*,#10914,.F.);
#16624=ORIENTED_EDGE('',*,*,#11360,.F.);
#16625=ORIENTED_EDGE('',*,*,#10868,.F.);
#16626=ORIENTED_EDGE('',*,*,#11356,.T.);
#16627=ORIENTED_EDGE('',*,*,#11361,.F.);
#16628=ORIENTED_EDGE('',*,*,#11362,.T.);
#16629=ORIENTED_EDGE('',*,*,#10871,.T.);
#16630=ORIENTED_EDGE('',*,*,#11359,.T.);
#16631=ORIENTED_EDGE('',*,*,#11363,.F.);
#16632=ORIENTED_EDGE('',*,*,#11364,.T.);
#16633=ORIENTED_EDGE('',*,*,#11361,.T.);
#16634=ORIENTED_EDGE('',*,*,#11358,.T.);
#16635=ORIENTED_EDGE('',*,*,#10911,.F.);
#16636=ORIENTED_EDGE('',*,*,#11365,.T.);
#16637=ORIENTED_EDGE('',*,*,#11363,.T.);
#16638=ORIENTED_EDGE('',*,*,#11366,.F.);
#16639=ORIENTED_EDGE('',*,*,#10874,.F.);
#16640=ORIENTED_EDGE('',*,*,#11367,.T.);
#16641=ORIENTED_EDGE('',*,*,#10908,.F.);
#16642=ORIENTED_EDGE('',*,*,#11368,.F.);
#16643=ORIENTED_EDGE('',*,*,#11369,.F.);
#16644=ORIENTED_EDGE('',*,*,#10873,.F.);
#16645=ORIENTED_EDGE('',*,*,#11370,.T.);
#16646=ORIENTED_EDGE('',*,*,#10909,.F.);
#16647=ORIENTED_EDGE('',*,*,#11367,.F.);
#16648=ORIENTED_EDGE('',*,*,#11362,.F.);
#16649=ORIENTED_EDGE('',*,*,#11364,.F.);
#16650=ORIENTED_EDGE('',*,*,#11365,.F.);
#16651=ORIENTED_EDGE('',*,*,#10910,.F.);
#16652=ORIENTED_EDGE('',*,*,#11370,.F.);
#16653=ORIENTED_EDGE('',*,*,#10872,.F.);
#16654=ORIENTED_EDGE('',*,*,#11366,.T.);
#16655=ORIENTED_EDGE('',*,*,#11371,.F.);
#16656=ORIENTED_EDGE('',*,*,#11372,.T.);
#16657=ORIENTED_EDGE('',*,*,#10875,.T.);
#16658=ORIENTED_EDGE('',*,*,#11369,.T.);
#16659=ORIENTED_EDGE('',*,*,#11373,.F.);
#16660=ORIENTED_EDGE('',*,*,#11374,.T.);
#16661=ORIENTED_EDGE('',*,*,#11371,.T.);
#16662=ORIENTED_EDGE('',*,*,#11368,.T.);
#16663=ORIENTED_EDGE('',*,*,#10907,.F.);
#16664=ORIENTED_EDGE('',*,*,#11375,.T.);
#16665=ORIENTED_EDGE('',*,*,#11373,.T.);
#16666=ORIENTED_EDGE('',*,*,#11376,.F.);
#16667=ORIENTED_EDGE('',*,*,#10878,.F.);
#16668=ORIENTED_EDGE('',*,*,#11377,.T.);
#16669=ORIENTED_EDGE('',*,*,#10904,.F.);
#16670=ORIENTED_EDGE('',*,*,#11378,.F.);
#16671=ORIENTED_EDGE('',*,*,#11379,.F.);
#16672=ORIENTED_EDGE('',*,*,#10877,.F.);
#16673=ORIENTED_EDGE('',*,*,#11380,.T.);
#16674=ORIENTED_EDGE('',*,*,#10905,.F.);
#16675=ORIENTED_EDGE('',*,*,#11377,.F.);
#16676=ORIENTED_EDGE('',*,*,#11372,.F.);
#16677=ORIENTED_EDGE('',*,*,#11374,.F.);
#16678=ORIENTED_EDGE('',*,*,#11375,.F.);
#16679=ORIENTED_EDGE('',*,*,#10906,.F.);
#16680=ORIENTED_EDGE('',*,*,#11380,.F.);
#16681=ORIENTED_EDGE('',*,*,#10876,.F.);
#16682=ORIENTED_EDGE('',*,*,#11138,.T.);
#16683=ORIENTED_EDGE('',*,*,#10879,.T.);
#16684=ORIENTED_EDGE('',*,*,#11376,.T.);
#16685=ORIENTED_EDGE('',*,*,#11381,.F.);
#16686=ORIENTED_EDGE('',*,*,#11139,.T.);
#16687=ORIENTED_EDGE('',*,*,#11381,.T.);
#16688=ORIENTED_EDGE('',*,*,#11379,.T.);
#16689=ORIENTED_EDGE('',*,*,#11382,.F.);
#16690=ORIENTED_EDGE('',*,*,#11140,.T.);
#16691=ORIENTED_EDGE('',*,*,#11382,.T.);
#16692=ORIENTED_EDGE('',*,*,#11378,.T.);
#16693=ORIENTED_EDGE('',*,*,#10903,.F.);
#16694=ORIENTED_EDGE('',*,*,#11127,.T.);
#16695=ORIENTED_EDGE('',*,*,#11383,.F.);
#16696=ORIENTED_EDGE('',*,*,#11131,.T.);
#16697=ORIENTED_EDGE('',*,*,#11047,.T.);
#16698=ORIENTED_EDGE('',*,*,#11126,.T.);
#16699=ORIENTED_EDGE('',*,*,#10729,.F.);
#16700=ORIENTED_EDGE('',*,*,#11129,.T.);
#16701=ORIENTED_EDGE('',*,*,#11383,.T.);
#18637=CYLINDRICAL_SURFACE('',#21303,3.03);
#18638=CYLINDRICAL_SURFACE('',#21388,7.1875);
#18639=CYLINDRICAL_SURFACE('',#21392,10.);
#18640=CYLINDRICAL_SURFACE('',#21394,7.1875);
#18641=CYLINDRICAL_SURFACE('',#21472,10.);
#18642=CYLINDRICAL_SURFACE('',#21475,7.1875);
#18643=CYLINDRICAL_SURFACE('',#21478,10.);
#18644=CYLINDRICAL_SURFACE('',#21479,7.1875);
#18645=CYLINDRICAL_SURFACE('',#21480,10.);
#18646=CYLINDRICAL_SURFACE('',#21483,7.1875);
#18647=CYLINDRICAL_SURFACE('',#21486,10.);
#18648=CYLINDRICAL_SURFACE('',#21487,7.1875);
#18649=CYLINDRICAL_SURFACE('',#21488,10.);
#18650=CYLINDRICAL_SURFACE('',#21491,7.1875);
#18651=CYLINDRICAL_SURFACE('',#21494,10.);
#18652=CYLINDRICAL_SURFACE('',#21495,7.1875);
#18653=CYLINDRICAL_SURFACE('',#21496,10.);
#18654=CYLINDRICAL_SURFACE('',#21499,7.1875);
#18655=CYLINDRICAL_SURFACE('',#21502,10.);
#18656=CYLINDRICAL_SURFACE('',#21503,7.1875);
#18657=CYLINDRICAL_SURFACE('',#21504,10.);
#18658=CYLINDRICAL_SURFACE('',#21507,7.1875);
#18659=CYLINDRICAL_SURFACE('',#21510,10.);
#18660=CYLINDRICAL_SURFACE('',#21511,7.1875);
#18661=CYLINDRICAL_SURFACE('',#21512,10.);
#18662=CYLINDRICAL_SURFACE('',#21515,7.1875);
#18663=CYLINDRICAL_SURFACE('',#21518,10.);
#18664=CYLINDRICAL_SURFACE('',#21519,7.1875);
#18665=CYLINDRICAL_SURFACE('',#21520,14.0625);
#18666=CYLINDRICAL_SURFACE('',#21523,16.875);
#18667=CYLINDRICAL_SURFACE('',#21526,14.0625);
#18668=CYLINDRICAL_SURFACE('',#21529,16.875);
#18669=CYLINDRICAL_SURFACE('',#21532,14.0625);
#18670=CYLINDRICAL_SURFACE('',#21535,16.875);
#18671=CYLINDRICAL_SURFACE('',#21538,14.0625);
#18672=CYLINDRICAL_SURFACE('',#21541,16.875);
#18673=CYLINDRICAL_SURFACE('',#21544,14.0625);
#18674=CYLINDRICAL_SURFACE('',#21547,16.875);
#18675=CYLINDRICAL_SURFACE('',#21550,14.0625);
#18676=CYLINDRICAL_SURFACE('',#21553,16.875);
#18677=CYLINDRICAL_SURFACE('',#21556,14.0625);
#18678=CYLINDRICAL_SURFACE('',#21559,16.875);
#18679=CYLINDRICAL_SURFACE('',#21562,14.0625);
#18680=CYLINDRICAL_SURFACE('',#21565,16.875);
#18681=CYLINDRICAL_SURFACE('',#21568,14.0625);
#18682=CYLINDRICAL_SURFACE('',#21571,16.875);
#18683=CYLINDRICAL_SURFACE('',#21574,14.0625);
#18684=CYLINDRICAL_SURFACE('',#21577,16.875);
#18685=CYLINDRICAL_SURFACE('',#21580,14.0625);
#18686=CYLINDRICAL_SURFACE('',#21583,16.875);
#18687=CYLINDRICAL_SURFACE('',#21586,14.0625);
#18688=CYLINDRICAL_SURFACE('',#21589,16.875);
#18689=CYLINDRICAL_SURFACE('',#21592,14.0625);
#18690=CYLINDRICAL_SURFACE('',#21595,16.875);
#18691=CYLINDRICAL_SURFACE('',#21598,14.0625);
#18692=CYLINDRICAL_SURFACE('',#21601,16.875);
#18693=CYLINDRICAL_SURFACE('',#21604,14.0625);
#18694=CYLINDRICAL_SURFACE('',#21607,16.875);
#18695=CYLINDRICAL_SURFACE('',#21610,14.0625);
#18696=CYLINDRICAL_SURFACE('',#21613,16.875);
#18697=CYLINDRICAL_SURFACE('',#21616,14.0625);
#18698=CYLINDRICAL_SURFACE('',#21619,16.875);
#18699=CYLINDRICAL_SURFACE('',#21622,14.0625);
#18700=CYLINDRICAL_SURFACE('',#21625,16.875);
#18701=CYLINDRICAL_SURFACE('',#21628,14.0625);
#18702=CYLINDRICAL_SURFACE('',#21631,16.875);
#18703=CYLINDRICAL_SURFACE('',#21634,14.0625);
#18704=CYLINDRICAL_SURFACE('',#21637,16.875);
#18705=CYLINDRICAL_SURFACE('',#21640,14.0625);
#18706=CYLINDRICAL_SURFACE('',#21643,16.875);
#18707=CYLINDRICAL_SURFACE('',#21646,14.0625);
#18708=CYLINDRICAL_SURFACE('',#21649,16.875);
#18709=CYLINDRICAL_SURFACE('',#21652,14.0625);
#18710=CYLINDRICAL_SURFACE('',#21655,16.875);
#18711=CYLINDRICAL_SURFACE('',#21658,14.0625);
#18712=CYLINDRICAL_SURFACE('',#21661,16.875);
#18713=CYLINDRICAL_SURFACE('',#21664,14.0625);
#18714=CYLINDRICAL_SURFACE('',#21667,16.875);
#18715=CYLINDRICAL_SURFACE('',#21670,10.);
#19448=ADVANCED_FACE('',(#1752),#423,.F.);
#19449=ADVANCED_FACE('',(#1753),#18637,.F.);
#19450=ADVANCED_FACE('',(#1754,#1115),#971,.T.);
#19451=ADVANCED_FACE('',(#1755),#424,.F.);
#19452=ADVANCED_FACE('',(#1756,#1116),#972,.T.);
#19453=ADVANCED_FACE('',(#1757),#530,.F.);
#19454=ADVANCED_FACE('',(#1758),#18638,.T.);
#19455=ADVANCED_FACE('',(#1759),#531,.F.);
#19456=ADVANCED_FACE('',(#1760),#425,.T.);
#19457=ADVANCED_FACE('',(#1761),#18639,.T.);
#19458=ADVANCED_FACE('',(#1762),#532,.F.);
#19459=ADVANCED_FACE('',(#1763),#18640,.T.);
#19460=ADVANCED_FACE('',(#1764),#533,.F.);
#19461=ADVANCED_FACE('',(#1765,#1117),#973,.T.);
#19462=ADVANCED_FACE('',(#1766),#18641,.T.);
#19463=ADVANCED_FACE('',(#1767),#426,.T.);
#19464=ADVANCED_FACE('',(#1768),#534,.F.);
#19465=ADVANCED_FACE('',(#1769),#18642,.T.);
#19466=ADVANCED_FACE('',(#1770),#535,.F.);
#19467=ADVANCED_FACE('',(#1771),#427,.T.);
#19468=ADVANCED_FACE('',(#1772),#18643,.T.);
#19469=ADVANCED_FACE('',(#1773),#536,.F.);
#19470=ADVANCED_FACE('',(#1774),#18644,.T.);
#19471=ADVANCED_FACE('',(#1775),#537,.F.);
#19472=ADVANCED_FACE('',(#1776),#18645,.T.);
#19473=ADVANCED_FACE('',(#1777),#428,.T.);
#19474=ADVANCED_FACE('',(#1778),#538,.F.);
#19475=ADVANCED_FACE('',(#1779),#18646,.T.);
#19476=ADVANCED_FACE('',(#1780),#539,.F.);
#19477=ADVANCED_FACE('',(#1781),#429,.T.);
#19478=ADVANCED_FACE('',(#1782),#18647,.T.);
#19479=ADVANCED_FACE('',(#1783),#540,.F.);
#19480=ADVANCED_FACE('',(#1784),#18648,.T.);
#19481=ADVANCED_FACE('',(#1785),#541,.F.);
#19482=ADVANCED_FACE('',(#1786),#18649,.T.);
#19483=ADVANCED_FACE('',(#1787),#430,.T.);
#19484=ADVANCED_FACE('',(#1788),#542,.F.);
#19485=ADVANCED_FACE('',(#1789),#18650,.T.);
#19486=ADVANCED_FACE('',(#1790),#543,.F.);
#19487=ADVANCED_FACE('',(#1791),#431,.T.);
#19488=ADVANCED_FACE('',(#1792),#18651,.T.);
#19489=ADVANCED_FACE('',(#1793),#544,.F.);
#19490=ADVANCED_FACE('',(#1794),#18652,.T.);
#19491=ADVANCED_FACE('',(#1795),#545,.F.);
#19492=ADVANCED_FACE('',(#1796),#18653,.T.);
#19493=ADVANCED_FACE('',(#1797),#432,.T.);
#19494=ADVANCED_FACE('',(#1798),#546,.F.);
#19495=ADVANCED_FACE('',(#1799),#18654,.T.);
#19496=ADVANCED_FACE('',(#1800),#547,.F.);
#19497=ADVANCED_FACE('',(#1801),#433,.T.);
#19498=ADVANCED_FACE('',(#1802),#18655,.T.);
#19499=ADVANCED_FACE('',(#1803),#548,.F.);
#19500=ADVANCED_FACE('',(#1804),#18656,.T.);
#19501=ADVANCED_FACE('',(#1805),#549,.F.);
#19502=ADVANCED_FACE('',(#1806),#18657,.T.);
#19503=ADVANCED_FACE('',(#1807),#434,.T.);
#19504=ADVANCED_FACE('',(#1808),#550,.F.);
#19505=ADVANCED_FACE('',(#1809),#18658,.T.);
#19506=ADVANCED_FACE('',(#1810),#551,.F.);
#19507=ADVANCED_FACE('',(#1811),#435,.T.);
#19508=ADVANCED_FACE('',(#1812),#18659,.T.);
#19509=ADVANCED_FACE('',(#1813),#552,.F.);
#19510=ADVANCED_FACE('',(#1814),#18660,.T.);
#19511=ADVANCED_FACE('',(#1815),#553,.F.);
#19512=ADVANCED_FACE('',(#1816),#18661,.T.);
#19513=ADVANCED_FACE('',(#1817),#436,.T.);
#19514=ADVANCED_FACE('',(#1818),#554,.F.);
#19515=ADVANCED_FACE('',(#1819),#18662,.T.);
#19516=ADVANCED_FACE('',(#1820),#555,.F.);
#19517=ADVANCED_FACE('',(#1821),#437,.T.);
#19518=ADVANCED_FACE('',(#1822),#18663,.T.);
#19519=ADVANCED_FACE('',(#1823),#556,.F.);
#19520=ADVANCED_FACE('',(#1824),#18664,.T.);
#19521=ADVANCED_FACE('',(#1825),#557,.F.);
#19522=ADVANCED_FACE('',(#1826),#558,.F.);
#19523=ADVANCED_FACE('',(#1827),#18665,.T.);
#19524=ADVANCED_FACE('',(#1828),#559,.F.);
#19525=ADVANCED_FACE('',(#1829),#438,.T.);
#19526=ADVANCED_FACE('',(#1830),#18666,.T.);
#19527=ADVANCED_FACE('',(#1831),#439,.T.);
#19528=ADVANCED_FACE('',(#1832),#560,.F.);
#19529=ADVANCED_FACE('',(#1833),#18667,.T.);
#19530=ADVANCED_FACE('',(#1834),#561,.F.);
#19531=ADVANCED_FACE('',(#1835),#440,.T.);
#19532=ADVANCED_FACE('',(#1836),#18668,.T.);
#19533=ADVANCED_FACE('',(#1837),#441,.T.);
#19534=ADVANCED_FACE('',(#1838),#562,.F.);
#19535=ADVANCED_FACE('',(#1839),#18669,.T.);
#19536=ADVANCED_FACE('',(#1840),#563,.F.);
#19537=ADVANCED_FACE('',(#1841),#442,.T.);
#19538=ADVANCED_FACE('',(#1842),#18670,.T.);
#19539=ADVANCED_FACE('',(#1843),#443,.T.);
#19540=ADVANCED_FACE('',(#1844),#564,.F.);
#19541=ADVANCED_FACE('',(#1845),#18671,.T.);
#19542=ADVANCED_FACE('',(#1846),#565,.F.);
#19543=ADVANCED_FACE('',(#1847),#444,.T.);
#19544=ADVANCED_FACE('',(#1848),#18672,.T.);
#19545=ADVANCED_FACE('',(#1849),#445,.T.);
#19546=ADVANCED_FACE('',(#1850),#566,.F.);
#19547=ADVANCED_FACE('',(#1851),#18673,.T.);
#19548=ADVANCED_FACE('',(#1852),#567,.F.);
#19549=ADVANCED_FACE('',(#1853),#446,.T.);
#19550=ADVANCED_FACE('',(#1854),#18674,.T.);
#19551=ADVANCED_FACE('',(#1855),#447,.T.);
#19552=ADVANCED_FACE('',(#1856),#568,.F.);
#19553=ADVANCED_FACE('',(#1857),#18675,.T.);
#19554=ADVANCED_FACE('',(#1858),#569,.F.);
#19555=ADVANCED_FACE('',(#1859),#448,.T.);
#19556=ADVANCED_FACE('',(#1860),#18676,.T.);
#19557=ADVANCED_FACE('',(#1861),#449,.T.);
#19558=ADVANCED_FACE('',(#1862),#570,.F.);
#19559=ADVANCED_FACE('',(#1863),#18677,.T.);
#19560=ADVANCED_FACE('',(#1864),#571,.F.);
#19561=ADVANCED_FACE('',(#1865),#450,.T.);
#19562=ADVANCED_FACE('',(#1866),#18678,.T.);
#19563=ADVANCED_FACE('',(#1867),#451,.T.);
#19564=ADVANCED_FACE('',(#1868),#572,.F.);
#19565=ADVANCED_FACE('',(#1869),#18679,.T.);
#19566=ADVANCED_FACE('',(#1870),#573,.F.);
#19567=ADVANCED_FACE('',(#1871),#452,.T.);
#19568=ADVANCED_FACE('',(#1872),#18680,.T.);
#19569=ADVANCED_FACE('',(#1873),#453,.T.);
#19570=ADVANCED_FACE('',(#1874),#574,.F.);
#19571=ADVANCED_FACE('',(#1875),#18681,.T.);
#19572=ADVANCED_FACE('',(#1876),#575,.F.);
#19573=ADVANCED_FACE('',(#1877),#454,.T.);
#19574=ADVANCED_FACE('',(#1878),#18682,.T.);
#19575=ADVANCED_FACE('',(#1879),#455,.T.);
#19576=ADVANCED_FACE('',(#1880),#576,.F.);
#19577=ADVANCED_FACE('',(#1881),#18683,.T.);
#19578=ADVANCED_FACE('',(#1882),#577,.F.);
#19579=ADVANCED_FACE('',(#1883),#456,.T.);
#19580=ADVANCED_FACE('',(#1884),#18684,.T.);
#19581=ADVANCED_FACE('',(#1885),#457,.T.);
#19582=ADVANCED_FACE('',(#1886),#578,.F.);
#19583=ADVANCED_FACE('',(#1887),#18685,.T.);
#19584=ADVANCED_FACE('',(#1888),#579,.F.);
#19585=ADVANCED_FACE('',(#1889),#458,.T.);
#19586=ADVANCED_FACE('',(#1890),#18686,.T.);
#19587=ADVANCED_FACE('',(#1891),#459,.T.);
#19588=ADVANCED_FACE('',(#1892),#580,.F.);
#19589=ADVANCED_FACE('',(#1893),#18687,.T.);
#19590=ADVANCED_FACE('',(#1894),#581,.F.);
#19591=ADVANCED_FACE('',(#1895),#460,.T.);
#19592=ADVANCED_FACE('',(#1896),#18688,.T.);
#19593=ADVANCED_FACE('',(#1897),#461,.T.);
#19594=ADVANCED_FACE('',(#1898),#582,.F.);
#19595=ADVANCED_FACE('',(#1899),#18689,.T.);
#19596=ADVANCED_FACE('',(#1900),#583,.F.);
#19597=ADVANCED_FACE('',(#1901),#462,.T.);
#19598=ADVANCED_FACE('',(#1902),#18690,.T.);
#19599=ADVANCED_FACE('',(#1903),#463,.T.);
#19600=ADVANCED_FACE('',(#1904),#584,.F.);
#19601=ADVANCED_FACE('',(#1905),#18691,.T.);
#19602=ADVANCED_FACE('',(#1906),#585,.F.);
#19603=ADVANCED_FACE('',(#1907),#464,.T.);
#19604=ADVANCED_FACE('',(#1908),#18692,.T.);
#19605=ADVANCED_FACE('',(#1909),#465,.T.);
#19606=ADVANCED_FACE('',(#1910),#586,.F.);
#19607=ADVANCED_FACE('',(#1911),#18693,.T.);
#19608=ADVANCED_FACE('',(#1912),#587,.F.);
#19609=ADVANCED_FACE('',(#1913),#466,.T.);
#19610=ADVANCED_FACE('',(#1914),#18694,.T.);
#19611=ADVANCED_FACE('',(#1915),#467,.T.);
#19612=ADVANCED_FACE('',(#1916),#588,.F.);
#19613=ADVANCED_FACE('',(#1917),#18695,.T.);
#19614=ADVANCED_FACE('',(#1918),#589,.F.);
#19615=ADVANCED_FACE('',(#1919),#468,.T.);
#19616=ADVANCED_FACE('',(#1920),#18696,.T.);
#19617=ADVANCED_FACE('',(#1921),#469,.T.);
#19618=ADVANCED_FACE('',(#1922),#590,.F.);
#19619=ADVANCED_FACE('',(#1923),#18697,.T.);
#19620=ADVANCED_FACE('',(#1924),#591,.F.);
#19621=ADVANCED_FACE('',(#1925),#470,.T.);
#19622=ADVANCED_FACE('',(#1926),#18698,.T.);
#19623=ADVANCED_FACE('',(#1927),#471,.T.);
#19624=ADVANCED_FACE('',(#1928),#592,.F.);
#19625=ADVANCED_FACE('',(#1929),#18699,.T.);
#19626=ADVANCED_FACE('',(#1930),#593,.F.);
#19627=ADVANCED_FACE('',(#1931),#472,.T.);
#19628=ADVANCED_FACE('',(#1932),#18700,.T.);
#19629=ADVANCED_FACE('',(#1933),#473,.T.);
#19630=ADVANCED_FACE('',(#1934),#594,.F.);
#19631=ADVANCED_FACE('',(#1935),#18701,.T.);
#19632=ADVANCED_FACE('',(#1936),#595,.F.);
#19633=ADVANCED_FACE('',(#1937),#474,.T.);
#19634=ADVANCED_FACE('',(#1938),#18702,.T.);
#19635=ADVANCED_FACE('',(#1939),#475,.T.);
#19636=ADVANCED_FACE('',(#1940),#596,.F.);
#19637=ADVANCED_FACE('',(#1941),#18703,.T.);
#19638=ADVANCED_FACE('',(#1942),#597,.F.);
#19639=ADVANCED_FACE('',(#1943),#476,.T.);
#19640=ADVANCED_FACE('',(#1944),#18704,.T.);
#19641=ADVANCED_FACE('',(#1945),#477,.T.);
#19642=ADVANCED_FACE('',(#1946),#598,.F.);
#19643=ADVANCED_FACE('',(#1947),#18705,.T.);
#19644=ADVANCED_FACE('',(#1948),#599,.F.);
#19645=ADVANCED_FACE('',(#1949),#478,.T.);
#19646=ADVANCED_FACE('',(#1950),#18706,.T.);
#19647=ADVANCED_FACE('',(#1951),#479,.T.);
#19648=ADVANCED_FACE('',(#1952),#600,.F.);
#19649=ADVANCED_FACE('',(#1953),#18707,.T.);
#19650=ADVANCED_FACE('',(#1954),#601,.F.);
#19651=ADVANCED_FACE('',(#1955),#480,.T.);
#19652=ADVANCED_FACE('',(#1956),#18708,.T.);
#19653=ADVANCED_FACE('',(#1957),#481,.T.);
#19654=ADVANCED_FACE('',(#1958),#602,.F.);
#19655=ADVANCED_FACE('',(#1959),#18709,.T.);
#19656=ADVANCED_FACE('',(#1960),#603,.F.);
#19657=ADVANCED_FACE('',(#1961),#482,.T.);
#19658=ADVANCED_FACE('',(#1962),#18710,.T.);
#19659=ADVANCED_FACE('',(#1963),#483,.T.);
#19660=ADVANCED_FACE('',(#1964),#604,.F.);
#19661=ADVANCED_FACE('',(#1965),#18711,.T.);
#19662=ADVANCED_FACE('',(#1966),#605,.F.);
#19663=ADVANCED_FACE('',(#1967),#484,.T.);
#19664=ADVANCED_FACE('',(#1968),#18712,.T.);
#19665=ADVANCED_FACE('',(#1969),#485,.T.);
#19666=ADVANCED_FACE('',(#1970),#606,.F.);
#19667=ADVANCED_FACE('',(#1971),#18713,.T.);
#19668=ADVANCED_FACE('',(#1972),#607,.F.);
#19669=ADVANCED_FACE('',(#1973),#486,.T.);
#19670=ADVANCED_FACE('',(#1974),#18714,.T.);
#19671=ADVANCED_FACE('',(#1975),#487,.T.);
#19672=ADVANCED_FACE('',(#1976),#18715,.T.);
#19673=ADVANCED_FACE('',(#1977),#488,.T.);
#20010=CLOSED_SHELL('',(#19448,#19449,#19450,#19451,#19452,#19453,#19454,
#19455,#19456,#19457,#19458,#19459,#19460,#19461,#19462,#19463,#19464,#19465,
#19466,#19467,#19468,#19469,#19470,#19471,#19472,#19473,#19474,#19475,#19476,
#19477,#19478,#19479,#19480,#19481,#19482,#19483,#19484,#19485,#19486,#19487,
#19488,#19489,#19490,#19491,#19492,#19493,#19494,#19495,#19496,#19497,#19498,
#19499,#19500,#19501,#19502,#19503,#19504,#19505,#19506,#19507,#19508,#19509,
#19510,#19511,#19512,#19513,#19514,#19515,#19516,#19517,#19518,#19519,#19520,
#19521,#19522,#19523,#19524,#19525,#19526,#19527,#19528,#19529,#19530,#19531,
#19532,#19533,#19534,#19535,#19536,#19537,#19538,#19539,#19540,#19541,#19542,
#19543,#19544,#19545,#19546,#19547,#19548,#19549,#19550,#19551,#19552,#19553,
#19554,#19555,#19556,#19557,#19558,#19559,#19560,#19561,#19562,#19563,#19564,
#19565,#19566,#19567,#19568,#19569,#19570,#19571,#19572,#19573,#19574,#19575,
#19576,#19577,#19578,#19579,#19580,#19581,#19582,#19583,#19584,#19585,#19586,
#19587,#19588,#19589,#19590,#19591,#19592,#19593,#19594,#19595,#19596,#19597,
#19598,#19599,#19600,#19601,#19602,#19603,#19604,#19605,#19606,#19607,#19608,
#19609,#19610,#19611,#19612,#19613,#19614,#19615,#19616,#19617,#19618,#19619,
#19620,#19621,#19622,#19623,#19624,#19625,#19626,#19627,#19628,#19629,#19630,
#19631,#19632,#19633,#19634,#19635,#19636,#19637,#19638,#19639,#19640,#19641,
#19642,#19643,#19644,#19645,#19646,#19647,#19648,#19649,#19650,#19651,#19652,
#19653,#19654,#19655,#19656,#19657,#19658,#19659,#19660,#19661,#19662,#19663,
#19664,#19665,#19666,#19667,#19668,#19669,#19670,#19671,#19672,#19673));
#21298=AXIS2_PLACEMENT_3D('',#49227,#25201,#25202);
#21299=AXIS2_PLACEMENT_3D('',#49228,#25203,#25204);
#21300=AXIS2_PLACEMENT_3D('',#49231,#25205,#25206);
#21301=AXIS2_PLACEMENT_3D('',#49232,#25207,#25208);
#21302=AXIS2_PLACEMENT_3D('',#49235,#25210,#25211);
#21303=AXIS2_PLACEMENT_3D('',#49236,#25212,#25213);
#21304=AXIS2_PLACEMENT_3D('',#49240,#25215,#25216);
#21305=AXIS2_PLACEMENT_3D('',#49241,#25217,#25218);
#21306=AXIS2_PLACEMENT_3D('',#49242,#25219,#25220);
#21307=AXIS2_PLACEMENT_3D('',#49271,#25221,#25222);
#21308=AXIS2_PLACEMENT_3D('',#49303,#25223,#25224);
#21309=AXIS2_PLACEMENT_3D('',#49331,#25225,#25226);
#21310=AXIS2_PLACEMENT_3D('',#49363,#25227,#25228);
#21311=AXIS2_PLACEMENT_3D('',#49391,#25229,#25230);
#21312=AXIS2_PLACEMENT_3D('',#49423,#25231,#25232);
#21313=AXIS2_PLACEMENT_3D('',#49451,#25233,#25234);
#21314=AXIS2_PLACEMENT_3D('',#49483,#25235,#25236);
#21315=AXIS2_PLACEMENT_3D('',#49511,#25237,#25238);
#21316=AXIS2_PLACEMENT_3D('',#49543,#25239,#25240);
#21317=AXIS2_PLACEMENT_3D('',#49571,#25241,#25242);
#21318=AXIS2_PLACEMENT_3D('',#49603,#25243,#25244);
#21319=AXIS2_PLACEMENT_3D('',#49631,#25245,#25246);
#21320=AXIS2_PLACEMENT_3D('',#49663,#25247,#25248);
#21321=AXIS2_PLACEMENT_3D('',#49691,#25249,#25250);
#21322=AXIS2_PLACEMENT_3D('',#49723,#25251,#25252);
#21323=AXIS2_PLACEMENT_3D('',#49751,#25253,#25254);
#21324=AXIS2_PLACEMENT_3D('',#49783,#25255,#25256);
#21325=AXIS2_PLACEMENT_3D('',#49811,#25257,#25258);
#21326=AXIS2_PLACEMENT_3D('',#49843,#25259,#25260);
#21327=AXIS2_PLACEMENT_3D('',#49871,#25261,#25262);
#21328=AXIS2_PLACEMENT_3D('',#49903,#25263,#25264);
#21329=AXIS2_PLACEMENT_3D('',#49931,#25265,#25266);
#21330=AXIS2_PLACEMENT_3D('',#49963,#25267,#25268);
#21331=AXIS2_PLACEMENT_3D('',#49991,#25269,#25270);
#21332=AXIS2_PLACEMENT_3D('',#50023,#25271,#25272);
#21333=AXIS2_PLACEMENT_3D('',#50051,#25273,#25274);
#21334=AXIS2_PLACEMENT_3D('',#50082,#25275,#25276);
#21335=AXIS2_PLACEMENT_3D('',#50083,#25277,#25278);
#21336=AXIS2_PLACEMENT_3D('',#50085,#25279,#25280);
#21337=AXIS2_PLACEMENT_3D('',#50087,#25282,#25283);
#21338=AXIS2_PLACEMENT_3D('',#50120,#25284,#25285);
#21339=AXIS2_PLACEMENT_3D('',#50149,#25286,#25287);
#21340=AXIS2_PLACEMENT_3D('',#50181,#25288,#25289);
#21341=AXIS2_PLACEMENT_3D('',#50210,#25290,#25291);
#21342=AXIS2_PLACEMENT_3D('',#50242,#25292,#25293);
#21343=AXIS2_PLACEMENT_3D('',#50271,#25294,#25295);
#21344=AXIS2_PLACEMENT_3D('',#50303,#25296,#25297);
#21345=AXIS2_PLACEMENT_3D('',#50332,#25298,#25299);
#21346=AXIS2_PLACEMENT_3D('',#50364,#25300,#25301);
#21347=AXIS2_PLACEMENT_3D('',#50393,#25302,#25303);
#21348=AXIS2_PLACEMENT_3D('',#50425,#25304,#25305);
#21349=AXIS2_PLACEMENT_3D('',#50454,#25306,#25307);
#21350=AXIS2_PLACEMENT_3D('',#50486,#25308,#25309);
#21351=AXIS2_PLACEMENT_3D('',#50515,#25310,#25311);
#21352=AXIS2_PLACEMENT_3D('',#50547,#25312,#25313);
#21353=AXIS2_PLACEMENT_3D('',#50576,#25314,#25315);
#21354=AXIS2_PLACEMENT_3D('',#50608,#25316,#25317);
#21355=AXIS2_PLACEMENT_3D('',#50637,#25318,#25319);
#21356=AXIS2_PLACEMENT_3D('',#50669,#25320,#25321);
#21357=AXIS2_PLACEMENT_3D('',#50698,#25322,#25323);
#21358=AXIS2_PLACEMENT_3D('',#50730,#25324,#25325);
#21359=AXIS2_PLACEMENT_3D('',#50759,#25326,#25327);
#21360=AXIS2_PLACEMENT_3D('',#50791,#25328,#25329);
#21361=AXIS2_PLACEMENT_3D('',#50820,#25330,#25331);
#21362=AXIS2_PLACEMENT_3D('',#50852,#25332,#25333);
#21363=AXIS2_PLACEMENT_3D('',#50881,#25334,#25335);
#21364=AXIS2_PLACEMENT_3D('',#50913,#25336,#25337);
#21365=AXIS2_PLACEMENT_3D('',#50942,#25338,#25339);
#21366=AXIS2_PLACEMENT_3D('',#50974,#25340,#25341);
#21367=AXIS2_PLACEMENT_3D('',#51003,#25342,#25343);
#21368=AXIS2_PLACEMENT_3D('',#51035,#25344,#25345);
#21369=AXIS2_PLACEMENT_3D('',#51064,#25346,#25347);
#21370=AXIS2_PLACEMENT_3D('',#51096,#25348,#25349);
#21371=AXIS2_PLACEMENT_3D('',#51125,#25350,#25351);
#21372=AXIS2_PLACEMENT_3D('',#51157,#25352,#25353);
#21373=AXIS2_PLACEMENT_3D('',#51186,#25354,#25355);
#21374=AXIS2_PLACEMENT_3D('',#51218,#25356,#25357);
#21375=AXIS2_PLACEMENT_3D('',#51247,#25358,#25359);
#21376=AXIS2_PLACEMENT_3D('',#51279,#25360,#25361);
#21377=AXIS2_PLACEMENT_3D('',#51308,#25362,#25363);
#21378=AXIS2_PLACEMENT_3D('',#51340,#25364,#25365);
#21379=AXIS2_PLACEMENT_3D('',#51369,#25366,#25367);
#21380=AXIS2_PLACEMENT_3D('',#51401,#25368,#25369);
#21381=AXIS2_PLACEMENT_3D('',#51430,#25370,#25371);
#21382=AXIS2_PLACEMENT_3D('',#51462,#25372,#25373);
#21383=AXIS2_PLACEMENT_3D('',#51491,#25374,#25375);
#21384=AXIS2_PLACEMENT_3D('',#51523,#25376,#25377);
#21385=AXIS2_PLACEMENT_3D('',#51552,#25378,#25379);
#21386=AXIS2_PLACEMENT_3D('',#51584,#25380,#25381);
#21387=AXIS2_PLACEMENT_3D('',#51612,#25382,#25383);
#21388=AXIS2_PLACEMENT_3D('',#51744,#25385,#25386);
#21389=AXIS2_PLACEMENT_3D('',#51746,#25387,#25388);
#21390=AXIS2_PLACEMENT_3D('',#51871,#25390,#25391);
#21391=AXIS2_PLACEMENT_3D('',#51873,#25392,#25393);
#21392=AXIS2_PLACEMENT_3D('',#51880,#25394,#25395);
#21393=AXIS2_PLACEMENT_3D('',#51882,#25396,#25397);
#21394=AXIS2_PLACEMENT_3D('',#52014,#25399,#25400);
#21395=AXIS2_PLACEMENT_3D('',#52016,#25401,#25402);
#21396=AXIS2_PLACEMENT_3D('',#52144,#25404,#25405);
#21397=AXIS2_PLACEMENT_3D('',#52177,#25406,#25407);
#21398=AXIS2_PLACEMENT_3D('',#52206,#25408,#25409);
#21399=AXIS2_PLACEMENT_3D('',#52238,#25410,#25411);
#21400=AXIS2_PLACEMENT_3D('',#52267,#25412,#25413);
#21401=AXIS2_PLACEMENT_3D('',#52299,#25414,#25415);
#21402=AXIS2_PLACEMENT_3D('',#52328,#25416,#25417);
#21403=AXIS2_PLACEMENT_3D('',#52360,#25418,#25419);
#21404=AXIS2_PLACEMENT_3D('',#52389,#25420,#25421);
#21405=AXIS2_PLACEMENT_3D('',#52421,#25422,#25423);
#21406=AXIS2_PLACEMENT_3D('',#52450,#25424,#25425);
#21407=AXIS2_PLACEMENT_3D('',#52482,#25426,#25427);
#21408=AXIS2_PLACEMENT_3D('',#52511,#25428,#25429);
#21409=AXIS2_PLACEMENT_3D('',#52543,#25430,#25431);
#21410=AXIS2_PLACEMENT_3D('',#52572,#25432,#25433);
#21411=AXIS2_PLACEMENT_3D('',#52604,#25434,#25435);
#21412=AXIS2_PLACEMENT_3D('',#52633,#25436,#25437);
#21413=AXIS2_PLACEMENT_3D('',#52665,#25438,#25439);
#21414=AXIS2_PLACEMENT_3D('',#52694,#25440,#25441);
#21415=AXIS2_PLACEMENT_3D('',#52726,#25442,#25443);
#21416=AXIS2_PLACEMENT_3D('',#52755,#25444,#25445);
#21417=AXIS2_PLACEMENT_3D('',#52787,#25446,#25447);
#21418=AXIS2_PLACEMENT_3D('',#52816,#25448,#25449);
#21419=AXIS2_PLACEMENT_3D('',#52848,#25450,#25451);
#21420=AXIS2_PLACEMENT_3D('',#52877,#25452,#25453);
#21421=AXIS2_PLACEMENT_3D('',#52909,#25454,#25455);
#21422=AXIS2_PLACEMENT_3D('',#52938,#25456,#25457);
#21423=AXIS2_PLACEMENT_3D('',#52970,#25458,#25459);
#21424=AXIS2_PLACEMENT_3D('',#52999,#25460,#25461);
#21425=AXIS2_PLACEMENT_3D('',#53031,#25462,#25463);
#21426=AXIS2_PLACEMENT_3D('',#53060,#25464,#25465);
#21427=AXIS2_PLACEMENT_3D('',#53092,#25466,#25467);
#21428=AXIS2_PLACEMENT_3D('',#53121,#25468,#25469);
#21429=AXIS2_PLACEMENT_3D('',#53153,#25470,#25471);
#21430=AXIS2_PLACEMENT_3D('',#53182,#25472,#25473);
#21431=AXIS2_PLACEMENT_3D('',#53214,#25474,#25475);
#21432=AXIS2_PLACEMENT_3D('',#53243,#25476,#25477);
#21433=AXIS2_PLACEMENT_3D('',#53275,#25478,#25479);
#21434=AXIS2_PLACEMENT_3D('',#53304,#25480,#25481);
#21435=AXIS2_PLACEMENT_3D('',#53336,#25482,#25483);
#21436=AXIS2_PLACEMENT_3D('',#53365,#25484,#25485);
#21437=AXIS2_PLACEMENT_3D('',#53397,#25486,#25487);
#21438=AXIS2_PLACEMENT_3D('',#53426,#25488,#25489);
#21439=AXIS2_PLACEMENT_3D('',#53458,#25490,#25491);
#21440=AXIS2_PLACEMENT_3D('',#53487,#25492,#25493);
#21441=AXIS2_PLACEMENT_3D('',#53519,#25494,#25495);
#21442=AXIS2_PLACEMENT_3D('',#53548,#25496,#25497);
#21443=AXIS2_PLACEMENT_3D('',#53580,#25498,#25499);
#21444=AXIS2_PLACEMENT_3D('',#53609,#25500,#25501);
#21445=AXIS2_PLACEMENT_3D('',#53641,#25502,#25503);
#21446=AXIS2_PLACEMENT_3D('',#53669,#25504,#25505);
#21447=AXIS2_PLACEMENT_3D('',#53670,#25506,#25507);
#21448=AXIS2_PLACEMENT_3D('',#53672,#25508,#25509);
#21449=AXIS2_PLACEMENT_3D('',#53709,#25510,#25511);
#21450=AXIS2_PLACEMENT_3D('',#53741,#25512,#25513);
#21451=AXIS2_PLACEMENT_3D('',#53778,#25514,#25515);
#21452=AXIS2_PLACEMENT_3D('',#53810,#25516,#25517);
#21453=AXIS2_PLACEMENT_3D('',#53847,#25518,#25519);
#21454=AXIS2_PLACEMENT_3D('',#53879,#25520,#25521);
#21455=AXIS2_PLACEMENT_3D('',#53916,#25522,#25523);
#21456=AXIS2_PLACEMENT_3D('',#53948,#25524,#25525);
#21457=AXIS2_PLACEMENT_3D('',#53985,#25526,#25527);
#21458=AXIS2_PLACEMENT_3D('',#54017,#25528,#25529);
#21459=AXIS2_PLACEMENT_3D('',#54054,#25530,#25531);
#21460=AXIS2_PLACEMENT_3D('',#54086,#25532,#25533);
#21461=AXIS2_PLACEMENT_3D('',#54123,#25534,#25535);
#21462=AXIS2_PLACEMENT_3D('',#54155,#25536,#25537);
#21463=AXIS2_PLACEMENT_3D('',#54192,#25538,#25539);
#21464=AXIS2_PLACEMENT_3D('',#54224,#25540,#25541);
#21465=AXIS2_PLACEMENT_3D('',#54261,#25542,#25543);
#21466=AXIS2_PLACEMENT_3D('',#54293,#25544,#25545);
#21467=AXIS2_PLACEMENT_3D('',#54330,#25546,#25547);
#21468=AXIS2_PLACEMENT_3D('',#54362,#25548,#25549);
#21469=AXIS2_PLACEMENT_3D('',#54399,#25550,#25551);
#21470=AXIS2_PLACEMENT_3D('',#54431,#25552,#25553);
#21471=AXIS2_PLACEMENT_3D('',#54468,#25554,#25555);
#21472=AXIS2_PLACEMENT_3D('',#54498,#25556,#25557);
#21473=AXIS2_PLACEMENT_3D('',#54500,#25558,#25559);
#21474=AXIS2_PLACEMENT_3D('',#54507,#25560,#25561);
#21475=AXIS2_PLACEMENT_3D('',#54593,#25563,#25564);
#21476=AXIS2_PLACEMENT_3D('',#54688,#25566,#25567);
#21477=AXIS2_PLACEMENT_3D('',#54689,#25568,#25569);
#21478=AXIS2_PLACEMENT_3D('',#54690,#25570,#25571);
#21479=AXIS2_PLACEMENT_3D('',#54785,#25573,#25574);
#21480=AXIS2_PLACEMENT_3D('',#54878,#25576,#25577);
#21481=AXIS2_PLACEMENT_3D('',#54880,#25578,#25579);
#21482=AXIS2_PLACEMENT_3D('',#54887,#25580,#25581);
#21483=AXIS2_PLACEMENT_3D('',#54979,#25583,#25584);
#21484=AXIS2_PLACEMENT_3D('',#55074,#25586,#25587);
#21485=AXIS2_PLACEMENT_3D('',#55075,#25588,#25589);
#21486=AXIS2_PLACEMENT_3D('',#55076,#25590,#25591);
#21487=AXIS2_PLACEMENT_3D('',#55171,#25593,#25594);
#21488=AXIS2_PLACEMENT_3D('',#55264,#25596,#25597);
#21489=AXIS2_PLACEMENT_3D('',#55266,#25598,#25599);
#21490=AXIS2_PLACEMENT_3D('',#55273,#25600,#25601);
#21491=AXIS2_PLACEMENT_3D('',#55359,#25603,#25604);
#21492=AXIS2_PLACEMENT_3D('',#55454,#25606,#25607);
#21493=AXIS2_PLACEMENT_3D('',#55455,#25608,#25609);
#21494=AXIS2_PLACEMENT_3D('',#55456,#25610,#25611);
#21495=AXIS2_PLACEMENT_3D('',#55551,#25613,#25614);
#21496=AXIS2_PLACEMENT_3D('',#55647,#25616,#25617);
#21497=AXIS2_PLACEMENT_3D('',#55649,#25618,#25619);
#21498=AXIS2_PLACEMENT_3D('',#55656,#25620,#25621);
#21499=AXIS2_PLACEMENT_3D('',#55742,#25623,#25624);
#21500=AXIS2_PLACEMENT_3D('',#55837,#25626,#25627);
#21501=AXIS2_PLACEMENT_3D('',#55838,#25628,#25629);
#21502=AXIS2_PLACEMENT_3D('',#55839,#25630,#25631);
#21503=AXIS2_PLACEMENT_3D('',#55934,#25633,#25634);
#21504=AXIS2_PLACEMENT_3D('',#56027,#25636,#25637);
#21505=AXIS2_PLACEMENT_3D('',#56029,#25638,#25639);
#21506=AXIS2_PLACEMENT_3D('',#56036,#25640,#25641);
#21507=AXIS2_PLACEMENT_3D('',#56122,#25643,#25644);
#21508=AXIS2_PLACEMENT_3D('',#56217,#25646,#25647);
#21509=AXIS2_PLACEMENT_3D('',#56218,#25648,#25649);
#21510=AXIS2_PLACEMENT_3D('',#56219,#25650,#25651);
#21511=AXIS2_PLACEMENT_3D('',#56314,#25653,#25654);
#21512=AXIS2_PLACEMENT_3D('',#56413,#25656,#25657);
#21513=AXIS2_PLACEMENT_3D('',#56415,#25658,#25659);
#21514=AXIS2_PLACEMENT_3D('',#56422,#25660,#25661);
#21515=AXIS2_PLACEMENT_3D('',#56508,#25663,#25664);
#21516=AXIS2_PLACEMENT_3D('',#56603,#25666,#25667);
#21517=AXIS2_PLACEMENT_3D('',#56604,#25668,#25669);
#21518=AXIS2_PLACEMENT_3D('',#56605,#25670,#25671);
#21519=AXIS2_PLACEMENT_3D('',#56698,#25673,#25674);
#21520=AXIS2_PLACEMENT_3D('',#56877,#25677,#25678);
#21521=AXIS2_PLACEMENT_3D('',#56985,#25680,#25681);
#21522=AXIS2_PLACEMENT_3D('',#56987,#25682,#25683);
#21523=AXIS2_PLACEMENT_3D('',#56992,#25684,#25685);
#21524=AXIS2_PLACEMENT_3D('',#56994,#25686,#25687);
#21525=AXIS2_PLACEMENT_3D('',#56999,#25688,#25689);
#21526=AXIS2_PLACEMENT_3D('',#57101,#25691,#25692);
#21527=AXIS2_PLACEMENT_3D('',#57183,#25694,#25695);
#21528=AXIS2_PLACEMENT_3D('',#57185,#25696,#25697);
#21529=AXIS2_PLACEMENT_3D('',#57190,#25698,#25699);
#21530=AXIS2_PLACEMENT_3D('',#57192,#25700,#25701);
#21531=AXIS2_PLACEMENT_3D('',#57197,#25702,#25703);
#21532=AXIS2_PLACEMENT_3D('',#57299,#25705,#25706);
#21533=AXIS2_PLACEMENT_3D('',#57381,#25708,#25709);
#21534=AXIS2_PLACEMENT_3D('',#57383,#25710,#25711);
#21535=AXIS2_PLACEMENT_3D('',#57388,#25712,#25713);
#21536=AXIS2_PLACEMENT_3D('',#57390,#25714,#25715);
#21537=AXIS2_PLACEMENT_3D('',#57395,#25716,#25717);
#21538=AXIS2_PLACEMENT_3D('',#57497,#25719,#25720);
#21539=AXIS2_PLACEMENT_3D('',#57579,#25722,#25723);
#21540=AXIS2_PLACEMENT_3D('',#57581,#25724,#25725);
#21541=AXIS2_PLACEMENT_3D('',#57586,#25726,#25727);
#21542=AXIS2_PLACEMENT_3D('',#57588,#25728,#25729);
#21543=AXIS2_PLACEMENT_3D('',#57593,#25730,#25731);
#21544=AXIS2_PLACEMENT_3D('',#57695,#25733,#25734);
#21545=AXIS2_PLACEMENT_3D('',#57777,#25736,#25737);
#21546=AXIS2_PLACEMENT_3D('',#57779,#25738,#25739);
#21547=AXIS2_PLACEMENT_3D('',#57784,#25740,#25741);
#21548=AXIS2_PLACEMENT_3D('',#57786,#25742,#25743);
#21549=AXIS2_PLACEMENT_3D('',#57791,#25744,#25745);
#21550=AXIS2_PLACEMENT_3D('',#57893,#25747,#25748);
#21551=AXIS2_PLACEMENT_3D('',#57975,#25750,#25751);
#21552=AXIS2_PLACEMENT_3D('',#57977,#25752,#25753);
#21553=AXIS2_PLACEMENT_3D('',#57988,#25754,#25755);
#21554=AXIS2_PLACEMENT_3D('',#57990,#25756,#25757);
#21555=AXIS2_PLACEMENT_3D('',#57995,#25758,#25759);
#21556=AXIS2_PLACEMENT_3D('',#58118,#25761,#25762);
#21557=AXIS2_PLACEMENT_3D('',#58200,#25764,#25765);
#21558=AXIS2_PLACEMENT_3D('',#58202,#25766,#25767);
#21559=AXIS2_PLACEMENT_3D('',#58207,#25768,#25769);
#21560=AXIS2_PLACEMENT_3D('',#58209,#25770,#25771);
#21561=AXIS2_PLACEMENT_3D('',#58214,#25772,#25773);
#21562=AXIS2_PLACEMENT_3D('',#58316,#25775,#25776);
#21563=AXIS2_PLACEMENT_3D('',#58398,#25778,#25779);
#21564=AXIS2_PLACEMENT_3D('',#58400,#25780,#25781);
#21565=AXIS2_PLACEMENT_3D('',#58405,#25782,#25783);
#21566=AXIS2_PLACEMENT_3D('',#58407,#25784,#25785);
#21567=AXIS2_PLACEMENT_3D('',#58412,#25786,#25787);
#21568=AXIS2_PLACEMENT_3D('',#58514,#25789,#25790);
#21569=AXIS2_PLACEMENT_3D('',#58596,#25792,#25793);
#21570=AXIS2_PLACEMENT_3D('',#58598,#25794,#25795);
#21571=AXIS2_PLACEMENT_3D('',#58603,#25796,#25797);
#21572=AXIS2_PLACEMENT_3D('',#58605,#25798,#25799);
#21573=AXIS2_PLACEMENT_3D('',#58610,#25800,#25801);
#21574=AXIS2_PLACEMENT_3D('',#58712,#25803,#25804);
#21575=AXIS2_PLACEMENT_3D('',#58794,#25806,#25807);
#21576=AXIS2_PLACEMENT_3D('',#58796,#25808,#25809);
#21577=AXIS2_PLACEMENT_3D('',#58801,#25810,#25811);
#21578=AXIS2_PLACEMENT_3D('',#58803,#25812,#25813);
#21579=AXIS2_PLACEMENT_3D('',#58808,#25814,#25815);
#21580=AXIS2_PLACEMENT_3D('',#58910,#25817,#25818);
#21581=AXIS2_PLACEMENT_3D('',#58992,#25820,#25821);
#21582=AXIS2_PLACEMENT_3D('',#58994,#25822,#25823);
#21583=AXIS2_PLACEMENT_3D('',#58999,#25824,#25825);
#21584=AXIS2_PLACEMENT_3D('',#59001,#25826,#25827);
#21585=AXIS2_PLACEMENT_3D('',#59006,#25828,#25829);
#21586=AXIS2_PLACEMENT_3D('',#59108,#25831,#25832);
#21587=AXIS2_PLACEMENT_3D('',#59190,#25834,#25835);
#21588=AXIS2_PLACEMENT_3D('',#59192,#25836,#25837);
#21589=AXIS2_PLACEMENT_3D('',#59203,#25838,#25839);
#21590=AXIS2_PLACEMENT_3D('',#59205,#25840,#25841);
#21591=AXIS2_PLACEMENT_3D('',#59210,#25842,#25843);
#21592=AXIS2_PLACEMENT_3D('',#59322,#25845,#25846);
#21593=AXIS2_PLACEMENT_3D('',#59404,#25848,#25849);
#21594=AXIS2_PLACEMENT_3D('',#59406,#25850,#25851);
#21595=AXIS2_PLACEMENT_3D('',#59417,#25852,#25853);
#21596=AXIS2_PLACEMENT_3D('',#59419,#25854,#25855);
#21597=AXIS2_PLACEMENT_3D('',#59424,#25856,#25857);
#21598=AXIS2_PLACEMENT_3D('',#59532,#25859,#25860);
#21599=AXIS2_PLACEMENT_3D('',#59614,#25862,#25863);
#21600=AXIS2_PLACEMENT_3D('',#59616,#25864,#25865);
#21601=AXIS2_PLACEMENT_3D('',#59621,#25866,#25867);
#21602=AXIS2_PLACEMENT_3D('',#59623,#25868,#25869);
#21603=AXIS2_PLACEMENT_3D('',#59628,#25870,#25871);
#21604=AXIS2_PLACEMENT_3D('',#59730,#25873,#25874);
#21605=AXIS2_PLACEMENT_3D('',#59812,#25876,#25877);
#21606=AXIS2_PLACEMENT_3D('',#59814,#25878,#25879);
#21607=AXIS2_PLACEMENT_3D('',#59819,#25880,#25881);
#21608=AXIS2_PLACEMENT_3D('',#59821,#25882,#25883);
#21609=AXIS2_PLACEMENT_3D('',#59826,#25884,#25885);
#21610=AXIS2_PLACEMENT_3D('',#59928,#25887,#25888);
#21611=AXIS2_PLACEMENT_3D('',#60010,#25890,#25891);
#21612=AXIS2_PLACEMENT_3D('',#60012,#25892,#25893);
#21613=AXIS2_PLACEMENT_3D('',#60017,#25894,#25895);
#21614=AXIS2_PLACEMENT_3D('',#60019,#25896,#25897);
#21615=AXIS2_PLACEMENT_3D('',#60024,#25898,#25899);
#21616=AXIS2_PLACEMENT_3D('',#60126,#25901,#25902);
#21617=AXIS2_PLACEMENT_3D('',#60208,#25904,#25905);
#21618=AXIS2_PLACEMENT_3D('',#60210,#25906,#25907);
#21619=AXIS2_PLACEMENT_3D('',#60215,#25908,#25909);
#21620=AXIS2_PLACEMENT_3D('',#60217,#25910,#25911);
#21621=AXIS2_PLACEMENT_3D('',#60222,#25912,#25913);
#21622=AXIS2_PLACEMENT_3D('',#60324,#25915,#25916);
#21623=AXIS2_PLACEMENT_3D('',#60406,#25918,#25919);
#21624=AXIS2_PLACEMENT_3D('',#60408,#25920,#25921);
#21625=AXIS2_PLACEMENT_3D('',#60419,#25922,#25923);
#21626=AXIS2_PLACEMENT_3D('',#60421,#25924,#25925);
#21627=AXIS2_PLACEMENT_3D('',#60426,#25926,#25927);
#21628=AXIS2_PLACEMENT_3D('',#60536,#25929,#25930);
#21629=AXIS2_PLACEMENT_3D('',#60618,#25932,#25933);
#21630=AXIS2_PLACEMENT_3D('',#60620,#25934,#25935);
#21631=AXIS2_PLACEMENT_3D('',#60631,#25936,#25937);
#21632=AXIS2_PLACEMENT_3D('',#60633,#25938,#25939);
#21633=AXIS2_PLACEMENT_3D('',#60638,#25940,#25941);
#21634=AXIS2_PLACEMENT_3D('',#60746,#25943,#25944);
#21635=AXIS2_PLACEMENT_3D('',#60828,#25946,#25947);
#21636=AXIS2_PLACEMENT_3D('',#60830,#25948,#25949);
#21637=AXIS2_PLACEMENT_3D('',#60835,#25950,#25951);
#21638=AXIS2_PLACEMENT_3D('',#60837,#25952,#25953);
#21639=AXIS2_PLACEMENT_3D('',#60842,#25954,#25955);
#21640=AXIS2_PLACEMENT_3D('',#60944,#25957,#25958);
#21641=AXIS2_PLACEMENT_3D('',#61026,#25960,#25961);
#21642=AXIS2_PLACEMENT_3D('',#61028,#25962,#25963);
#21643=AXIS2_PLACEMENT_3D('',#61033,#25964,#25965);
#21644=AXIS2_PLACEMENT_3D('',#61035,#25966,#25967);
#21645=AXIS2_PLACEMENT_3D('',#61040,#25968,#25969);
#21646=AXIS2_PLACEMENT_3D('',#61142,#25971,#25972);
#21647=AXIS2_PLACEMENT_3D('',#61224,#25974,#25975);
#21648=AXIS2_PLACEMENT_3D('',#61226,#25976,#25977);
#21649=AXIS2_PLACEMENT_3D('',#61231,#25978,#25979);
#21650=AXIS2_PLACEMENT_3D('',#61233,#25980,#25981);
#21651=AXIS2_PLACEMENT_3D('',#61238,#25982,#25983);
#21652=AXIS2_PLACEMENT_3D('',#61340,#25985,#25986);
#21653=AXIS2_PLACEMENT_3D('',#61422,#25988,#25989);
#21654=AXIS2_PLACEMENT_3D('',#61424,#25990,#25991);
#21655=AXIS2_PLACEMENT_3D('',#61429,#25992,#25993);
#21656=AXIS2_PLACEMENT_3D('',#61431,#25994,#25995);
#21657=AXIS2_PLACEMENT_3D('',#61436,#25996,#25997);
#21658=AXIS2_PLACEMENT_3D('',#61538,#25999,#26000);
#21659=AXIS2_PLACEMENT_3D('',#61620,#26002,#26003);
#21660=AXIS2_PLACEMENT_3D('',#61622,#26004,#26005);
#21661=AXIS2_PLACEMENT_3D('',#61627,#26006,#26007);
#21662=AXIS2_PLACEMENT_3D('',#61629,#26008,#26009);
#21663=AXIS2_PLACEMENT_3D('',#61634,#26010,#26011);
#21664=AXIS2_PLACEMENT_3D('',#61736,#26013,#26014);
#21665=AXIS2_PLACEMENT_3D('',#61818,#26016,#26017);
#21666=AXIS2_PLACEMENT_3D('',#61819,#26018,#26019);
#21667=AXIS2_PLACEMENT_3D('',#61820,#26020,#26021);
#21668=AXIS2_PLACEMENT_3D('',#61821,#26022,#26023);
#21669=AXIS2_PLACEMENT_3D('',#61822,#26024,#26025);
#21670=AXIS2_PLACEMENT_3D('',#61823,#26026,#26027);
#21671=AXIS2_PLACEMENT_3D('',#61824,#26028,#26029);
#21672=AXIS2_PLACEMENT_3D('',#61825,#26030,#26031);
#25201=DIRECTION('axis',(0.,0.,1.));
#25202=DIRECTION('refdir',(1.,0.,0.));
#25203=DIRECTION('center_axis',(1.,0.,0.));
#25204=DIRECTION('ref_axis',(0.,-1.,0.));
#25205=DIRECTION('center_axis',(-1.,0.,0.));
#25206=DIRECTION('ref_axis',(0.,-1.,0.));
#25207=DIRECTION('center_axis',(-1.,0.,0.));
#25208=DIRECTION('ref_axis',(0.,-1.,0.));
#25209=DIRECTION('',(0.707106781186546,0.70710678118655,-8.65956056235496E-17));
#25210=DIRECTION('center_axis',(1.,0.,0.));
#25211=DIRECTION('ref_axis',(0.,-1.,0.));
#25212=DIRECTION('center_axis',(1.,0.,0.));
#25213=DIRECTION('ref_axis',(0.,1.,0.));
#25214=DIRECTION('',(-1.,0.,0.));
#25215=DIRECTION('center_axis',(1.,0.,0.));
#25216=DIRECTION('ref_axis',(0.,-1.,0.));
#25217=DIRECTION('center_axis',(1.,0.,0.));
#25218=DIRECTION('ref_axis',(0.,-1.,0.));
#25219=DIRECTION('center_axis',(1.,0.,0.));
#25220=DIRECTION('ref_axis',(0.,0.,-1.));
#25221=DIRECTION('center_axis',(1.,0.,0.));
#25222=DIRECTION('ref_axis',(0.,0.947793690616251,-0.318884179645254));
#25223=DIRECTION('center_axis',(1.,0.,0.));
#25224=DIRECTION('ref_axis',(0.,0.,-1.));
#25225=DIRECTION('center_axis',(1.,0.,0.));
#25226=DIRECTION('ref_axis',(0.,0.992291268649497,0.123927552069634));
#25227=DIRECTION('center_axis',(1.,0.,0.));
#25228=DIRECTION('ref_axis',(0.,0.,-1.));
#25229=DIRECTION('center_axis',(1.,0.,0.));
#25230=DIRECTION('ref_axis',(0.,0.840253391272934,0.542193912225445));
#25231=DIRECTION('center_axis',(1.,0.,0.));
#25232=DIRECTION('ref_axis',(0.,0.,-1.));
#25233=DIRECTION('center_axis',(1.,0.,0.));
#25234=DIRECTION('ref_axis',(0.,0.521793024723191,0.853072118493052));
#25235=DIRECTION('center_axis',(1.,0.,0.));
#25236=DIRECTION('ref_axis',(0.,0.,-1.));
#25237=DIRECTION('center_axis',(1.,0.,0.));
#25238=DIRECTION('ref_axis',(0.,0.0999851502555302,0.994988929450162));
#25239=DIRECTION('center_axis',(1.,0.,0.));
#25240=DIRECTION('ref_axis',(0.,0.,-1.));
#25241=DIRECTION('center_axis',(1.,0.,0.));
#25242=DIRECTION('ref_axis',(0.,-0.341626009457634,0.939835980191253));
#25243=DIRECTION('center_axis',(1.,0.,0.));
#25244=DIRECTION('ref_axis',(0.,0.,-1.));
#25245=DIRECTION('center_axis',(1.,0.,0.));
#25246=DIRECTION('ref_axis',(0.,-0.715573948229662,0.698536988723585));
#25247=DIRECTION('center_axis',(1.,0.,0.));
#25248=DIRECTION('ref_axis',(0.,0.,-1.));
#25249=DIRECTION('center_axis',(1.,0.,0.));
#25250=DIRECTION('ref_axis',(0.,-0.947793690616251,0.318884179645253));
#25251=DIRECTION('center_axis',(1.,0.,0.));
#25252=DIRECTION('ref_axis',(0.,0.,-1.));
#25253=DIRECTION('center_axis',(1.,0.,0.));
#25254=DIRECTION('ref_axis',(0.,-0.992291268649497,-0.123927552069633));
#25255=DIRECTION('center_axis',(1.,0.,0.));
#25256=DIRECTION('ref_axis',(0.,0.,-1.));
#25257=DIRECTION('center_axis',(1.,0.,0.));
#25258=DIRECTION('ref_axis',(0.,-0.840253391272934,-0.542193912225445));
#25259=DIRECTION('center_axis',(1.,0.,0.));
#25260=DIRECTION('ref_axis',(0.,0.,-1.));
#25261=DIRECTION('center_axis',(1.,0.,0.));
#25262=DIRECTION('ref_axis',(0.,-0.521793024723191,-0.853072118493052));
#25263=DIRECTION('center_axis',(1.,0.,0.));
#25264=DIRECTION('ref_axis',(0.,0.,-1.));
#25265=DIRECTION('center_axis',(1.,0.,0.));
#25266=DIRECTION('ref_axis',(0.,-0.0999851502555303,-0.994988929450162));
#25267=DIRECTION('center_axis',(1.,0.,0.));
#25268=DIRECTION('ref_axis',(0.,0.,-1.));
#25269=DIRECTION('center_axis',(1.,0.,0.));
#25270=DIRECTION('ref_axis',(0.,0.341626009457634,-0.939835980191253));
#25271=DIRECTION('center_axis',(1.,0.,0.));
#25272=DIRECTION('ref_axis',(0.,0.,-1.));
#25273=DIRECTION('center_axis',(1.,0.,0.));
#25274=DIRECTION('ref_axis',(0.,0.715573948229662,-0.698536988723585));
#25275=DIRECTION('center_axis',(1.,0.,0.));
#25276=DIRECTION('ref_axis',(0.,0.,-1.));
#25277=DIRECTION('center_axis',(-1.,0.,0.));
#25278=DIRECTION('ref_axis',(0.,-1.,0.));
#25279=DIRECTION('center_axis',(-1.,0.,0.));
#25280=DIRECTION('ref_axis',(0.,-1.,0.));
#25281=DIRECTION('',(0.707106781186551,-0.707106781186544,8.65956056235489E-17));
#25282=DIRECTION('center_axis',(-1.,0.,0.));
#25283=DIRECTION('ref_axis',(0.,0.,1.));
#25284=DIRECTION('center_axis',(-1.,0.,0.));
#25285=DIRECTION('ref_axis',(0.,0.984693235726434,-0.174296389849606));
#25286=DIRECTION('center_axis',(1.,0.,0.));
#25287=DIRECTION('ref_axis',(0.,0.,-1.));
#25288=DIRECTION('center_axis',(-1.,0.,0.));
#25289=DIRECTION('ref_axis',(0.,0.910411537476949,-0.413703797938643));
#25290=DIRECTION('center_axis',(1.,0.,0.));
#25291=DIRECTION('ref_axis',(0.,0.,-1.));
#25292=DIRECTION('center_axis',(-1.,0.,0.));
#25293=DIRECTION('ref_axis',(0.,0.778925334068368,-0.627116674907055));
#25294=DIRECTION('center_axis',(1.,0.,0.));
#25295=DIRECTION('ref_axis',(0.,0.,-1.));
#25296=DIRECTION('center_axis',(-1.,0.,0.));
#25297=DIRECTION('ref_axis',(0.,0.598496387233281,-0.801125504817261));
#25298=DIRECTION('center_axis',(1.,0.,0.));
#25299=DIRECTION('ref_axis',(0.,0.,-1.));
#25300=DIRECTION('center_axis',(-1.,0.,0.));
#25301=DIRECTION('ref_axis',(0.,0.380461711272584,-0.924796672926291));
#25302=DIRECTION('center_axis',(1.,0.,0.));
#25303=DIRECTION('ref_axis',(0.,0.,-1.));
#25304=DIRECTION('center_axis',(-1.,0.,0.));
#25305=DIRECTION('ref_axis',(0.,0.138521226752336,-0.990359464911114));
#25306=DIRECTION('center_axis',(1.,0.,0.));
#25307=DIRECTION('ref_axis',(0.,0.,-1.));
#25308=DIRECTION('center_axis',(-1.,0.,0.));
#25309=DIRECTION('ref_axis',(0.,-0.112123055890198,-0.993694329428242));
#25310=DIRECTION('center_axis',(1.,0.,0.));
#25311=DIRECTION('ref_axis',(0.,0.,-1.));
#25312=DIRECTION('center_axis',(-1.,0.,0.));
#25313=DIRECTION('ref_axis',(0.,-0.355722234571395,-0.93459172467529));
#25314=DIRECTION('center_axis',(1.,0.,0.));
#25315=DIRECTION('ref_axis',(0.,0.,-1.));
#25316=DIRECTION('center_axis',(-1.,0.,0.));
#25317=DIRECTION('ref_axis',(0.,-0.576970076999607,-0.816765284673061));
#25318=DIRECTION('center_axis',(1.,0.,0.));
#25319=DIRECTION('ref_axis',(0.,0.,-1.));
#25320=DIRECTION('center_axis',(-1.,0.,0.));
#25321=DIRECTION('ref_axis',(0.,-0.761964767542423,-0.64761847798223));
#25322=DIRECTION('center_axis',(1.,0.,0.));
#25323=DIRECTION('ref_axis',(0.,0.,-1.));
#25324=DIRECTION('center_axis',(-1.,0.,0.));
#25325=DIRECTION('ref_axis',(0.,-0.899082409430159,-0.437779420545621));
#25326=DIRECTION('center_axis',(1.,0.,0.));
#25327=DIRECTION('ref_axis',(0.,0.,-1.));
#25328=DIRECTION('center_axis',(-1.,0.,0.));
#25329=DIRECTION('ref_axis',(0.,-0.979707396939596,-0.200433072076046));
#25330=DIRECTION('center_axis',(1.,0.,0.));
#25331=DIRECTION('ref_axis',(0.,0.,-1.));
#25332=DIRECTION('center_axis',(-1.,0.,0.));
#25333=DIRECTION('ref_axis',(0.,-0.998773765587553,0.0495072234533422));
#25334=DIRECTION('center_axis',(1.,0.,0.));
#25335=DIRECTION('ref_axis',(0.,0.,-1.));
#25336=DIRECTION('center_axis',(-1.,0.,0.));
#25337=DIRECTION('ref_axis',(0.,-0.955083505310682,0.296336798058325));
#25338=DIRECTION('center_axis',(1.,0.,0.));
#25339=DIRECTION('ref_axis',(0.,0.,-1.));
#25340=DIRECTION('center_axis',(-1.,0.,0.));
#25341=DIRECTION('ref_axis',(0.,-0.851381835843715,0.524546441790797));
#25342=DIRECTION('center_axis',(1.,0.,0.));
#25343=DIRECTION('ref_axis',(0.,0.,-1.));
#25344=DIRECTION('center_axis',(-1.,0.,0.));
#25345=DIRECTION('ref_axis',(0.,-0.694184714467323,0.719796903438686));
#25346=DIRECTION('center_axis',(1.,0.,0.));
#25347=DIRECTION('ref_axis',(0.,0.,-1.));
#25348=DIRECTION('center_axis',(-1.,0.,0.));
#25349=DIRECTION('ref_axis',(0.,-0.493369414448157,0.869819878415688));
#25350=DIRECTION('center_axis',(1.,0.,0.));
#25351=DIRECTION('ref_axis',(0.,0.,-1.));
#25352=DIRECTION('center_axis',(-1.,0.,0.));
#25353=DIRECTION('ref_axis',(0.,-0.261553899633433,0.965188871458091));
#25354=DIRECTION('center_axis',(1.,0.,0.));
#25355=DIRECTION('ref_axis',(0.,0.,-1.));
#25356=DIRECTION('center_axis',(-1.,0.,0.));
#25357=DIRECTION('ref_axis',(0.,-0.0133039913767846,0.99991149799042));
#25358=DIRECTION('center_axis',(1.,0.,0.));
#25359=DIRECTION('ref_axis',(0.,0.,-1.));
#25360=DIRECTION('center_axis',(-1.,0.,0.));
#25361=DIRECTION('ref_axis',(0.,0.235781855586725,0.971806007686761));
#25362=DIRECTION('center_axis',(1.,0.,0.));
#25363=DIRECTION('ref_axis',(0.,0.,-1.));
#25364=DIRECTION('center_axis',(-1.,0.,0.));
#25365=DIRECTION('ref_axis',(0.,0.470052661418713,0.882638371867655));
#25366=DIRECTION('center_axis',(1.,0.,0.));
#25367=DIRECTION('ref_axis',(0.,0.,-1.));
#25368=DIRECTION('center_axis',(-1.,0.,0.));
#25369=DIRECTION('ref_axis',(0.,0.674788329801001,0.738011321027242));
#25370=DIRECTION('center_axis',(1.,0.,0.));
#25371=DIRECTION('ref_axis',(0.,0.,-1.));
#25372=DIRECTION('center_axis',(-1.,0.,0.));
#25373=DIRECTION('ref_axis',(0.,0.837124565724013,0.547012304670911));
#25374=DIRECTION('center_axis',(1.,0.,0.));
#25375=DIRECTION('ref_axis',(0.,0.,-1.));
#25376=DIRECTION('center_axis',(-1.,0.,0.));
#25377=DIRECTION('ref_axis',(0.,0.946861186453793,0.321642493441576));
#25378=DIRECTION('center_axis',(1.,0.,0.));
#25379=DIRECTION('ref_axis',(0.,0.,-1.));
#25380=DIRECTION('center_axis',(-1.,0.,0.));
#25381=DIRECTION('ref_axis',(0.,0.99710303652683,0.0760627014309627));
#25382=DIRECTION('center_axis',(1.,0.,0.));
#25383=DIRECTION('ref_axis',(0.,0.,-1.));
#25384=DIRECTION('',(1.,0.,0.));
#25385=DIRECTION('center_axis',(1.,0.,0.));
#25386=DIRECTION('ref_axis',(0.,0.947793690616251,-0.318884179645254));
#25387=DIRECTION('center_axis',(1.,0.,0.));
#25388=DIRECTION('ref_axis',(0.,0.947793690616251,-0.318884179645254));
#25389=DIRECTION('',(1.,0.,0.));
#25390=DIRECTION('center_axis',(-1.,0.,0.));
#25391=DIRECTION('ref_axis',(0.,1.,0.));
#25392=DIRECTION('center_axis',(1.,0.,0.));
#25393=DIRECTION('ref_axis',(0.,0.,-1.));
#25394=DIRECTION('center_axis',(1.,0.,0.));
#25395=DIRECTION('ref_axis',(0.,1.,0.));
#25396=DIRECTION('center_axis',(1.,0.,0.));
#25397=DIRECTION('ref_axis',(0.,0.,-1.));
#25398=DIRECTION('',(1.,0.,0.));
#25399=DIRECTION('center_axis',(1.,0.,0.));
#25400=DIRECTION('ref_axis',(0.,0.715573948229662,-0.698536988723585));
#25401=DIRECTION('center_axis',(1.,0.,0.));
#25402=DIRECTION('ref_axis',(0.,0.715573948229662,-0.698536988723585));
#25403=DIRECTION('',(1.,0.,0.));
#25404=DIRECTION('center_axis',(1.,0.,0.));
#25405=DIRECTION('ref_axis',(0.,0.,-1.));
#25406=DIRECTION('center_axis',(1.,0.,0.));
#25407=DIRECTION('ref_axis',(0.,0.,-1.));
#25408=DIRECTION('center_axis',(1.,0.,0.));
#25409=DIRECTION('ref_axis',(0.,0.99710303652683,0.0760627014309627));
#25410=DIRECTION('center_axis',(1.,0.,0.));
#25411=DIRECTION('ref_axis',(0.,0.,-1.));
#25412=DIRECTION('center_axis',(1.,0.,0.));
#25413=DIRECTION('ref_axis',(0.,0.946861186453793,0.321642493441576));
#25414=DIRECTION('center_axis',(1.,0.,0.));
#25415=DIRECTION('ref_axis',(0.,0.,-1.));
#25416=DIRECTION('center_axis',(1.,0.,0.));
#25417=DIRECTION('ref_axis',(0.,0.837124565724013,0.547012304670911));
#25418=DIRECTION('center_axis',(1.,0.,0.));
#25419=DIRECTION('ref_axis',(0.,0.,-1.));
#25420=DIRECTION('center_axis',(1.,0.,0.));
#25421=DIRECTION('ref_axis',(0.,0.674788329801001,0.738011321027242));
#25422=DIRECTION('center_axis',(1.,0.,0.));
#25423=DIRECTION('ref_axis',(0.,0.,-1.));
#25424=DIRECTION('center_axis',(1.,0.,0.));
#25425=DIRECTION('ref_axis',(0.,0.470052661418713,0.882638371867655));
#25426=DIRECTION('center_axis',(1.,0.,0.));
#25427=DIRECTION('ref_axis',(0.,0.,-1.));
#25428=DIRECTION('center_axis',(1.,0.,0.));
#25429=DIRECTION('ref_axis',(0.,0.235781855586725,0.971806007686761));
#25430=DIRECTION('center_axis',(1.,0.,0.));
#25431=DIRECTION('ref_axis',(0.,0.,-1.));
#25432=DIRECTION('center_axis',(1.,0.,0.));
#25433=DIRECTION('ref_axis',(0.,-0.0133039913767846,0.99991149799042));
#25434=DIRECTION('center_axis',(1.,0.,0.));
#25435=DIRECTION('ref_axis',(0.,0.,-1.));
#25436=DIRECTION('center_axis',(1.,0.,0.));
#25437=DIRECTION('ref_axis',(0.,-0.261553899633433,0.965188871458091));
#25438=DIRECTION('center_axis',(1.,0.,0.));
#25439=DIRECTION('ref_axis',(0.,0.,-1.));
#25440=DIRECTION('center_axis',(1.,0.,0.));
#25441=DIRECTION('ref_axis',(0.,-0.493369414448157,0.869819878415688));
#25442=DIRECTION('center_axis',(1.,0.,0.));
#25443=DIRECTION('ref_axis',(0.,0.,-1.));
#25444=DIRECTION('center_axis',(1.,0.,0.));
#25445=DIRECTION('ref_axis',(0.,-0.694184714467323,0.719796903438686));
#25446=DIRECTION('center_axis',(1.,0.,0.));
#25447=DIRECTION('ref_axis',(0.,0.,-1.));
#25448=DIRECTION('center_axis',(1.,0.,0.));
#25449=DIRECTION('ref_axis',(0.,-0.851381835843715,0.524546441790797));
#25450=DIRECTION('center_axis',(1.,0.,0.));
#25451=DIRECTION('ref_axis',(0.,0.,-1.));
#25452=DIRECTION('center_axis',(1.,0.,0.));
#25453=DIRECTION('ref_axis',(0.,-0.955083505310682,0.296336798058325));
#25454=DIRECTION('center_axis',(1.,0.,0.));
#25455=DIRECTION('ref_axis',(0.,0.,-1.));
#25456=DIRECTION('center_axis',(1.,0.,0.));
#25457=DIRECTION('ref_axis',(0.,-0.998773765587553,0.0495072234533422));
#25458=DIRECTION('center_axis',(1.,0.,0.));
#25459=DIRECTION('ref_axis',(0.,0.,-1.));
#25460=DIRECTION('center_axis',(1.,0.,0.));
#25461=DIRECTION('ref_axis',(0.,-0.979707396939596,-0.200433072076046));
#25462=DIRECTION('center_axis',(1.,0.,0.));
#25463=DIRECTION('ref_axis',(0.,0.,-1.));
#25464=DIRECTION('center_axis',(1.,0.,0.));
#25465=DIRECTION('ref_axis',(0.,-0.899082409430159,-0.437779420545621));
#25466=DIRECTION('center_axis',(1.,0.,0.));
#25467=DIRECTION('ref_axis',(0.,0.,-1.));
#25468=DIRECTION('center_axis',(1.,0.,0.));
#25469=DIRECTION('ref_axis',(0.,-0.761964767542423,-0.64761847798223));
#25470=DIRECTION('center_axis',(1.,0.,0.));
#25471=DIRECTION('ref_axis',(0.,0.,-1.));
#25472=DIRECTION('center_axis',(1.,0.,0.));
#25473=DIRECTION('ref_axis',(0.,-0.576970076999607,-0.816765284673061));
#25474=DIRECTION('center_axis',(1.,0.,0.));
#25475=DIRECTION('ref_axis',(0.,0.,-1.));
#25476=DIRECTION('center_axis',(1.,0.,0.));
#25477=DIRECTION('ref_axis',(0.,-0.355722234571395,-0.93459172467529));
#25478=DIRECTION('center_axis',(1.,0.,0.));
#25479=DIRECTION('ref_axis',(0.,0.,-1.));
#25480=DIRECTION('center_axis',(1.,0.,0.));
#25481=DIRECTION('ref_axis',(0.,-0.112123055890198,-0.993694329428242));
#25482=DIRECTION('center_axis',(1.,0.,0.));
#25483=DIRECTION('ref_axis',(0.,0.,-1.));
#25484=DIRECTION('center_axis',(1.,0.,0.));
#25485=DIRECTION('ref_axis',(0.,0.138521226752336,-0.990359464911114));
#25486=DIRECTION('center_axis',(1.,0.,0.));
#25487=DIRECTION('ref_axis',(0.,0.,-1.));
#25488=DIRECTION('center_axis',(1.,0.,0.));
#25489=DIRECTION('ref_axis',(0.,0.380461711272584,-0.924796672926291));
#25490=DIRECTION('center_axis',(1.,0.,0.));
#25491=DIRECTION('ref_axis',(0.,0.,-1.));
#25492=DIRECTION('center_axis',(1.,0.,0.));
#25493=DIRECTION('ref_axis',(0.,0.598496387233281,-0.801125504817261));
#25494=DIRECTION('center_axis',(1.,0.,0.));
#25495=DIRECTION('ref_axis',(0.,0.,-1.));
#25496=DIRECTION('center_axis',(1.,0.,0.));
#25497=DIRECTION('ref_axis',(0.,0.778925334068368,-0.627116674907055));
#25498=DIRECTION('center_axis',(1.,0.,0.));
#25499=DIRECTION('ref_axis',(0.,0.,-1.));
#25500=DIRECTION('center_axis',(1.,0.,0.));
#25501=DIRECTION('ref_axis',(0.,0.910411537476949,-0.413703797938643));
#25502=DIRECTION('center_axis',(1.,0.,0.));
#25503=DIRECTION('ref_axis',(0.,0.,-1.));
#25504=DIRECTION('center_axis',(1.,0.,0.));
#25505=DIRECTION('ref_axis',(0.,0.984693235726434,-0.174296389849606));
#25506=DIRECTION('center_axis',(1.,0.,0.));
#25507=DIRECTION('ref_axis',(0.,0.,-1.));
#25508=DIRECTION('center_axis',(1.,0.,0.));
#25509=DIRECTION('ref_axis',(0.,0.,-1.));
#25510=DIRECTION('center_axis',(1.,0.,0.));
#25511=DIRECTION('ref_axis',(0.,0.341626009457634,-0.939835980191253));
#25512=DIRECTION('center_axis',(1.,0.,0.));
#25513=DIRECTION('ref_axis',(0.,0.,-1.));
#25514=DIRECTION('center_axis',(1.,0.,0.));
#25515=DIRECTION('ref_axis',(0.,-0.0999851502555303,-0.994988929450162));
#25516=DIRECTION('center_axis',(1.,0.,0.));
#25517=DIRECTION('ref_axis',(0.,0.,-1.));
#25518=DIRECTION('center_axis',(1.,0.,0.));
#25519=DIRECTION('ref_axis',(0.,-0.521793024723191,-0.853072118493052));
#25520=DIRECTION('center_axis',(1.,0.,0.));
#25521=DIRECTION('ref_axis',(0.,0.,-1.));
#25522=DIRECTION('center_axis',(1.,0.,0.));
#25523=DIRECTION('ref_axis',(0.,-0.840253391272934,-0.542193912225445));
#25524=DIRECTION('center_axis',(1.,0.,0.));
#25525=DIRECTION('ref_axis',(0.,0.,-1.));
#25526=DIRECTION('center_axis',(1.,0.,0.));
#25527=DIRECTION('ref_axis',(0.,-0.992291268649497,-0.123927552069633));
#25528=DIRECTION('center_axis',(1.,0.,0.));
#25529=DIRECTION('ref_axis',(0.,0.,-1.));
#25530=DIRECTION('center_axis',(1.,0.,0.));
#25531=DIRECTION('ref_axis',(0.,-0.947793690616251,0.318884179645253));
#25532=DIRECTION('center_axis',(1.,0.,0.));
#25533=DIRECTION('ref_axis',(0.,0.,-1.));
#25534=DIRECTION('center_axis',(1.,0.,0.));
#25535=DIRECTION('ref_axis',(0.,-0.715573948229662,0.698536988723585));
#25536=DIRECTION('center_axis',(1.,0.,0.));
#25537=DIRECTION('ref_axis',(0.,0.,-1.));
#25538=DIRECTION('center_axis',(1.,0.,0.));
#25539=DIRECTION('ref_axis',(0.,-0.341626009457634,0.939835980191253));
#25540=DIRECTION('center_axis',(1.,0.,0.));
#25541=DIRECTION('ref_axis',(0.,0.,-1.));
#25542=DIRECTION('center_axis',(1.,0.,0.));
#25543=DIRECTION('ref_axis',(0.,0.0999851502555302,0.994988929450162));
#25544=DIRECTION('center_axis',(1.,0.,0.));
#25545=DIRECTION('ref_axis',(0.,0.,-1.));
#25546=DIRECTION('center_axis',(1.,0.,0.));
#25547=DIRECTION('ref_axis',(0.,0.521793024723191,0.853072118493052));
#25548=DIRECTION('center_axis',(1.,0.,0.));
#25549=DIRECTION('ref_axis',(0.,0.,-1.));
#25550=DIRECTION('center_axis',(1.,0.,0.));
#25551=DIRECTION('ref_axis',(0.,0.840253391272934,0.542193912225445));
#25552=DIRECTION('center_axis',(1.,0.,0.));
#25553=DIRECTION('ref_axis',(0.,0.,-1.));
#25554=DIRECTION('center_axis',(1.,0.,0.));
#25555=DIRECTION('ref_axis',(0.,0.992291268649497,0.123927552069634));
#25556=DIRECTION('center_axis',(1.,0.,0.));
#25557=DIRECTION('ref_axis',(0.,1.,0.));
#25558=DIRECTION('center_axis',(1.,0.,0.));
#25559=DIRECTION('ref_axis',(0.,0.,-1.));
#25560=DIRECTION('center_axis',(-1.,0.,0.));
#25561=DIRECTION('ref_axis',(0.,1.,0.));
#25562=DIRECTION('',(1.,0.,0.));
#25563=DIRECTION('center_axis',(1.,0.,0.));
#25564=DIRECTION('ref_axis',(0.,0.341626009457634,-0.939835980191253));
#25565=DIRECTION('',(1.,0.,0.));
#25566=DIRECTION('center_axis',(-1.,0.,0.));
#25567=DIRECTION('ref_axis',(0.,1.,0.));
#25568=DIRECTION('center_axis',(1.,0.,0.));
#25569=DIRECTION('ref_axis',(0.,0.,-1.));
#25570=DIRECTION('center_axis',(1.,0.,0.));
#25571=DIRECTION('ref_axis',(0.,1.,0.));
#25572=DIRECTION('',(1.,0.,0.));
#25573=DIRECTION('center_axis',(1.,0.,0.));
#25574=DIRECTION('ref_axis',(0.,-0.0999851502555303,-0.994988929450162));
#25575=DIRECTION('',(1.,0.,0.));
#25576=DIRECTION('center_axis',(1.,0.,0.));
#25577=DIRECTION('ref_axis',(0.,1.,0.));
#25578=DIRECTION('center_axis',(1.,0.,0.));
#25579=DIRECTION('ref_axis',(0.,0.,-1.));
#25580=DIRECTION('center_axis',(-1.,0.,0.));
#25581=DIRECTION('ref_axis',(0.,1.,0.));
#25582=DIRECTION('',(1.,0.,0.));
#25583=DIRECTION('center_axis',(1.,0.,0.));
#25584=DIRECTION('ref_axis',(0.,-0.521793024723191,-0.853072118493052));
#25585=DIRECTION('',(1.,0.,0.));
#25586=DIRECTION('center_axis',(-1.,0.,0.));
#25587=DIRECTION('ref_axis',(0.,1.,0.));
#25588=DIRECTION('center_axis',(1.,0.,0.));
#25589=DIRECTION('ref_axis',(0.,0.,-1.));
#25590=DIRECTION('center_axis',(1.,0.,0.));
#25591=DIRECTION('ref_axis',(0.,1.,0.));
#25592=DIRECTION('',(1.,0.,0.));
#25593=DIRECTION('center_axis',(1.,0.,0.));
#25594=DIRECTION('ref_axis',(0.,-0.840253391272934,-0.542193912225445));
#25595=DIRECTION('',(1.,0.,0.));
#25596=DIRECTION('center_axis',(1.,0.,0.));
#25597=DIRECTION('ref_axis',(0.,1.,0.));
#25598=DIRECTION('center_axis',(1.,0.,0.));
#25599=DIRECTION('ref_axis',(0.,0.,-1.));
#25600=DIRECTION('center_axis',(-1.,0.,0.));
#25601=DIRECTION('ref_axis',(0.,1.,0.));
#25602=DIRECTION('',(1.,0.,0.));
#25603=DIRECTION('center_axis',(1.,0.,0.));
#25604=DIRECTION('ref_axis',(0.,-0.992291268649497,-0.123927552069633));
#25605=DIRECTION('',(1.,0.,0.));
#25606=DIRECTION('center_axis',(-1.,0.,0.));
#25607=DIRECTION('ref_axis',(0.,1.,0.));
#25608=DIRECTION('center_axis',(1.,0.,0.));
#25609=DIRECTION('ref_axis',(0.,0.,-1.));
#25610=DIRECTION('center_axis',(1.,0.,0.));
#25611=DIRECTION('ref_axis',(0.,1.,0.));
#25612=DIRECTION('',(1.,0.,0.));
#25613=DIRECTION('center_axis',(1.,0.,0.));
#25614=DIRECTION('ref_axis',(0.,-0.947793690616251,0.318884179645253));
#25615=DIRECTION('',(1.,0.,0.));
#25616=DIRECTION('center_axis',(1.,0.,0.));
#25617=DIRECTION('ref_axis',(0.,1.,0.));
#25618=DIRECTION('center_axis',(1.,0.,0.));
#25619=DIRECTION('ref_axis',(0.,0.,-1.));
#25620=DIRECTION('center_axis',(-1.,0.,0.));
#25621=DIRECTION('ref_axis',(0.,1.,0.));
#25622=DIRECTION('',(1.,0.,0.));
#25623=DIRECTION('center_axis',(1.,0.,0.));
#25624=DIRECTION('ref_axis',(0.,-0.715573948229662,0.698536988723585));
#25625=DIRECTION('',(1.,0.,0.));
#25626=DIRECTION('center_axis',(-1.,0.,0.));
#25627=DIRECTION('ref_axis',(0.,-0.99999975051671,-0.000706375620521827));
#25628=DIRECTION('center_axis',(1.,0.,0.));
#25629=DIRECTION('ref_axis',(0.,0.,-1.));
#25630=DIRECTION('center_axis',(1.,0.,0.));
#25631=DIRECTION('ref_axis',(0.,-0.99999795302892,0.00202334820765901));
#25632=DIRECTION('',(1.,0.,0.));
#25633=DIRECTION('center_axis',(1.,0.,0.));
#25634=DIRECTION('ref_axis',(0.,-0.341626009457634,0.939835980191253));
#25635=DIRECTION('',(1.,0.,0.));
#25636=DIRECTION('center_axis',(1.,0.,0.));
#25637=DIRECTION('ref_axis',(0.,1.,0.));
#25638=DIRECTION('center_axis',(1.,0.,0.));
#25639=DIRECTION('ref_axis',(0.,0.,-1.));
#25640=DIRECTION('center_axis',(-1.,0.,0.));
#25641=DIRECTION('ref_axis',(0.,1.,0.));
#25642=DIRECTION('',(1.,0.,0.));
#25643=DIRECTION('center_axis',(1.,0.,0.));
#25644=DIRECTION('ref_axis',(0.,0.0999851502555302,0.994988929450162));
#25645=DIRECTION('',(1.,0.,0.));
#25646=DIRECTION('center_axis',(-1.,0.,0.));
#25647=DIRECTION('ref_axis',(0.,1.,0.));
#25648=DIRECTION('center_axis',(1.,0.,0.));
#25649=DIRECTION('ref_axis',(0.,0.,-1.));
#25650=DIRECTION('center_axis',(1.,0.,0.));
#25651=DIRECTION('ref_axis',(0.,1.,0.));
#25652=DIRECTION('',(1.,0.,0.));
#25653=DIRECTION('center_axis',(1.,0.,0.));
#25654=DIRECTION('ref_axis',(0.,0.521793024723191,0.853072118493052));
#25655=DIRECTION('',(1.,0.,0.));
#25656=DIRECTION('center_axis',(1.,0.,0.));
#25657=DIRECTION('ref_axis',(0.,1.,0.));
#25658=DIRECTION('center_axis',(1.,0.,0.));
#25659=DIRECTION('ref_axis',(0.,0.,-1.));
#25660=DIRECTION('center_axis',(-1.,0.,0.));
#25661=DIRECTION('ref_axis',(0.,1.,0.));
#25662=DIRECTION('',(1.,0.,0.));
#25663=DIRECTION('center_axis',(1.,0.,0.));
#25664=DIRECTION('ref_axis',(0.,0.840253391272934,0.542193912225445));
#25665=DIRECTION('',(1.,0.,0.));
#25666=DIRECTION('center_axis',(-1.,0.,0.));
#25667=DIRECTION('ref_axis',(0.,1.,0.));
#25668=DIRECTION('center_axis',(1.,0.,0.));
#25669=DIRECTION('ref_axis',(0.,0.,-1.));
#25670=DIRECTION('center_axis',(1.,0.,0.));
#25671=DIRECTION('ref_axis',(0.,1.,0.));
#25672=DIRECTION('',(1.,0.,0.));
#25673=DIRECTION('center_axis',(1.,0.,0.));
#25674=DIRECTION('ref_axis',(0.,0.992291268649497,0.123927552069634));
#25675=DIRECTION('',(1.,0.,0.));
#25676=DIRECTION('',(1.,0.,0.));
#25677=DIRECTION('center_axis',(1.,0.,0.));
#25678=DIRECTION('ref_axis',(0.,0.984693235726434,-0.174296389849606));
#25679=DIRECTION('',(1.,0.,0.));
#25680=DIRECTION('center_axis',(1.,0.,0.));
#25681=DIRECTION('ref_axis',(0.,1.,0.));
#25682=DIRECTION('center_axis',(1.,0.,0.));
#25683=DIRECTION('ref_axis',(0.,0.,-1.));
#25684=DIRECTION('center_axis',(1.,0.,0.));
#25685=DIRECTION('ref_axis',(0.,1.,0.));
#25686=DIRECTION('center_axis',(1.,0.,0.));
#25687=DIRECTION('ref_axis',(0.,0.,-1.));
#25688=DIRECTION('center_axis',(-1.,0.,0.));
#25689=DIRECTION('ref_axis',(0.,1.,0.));
#25690=DIRECTION('',(1.,0.,0.));
#25691=DIRECTION('center_axis',(1.,0.,0.));
#25692=DIRECTION('ref_axis',(0.,0.910411537476949,-0.413703797938643));
#25693=DIRECTION('',(1.,0.,0.));
#25694=DIRECTION('center_axis',(1.,0.,0.));
#25695=DIRECTION('ref_axis',(0.,1.,0.));
#25696=DIRECTION('center_axis',(1.,0.,0.));
#25697=DIRECTION('ref_axis',(0.,0.,-1.));
#25698=DIRECTION('center_axis',(1.,0.,0.));
#25699=DIRECTION('ref_axis',(0.,1.,0.));
#25700=DIRECTION('center_axis',(1.,0.,0.));
#25701=DIRECTION('ref_axis',(0.,0.,-1.));
#25702=DIRECTION('center_axis',(-1.,0.,0.));
#25703=DIRECTION('ref_axis',(0.,1.,0.));
#25704=DIRECTION('',(1.,0.,0.));
#25705=DIRECTION('center_axis',(1.,0.,0.));
#25706=DIRECTION('ref_axis',(0.,0.778925334068368,-0.627116674907055));
#25707=DIRECTION('',(1.,0.,0.));
#25708=DIRECTION('center_axis',(1.,0.,0.));
#25709=DIRECTION('ref_axis',(0.,1.,0.));
#25710=DIRECTION('center_axis',(1.,0.,0.));
#25711=DIRECTION('ref_axis',(0.,0.,-1.));
#25712=DIRECTION('center_axis',(1.,0.,0.));
#25713=DIRECTION('ref_axis',(0.,1.,0.));
#25714=DIRECTION('center_axis',(1.,0.,0.));
#25715=DIRECTION('ref_axis',(0.,0.,-1.));
#25716=DIRECTION('center_axis',(-1.,0.,0.));
#25717=DIRECTION('ref_axis',(0.,1.,0.));
#25718=DIRECTION('',(1.,0.,0.));
#25719=DIRECTION('center_axis',(1.,0.,0.));
#25720=DIRECTION('ref_axis',(0.,0.598496387233281,-0.801125504817261));
#25721=DIRECTION('',(1.,0.,0.));
#25722=DIRECTION('center_axis',(1.,0.,0.));
#25723=DIRECTION('ref_axis',(0.,1.,0.));
#25724=DIRECTION('center_axis',(1.,0.,0.));
#25725=DIRECTION('ref_axis',(0.,0.,-1.));
#25726=DIRECTION('center_axis',(1.,0.,0.));
#25727=DIRECTION('ref_axis',(0.,1.,0.));
#25728=DIRECTION('center_axis',(1.,0.,0.));
#25729=DIRECTION('ref_axis',(0.,0.,-1.));
#25730=DIRECTION('center_axis',(-1.,0.,0.));
#25731=DIRECTION('ref_axis',(0.,1.,0.));
#25732=DIRECTION('',(1.,0.,0.));
#25733=DIRECTION('center_axis',(1.,0.,0.));
#25734=DIRECTION('ref_axis',(0.,0.380461711272584,-0.924796672926291));
#25735=DIRECTION('',(1.,0.,0.));
#25736=DIRECTION('center_axis',(1.,0.,0.));
#25737=DIRECTION('ref_axis',(0.,1.,0.));
#25738=DIRECTION('center_axis',(1.,0.,0.));
#25739=DIRECTION('ref_axis',(0.,0.,-1.));
#25740=DIRECTION('center_axis',(1.,0.,0.));
#25741=DIRECTION('ref_axis',(0.,1.,0.));
#25742=DIRECTION('center_axis',(1.,0.,0.));
#25743=DIRECTION('ref_axis',(0.,0.,-1.));
#25744=DIRECTION('center_axis',(-1.,0.,0.));
#25745=DIRECTION('ref_axis',(0.,1.,0.));
#25746=DIRECTION('',(1.,0.,0.));
#25747=DIRECTION('center_axis',(1.,0.,0.));
#25748=DIRECTION('ref_axis',(0.,0.138521226752336,-0.990359464911114));
#25749=DIRECTION('',(1.,0.,0.));
#25750=DIRECTION('center_axis',(1.,0.,0.));
#25751=DIRECTION('ref_axis',(0.,1.,0.));
#25752=DIRECTION('center_axis',(1.,0.,0.));
#25753=DIRECTION('ref_axis',(0.,0.,-1.));
#25754=DIRECTION('center_axis',(1.,0.,0.));
#25755=DIRECTION('ref_axis',(0.,1.,0.));
#25756=DIRECTION('center_axis',(1.,0.,0.));
#25757=DIRECTION('ref_axis',(0.,0.,-1.));
#25758=DIRECTION('center_axis',(-1.,0.,0.));
#25759=DIRECTION('ref_axis',(0.,1.,0.));
#25760=DIRECTION('',(1.,0.,0.));
#25761=DIRECTION('center_axis',(1.,0.,0.));
#25762=DIRECTION('ref_axis',(0.,-0.112123055890198,-0.993694329428242));
#25763=DIRECTION('',(1.,0.,0.));
#25764=DIRECTION('center_axis',(1.,0.,0.));
#25765=DIRECTION('ref_axis',(0.,1.,0.));
#25766=DIRECTION('center_axis',(1.,0.,0.));
#25767=DIRECTION('ref_axis',(0.,0.,-1.));
#25768=DIRECTION('center_axis',(1.,0.,0.));
#25769=DIRECTION('ref_axis',(0.,1.,0.));
#25770=DIRECTION('center_axis',(1.,0.,0.));
#25771=DIRECTION('ref_axis',(0.,0.,-1.));
#25772=DIRECTION('center_axis',(-1.,0.,0.));
#25773=DIRECTION('ref_axis',(0.,1.,0.));
#25774=DIRECTION('',(1.,0.,0.));
#25775=DIRECTION('center_axis',(1.,0.,0.));
#25776=DIRECTION('ref_axis',(0.,-0.355722234571395,-0.93459172467529));
#25777=DIRECTION('',(1.,0.,0.));
#25778=DIRECTION('center_axis',(1.,0.,0.));
#25779=DIRECTION('ref_axis',(0.,1.,0.));
#25780=DIRECTION('center_axis',(1.,0.,0.));
#25781=DIRECTION('ref_axis',(0.,0.,-1.));
#25782=DIRECTION('center_axis',(1.,0.,0.));
#25783=DIRECTION('ref_axis',(0.,1.,0.));
#25784=DIRECTION('center_axis',(1.,0.,0.));
#25785=DIRECTION('ref_axis',(0.,0.,-1.));
#25786=DIRECTION('center_axis',(-1.,0.,0.));
#25787=DIRECTION('ref_axis',(0.,1.,0.));
#25788=DIRECTION('',(1.,0.,0.));
#25789=DIRECTION('center_axis',(1.,0.,0.));
#25790=DIRECTION('ref_axis',(0.,-0.576970076999607,-0.816765284673061));
#25791=DIRECTION('',(1.,0.,0.));
#25792=DIRECTION('center_axis',(1.,0.,0.));
#25793=DIRECTION('ref_axis',(0.,1.,0.));
#25794=DIRECTION('center_axis',(1.,0.,0.));
#25795=DIRECTION('ref_axis',(0.,0.,-1.));
#25796=DIRECTION('center_axis',(1.,0.,0.));
#25797=DIRECTION('ref_axis',(0.,1.,0.));
#25798=DIRECTION('center_axis',(1.,0.,0.));
#25799=DIRECTION('ref_axis',(0.,0.,-1.));
#25800=DIRECTION('center_axis',(-1.,0.,0.));
#25801=DIRECTION('ref_axis',(0.,1.,0.));
#25802=DIRECTION('',(1.,0.,0.));
#25803=DIRECTION('center_axis',(1.,0.,0.));
#25804=DIRECTION('ref_axis',(0.,-0.761964767542423,-0.64761847798223));
#25805=DIRECTION('',(1.,0.,0.));
#25806=DIRECTION('center_axis',(1.,0.,0.));
#25807=DIRECTION('ref_axis',(0.,1.,0.));
#25808=DIRECTION('center_axis',(1.,0.,0.));
#25809=DIRECTION('ref_axis',(0.,0.,-1.));
#25810=DIRECTION('center_axis',(1.,0.,0.));
#25811=DIRECTION('ref_axis',(0.,1.,0.));
#25812=DIRECTION('center_axis',(1.,0.,0.));
#25813=DIRECTION('ref_axis',(0.,0.,-1.));
#25814=DIRECTION('center_axis',(-1.,0.,0.));
#25815=DIRECTION('ref_axis',(0.,1.,0.));
#25816=DIRECTION('',(1.,0.,0.));
#25817=DIRECTION('center_axis',(1.,0.,0.));
#25818=DIRECTION('ref_axis',(0.,-0.899082409430159,-0.437779420545621));
#25819=DIRECTION('',(1.,0.,0.));
#25820=DIRECTION('center_axis',(1.,0.,0.));
#25821=DIRECTION('ref_axis',(0.,1.,0.));
#25822=DIRECTION('center_axis',(1.,0.,0.));
#25823=DIRECTION('ref_axis',(0.,0.,-1.));
#25824=DIRECTION('center_axis',(1.,0.,0.));
#25825=DIRECTION('ref_axis',(0.,1.,0.));
#25826=DIRECTION('center_axis',(1.,0.,0.));
#25827=DIRECTION('ref_axis',(0.,0.,-1.));
#25828=DIRECTION('center_axis',(-1.,0.,0.));
#25829=DIRECTION('ref_axis',(0.,1.,0.));
#25830=DIRECTION('',(1.,0.,0.));
#25831=DIRECTION('center_axis',(1.,0.,0.));
#25832=DIRECTION('ref_axis',(0.,-0.979707396939596,-0.200433072076046));
#25833=DIRECTION('',(1.,0.,0.));
#25834=DIRECTION('center_axis',(1.,0.,0.));
#25835=DIRECTION('ref_axis',(0.,1.,0.));
#25836=DIRECTION('center_axis',(1.,0.,0.));
#25837=DIRECTION('ref_axis',(0.,0.,-1.));
#25838=DIRECTION('center_axis',(1.,0.,0.));
#25839=DIRECTION('ref_axis',(0.,1.,0.));
#25840=DIRECTION('center_axis',(1.,0.,0.));
#25841=DIRECTION('ref_axis',(0.,0.,-1.));
#25842=DIRECTION('center_axis',(-1.,0.,0.));
#25843=DIRECTION('ref_axis',(0.,1.,0.));
#25844=DIRECTION('',(1.,0.,0.));
#25845=DIRECTION('center_axis',(1.,0.,0.));
#25846=DIRECTION('ref_axis',(0.,-0.998773765587553,0.0495072234533422));
#25847=DIRECTION('',(1.,0.,0.));
#25848=DIRECTION('center_axis',(1.,0.,0.));
#25849=DIRECTION('ref_axis',(0.,1.,0.));
#25850=DIRECTION('center_axis',(1.,0.,0.));
#25851=DIRECTION('ref_axis',(0.,0.,-1.));
#25852=DIRECTION('center_axis',(1.,0.,0.));
#25853=DIRECTION('ref_axis',(0.,1.,0.));
#25854=DIRECTION('center_axis',(1.,0.,0.));
#25855=DIRECTION('ref_axis',(0.,0.,-1.));
#25856=DIRECTION('center_axis',(-1.,0.,0.));
#25857=DIRECTION('ref_axis',(0.,1.,0.));
#25858=DIRECTION('',(1.,0.,0.));
#25859=DIRECTION('center_axis',(1.,0.,0.));
#25860=DIRECTION('ref_axis',(0.,-0.955083505310682,0.296336798058325));
#25861=DIRECTION('',(1.,0.,0.));
#25862=DIRECTION('center_axis',(1.,0.,0.));
#25863=DIRECTION('ref_axis',(0.,1.,0.));
#25864=DIRECTION('center_axis',(1.,0.,0.));
#25865=DIRECTION('ref_axis',(0.,0.,-1.));
#25866=DIRECTION('center_axis',(1.,0.,0.));
#25867=DIRECTION('ref_axis',(0.,1.,0.));
#25868=DIRECTION('center_axis',(1.,0.,0.));
#25869=DIRECTION('ref_axis',(0.,0.,-1.));
#25870=DIRECTION('center_axis',(-1.,0.,0.));
#25871=DIRECTION('ref_axis',(0.,1.,0.));
#25872=DIRECTION('',(1.,0.,0.));
#25873=DIRECTION('center_axis',(1.,0.,0.));
#25874=DIRECTION('ref_axis',(0.,-0.851381835843715,0.524546441790797));
#25875=DIRECTION('',(1.,0.,0.));
#25876=DIRECTION('center_axis',(1.,0.,0.));
#25877=DIRECTION('ref_axis',(0.,1.,0.));
#25878=DIRECTION('center_axis',(1.,0.,0.));
#25879=DIRECTION('ref_axis',(0.,0.,-1.));
#25880=DIRECTION('center_axis',(1.,0.,0.));
#25881=DIRECTION('ref_axis',(0.,1.,0.));
#25882=DIRECTION('center_axis',(1.,0.,0.));
#25883=DIRECTION('ref_axis',(0.,0.,-1.));
#25884=DIRECTION('center_axis',(-1.,0.,0.));
#25885=DIRECTION('ref_axis',(0.,1.,0.));
#25886=DIRECTION('',(1.,0.,0.));
#25887=DIRECTION('center_axis',(1.,0.,0.));
#25888=DIRECTION('ref_axis',(0.,-0.694184714467323,0.719796903438686));
#25889=DIRECTION('',(1.,0.,0.));
#25890=DIRECTION('center_axis',(1.,0.,0.));
#25891=DIRECTION('ref_axis',(0.,1.,0.));
#25892=DIRECTION('center_axis',(1.,0.,0.));
#25893=DIRECTION('ref_axis',(0.,0.,-1.));
#25894=DIRECTION('center_axis',(1.,0.,0.));
#25895=DIRECTION('ref_axis',(0.,1.,0.));
#25896=DIRECTION('center_axis',(1.,0.,0.));
#25897=DIRECTION('ref_axis',(0.,0.,-1.));
#25898=DIRECTION('center_axis',(-1.,0.,0.));
#25899=DIRECTION('ref_axis',(0.,1.,0.));
#25900=DIRECTION('',(1.,0.,0.));
#25901=DIRECTION('center_axis',(1.,0.,0.));
#25902=DIRECTION('ref_axis',(0.,-0.493369414448157,0.869819878415688));
#25903=DIRECTION('',(1.,0.,0.));
#25904=DIRECTION('center_axis',(1.,0.,0.));
#25905=DIRECTION('ref_axis',(0.,1.,0.));
#25906=DIRECTION('center_axis',(1.,0.,0.));
#25907=DIRECTION('ref_axis',(0.,0.,-1.));
#25908=DIRECTION('center_axis',(1.,0.,0.));
#25909=DIRECTION('ref_axis',(0.,1.,0.));
#25910=DIRECTION('center_axis',(1.,0.,0.));
#25911=DIRECTION('ref_axis',(0.,0.,-1.));
#25912=DIRECTION('center_axis',(-1.,0.,0.));
#25913=DIRECTION('ref_axis',(0.,1.,0.));
#25914=DIRECTION('',(1.,0.,0.));
#25915=DIRECTION('center_axis',(1.,0.,0.));
#25916=DIRECTION('ref_axis',(0.,-0.261553899633433,0.965188871458091));
#25917=DIRECTION('',(1.,0.,0.));
#25918=DIRECTION('center_axis',(1.,0.,0.));
#25919=DIRECTION('ref_axis',(0.,1.,0.));
#25920=DIRECTION('center_axis',(1.,0.,0.));
#25921=DIRECTION('ref_axis',(0.,0.,-1.));
#25922=DIRECTION('center_axis',(1.,0.,0.));
#25923=DIRECTION('ref_axis',(0.,1.,0.));
#25924=DIRECTION('center_axis',(1.,0.,0.));
#25925=DIRECTION('ref_axis',(0.,0.,-1.));
#25926=DIRECTION('center_axis',(-1.,0.,0.));
#25927=DIRECTION('ref_axis',(0.,1.,0.));
#25928=DIRECTION('',(1.,0.,0.));
#25929=DIRECTION('center_axis',(1.,0.,0.));
#25930=DIRECTION('ref_axis',(0.,-0.0133039913767846,0.99991149799042));
#25931=DIRECTION('',(1.,0.,0.));
#25932=DIRECTION('center_axis',(1.,0.,0.));
#25933=DIRECTION('ref_axis',(0.,1.,0.));
#25934=DIRECTION('center_axis',(1.,0.,0.));
#25935=DIRECTION('ref_axis',(0.,0.,-1.));
#25936=DIRECTION('center_axis',(1.,0.,0.));
#25937=DIRECTION('ref_axis',(0.,1.,0.));
#25938=DIRECTION('center_axis',(1.,0.,0.));
#25939=DIRECTION('ref_axis',(0.,0.,-1.));
#25940=DIRECTION('center_axis',(-1.,0.,0.));
#25941=DIRECTION('ref_axis',(0.,1.,0.));
#25942=DIRECTION('',(1.,0.,0.));
#25943=DIRECTION('center_axis',(1.,0.,0.));
#25944=DIRECTION('ref_axis',(0.,0.235781855586725,0.971806007686761));
#25945=DIRECTION('',(1.,0.,0.));
#25946=DIRECTION('center_axis',(1.,0.,0.));
#25947=DIRECTION('ref_axis',(0.,1.,0.));
#25948=DIRECTION('center_axis',(1.,0.,0.));
#25949=DIRECTION('ref_axis',(0.,0.,-1.));
#25950=DIRECTION('center_axis',(1.,0.,0.));
#25951=DIRECTION('ref_axis',(0.,1.,0.));
#25952=DIRECTION('center_axis',(1.,0.,0.));
#25953=DIRECTION('ref_axis',(0.,0.,-1.));
#25954=DIRECTION('center_axis',(-1.,0.,0.));
#25955=DIRECTION('ref_axis',(0.,1.,0.));
#25956=DIRECTION('',(1.,0.,0.));
#25957=DIRECTION('center_axis',(1.,0.,0.));
#25958=DIRECTION('ref_axis',(0.,0.470052661418713,0.882638371867655));
#25959=DIRECTION('',(1.,0.,0.));
#25960=DIRECTION('center_axis',(1.,0.,0.));
#25961=DIRECTION('ref_axis',(0.,1.,0.));
#25962=DIRECTION('center_axis',(1.,0.,0.));
#25963=DIRECTION('ref_axis',(0.,0.,-1.));
#25964=DIRECTION('center_axis',(1.,0.,0.));
#25965=DIRECTION('ref_axis',(0.,1.,0.));
#25966=DIRECTION('center_axis',(1.,0.,0.));
#25967=DIRECTION('ref_axis',(0.,0.,-1.));
#25968=DIRECTION('center_axis',(-1.,0.,0.));
#25969=DIRECTION('ref_axis',(0.,1.,0.));
#25970=DIRECTION('',(1.,0.,0.));
#25971=DIRECTION('center_axis',(1.,0.,0.));
#25972=DIRECTION('ref_axis',(0.,0.674788329801001,0.738011321027242));
#25973=DIRECTION('',(1.,0.,0.));
#25974=DIRECTION('center_axis',(1.,0.,0.));
#25975=DIRECTION('ref_axis',(0.,1.,0.));
#25976=DIRECTION('center_axis',(1.,0.,0.));
#25977=DIRECTION('ref_axis',(0.,0.,-1.));
#25978=DIRECTION('center_axis',(1.,0.,0.));
#25979=DIRECTION('ref_axis',(0.,1.,0.));
#25980=DIRECTION('center_axis',(1.,0.,0.));
#25981=DIRECTION('ref_axis',(0.,0.,-1.));
#25982=DIRECTION('center_axis',(-1.,0.,0.));
#25983=DIRECTION('ref_axis',(0.,1.,0.));
#25984=DIRECTION('',(1.,0.,0.));
#25985=DIRECTION('center_axis',(1.,0.,0.));
#25986=DIRECTION('ref_axis',(0.,0.837124565724013,0.547012304670911));
#25987=DIRECTION('',(1.,0.,0.));
#25988=DIRECTION('center_axis',(1.,0.,0.));
#25989=DIRECTION('ref_axis',(0.,1.,0.));
#25990=DIRECTION('center_axis',(1.,0.,0.));
#25991=DIRECTION('ref_axis',(0.,0.,-1.));
#25992=DIRECTION('center_axis',(1.,0.,0.));
#25993=DIRECTION('ref_axis',(0.,1.,0.));
#25994=DIRECTION('center_axis',(1.,0.,0.));
#25995=DIRECTION('ref_axis',(0.,0.,-1.));
#25996=DIRECTION('center_axis',(-1.,0.,0.));
#25997=DIRECTION('ref_axis',(0.,1.,0.));
#25998=DIRECTION('',(1.,0.,0.));
#25999=DIRECTION('center_axis',(1.,0.,0.));
#26000=DIRECTION('ref_axis',(0.,0.946861186453793,0.321642493441576));
#26001=DIRECTION('',(1.,0.,0.));
#26002=DIRECTION('center_axis',(1.,0.,0.));
#26003=DIRECTION('ref_axis',(0.,1.,0.));
#26004=DIRECTION('center_axis',(1.,0.,0.));
#26005=DIRECTION('ref_axis',(0.,0.,-1.));
#26006=DIRECTION('center_axis',(1.,0.,0.));
#26007=DIRECTION('ref_axis',(0.,1.,0.));
#26008=DIRECTION('center_axis',(1.,0.,0.));
#26009=DIRECTION('ref_axis',(0.,0.,-1.));
#26010=DIRECTION('center_axis',(-1.,0.,0.));
#26011=DIRECTION('ref_axis',(0.,1.,0.));
#26012=DIRECTION('',(1.,0.,0.));
#26013=DIRECTION('center_axis',(1.,0.,0.));
#26014=DIRECTION('ref_axis',(0.,0.99710303652683,0.0760627014309627));
#26015=DIRECTION('',(1.,0.,0.));
#26016=DIRECTION('center_axis',(1.,0.,0.));
#26017=DIRECTION('ref_axis',(0.,1.,0.));
#26018=DIRECTION('center_axis',(1.,0.,0.));
#26019=DIRECTION('ref_axis',(0.,0.,-1.));
#26020=DIRECTION('center_axis',(1.,0.,0.));
#26021=DIRECTION('ref_axis',(0.,1.,0.));
#26022=DIRECTION('center_axis',(1.,0.,0.));
#26023=DIRECTION('ref_axis',(0.,0.,-1.));
#26024=DIRECTION('center_axis',(-1.,0.,0.));
#26025=DIRECTION('ref_axis',(0.,1.,0.));
#26026=DIRECTION('center_axis',(1.,0.,0.));
#26027=DIRECTION('ref_axis',(0.,1.,0.));
#26028=DIRECTION('center_axis',(1.,0.,0.));
#26029=DIRECTION('ref_axis',(0.,0.,-1.));
#26030=DIRECTION('center_axis',(-1.,0.,0.));
#26031=DIRECTION('ref_axis',(0.,1.,0.));
#49227=CARTESIAN_POINT('',(0.,0.,0.));
#49228=CARTESIAN_POINT('Origin',(-21.15,0.,0.));
#49229=CARTESIAN_POINT('',(-21.3,3.03,-3.71067980141648E-16));
#49230=CARTESIAN_POINT('',(-21.3,-3.03,-3.71067980141648E-16));
#49231=CARTESIAN_POINT('Origin',(-21.3,0.,0.));
#49232=CARTESIAN_POINT('Origin',(-21.3,0.,0.));
#49233=CARTESIAN_POINT('',(-21.,3.33,4.07807384116069E-16));
#49234=CARTESIAN_POINT('',(-21.15,3.18,-3.89437682128858E-16));
#49235=CARTESIAN_POINT('Origin',(-21.,0.,0.));
#49236=CARTESIAN_POINT('Origin',(-43.5,0.,0.));
#49237=CARTESIAN_POINT('',(-65.7,-3.03,-3.71067980141648E-16));
#49238=CARTESIAN_POINT('',(-43.5,-3.03,-3.71067980141648E-16));
#49239=CARTESIAN_POINT('',(-65.7,3.03,3.71067980141648E-16));
#49240=CARTESIAN_POINT('Origin',(-65.7,0.,0.));
#49241=CARTESIAN_POINT('Origin',(-65.7,0.,0.));
#49242=CARTESIAN_POINT('Origin',(-21.,3.03,0.));
#49243=CARTESIAN_POINT('',(-21.,8.83189477299562,-3.49966208636385));
#49244=CARTESIAN_POINT('',(-21.,6.8122671513043,-2.29198004120026));
#49245=CARTESIAN_POINT('Ctrl Pts',(-21.,8.83189477299562,-3.49966208636385));
#49246=CARTESIAN_POINT('Ctrl Pts',(-21.,8.82094392654054,-3.48448547507508));
#49247=CARTESIAN_POINT('Ctrl Pts',(-21.,8.7936907445869,-3.44793862615663));
#49248=CARTESIAN_POINT('Ctrl Pts',(-21.,8.74934377286772,-3.39315507789778));
#49249=CARTESIAN_POINT('Ctrl Pts',(-21.,8.68667704834295,-3.32467389681987));
#49250=CARTESIAN_POINT('Ctrl Pts',(-21.,8.60460841273967,-3.24456764186082));
#49251=CARTESIAN_POINT('Ctrl Pts',(-21.,8.51516539363766,-3.16038325236223));
#49252=CARTESIAN_POINT('Ctrl Pts',(-21.,8.4243384303954,-3.07426635319921));
#49253=CARTESIAN_POINT('Ctrl Pts',(-21.,8.33184183835821,-2.98721060740199));
#49254=CARTESIAN_POINT('Ctrl Pts',(-21.,8.2370828133169,-2.90227874531213));
#49255=CARTESIAN_POINT('Ctrl Pts',(-21.,8.13939365460193,-2.82329483425037));
#49256=CARTESIAN_POINT('Ctrl Pts',(-21.,8.03835937937461,-2.75296659957235));
#49257=CARTESIAN_POINT('Ctrl Pts',(-21.,7.93399262158453,-2.69188736687836));
#49258=CARTESIAN_POINT('Ctrl Pts',(-21.,7.82659266808561,-2.63932460382938));
#49259=CARTESIAN_POINT('Ctrl Pts',(-21.,7.71666617412861,-2.59365833862295));
#49260=CARTESIAN_POINT('Ctrl Pts',(-21.,7.60482241577417,-2.55297760756074));
#49261=CARTESIAN_POINT('Ctrl Pts',(-21.,7.49168859641892,-2.51552733857386));
#49262=CARTESIAN_POINT('Ctrl Pts',(-21.,7.37786505179862,-2.47974127678492));
#49263=CARTESIAN_POINT('Ctrl Pts',(-21.,7.26387759821705,-2.44432136933076));
#49264=CARTESIAN_POINT('Ctrl Pts',(-21.,7.15012820840451,-2.4083053284885));
#49265=CARTESIAN_POINT('Ctrl Pts',(-21.,7.03685278876406,-2.37112767623027));
#49266=CARTESIAN_POINT('Ctrl Pts',(-21.,6.94670492800217,-2.3402328805745));
#49267=CARTESIAN_POINT('Ctrl Pts',(-21.,6.8793763726903,-2.31637371632821));
#49268=CARTESIAN_POINT('Ctrl Pts',(-21.,6.83461600336474,-2.30016217089616));
#49269=CARTESIAN_POINT('Ctrl Pts',(-21.,6.8122671513043,-2.29198004120026));
#49270=CARTESIAN_POINT('',(-21.,7.13209349341826,-0.890729280500487));
#49271=CARTESIAN_POINT('Origin',(-21.,0.,0.));
#49272=CARTESIAN_POINT('',(-21.,9.47665840807863,-0.665541446186862));
#49273=CARTESIAN_POINT('Ctrl Pts',(-21.,7.13209349341826,-0.890729280500493));
#49274=CARTESIAN_POINT('Ctrl Pts',(-21.,7.15211036864424,-0.892482057440589));
#49275=CARTESIAN_POINT('Ctrl Pts',(-21.,7.19212249719958,-0.896150298874621));
#49276=CARTESIAN_POINT('Ctrl Pts',(-21.,7.25207582250743,-0.902140734147995));
#49277=CARTESIAN_POINT('Ctrl Pts',(-21.,7.33188369780814,-0.9111053356665));
#49278=CARTESIAN_POINT('Ctrl Pts',(-21.,7.43143474677318,-0.923884053007732));
#49279=CARTESIAN_POINT('Ctrl Pts',(-21.,7.53080214904746,-0.938052795086853));
#49280=CARTESIAN_POINT('Ctrl Pts',(-21.,7.63003710778607,-0.953237934402832));
#49281=CARTESIAN_POINT('Ctrl Pts',(-21.,7.7292275500742,-0.968799418422936));
#49282=CARTESIAN_POINT('Ctrl Pts',(-21.,7.82850348500033,-0.983785216334556));
#49283=CARTESIAN_POINT('Ctrl Pts',(-21.,7.92800888935854,-0.997080466154163));
#49284=CARTESIAN_POINT('Ctrl Pts',(-21.,8.02787639670185,-1.00753800115478));
#49285=CARTESIAN_POINT('Ctrl Pts',(-21.,8.12820273854248,-1.01410892133532));
#49286=CARTESIAN_POINT('Ctrl Pts',(-21.,8.2290192302709,-1.01599010763451));
#49287=CARTESIAN_POINT('Ctrl Pts',(-21.,8.33027821569813,-1.01271355471894));
#49288=CARTESIAN_POINT('Ctrl Pts',(-21.,8.43188165539955,-1.00407739851957));
#49289=CARTESIAN_POINT('Ctrl Pts',(-21.,8.53370212161309,-0.990109101007578));
#49290=CARTESIAN_POINT('Ctrl Pts',(-21.,8.63560512714608,-0.971017102543952));
#49291=CARTESIAN_POINT('Ctrl Pts',(-21.,8.73747423363077,-0.947150867813171));
#49292=CARTESIAN_POINT('Ctrl Pts',(-21.,8.83922276353739,-0.91895289219465));
#49293=CARTESIAN_POINT('Ctrl Pts',(-21.,8.94078425956014,-0.886903960171006));
#49294=CARTESIAN_POINT('Ctrl Pts',(-21.,9.04210805084257,-0.851468211346448));
#49295=CARTESIAN_POINT('Ctrl Pts',(-21.,9.14315312384119,-0.813043722977556));
#49296=CARTESIAN_POINT('Ctrl Pts',(-21.,9.24388219451327,-0.771898853704204));
#49297=CARTESIAN_POINT('Ctrl Pts',(-21.,9.33073157135268,-0.734052451290808));
#49298=CARTESIAN_POINT('Ctrl Pts',(-21.,9.39728977570677,-0.703536138917769));
#49299=CARTESIAN_POINT('Ctrl Pts',(-21.,9.44372410361834,-0.681495939481608));
#49300=CARTESIAN_POINT('Ctrl Pts',(-21.,9.47015861118831,-0.668702181892299));
#49301=CARTESIAN_POINT('Ctrl Pts',(-21.,9.47665840807863,-0.665541446186862));
#49302=CARTESIAN_POINT('',(-21.,9.47570870673866,0.678928939607903));
#49303=CARTESIAN_POINT('Origin',(-21.,0.,0.));
#49304=CARTESIAN_POINT('',(-21.,7.13209349341826,0.890729280500491));
#49305=CARTESIAN_POINT('Ctrl Pts',(-21.,9.47570870673866,0.678928939607903));
#49306=CARTESIAN_POINT('Ctrl Pts',(-21.,9.45925745015235,0.687851199692914));
#49307=CARTESIAN_POINT('Ctrl Pts',(-21.,9.41884609819914,0.708954060299467));
#49308=CARTESIAN_POINT('Ctrl Pts',(-21.,9.35512116653373,0.739070901845868));
#49309=CARTESIAN_POINT('Ctrl Pts',(-21.,9.26894752777823,0.773580241279191));
#49310=CARTESIAN_POINT('Ctrl Pts',(-21.,9.1602494406401,0.810145236641718));
#49311=CARTESIAN_POINT('Ctrl Pts',(-21.,9.04313782728701,0.847184879177382));
#49312=CARTESIAN_POINT('Ctrl Pts',(-21.,8.92394083882956,0.885365181899305));
#49313=CARTESIAN_POINT('Ctrl Pts',(-21.,8.80283221651881,0.923666931425907));
#49314=CARTESIAN_POINT('Ctrl Pts',(-21.,8.68060673111004,0.95907349496179));
#49315=CARTESIAN_POINT('Ctrl Pts',(-21.,8.55832200571467,0.987849802439111));
#49316=CARTESIAN_POINT('Ctrl Pts',(-21.,8.43677899171613,1.00737622330388));
#49317=CARTESIAN_POINT('Ctrl Pts',(-21.,8.31624650623966,1.017123671327));
#49318=CARTESIAN_POINT('Ctrl Pts',(-21.,8.19667636355292,1.01788199103989));
#49319=CARTESIAN_POINT('Ctrl Pts',(-21.,8.0778221648407,1.01133055607812));
#49320=CARTESIAN_POINT('Ctrl Pts',(-21.,7.95940371279084,0.999455440216893));
#49321=CARTESIAN_POINT('Ctrl Pts',(-21.,7.84122460090589,0.984110042106143));
#49322=CARTESIAN_POINT('Ctrl Pts',(-21.,7.72314614047142,0.966965984543333));
#49323=CARTESIAN_POINT('Ctrl Pts',(-21.,7.60507887157754,0.949420915891057));
#49324=CARTESIAN_POINT('Ctrl Pts',(-21.,7.4869674381447,0.932516236860827));
#49325=CARTESIAN_POINT('Ctrl Pts',(-21.,7.36877903277666,0.916863781503487));
#49326=CARTESIAN_POINT('Ctrl Pts',(-21.,7.27415386726379,0.90558533966873));
#49327=CARTESIAN_POINT('Ctrl Pts',(-21.,7.20314083161155,0.897868938540711));
#49328=CARTESIAN_POINT('Ctrl Pts',(-21.,7.15577920638447,0.893054239868309));
#49329=CARTESIAN_POINT('Ctrl Pts',(-21.,7.13209349341826,0.890729280500491));
#49330=CARTESIAN_POINT('',(-21.,6.8122671513043,2.29198004120026));
#49331=CARTESIAN_POINT('Origin',(-21.,0.,0.));
#49332=CARTESIAN_POINT('',(-21.,8.82694180863381,3.51213586112388));
#49333=CARTESIAN_POINT('Ctrl Pts',(-21.,6.8122671513043,2.29198004120026));
#49334=CARTESIAN_POINT('Ctrl Pts',(-21.,6.8310622341282,2.29908584041335));
#49335=CARTESIAN_POINT('Ctrl Pts',(-21.,6.86870350660446,2.31314148102898));
#49336=CARTESIAN_POINT('Ctrl Pts',(-21.,6.92531873868941,2.33375705829959));
#49337=CARTESIAN_POINT('Ctrl Pts',(-21.,7.00111274457534,2.36030757076476));
#49338=CARTESIAN_POINT('Ctrl Pts',(-21.,7.09634961812101,2.39198792562662));
#49339=CARTESIAN_POINT('Ctrl Pts',(-21.,7.19202414084635,2.42233623016115));
#49340=CARTESIAN_POINT('Ctrl Pts',(-21.,7.28802033430286,2.45171132733138));
#49341=CARTESIAN_POINT('Ctrl Pts',(-21.,7.3841397096708,2.4807280346756));
#49342=CARTESIAN_POINT('Ctrl Pts',(-21.,7.4800863304027,2.5103005111467));
#49343=CARTESIAN_POINT('Ctrl Pts',(-21.,7.57550619462173,2.54149568187359));
#49344=CARTESIAN_POINT('Ctrl Pts',(-21.,7.67002106404108,2.5754046559055));
#49345=CARTESIAN_POINT('Ctrl Pts',(-21.,7.76326299008741,2.61301442971916));
#49346=CARTESIAN_POINT('Ctrl Pts',(-21.,7.85491172665132,2.65506217582471));
#49347=CARTESIAN_POINT('Ctrl Pts',(-21.,7.94472127708621,2.70194887521209));
#49348=CARTESIAN_POINT('Ctrl Pts',(-21.,8.03251572538561,2.75381386341092));
#49349=CARTESIAN_POINT('Ctrl Pts',(-21.,8.11819217840571,2.81057710920625));
#49350=CARTESIAN_POINT('Ctrl Pts',(-21.,8.201719906256,2.87199246251599));
#49351=CARTESIAN_POINT('Ctrl Pts',(-21.,8.28314562863609,2.93769454582461));
#49352=CARTESIAN_POINT('Ctrl Pts',(-21.,8.36258324333989,3.00724707660037));
#49353=CARTESIAN_POINT('Ctrl Pts',(-21.,8.44018147897284,3.08018804824792));
#49354=CARTESIAN_POINT('Ctrl Pts',(-21.,8.51609606529771,3.15607730017284));
#49355=CARTESIAN_POINT('Ctrl Pts',(-21.,8.59046276963722,3.23453838205034));
#49356=CARTESIAN_POINT('Ctrl Pts',(-21.,8.66336443667969,3.31531333416059));
#49357=CARTESIAN_POINT('Ctrl Pts',(-21.,8.72519208281745,3.38709429686028));
#49358=CARTESIAN_POINT('Ctrl Pts',(-21.,8.77191842112748,3.44346706684567));
#49359=CARTESIAN_POINT('Ctrl Pts',(-21.,8.80419142083552,3.4834717001977));
#49360=CARTESIAN_POINT('Ctrl Pts',(-21.,8.82245708581418,3.50646798047534));
#49361=CARTESIAN_POINT('Ctrl Pts',(-21.,8.82694180863381,3.51213586112388));
#49362=CARTESIAN_POINT('',(-21.,8.24274231917123,4.72304976257329));
#49363=CARTESIAN_POINT('Origin',(-21.,0.,0.));
#49364=CARTESIAN_POINT('',(-21.,6.03932124977421,3.89701874412038));
#49365=CARTESIAN_POINT('Ctrl Pts',(-21.,8.24274231917123,4.72304976257329));
#49366=CARTESIAN_POINT('Ctrl Pts',(-21.,8.22404902558203,4.72395050842036));
#49367=CARTESIAN_POINT('Ctrl Pts',(-21.,8.17848346749629,4.7254297003623));
#49368=CARTESIAN_POINT('Ctrl Pts',(-21.,8.10800208013598,4.72491482536916));
#49369=CARTESIAN_POINT('Ctrl Pts',(-21.,8.0153892731556,4.71861732525386));
#49370=CARTESIAN_POINT('Ctrl Pts',(-21.,7.9015907237349,4.70439891524807));
#49371=CARTESIAN_POINT('Ctrl Pts',(-21.,7.78000590743498,4.68695765535521));
#49372=CARTESIAN_POINT('Ctrl Pts',(-21.,7.65604731918147,4.66963928443128));
#49373=CARTESIAN_POINT('Ctrl Pts',(-21.,7.53031371454558,4.65160090645339));
#49374=CARTESIAN_POINT('Ctrl Pts',(-21.,7.40483002515176,4.63046946729401));
#49375=CARTESIAN_POINT('Ctrl Pts',(-21.,7.28216972266428,4.60333867057275));
#49376=CARTESIAN_POINT('Ctrl Pts',(-21.,7.16419105444418,4.56819583049617));
#49377=CARTESIAN_POINT('Ctrl Pts',(-21.,7.05136577826386,4.52468089222283));
#49378=CARTESIAN_POINT('Ctrl Pts',(-21.,6.94330777957998,4.47348457408032));
#49379=CARTESIAN_POINT('Ctrl Pts',(-21.,6.83906640781858,4.4160130309926));
#49380=CARTESIAN_POINT('Ctrl Pts',(-21.,6.73752748880879,4.35393408054299));
#49381=CARTESIAN_POINT('Ctrl Pts',(-21.,6.63770990687462,4.2888323596294));
#49382=CARTESIAN_POINT('Ctrl Pts',(-21.,6.53876341785232,4.22215377357323));
#49383=CARTESIAN_POINT('Ctrl Pts',(-21.,6.44000100425059,4.15511874483725));
#49384=CARTESIAN_POINT('Ctrl Pts',(-21.,6.34092094513049,4.08864152493875));
#49385=CARTESIAN_POINT('Ctrl Pts',(-21.,6.24122821720367,4.02325912271413));
#49386=CARTESIAN_POINT('Ctrl Pts',(-21.,6.16086742147114,3.97204127711522));
#49387=CARTESIAN_POINT('Ctrl Pts',(-21.,6.10023490810719,3.93427763849175));
#49388=CARTESIAN_POINT('Ctrl Pts',(-21.,6.05965257770704,3.90939030583537));
#49389=CARTESIAN_POINT('Ctrl Pts',(-21.,6.03932124977421,3.89701874412038));
#49390=CARTESIAN_POINT('',(-21.,5.14318775290069,5.02073460645077));
#49391=CARTESIAN_POINT('Origin',(-21.,0.,0.));
#49392=CARTESIAN_POINT('',(-21.,6.42894112865204,6.99419158761942));
#49393=CARTESIAN_POINT('Ctrl Pts',(-21.,5.14318775290069,5.02073460645076));
#49394=CARTESIAN_POINT('Ctrl Pts',(-21.,5.15703844666268,5.03529159113598));
#49395=CARTESIAN_POINT('Ctrl Pts',(-21.,5.18485354740602,5.06428722179623));
#49396=CARTESIAN_POINT('Ctrl Pts',(-21.,5.22691734521339,5.10742564369892));
#49397=CARTESIAN_POINT('Ctrl Pts',(-21.,5.28368554926634,5.16423261553338));
#49398=CARTESIAN_POINT('Ctrl Pts',(-21.,5.35574541658332,5.23409735978387));
#49399=CARTESIAN_POINT('Ctrl Pts',(-21.,5.42877754716296,5.30295185702147));
#49400=CARTESIAN_POINT('Ctrl Pts',(-21.,5.50252175190725,5.37106909242141));
#49401=CARTESIAN_POINT('Ctrl Pts',(-21.,5.57653243923659,5.43891687637388));
#49402=CARTESIAN_POINT('Ctrl Pts',(-21.,5.65014634083023,5.50719043557996));
#49403=CARTESIAN_POINT('Ctrl Pts',(-21.,5.72258159055366,5.57669744070723));
#49404=CARTESIAN_POINT('Ctrl Pts',(-21.,5.79302399301176,5.64825683559838));
#49405=CARTESIAN_POINT('Ctrl Pts',(-21.,5.86071379627312,5.72259822644884));
#49406=CARTESIAN_POINT('Ctrl Pts',(-21.,5.92504262139805,5.80024683316115));
#49407=CARTESIAN_POINT('Ctrl Pts',(-21.,5.98561485393513,5.88145719317904));
#49408=CARTESIAN_POINT('Ctrl Pts',(-21.,6.04221154361855,5.96627851638222));
#49409=CARTESIAN_POINT('Ctrl Pts',(-21.,6.09477471117184,6.05459405347559));
#49410=CARTESIAN_POINT('Ctrl Pts',(-21.,6.14338347043832,6.14616869769857));
#49411=CARTESIAN_POINT('Ctrl Pts',(-21.,6.18823844577549,6.2406935262026));
#49412=CARTESIAN_POINT('Ctrl Pts',(-21.,6.22963155144596,6.33782488040965));
#49413=CARTESIAN_POINT('Ctrl Pts',(-21.,6.2678972444421,6.43721103768399));
#49414=CARTESIAN_POINT('Ctrl Pts',(-21.,6.30336681095649,6.53852299564495));
#49415=CARTESIAN_POINT('Ctrl Pts',(-21.,6.33632590879467,6.64148049150319));
#49416=CARTESIAN_POINT('Ctrl Pts',(-21.,6.36696110296949,6.74588705654512));
#49417=CARTESIAN_POINT('Ctrl Pts',(-21.,6.3915212948217,6.8373854795327));
#49418=CARTESIAN_POINT('Ctrl Pts',(-21.,6.40916104272443,6.90844938866819));
#49419=CARTESIAN_POINT('Ctrl Pts',(-21.,6.42088065083439,6.95849504767608));
#49420=CARTESIAN_POINT('Ctrl Pts',(-21.,6.42735973425904,6.98713915530221));
#49421=CARTESIAN_POINT('Ctrl Pts',(-21.,6.42894112865204,6.99419158761942));
#49422=CARTESIAN_POINT('',(-21.,5.37719972469147,7.83171265565699));
#49423=CARTESIAN_POINT('Origin',(-21.,0.,0.));
#49424=CARTESIAN_POINT('',(-21.,3.75038736519793,6.13145585166881));
#49425=CARTESIAN_POINT('Ctrl Pts',(-21.,5.37719972469147,7.83171265565699));
#49426=CARTESIAN_POINT('Ctrl Pts',(-21.,5.35996683015292,7.82441348350419));
#49427=CARTESIAN_POINT('Ctrl Pts',(-21.,5.31827188353843,7.80597603467631));
#49428=CARTESIAN_POINT('Ctrl Pts',(-21.,5.25499374364742,7.77493142045055));
#49429=CARTESIAN_POINT('Ctrl Pts',(-21.,5.17428487068616,7.72907437791822));
#49430=CARTESIAN_POINT('Ctrl Pts',(-21.,5.07792505734327,7.66688869302314));
#49431=CARTESIAN_POINT('Ctrl Pts',(-21.,4.97594840210465,7.59842098612655));
#49432=CARTESIAN_POINT('Ctrl Pts',(-21.,4.87177973271099,7.52903405731413));
#49433=CARTESIAN_POINT('Ctrl Pts',(-21.,4.76632422816958,7.45822827381644));
#49434=CARTESIAN_POINT('Ctrl Pts',(-21.,4.66243591843161,7.38474417264741));
#49435=CARTESIAN_POINT('Ctrl Pts',(-21.,4.56369441608956,7.30707985875561));
#49436=CARTESIAN_POINT('Ctrl Pts',(-21.,4.4726472158023,7.22422822821349));
#49437=CARTESIAN_POINT('Ctrl Pts',(-21.,4.38987557857684,7.13606957084443));
#49438=CARTESIAN_POINT('Ctrl Pts',(-21.,4.31473193577955,7.04305867353628));
#49439=CARTESIAN_POINT('Ctrl Pts',(-21.,4.24574967308284,6.94604996627335));
#49440=CARTESIAN_POINT('Ctrl Pts',(-21.,4.18120131531612,6.84606267872027));
#49441=CARTESIAN_POINT('Ctrl Pts',(-21.,4.11951535961712,6.74409882925098));
#49442=CARTESIAN_POINT('Ctrl Pts',(-21.,4.05929840765689,6.64109222642907));
#49443=CARTESIAN_POINT('Ctrl Pts',(-21.,3.99940195660266,6.53784434718121));
#49444=CARTESIAN_POINT('Ctrl Pts',(-21.,3.93897729264122,6.43496121510494));
#49445=CARTESIAN_POINT('Ctrl Pts',(-21.,3.87752560957259,6.33279865263617));
#49446=CARTESIAN_POINT('Ctrl Pts',(-21.,3.82734562477572,6.25178572573963));
#49447=CARTESIAN_POINT('Ctrl Pts',(-21.,3.78910264658076,6.19145440139071));
#49448=CARTESIAN_POINT('Ctrl Pts',(-21.,3.7633374392529,6.15142367620606));
#49449=CARTESIAN_POINT('Ctrl Pts',(-21.,3.75038736519793,6.13145585166881));
#49450=CARTESIAN_POINT('',(-21.,2.45543694297674,6.75507110762463));
#49451=CARTESIAN_POINT('Origin',(-21.,0.,0.));
#49452=CARTESIAN_POINT('',(-21.,2.75760981235205,9.09096189205629));
#49453=CARTESIAN_POINT('Ctrl Pts',(-21.,2.45543694297675,6.75507110762463));
#49454=CARTESIAN_POINT('Ctrl Pts',(-21.,2.46159994790965,6.77419608843537));
#49455=CARTESIAN_POINT('Ctrl Pts',(-21.,2.47407975508802,6.8123887688799));
#49456=CARTESIAN_POINT('Ctrl Pts',(-21.,2.49326086758344,6.8695059418988));
#49457=CARTESIAN_POINT('Ctrl Pts',(-21.,2.5197596307744,6.94531805563895));
#49458=CARTESIAN_POINT('Ctrl Pts',(-21.,2.55437015138428,7.03952961984441));
#49459=CARTESIAN_POINT('Ctrl Pts',(-21.,2.59029498067661,7.13325283216217));
#49460=CARTESIAN_POINT('Ctrl Pts',(-21.,2.62718125254576,7.22662075191781));
#49461=CARTESIAN_POINT('Ctrl Pts',(-21.,2.66442452752942,7.31986152676826));
#49462=CARTESIAN_POINT('Ctrl Pts',(-21.,2.70112557395893,7.41331375298832));
#49463=CARTESIAN_POINT('Ctrl Pts',(-21.,2.73622951961898,7.50736587770304));
#49464=CARTESIAN_POINT('Ctrl Pts',(-21.,2.76864747338962,7.60240247767684));
#49465=CARTESIAN_POINT('Ctrl Pts',(-21.,2.79737835816915,7.69875126136884));
#49466=CARTESIAN_POINT('Ctrl Pts',(-21.,2.82164615909785,7.79662146983088));
#49467=CARTESIAN_POINT('Ctrl Pts',(-21.,2.84098400021345,7.89607078269802));
#49468=CARTESIAN_POINT('Ctrl Pts',(-21.,2.85517326277626,7.9970485375799));
#49469=CARTESIAN_POINT('Ctrl Pts',(-21.,2.86421236488386,8.099424390731));
#49470=CARTESIAN_POINT('Ctrl Pts',(-21.,2.8682745946465,8.20302084448955));
#49471=CARTESIAN_POINT('Ctrl Pts',(-21.,2.86767474496505,8.30764661663281));
#49472=CARTESIAN_POINT('Ctrl Pts',(-21.,2.86282492937103,8.41311873833255));
#49473=CARTESIAN_POINT('Ctrl Pts',(-21.,2.85417908993455,8.51926543389428));
#49474=CARTESIAN_POINT('Ctrl Pts',(-21.,2.84217845398458,8.62593402210748));
#49475=CARTESIAN_POINT('Ctrl Pts',(-21.,2.82720199177778,8.73299593720093));
#49476=CARTESIAN_POINT('Ctrl Pts',(-21.,2.80950303716262,8.84035511450549));
#49477=CARTESIAN_POINT('Ctrl Pts',(-21.,2.79193132752196,8.93344861295375));
#49478=CARTESIAN_POINT('Ctrl Pts',(-21.,2.77699071660796,9.0051285824934));
#49479=CARTESIAN_POINT('Ctrl Pts',(-21.,2.76583572100211,9.05530311062091));
#49480=CARTESIAN_POINT('Ctrl Pts',(-21.,2.75924496093974,9.08392172878324));
#49481=CARTESIAN_POINT('Ctrl Pts',(-21.,2.75760981235205,9.09096189205629));
#49482=CARTESIAN_POINT('',(-21.,1.44663677770972,9.38920880763537));
#49483=CARTESIAN_POINT('Origin',(-21.,0.,0.));
#49484=CARTESIAN_POINT('',(-21.,0.718643267461623,7.15148293042304));
#49485=CARTESIAN_POINT('Ctrl Pts',(-21.,1.44663677770972,9.38920880763537));
#49486=CARTESIAN_POINT('Ctrl Pts',(-21.,1.43427746833275,9.37515540804603));
#49487=CARTESIAN_POINT('Ctrl Pts',(-21.,1.40471132872148,9.34045308130916));
#49488=CARTESIAN_POINT('Ctrl Pts',(-21.,1.36116944796064,9.28502749443539));
#49489=CARTESIAN_POINT('Ctrl Pts',(-21.,1.30834989113785,9.2086934591593));
#49490=CARTESIAN_POINT('Ctrl Pts',(-21.,1.24851405668088,9.11085713692575));
#49491=CARTESIAN_POINT('Ctrl Pts',(-21.,1.18634328973517,9.00492385207762));
#49492=CARTESIAN_POINT('Ctrl Pts',(-21.,1.12259642171968,8.89721129760285));
#49493=CARTESIAN_POINT('Ctrl Pts',(-21.,1.05830577327405,8.78766206238304));
#49494=CARTESIAN_POINT('Ctrl Pts',(-21.,0.996589197042052,8.67637972666424));
#49495=CARTESIAN_POINT('Ctrl Pts',(-21.,0.941323460369316,8.56356426545847));
#49496=CARTESIAN_POINT('Ctrl Pts',(-21.,0.895240742652423,8.44941362598824));
#49497=CARTESIAN_POINT('Ctrl Pts',(-21.,0.858916682261844,8.33407215281038));
#49498=CARTESIAN_POINT('Ctrl Pts',(-21.,0.831570515383446,8.21766862525226));
#49499=CARTESIAN_POINT('Ctrl Pts',(-21.,0.811510144890448,8.10033651802127));
#49500=CARTESIAN_POINT('Ctrl Pts',(-21.,0.796736942256154,7.98224460192821));
#49501=CARTESIAN_POINT('Ctrl Pts',(-21.,0.785400272847098,7.86361381479518));
#49502=CARTESIAN_POINT('Ctrl Pts',(-21.,0.775839563797132,7.74468091618948));
#49503=CARTESIAN_POINT('Ctrl Pts',(-21.,0.766672302003445,7.62566969516693));
#49504=CARTESIAN_POINT('Ctrl Pts',(-21.,0.756870878958096,7.5067579169994));
#49505=CARTESIAN_POINT('Ctrl Pts',(-21.,0.745831500234843,7.38804974272502));
#49506=CARTESIAN_POINT('Ctrl Pts',(-21.,0.735771087779772,7.29328733826105));
#49507=CARTESIAN_POINT('Ctrl Pts',(-21.,0.72749213560466,7.22233768688913));
#49508=CARTESIAN_POINT('Ctrl Pts',(-21.,0.721647166649911,7.17509214524366));
#49509=CARTESIAN_POINT('Ctrl Pts',(-21.,0.718643267461623,7.15148293042304));
#49510=CARTESIAN_POINT('',(-21.,-0.718643267461628,7.15148293042304));
#49511=CARTESIAN_POINT('Origin',(-21.,0.,0.));
#49512=CARTESIAN_POINT('',(-21.,-1.45989994714919,9.38715570044056));
#49513=CARTESIAN_POINT('Ctrl Pts',(-21.,-0.718643267461623,7.15148293042304));
#49514=CARTESIAN_POINT('Ctrl Pts',(-21.,-0.721388610069065,7.17138797035723));
#49515=CARTESIAN_POINT('Ctrl Pts',(-21.,-0.726715875322121,7.21121317182152));
#49516=CARTESIAN_POINT('Ctrl Pts',(-21.,-0.734216502709279,7.2709963393441));
#49517=CARTESIAN_POINT('Ctrl Pts',(-21.,-0.743235585416284,7.35079807608913));
#49518=CARTESIAN_POINT('Ctrl Pts',(-21.,-0.752929449590466,7.45069670452966));
#49519=CARTESIAN_POINT('Ctrl Pts',(-21.,-0.761227274615912,7.55072560028829));
#49520=CARTESIAN_POINT('Ctrl Pts',(-21.,-0.768504714146027,7.65085154280962));
#49521=CARTESIAN_POINT('Ctrl Pts',(-21.,-0.775405338877351,7.75101782957587));
#49522=CARTESIAN_POINT('Ctrl Pts',(-21.,-0.782886239966145,7.85113936329068));
#49523=CARTESIAN_POINT('Ctrl Pts',(-21.,-0.792066365329069,7.95110843081948));
#49524=CARTESIAN_POINT('Ctrl Pts',(-21.,-0.804093633570273,8.05079907170372));
#49525=CARTESIAN_POINT('Ctrl Pts',(-21.,-0.82001217136434,8.15007218998677));
#49526=CARTESIAN_POINT('Ctrl Pts',(-21.,-0.840611930230858,8.24877960511329));
#49527=CARTESIAN_POINT('Ctrl Pts',(-21.,-0.86633857713272,8.34677071475058));
#49528=CARTESIAN_POINT('Ctrl Pts',(-21.,-0.897367099160985,8.4439050185459));
#49529=CARTESIAN_POINT('Ctrl Pts',(-21.,-0.933642367528788,8.5400643944807));
#49530=CARTESIAN_POINT('Ctrl Pts',(-21.,-0.974931241694467,8.63516410958082));
#49531=CARTESIAN_POINT('Ctrl Pts',(-21.,-1.02086710880846,8.72916840803945));
#49532=CARTESIAN_POINT('Ctrl Pts',(-21.,-1.07099928020948,8.82209124999857));
#49533=CARTESIAN_POINT('Ctrl Pts',(-21.,-1.12484423754393,8.91397482898789));
#49534=CARTESIAN_POINT('Ctrl Pts',(-21.,-1.18193820283021,9.00487302535333));
#49535=CARTESIAN_POINT('Ctrl Pts',(-21.,-1.24188395306769,9.09483443436949));
#49536=CARTESIAN_POINT('Ctrl Pts',(-21.,-1.30441156144786,9.18388242219763));
#49537=CARTESIAN_POINT('Ctrl Pts',(-21.,-1.36063487998417,9.26013268702205));
#49538=CARTESIAN_POINT('Ctrl Pts',(-21.,-1.40519667848884,9.3182316199014));
#49539=CARTESIAN_POINT('Ctrl Pts',(-21.,-1.43701689412372,9.35859733650268));
#49540=CARTESIAN_POINT('Ctrl Pts',(-21.,-1.45537211681237,9.38152219688984));
#49541=CARTESIAN_POINT('Ctrl Pts',(-21.,-1.45989994714919,9.38715570044056));
#49542=CARTESIAN_POINT('',(-21.,-2.77045032493322,9.08705700417233));
#49543=CARTESIAN_POINT('Origin',(-21.,0.,0.));
#49544=CARTESIAN_POINT('',(-21.,-2.45543694297674,6.75507110762463));
#49545=CARTESIAN_POINT('Ctrl Pts',(-21.,-2.77045032493322,9.08705700417233));
#49546=CARTESIAN_POINT('Ctrl Pts',(-21.,-2.7754881363495,9.06903282528875));
#49547=CARTESIAN_POINT('Ctrl Pts',(-21.,-2.78706953240265,9.02493884204925));
#49548=CARTESIAN_POINT('Ctrl Pts',(-21.,-2.8022511505425,8.95610999975804));
#49549=CARTESIAN_POINT('Ctrl Pts',(-21.,-2.81671983020872,8.86441786360011));
#49550=CARTESIAN_POINT('Ctrl Pts',(-21.,-2.8281804649272,8.7503085875302));
#49551=CARTESIAN_POINT('Ctrl Pts',(-21.,-2.838231660712,8.62789111098118));
#49552=CARTESIAN_POINT('Ctrl Pts',(-21.,-2.84893087833482,8.50318672326558));
#49553=CARTESIAN_POINT('Ctrl Pts',(-21.,-2.85932311928695,8.37659160589212));
#49554=CARTESIAN_POINT('Ctrl Pts',(-21.,-2.8666442371861,8.24955186700095));
#49555=CARTESIAN_POINT('Ctrl Pts',(-21.,-2.86748815125169,8.12392974416385));
#49556=CARTESIAN_POINT('Ctrl Pts',(-21.,-2.85947913898695,8.00108902987832));
#49557=CARTESIAN_POINT('Ctrl Pts',(-21.,-2.84216119689693,7.88140953422486));
#49558=CARTESIAN_POINT('Ctrl Pts',(-21.,-2.81629364412744,7.76466852264525));
#49559=CARTESIAN_POINT('Ctrl Pts',(-21.,-2.78345892001629,7.65025207826714));
#49560=CARTESIAN_POINT('Ctrl Pts',(-21.,-2.74553095355499,7.53744508591865));
#49561=CARTESIAN_POINT('Ctrl Pts',(-21.,-2.70427297026251,7.42564364342468));
#49562=CARTESIAN_POINT('Ctrl Pts',(-21.,-2.66128382072048,7.31434056822034));
#49563=CARTESIAN_POINT('Ctrl Pts',(-21.,-2.61790620462629,7.20313763732345));
#49564=CARTESIAN_POINT('Ctrl Pts',(-21.,-2.57514309471485,7.09174914908801));
#49565=CARTESIAN_POINT('Ctrl Pts',(-21.,-2.53358368474749,6.98000697278327));
#49566=CARTESIAN_POINT('Ctrl Pts',(-21.,-2.50153193679118,6.89026394714059));
#49567=CARTESIAN_POINT('Ctrl Pts',(-21.,-2.47820711493347,6.82274841734025));
#49568=CARTESIAN_POINT('Ctrl Pts',(-21.,-2.46297417772978,6.77764561818537));
#49569=CARTESIAN_POINT('Ctrl Pts',(-21.,-2.45543694297674,6.75507110762463));
#49570=CARTESIAN_POINT('',(-21.,-3.75038736519794,6.13145585166881));
#49571=CARTESIAN_POINT('Origin',(-21.,0.,0.));
#49572=CARTESIAN_POINT('',(-21.,-5.38825861761966,7.82410819644306));
#49573=CARTESIAN_POINT('Ctrl Pts',(-21.,-3.75038736519793,6.13145585166881));
#49574=CARTESIAN_POINT('Ctrl Pts',(-21.,-3.7614973065729,6.1481985134482));
#49575=CARTESIAN_POINT('Ctrl Pts',(-21.,-3.78357651403939,6.1817683663582));
#49576=CARTESIAN_POINT('Ctrl Pts',(-21.,-3.81627329006595,6.23237673886416));
#49577=CARTESIAN_POINT('Ctrl Pts',(-21.,-3.859023878729,6.30036238594766));
#49578=CARTESIAN_POINT('Ctrl Pts',(-21.,-3.91110213900011,6.38616193008433));
#49579=CARTESIAN_POINT('Ctrl Pts',(-21.,-3.96197913233089,6.47268455970493));
#49580=CARTESIAN_POINT('Ctrl Pts',(-21.,-4.01197889710939,6.55973735411151));
#49581=CARTESIAN_POINT('Ctrl Pts',(-21.,-4.06165666819706,6.64698999124062));
#49582=CARTESIAN_POINT('Ctrl Pts',(-21.,-4.11183783259628,6.73395053478792));
#49583=CARTESIAN_POINT('Ctrl Pts',(-21.,-4.16348379256721,6.82003644526658));
#49584=CARTESIAN_POINT('Ctrl Pts',(-21.,-4.21757413484033,6.90463617300865));
#49585=CARTESIAN_POINT('Ctrl Pts',(-21.,-4.27498923356982,6.98717136730191));
#49586=CARTESIAN_POINT('Ctrl Pts',(-21.,-4.33637651734857,7.06716577496009));
#49587=CARTESIAN_POINT('Ctrl Pts',(-21.,-4.40207217433237,7.14429034032177));
#49588=CARTESIAN_POINT('Ctrl Pts',(-21.,-4.47217290162416,7.21834255288981));
#49589=CARTESIAN_POINT('Ctrl Pts',(-21.,-4.54657777868016,7.28923990788708));
#49590=CARTESIAN_POINT('Ctrl Pts',(-21.,-4.62503998887083,7.35700721943171));
#49591=CARTESIAN_POINT('Ctrl Pts',(-21.,-4.70721371156899,7.42177134000892));
#49592=CARTESIAN_POINT('Ctrl Pts',(-21.,-4.79269894740031,7.48374039375355));
#49593=CARTESIAN_POINT('Ctrl Pts',(-21.,-4.88107836846757,7.54316218647348));
#49594=CARTESIAN_POINT('Ctrl Pts',(-21.,-4.9719575030537,7.60028648840776));
#49595=CARTESIAN_POINT('Ctrl Pts',(-21.,-5.06499955030094,7.65532943098672));
#49596=CARTESIAN_POINT('Ctrl Pts',(-21.,-5.15997145275563,7.70842918324715));
#49597=CARTESIAN_POINT('Ctrl Pts',(-21.,-5.24371066241773,7.75273391435114));
#49598=CARTESIAN_POINT('Ctrl Pts',(-21.,-5.30906763780461,7.78574460437678));
#49599=CARTESIAN_POINT('Ctrl Pts',(-21.,-5.3552506895127,7.80830658422592));
#49600=CARTESIAN_POINT('Ctrl Pts',(-21.,-5.38173489786212,7.82099713708327));
#49601=CARTESIAN_POINT('Ctrl Pts',(-21.,-5.38825861761966,7.82410819644306));
#49602=CARTESIAN_POINT('',(-21.,-6.43881576337966,6.98510211559242));
#49603=CARTESIAN_POINT('Origin',(-21.,0.,0.));
#49604=CARTESIAN_POINT('',(-21.,-5.14318775290069,5.02073460645076));
#49605=CARTESIAN_POINT('Ctrl Pts',(-21.,-6.43881576337966,6.98510211559242));
#49606=CARTESIAN_POINT('Ctrl Pts',(-21.,-6.43553427649956,6.96667706709454));
#49607=CARTESIAN_POINT('Ctrl Pts',(-21.,-6.42683709146975,6.92192478151019));
#49608=CARTESIAN_POINT('Ctrl Pts',(-21.,-6.4106515413257,6.85332508014768));
#49609=CARTESIAN_POINT('Ctrl Pts',(-21.,-6.38390364438073,6.76443559520424));
#49610=CARTESIAN_POINT('Ctrl Pts',(-21.,-6.34471916009928,6.65665410688205));
#49611=CARTESIAN_POINT('Ctrl Pts',(-21.,-6.30066002212815,6.5419987212145));
#49612=CARTESIAN_POINT('Ctrl Pts',(-21.,-6.25619247809081,6.42500173364409));
#49613=CARTESIAN_POINT('Ctrl Pts',(-21.,-6.2106280007764,6.30643444970003));
#49614=CARTESIAN_POINT('Ctrl Pts',(-21.,-6.16210362315516,6.18879908596403));
#49615=CARTESIAN_POINT('Ctrl Pts',(-21.,-6.108358567083,6.07525130357771));
#49616=CARTESIAN_POINT('Ctrl Pts',(-21.,-6.04784410793973,5.96805062448362));
#49617=CARTESIAN_POINT('Ctrl Pts',(-21.,-5.98031419419066,5.86773709824143));
#49618=CARTESIAN_POINT('Ctrl Pts',(-21.,-5.906356307844,5.77378059171821));
#49619=CARTESIAN_POINT('Ctrl Pts',(-21.,-5.82712980893039,5.68494139022769));
#49620=CARTESIAN_POINT('Ctrl Pts',(-21.,-5.74401277228714,5.59976212994534));
#49621=CARTESIAN_POINT('Ctrl Pts',(-21.,-5.65833178588016,5.51693367893109));
#49622=CARTESIAN_POINT('Ctrl Pts',(-21.,-5.57130730604024,5.43530536621495));
#49623=CARTESIAN_POINT('Ctrl Pts',(-21.,-5.48397628091718,5.35393582972231));
#49624=CARTESIAN_POINT('Ctrl Pts',(-21.,-5.39711839642203,5.27213248760413));
#49625=CARTESIAN_POINT('Ctrl Pts',(-21.,-5.31119154860082,5.18948821771405));
#49626=CARTESIAN_POINT('Ctrl Pts',(-21.,-5.24337588200476,5.12253927774717));
#49627=CARTESIAN_POINT('Ctrl Pts',(-21.,-5.19306705314332,5.071830148219));
#49628=CARTESIAN_POINT('Ctrl Pts',(-21.,-5.1597732798141,5.03780325407688));
#49629=CARTESIAN_POINT('Ctrl Pts',(-21.,-5.14318775290069,5.02073460645076));
#49630=CARTESIAN_POINT('',(-21.,-6.03932124977422,3.89701874412038));
#49631=CARTESIAN_POINT('Origin',(-21.,0.,0.));
#49632=CARTESIAN_POINT('',(-21.,-8.24940658621529,4.71140010775012));
#49633=CARTESIAN_POINT('Ctrl Pts',(-21.,-6.03932124977421,3.89701874412039));
#49634=CARTESIAN_POINT('Ctrl Pts',(-21.,-6.0565953297729,3.90728293824429));
#49635=CARTESIAN_POINT('Ctrl Pts',(-21.,-6.09105342163039,3.92794852152394));
#49636=CARTESIAN_POINT('Ctrl Pts',(-21.,-6.14247034880463,3.95935849016754));
#49637=CARTESIAN_POINT('Ctrl Pts',(-21.,-6.21048516503746,4.00206265639536));
#49638=CARTESIAN_POINT('Ctrl Pts',(-21.,-6.29463308326085,4.05676946424956));
#49639=CARTESIAN_POINT('Ctrl Pts',(-21.,-6.37801243240243,4.11264895980536));
#49640=CARTESIAN_POINT('Ctrl Pts',(-21.,-6.46083145580807,4.1693867325325));
#49641=CARTESIAN_POINT('Ctrl Pts',(-21.,-6.54344708143028,4.22644426515767));
#49642=CARTESIAN_POINT('Ctrl Pts',(-21.,-6.62638951409907,4.28302021638686));
#49643=CARTESIAN_POINT('Ctrl Pts',(-21.,-6.71027219290964,4.33817259947066));
#49644=CARTESIAN_POINT('Ctrl Pts',(-21.,-6.79571235355295,4.39092540044367));
#49645=CARTESIAN_POINT('Ctrl Pts',(-21.,-6.88325224876452,4.44037556328962));
#49646=CARTESIAN_POINT('Ctrl Pts',(-21.,-6.9732685530375,4.48581308997575));
#49647=CARTESIAN_POINT('Ctrl Pts',(-21.,-7.06592138953324,4.5267956450212));
#49648=CARTESIAN_POINT('Ctrl Pts',(-21.,-7.16121001331941,4.56309881747208));
#49649=CARTESIAN_POINT('Ctrl Pts',(-21.,-7.25900770064673,4.59469206087561));
#49650=CARTESIAN_POINT('Ctrl Pts',(-21.,-7.35910284385827,4.62170482170181));
#49651=CARTESIAN_POINT('Ctrl Pts',(-21.,-7.46123890856565,4.64440143603747));
#49652=CARTESIAN_POINT('Ctrl Pts',(-21.,-7.56514580946327,4.66314297047291));
#49653=CARTESIAN_POINT('Ctrl Pts',(-21.,-7.67055506601851,4.67833376211481));
#49654=CARTESIAN_POINT('Ctrl Pts',(-21.,-7.77721964274024,4.69037000103626));
#49655=CARTESIAN_POINT('Ctrl Pts',(-21.,-7.8849298684541,4.69959254734285));
#49656=CARTESIAN_POINT('Ctrl Pts',(-21.,-7.99353571494822,4.70622700687469));
#49657=CARTESIAN_POINT('Ctrl Pts',(-21.,-8.08820523826853,4.70981110890122));
#49658=CARTESIAN_POINT('Ctrl Pts',(-21.,-8.16141264001154,4.71119538406403));
#49659=CARTESIAN_POINT('Ctrl Pts',(-21.,-8.2128114080041,4.71148495034738));
#49660=CARTESIAN_POINT('Ctrl Pts',(-21.,-8.24217907974318,4.71142767604211));
#49661=CARTESIAN_POINT('Ctrl Pts',(-21.,-8.24940658621529,4.71140010775012));
#49662=CARTESIAN_POINT('',(-21.,-8.83189477299562,3.49966208636385));
#49663=CARTESIAN_POINT('Origin',(-21.,0.,0.));
#49664=CARTESIAN_POINT('',(-21.,-6.8122671513043,2.29198004120026));
#49665=CARTESIAN_POINT('Ctrl Pts',(-21.,-8.83189477299562,3.49966208636385));
#49666=CARTESIAN_POINT('Ctrl Pts',(-21.,-8.82094392654054,3.48448547507508));
#49667=CARTESIAN_POINT('Ctrl Pts',(-21.,-8.7936907445869,3.44793862615663));
#49668=CARTESIAN_POINT('Ctrl Pts',(-21.,-8.74934377286773,3.39315507789778));
#49669=CARTESIAN_POINT('Ctrl Pts',(-21.,-8.68667704834296,3.32467389681987));
#49670=CARTESIAN_POINT('Ctrl Pts',(-21.,-8.60460841273967,3.24456764186082));
#49671=CARTESIAN_POINT('Ctrl Pts',(-21.,-8.51516539363766,3.16038325236223));
#49672=CARTESIAN_POINT('Ctrl Pts',(-21.,-8.4243384303954,3.07426635319921));
#49673=CARTESIAN_POINT('Ctrl Pts',(-21.,-8.33184183835821,2.98721060740198));
#49674=CARTESIAN_POINT('Ctrl Pts',(-21.,-8.2370828133169,2.90227874531213));
#49675=CARTESIAN_POINT('Ctrl Pts',(-21.,-8.13939365460193,2.82329483425037));
#49676=CARTESIAN_POINT('Ctrl Pts',(-21.,-8.03835937937461,2.75296659957235));
#49677=CARTESIAN_POINT('Ctrl Pts',(-21.,-7.93399262158453,2.69188736687836));
#49678=CARTESIAN_POINT('Ctrl Pts',(-21.,-7.82659266808561,2.63932460382938));
#49679=CARTESIAN_POINT('Ctrl Pts',(-21.,-7.71666617412861,2.59365833862295));
#49680=CARTESIAN_POINT('Ctrl Pts',(-21.,-7.60482241577417,2.55297760756074));
#49681=CARTESIAN_POINT('Ctrl Pts',(-21.,-7.49168859641893,2.51552733857386));
#49682=CARTESIAN_POINT('Ctrl Pts',(-21.,-7.37786505179862,2.47974127678492));
#49683=CARTESIAN_POINT('Ctrl Pts',(-21.,-7.26387759821705,2.44432136933076));
#49684=CARTESIAN_POINT('Ctrl Pts',(-21.,-7.15012820840451,2.4083053284885));
#49685=CARTESIAN_POINT('Ctrl Pts',(-21.,-7.03685278876406,2.37112767623027));
#49686=CARTESIAN_POINT('Ctrl Pts',(-21.,-6.94670492800217,2.34023288057449));
#49687=CARTESIAN_POINT('Ctrl Pts',(-21.,-6.8793763726903,2.31637371632821));
#49688=CARTESIAN_POINT('Ctrl Pts',(-21.,-6.83461600336474,2.30016217089616));
#49689=CARTESIAN_POINT('Ctrl Pts',(-21.,-6.8122671513043,2.29198004120026));
#49690=CARTESIAN_POINT('',(-21.,-7.13209349341826,0.890729280500487));
#49691=CARTESIAN_POINT('Origin',(-21.,0.,0.));
#49692=CARTESIAN_POINT('',(-21.,-9.47665840807863,0.665541446186861));
#49693=CARTESIAN_POINT('Ctrl Pts',(-21.,-7.13209349341826,0.890729280500492));
#49694=CARTESIAN_POINT('Ctrl Pts',(-21.,-7.15211036864424,0.892482057440589));
#49695=CARTESIAN_POINT('Ctrl Pts',(-21.,-7.19212249719958,0.89615029887462));
#49696=CARTESIAN_POINT('Ctrl Pts',(-21.,-7.25207582250743,0.902140734147994));
#49697=CARTESIAN_POINT('Ctrl Pts',(-21.,-7.33188369780814,0.911105335666499));
#49698=CARTESIAN_POINT('Ctrl Pts',(-21.,-7.43143474677318,0.923884053007731));
#49699=CARTESIAN_POINT('Ctrl Pts',(-21.,-7.53080214904746,0.938052795086852));
#49700=CARTESIAN_POINT('Ctrl Pts',(-21.,-7.63003710778607,0.953237934402831));
#49701=CARTESIAN_POINT('Ctrl Pts',(-21.,-7.7292275500742,0.968799418422935));
#49702=CARTESIAN_POINT('Ctrl Pts',(-21.,-7.82850348500033,0.983785216334555));
#49703=CARTESIAN_POINT('Ctrl Pts',(-21.,-7.92800888935854,0.997080466154163));
#49704=CARTESIAN_POINT('Ctrl Pts',(-21.,-8.02787639670185,1.00753800115478));
#49705=CARTESIAN_POINT('Ctrl Pts',(-21.,-8.12820273854249,1.01410892133532));
#49706=CARTESIAN_POINT('Ctrl Pts',(-21.,-8.2290192302709,1.01599010763451));
#49707=CARTESIAN_POINT('Ctrl Pts',(-21.,-8.33027821569813,1.01271355471894));
#49708=CARTESIAN_POINT('Ctrl Pts',(-21.,-8.43188165539955,1.00407739851957));
#49709=CARTESIAN_POINT('Ctrl Pts',(-21.,-8.53370212161309,0.990109101007577));
#49710=CARTESIAN_POINT('Ctrl Pts',(-21.,-8.63560512714608,0.971017102543951));
#49711=CARTESIAN_POINT('Ctrl Pts',(-21.,-8.73747423363077,0.947150867813171));
#49712=CARTESIAN_POINT('Ctrl Pts',(-21.,-8.83922276353739,0.918952892194649));
#49713=CARTESIAN_POINT('Ctrl Pts',(-21.,-8.94078425956014,0.886903960171005));
#49714=CARTESIAN_POINT('Ctrl Pts',(-21.,-9.04210805084257,0.851468211346448));
#49715=CARTESIAN_POINT('Ctrl Pts',(-21.,-9.14315312384119,0.813043722977555));
#49716=CARTESIAN_POINT('Ctrl Pts',(-21.,-9.24388219451328,0.771898853704203));
#49717=CARTESIAN_POINT('Ctrl Pts',(-21.,-9.33073157135269,0.734052451290806));
#49718=CARTESIAN_POINT('Ctrl Pts',(-21.,-9.39728977570677,0.703536138917768));
#49719=CARTESIAN_POINT('Ctrl Pts',(-21.,-9.44372410361835,0.681495939481608));
#49720=CARTESIAN_POINT('Ctrl Pts',(-21.,-9.47015861118831,0.668702181892298));
#49721=CARTESIAN_POINT('Ctrl Pts',(-21.,-9.47665840807863,0.665541446186861));
#49722=CARTESIAN_POINT('',(-21.,-9.47570870673866,-0.6789289396079));
#49723=CARTESIAN_POINT('Origin',(-21.,0.,0.));
#49724=CARTESIAN_POINT('',(-21.,-7.13209349341826,-0.89072928050049));
#49725=CARTESIAN_POINT('Ctrl Pts',(-21.,-9.47570870673866,-0.6789289396079));
#49726=CARTESIAN_POINT('Ctrl Pts',(-21.,-9.45925745015235,-0.687851199692912));
#49727=CARTESIAN_POINT('Ctrl Pts',(-21.,-9.41884609819914,-0.708954060299465));
#49728=CARTESIAN_POINT('Ctrl Pts',(-21.,-9.35512116653373,-0.739070901845867));
#49729=CARTESIAN_POINT('Ctrl Pts',(-21.,-9.26894752777823,-0.77358024127919));
#49730=CARTESIAN_POINT('Ctrl Pts',(-21.,-9.1602494406401,-0.810145236641717));
#49731=CARTESIAN_POINT('Ctrl Pts',(-21.,-9.04313782728701,-0.847184879177381));
#49732=CARTESIAN_POINT('Ctrl Pts',(-21.,-8.92394083882956,-0.885365181899303));
#49733=CARTESIAN_POINT('Ctrl Pts',(-21.,-8.80283221651881,-0.923666931425906));
#49734=CARTESIAN_POINT('Ctrl Pts',(-21.,-8.68060673111004,-0.959073494961789));
#49735=CARTESIAN_POINT('Ctrl Pts',(-21.,-8.55832200571467,-0.98784980243911));
#49736=CARTESIAN_POINT('Ctrl Pts',(-21.,-8.43677899171613,-1.00737622330388));
#49737=CARTESIAN_POINT('Ctrl Pts',(-21.,-8.31624650623966,-1.017123671327));
#49738=CARTESIAN_POINT('Ctrl Pts',(-21.,-8.19667636355292,-1.01788199103989));
#49739=CARTESIAN_POINT('Ctrl Pts',(-21.,-8.0778221648407,-1.01133055607812));
#49740=CARTESIAN_POINT('Ctrl Pts',(-21.,-7.95940371279084,-0.999455440216892));
#49741=CARTESIAN_POINT('Ctrl Pts',(-21.,-7.84122460090589,-0.984110042106142));
#49742=CARTESIAN_POINT('Ctrl Pts',(-21.,-7.72314614047142,-0.966965984543332));
#49743=CARTESIAN_POINT('Ctrl Pts',(-21.,-7.60507887157754,-0.949420915891056));
#49744=CARTESIAN_POINT('Ctrl Pts',(-21.,-7.4869674381447,-0.932516236860826));
#49745=CARTESIAN_POINT('Ctrl Pts',(-21.,-7.36877903277666,-0.916863781503486));
#49746=CARTESIAN_POINT('Ctrl Pts',(-21.,-7.27415386726379,-0.90558533966873));
#49747=CARTESIAN_POINT('Ctrl Pts',(-21.,-7.20314083161155,-0.89786893854071));
#49748=CARTESIAN_POINT('Ctrl Pts',(-21.,-7.15577920638447,-0.893054239868308));
#49749=CARTESIAN_POINT('Ctrl Pts',(-21.,-7.13209349341826,-0.89072928050049));
#49750=CARTESIAN_POINT('',(-21.,-6.8122671513043,-2.29198004120026));
#49751=CARTESIAN_POINT('Origin',(-21.,0.,0.));
#49752=CARTESIAN_POINT('',(-21.,-8.82694180863381,-3.51213586112389));
#49753=CARTESIAN_POINT('Ctrl Pts',(-21.,-6.8122671513043,-2.29198004120026));
#49754=CARTESIAN_POINT('Ctrl Pts',(-21.,-6.8310622341282,-2.29908584041335));
#49755=CARTESIAN_POINT('Ctrl Pts',(-21.,-6.86870350660446,-2.31314148102898));
#49756=CARTESIAN_POINT('Ctrl Pts',(-21.,-6.92531873868941,-2.33375705829959));
#49757=CARTESIAN_POINT('Ctrl Pts',(-21.,-7.00111274457534,-2.36030757076476));
#49758=CARTESIAN_POINT('Ctrl Pts',(-21.,-7.09634961812101,-2.39198792562662));
#49759=CARTESIAN_POINT('Ctrl Pts',(-21.,-7.19202414084635,-2.42233623016115));
#49760=CARTESIAN_POINT('Ctrl Pts',(-21.,-7.28802033430286,-2.45171132733138));
#49761=CARTESIAN_POINT('Ctrl Pts',(-21.,-7.3841397096708,-2.4807280346756));
#49762=CARTESIAN_POINT('Ctrl Pts',(-21.,-7.4800863304027,-2.5103005111467));
#49763=CARTESIAN_POINT('Ctrl Pts',(-21.,-7.57550619462173,-2.54149568187359));
#49764=CARTESIAN_POINT('Ctrl Pts',(-21.,-7.67002106404108,-2.5754046559055));
#49765=CARTESIAN_POINT('Ctrl Pts',(-21.,-7.76326299008741,-2.61301442971916));
#49766=CARTESIAN_POINT('Ctrl Pts',(-21.,-7.85491172665132,-2.65506217582471));
#49767=CARTESIAN_POINT('Ctrl Pts',(-21.,-7.94472127708621,-2.70194887521209));
#49768=CARTESIAN_POINT('Ctrl Pts',(-21.,-8.03251572538561,-2.75381386341092));
#49769=CARTESIAN_POINT('Ctrl Pts',(-21.,-8.11819217840571,-2.81057710920625));
#49770=CARTESIAN_POINT('Ctrl Pts',(-21.,-8.201719906256,-2.87199246251599));
#49771=CARTESIAN_POINT('Ctrl Pts',(-21.,-8.28314562863609,-2.93769454582461));
#49772=CARTESIAN_POINT('Ctrl Pts',(-21.,-8.36258324333989,-3.00724707660037));
#49773=CARTESIAN_POINT('Ctrl Pts',(-21.,-8.44018147897284,-3.08018804824792));
#49774=CARTESIAN_POINT('Ctrl Pts',(-21.,-8.51609606529771,-3.15607730017284));
#49775=CARTESIAN_POINT('Ctrl Pts',(-21.,-8.59046276963722,-3.23453838205034));
#49776=CARTESIAN_POINT('Ctrl Pts',(-21.,-8.66336443667969,-3.31531333416059));
#49777=CARTESIAN_POINT('Ctrl Pts',(-21.,-8.72519208281745,-3.38709429686028));
#49778=CARTESIAN_POINT('Ctrl Pts',(-21.,-8.77191842112748,-3.44346706684567));
#49779=CARTESIAN_POINT('Ctrl Pts',(-21.,-8.80419142083552,-3.4834717001977));
#49780=CARTESIAN_POINT('Ctrl Pts',(-21.,-8.82245708581418,-3.50646798047535));
#49781=CARTESIAN_POINT('Ctrl Pts',(-21.,-8.82694180863381,-3.51213586112389));
#49782=CARTESIAN_POINT('',(-21.,-8.24274231917123,-4.72304976257329));
#49783=CARTESIAN_POINT('Origin',(-21.,0.,0.));
#49784=CARTESIAN_POINT('',(-21.,-6.03932124977421,-3.89701874412038));
#49785=CARTESIAN_POINT('Ctrl Pts',(-21.,-8.24274231917123,-4.72304976257329));
#49786=CARTESIAN_POINT('Ctrl Pts',(-21.,-8.22404902558203,-4.72395050842036));
#49787=CARTESIAN_POINT('Ctrl Pts',(-21.,-8.17848346749629,-4.7254297003623));
#49788=CARTESIAN_POINT('Ctrl Pts',(-21.,-8.10800208013598,-4.72491482536916));
#49789=CARTESIAN_POINT('Ctrl Pts',(-21.,-8.0153892731556,-4.71861732525386));
#49790=CARTESIAN_POINT('Ctrl Pts',(-21.,-7.9015907237349,-4.70439891524807));
#49791=CARTESIAN_POINT('Ctrl Pts',(-21.,-7.78000590743498,-4.68695765535521));
#49792=CARTESIAN_POINT('Ctrl Pts',(-21.,-7.65604731918147,-4.66963928443128));
#49793=CARTESIAN_POINT('Ctrl Pts',(-21.,-7.53031371454558,-4.65160090645338));
#49794=CARTESIAN_POINT('Ctrl Pts',(-21.,-7.40483002515176,-4.63046946729401));
#49795=CARTESIAN_POINT('Ctrl Pts',(-21.,-7.28216972266428,-4.60333867057275));
#49796=CARTESIAN_POINT('Ctrl Pts',(-21.,-7.16419105444418,-4.56819583049617));
#49797=CARTESIAN_POINT('Ctrl Pts',(-21.,-7.05136577826386,-4.52468089222283));
#49798=CARTESIAN_POINT('Ctrl Pts',(-21.,-6.94330777957998,-4.47348457408032));
#49799=CARTESIAN_POINT('Ctrl Pts',(-21.,-6.83906640781858,-4.4160130309926));
#49800=CARTESIAN_POINT('Ctrl Pts',(-21.,-6.73752748880879,-4.35393408054299));
#49801=CARTESIAN_POINT('Ctrl Pts',(-21.,-6.63770990687462,-4.2888323596294));
#49802=CARTESIAN_POINT('Ctrl Pts',(-21.,-6.53876341785232,-4.22215377357323));
#49803=CARTESIAN_POINT('Ctrl Pts',(-21.,-6.44000100425059,-4.15511874483724));
#49804=CARTESIAN_POINT('Ctrl Pts',(-21.,-6.34092094513049,-4.08864152493875));
#49805=CARTESIAN_POINT('Ctrl Pts',(-21.,-6.24122821720367,-4.02325912271413));
#49806=CARTESIAN_POINT('Ctrl Pts',(-21.,-6.16086742147115,-3.97204127711522));
#49807=CARTESIAN_POINT('Ctrl Pts',(-21.,-6.10023490810719,-3.93427763849175));
#49808=CARTESIAN_POINT('Ctrl Pts',(-21.,-6.05965257770704,-3.90939030583537));
#49809=CARTESIAN_POINT('Ctrl Pts',(-21.,-6.03932124977421,-3.89701874412038));
#49810=CARTESIAN_POINT('',(-21.,-5.14318775290069,-5.02073460645077));
#49811=CARTESIAN_POINT('Origin',(-21.,0.,0.));
#49812=CARTESIAN_POINT('',(-21.,-6.42894112865204,-6.99419158761942));
#49813=CARTESIAN_POINT('Ctrl Pts',(-21.,-5.14318775290069,-5.02073460645076));
#49814=CARTESIAN_POINT('Ctrl Pts',(-21.,-5.15703844666268,-5.03529159113598));
#49815=CARTESIAN_POINT('Ctrl Pts',(-21.,-5.18485354740602,-5.06428722179623));
#49816=CARTESIAN_POINT('Ctrl Pts',(-21.,-5.22691734521339,-5.10742564369891));
#49817=CARTESIAN_POINT('Ctrl Pts',(-21.,-5.28368554926634,-5.16423261553338));
#49818=CARTESIAN_POINT('Ctrl Pts',(-21.,-5.35574541658332,-5.23409735978387));
#49819=CARTESIAN_POINT('Ctrl Pts',(-21.,-5.42877754716296,-5.30295185702147));
#49820=CARTESIAN_POINT('Ctrl Pts',(-21.,-5.50252175190725,-5.37106909242141));
#49821=CARTESIAN_POINT('Ctrl Pts',(-21.,-5.57653243923659,-5.43891687637388));
#49822=CARTESIAN_POINT('Ctrl Pts',(-21.,-5.65014634083023,-5.50719043557996));
#49823=CARTESIAN_POINT('Ctrl Pts',(-21.,-5.72258159055366,-5.57669744070723));
#49824=CARTESIAN_POINT('Ctrl Pts',(-21.,-5.79302399301176,-5.64825683559838));
#49825=CARTESIAN_POINT('Ctrl Pts',(-21.,-5.86071379627312,-5.72259822644884));
#49826=CARTESIAN_POINT('Ctrl Pts',(-21.,-5.92504262139805,-5.80024683316115));
#49827=CARTESIAN_POINT('Ctrl Pts',(-21.,-5.98561485393513,-5.88145719317904));
#49828=CARTESIAN_POINT('Ctrl Pts',(-21.,-6.04221154361855,-5.96627851638222));
#49829=CARTESIAN_POINT('Ctrl Pts',(-21.,-6.09477471117184,-6.05459405347559));
#49830=CARTESIAN_POINT('Ctrl Pts',(-21.,-6.14338347043832,-6.14616869769857));
#49831=CARTESIAN_POINT('Ctrl Pts',(-21.,-6.18823844577549,-6.2406935262026));
#49832=CARTESIAN_POINT('Ctrl Pts',(-21.,-6.22963155144596,-6.33782488040964));
#49833=CARTESIAN_POINT('Ctrl Pts',(-21.,-6.2678972444421,-6.43721103768399));
#49834=CARTESIAN_POINT('Ctrl Pts',(-21.,-6.30336681095649,-6.53852299564495));
#49835=CARTESIAN_POINT('Ctrl Pts',(-21.,-6.33632590879467,-6.64148049150319));
#49836=CARTESIAN_POINT('Ctrl Pts',(-21.,-6.36696110296949,-6.74588705654512));
#49837=CARTESIAN_POINT('Ctrl Pts',(-21.,-6.3915212948217,-6.8373854795327));
#49838=CARTESIAN_POINT('Ctrl Pts',(-21.,-6.40916104272443,-6.90844938866819));
#49839=CARTESIAN_POINT('Ctrl Pts',(-21.,-6.42088065083439,-6.95849504767608));
#49840=CARTESIAN_POINT('Ctrl Pts',(-21.,-6.42735973425904,-6.9871391553022));
#49841=CARTESIAN_POINT('Ctrl Pts',(-21.,-6.42894112865204,-6.99419158761942));
#49842=CARTESIAN_POINT('',(-21.,-5.37719972469147,-7.83171265565699));
#49843=CARTESIAN_POINT('Origin',(-21.,0.,0.));
#49844=CARTESIAN_POINT('',(-21.,-3.75038736519793,-6.13145585166881));
#49845=CARTESIAN_POINT('Ctrl Pts',(-21.,-5.37719972469147,-7.83171265565699));
#49846=CARTESIAN_POINT('Ctrl Pts',(-21.,-5.35996683015292,-7.82441348350419));
#49847=CARTESIAN_POINT('Ctrl Pts',(-21.,-5.31827188353843,-7.80597603467631));
#49848=CARTESIAN_POINT('Ctrl Pts',(-21.,-5.25499374364742,-7.77493142045055));
#49849=CARTESIAN_POINT('Ctrl Pts',(-21.,-5.17428487068616,-7.72907437791823));
#49850=CARTESIAN_POINT('Ctrl Pts',(-21.,-5.07792505734327,-7.66688869302314));
#49851=CARTESIAN_POINT('Ctrl Pts',(-21.,-4.97594840210465,-7.59842098612654));
#49852=CARTESIAN_POINT('Ctrl Pts',(-21.,-4.87177973271099,-7.52903405731413));
#49853=CARTESIAN_POINT('Ctrl Pts',(-21.,-4.76632422816958,-7.45822827381644));
#49854=CARTESIAN_POINT('Ctrl Pts',(-21.,-4.66243591843162,-7.38474417264741));
#49855=CARTESIAN_POINT('Ctrl Pts',(-21.,-4.56369441608956,-7.30707985875561));
#49856=CARTESIAN_POINT('Ctrl Pts',(-21.,-4.4726472158023,-7.22422822821349));
#49857=CARTESIAN_POINT('Ctrl Pts',(-21.,-4.38987557857684,-7.13606957084443));
#49858=CARTESIAN_POINT('Ctrl Pts',(-21.,-4.31473193577955,-7.04305867353628));
#49859=CARTESIAN_POINT('Ctrl Pts',(-21.,-4.24574967308285,-6.94604996627335));
#49860=CARTESIAN_POINT('Ctrl Pts',(-21.,-4.18120131531612,-6.84606267872027));
#49861=CARTESIAN_POINT('Ctrl Pts',(-21.,-4.11951535961712,-6.74409882925098));
#49862=CARTESIAN_POINT('Ctrl Pts',(-21.,-4.0592984076569,-6.64109222642907));
#49863=CARTESIAN_POINT('Ctrl Pts',(-21.,-3.99940195660266,-6.53784434718121));
#49864=CARTESIAN_POINT('Ctrl Pts',(-21.,-3.93897729264122,-6.43496121510494));
#49865=CARTESIAN_POINT('Ctrl Pts',(-21.,-3.87752560957259,-6.33279865263617));
#49866=CARTESIAN_POINT('Ctrl Pts',(-21.,-3.82734562477572,-6.25178572573963));
#49867=CARTESIAN_POINT('Ctrl Pts',(-21.,-3.78910264658076,-6.19145440139071));
#49868=CARTESIAN_POINT('Ctrl Pts',(-21.,-3.7633374392529,-6.15142367620606));
#49869=CARTESIAN_POINT('Ctrl Pts',(-21.,-3.75038736519793,-6.13145585166881));
#49870=CARTESIAN_POINT('',(-21.,-2.45543694297674,-6.75507110762463));
#49871=CARTESIAN_POINT('Origin',(-21.,0.,0.));
#49872=CARTESIAN_POINT('',(-21.,-2.75760981235205,-9.09096189205629));
#49873=CARTESIAN_POINT('Ctrl Pts',(-21.,-2.45543694297675,-6.75507110762463));
#49874=CARTESIAN_POINT('Ctrl Pts',(-21.,-2.46159994790965,-6.77419608843536));
#49875=CARTESIAN_POINT('Ctrl Pts',(-21.,-2.47407975508802,-6.8123887688799));
#49876=CARTESIAN_POINT('Ctrl Pts',(-21.,-2.49326086758344,-6.8695059418988));
#49877=CARTESIAN_POINT('Ctrl Pts',(-21.,-2.5197596307744,-6.94531805563895));
#49878=CARTESIAN_POINT('Ctrl Pts',(-21.,-2.55437015138428,-7.03952961984441));
#49879=CARTESIAN_POINT('Ctrl Pts',(-21.,-2.59029498067661,-7.13325283216217));
#49880=CARTESIAN_POINT('Ctrl Pts',(-21.,-2.62718125254576,-7.22662075191781));
#49881=CARTESIAN_POINT('Ctrl Pts',(-21.,-2.66442452752942,-7.31986152676826));
#49882=CARTESIAN_POINT('Ctrl Pts',(-21.,-2.70112557395893,-7.41331375298832));
#49883=CARTESIAN_POINT('Ctrl Pts',(-21.,-2.73622951961898,-7.50736587770304));
#49884=CARTESIAN_POINT('Ctrl Pts',(-21.,-2.76864747338962,-7.60240247767684));
#49885=CARTESIAN_POINT('Ctrl Pts',(-21.,-2.79737835816915,-7.69875126136884));
#49886=CARTESIAN_POINT('Ctrl Pts',(-21.,-2.82164615909785,-7.79662146983088));
#49887=CARTESIAN_POINT('Ctrl Pts',(-21.,-2.84098400021346,-7.89607078269802));
#49888=CARTESIAN_POINT('Ctrl Pts',(-21.,-2.85517326277626,-7.9970485375799));
#49889=CARTESIAN_POINT('Ctrl Pts',(-21.,-2.86421236488387,-8.099424390731));
#49890=CARTESIAN_POINT('Ctrl Pts',(-21.,-2.8682745946465,-8.20302084448955));
#49891=CARTESIAN_POINT('Ctrl Pts',(-21.,-2.86767474496505,-8.30764661663281));
#49892=CARTESIAN_POINT('Ctrl Pts',(-21.,-2.86282492937103,-8.41311873833255));
#49893=CARTESIAN_POINT('Ctrl Pts',(-21.,-2.85417908993455,-8.51926543389428));
#49894=CARTESIAN_POINT('Ctrl Pts',(-21.,-2.84217845398458,-8.62593402210748));
#49895=CARTESIAN_POINT('Ctrl Pts',(-21.,-2.82720199177778,-8.73299593720093));
#49896=CARTESIAN_POINT('Ctrl Pts',(-21.,-2.80950303716262,-8.84035511450549));
#49897=CARTESIAN_POINT('Ctrl Pts',(-21.,-2.79193132752197,-8.93344861295375));
#49898=CARTESIAN_POINT('Ctrl Pts',(-21.,-2.77699071660796,-9.0051285824934));
#49899=CARTESIAN_POINT('Ctrl Pts',(-21.,-2.76583572100211,-9.05530311062091));
#49900=CARTESIAN_POINT('Ctrl Pts',(-21.,-2.75924496093975,-9.08392172878324));
#49901=CARTESIAN_POINT('Ctrl Pts',(-21.,-2.75760981235205,-9.09096189205629));
#49902=CARTESIAN_POINT('',(-21.,-1.44663677770972,-9.38920880763537));
#49903=CARTESIAN_POINT('Origin',(-21.,0.,0.));
#49904=CARTESIAN_POINT('',(-21.,-0.718643267461624,-7.15148293042304));
#49905=CARTESIAN_POINT('Ctrl Pts',(-21.,-1.44663677770972,-9.38920880763537));
#49906=CARTESIAN_POINT('Ctrl Pts',(-21.,-1.43427746833275,-9.37515540804603));
#49907=CARTESIAN_POINT('Ctrl Pts',(-21.,-1.40471132872148,-9.34045308130916));
#49908=CARTESIAN_POINT('Ctrl Pts',(-21.,-1.36116944796064,-9.28502749443539));
#49909=CARTESIAN_POINT('Ctrl Pts',(-21.,-1.30834989113785,-9.2086934591593));
#49910=CARTESIAN_POINT('Ctrl Pts',(-21.,-1.24851405668088,-9.11085713692575));
#49911=CARTESIAN_POINT('Ctrl Pts',(-21.,-1.18634328973517,-9.00492385207762));
#49912=CARTESIAN_POINT('Ctrl Pts',(-21.,-1.12259642171968,-8.89721129760285));
#49913=CARTESIAN_POINT('Ctrl Pts',(-21.,-1.05830577327405,-8.78766206238304));
#49914=CARTESIAN_POINT('Ctrl Pts',(-21.,-0.996589197042053,-8.67637972666424));
#49915=CARTESIAN_POINT('Ctrl Pts',(-21.,-0.941323460369318,-8.56356426545847));
#49916=CARTESIAN_POINT('Ctrl Pts',(-21.,-0.895240742652424,-8.44941362598824));
#49917=CARTESIAN_POINT('Ctrl Pts',(-21.,-0.858916682261846,-8.33407215281038));
#49918=CARTESIAN_POINT('Ctrl Pts',(-21.,-0.831570515383447,-8.21766862525226));
#49919=CARTESIAN_POINT('Ctrl Pts',(-21.,-0.811510144890449,-8.10033651802127));
#49920=CARTESIAN_POINT('Ctrl Pts',(-21.,-0.796736942256156,-7.98224460192821));
#49921=CARTESIAN_POINT('Ctrl Pts',(-21.,-0.785400272847099,-7.86361381479518));
#49922=CARTESIAN_POINT('Ctrl Pts',(-21.,-0.775839563797133,-7.74468091618948));
#49923=CARTESIAN_POINT('Ctrl Pts',(-21.,-0.766672302003446,-7.62566969516693));
#49924=CARTESIAN_POINT('Ctrl Pts',(-21.,-0.756870878958097,-7.5067579169994));
#49925=CARTESIAN_POINT('Ctrl Pts',(-21.,-0.745831500234844,-7.38804974272502));
#49926=CARTESIAN_POINT('Ctrl Pts',(-21.,-0.735771087779772,-7.29328733826105));
#49927=CARTESIAN_POINT('Ctrl Pts',(-21.,-0.72749213560466,-7.22233768688913));
#49928=CARTESIAN_POINT('Ctrl Pts',(-21.,-0.721647166649912,-7.17509214524366));
#49929=CARTESIAN_POINT('Ctrl Pts',(-21.,-0.718643267461624,-7.15148293042304));
#49930=CARTESIAN_POINT('',(-21.,0.718643267461627,-7.15148293042304));
#49931=CARTESIAN_POINT('Origin',(-21.,0.,0.));
#49932=CARTESIAN_POINT('',(-21.,1.45989994714919,-9.38715570044056));
#49933=CARTESIAN_POINT('Ctrl Pts',(-21.,0.718643267461621,-7.15148293042304));
#49934=CARTESIAN_POINT('Ctrl Pts',(-21.,0.721388610069064,-7.17138797035723));
#49935=CARTESIAN_POINT('Ctrl Pts',(-21.,0.72671587532212,-7.21121317182152));
#49936=CARTESIAN_POINT('Ctrl Pts',(-21.,0.734216502709278,-7.2709963393441));
#49937=CARTESIAN_POINT('Ctrl Pts',(-21.,0.743235585416283,-7.35079807608913));
#49938=CARTESIAN_POINT('Ctrl Pts',(-21.,0.752929449590465,-7.45069670452966));
#49939=CARTESIAN_POINT('Ctrl Pts',(-21.,0.761227274615911,-7.55072560028829));
#49940=CARTESIAN_POINT('Ctrl Pts',(-21.,0.768504714146026,-7.65085154280962));
#49941=CARTESIAN_POINT('Ctrl Pts',(-21.,0.775405338877349,-7.75101782957587));
#49942=CARTESIAN_POINT('Ctrl Pts',(-21.,0.782886239966143,-7.85113936329068));
#49943=CARTESIAN_POINT('Ctrl Pts',(-21.,0.792066365329068,-7.95110843081948));
#49944=CARTESIAN_POINT('Ctrl Pts',(-21.,0.804093633570272,-8.05079907170372));
#49945=CARTESIAN_POINT('Ctrl Pts',(-21.,0.820012171364339,-8.15007218998677));
#49946=CARTESIAN_POINT('Ctrl Pts',(-21.,0.840611930230857,-8.24877960511329));
#49947=CARTESIAN_POINT('Ctrl Pts',(-21.,0.866338577132719,-8.34677071475058));
#49948=CARTESIAN_POINT('Ctrl Pts',(-21.,0.897367099160984,-8.4439050185459));
#49949=CARTESIAN_POINT('Ctrl Pts',(-21.,0.933642367528787,-8.5400643944807));
#49950=CARTESIAN_POINT('Ctrl Pts',(-21.,0.974931241694465,-8.63516410958082));
#49951=CARTESIAN_POINT('Ctrl Pts',(-21.,1.02086710880845,-8.72916840803945));
#49952=CARTESIAN_POINT('Ctrl Pts',(-21.,1.07099928020948,-8.82209124999857));
#49953=CARTESIAN_POINT('Ctrl Pts',(-21.,1.12484423754393,-8.91397482898789));
#49954=CARTESIAN_POINT('Ctrl Pts',(-21.,1.18193820283021,-9.00487302535333));
#49955=CARTESIAN_POINT('Ctrl Pts',(-21.,1.24188395306769,-9.09483443436949));
#49956=CARTESIAN_POINT('Ctrl Pts',(-21.,1.30441156144786,-9.18388242219763));
#49957=CARTESIAN_POINT('Ctrl Pts',(-21.,1.36063487998417,-9.26013268702205));
#49958=CARTESIAN_POINT('Ctrl Pts',(-21.,1.40519667848883,-9.3182316199014));
#49959=CARTESIAN_POINT('Ctrl Pts',(-21.,1.43701689412372,-9.35859733650268));
#49960=CARTESIAN_POINT('Ctrl Pts',(-21.,1.45537211681237,-9.38152219688984));
#49961=CARTESIAN_POINT('Ctrl Pts',(-21.,1.45989994714919,-9.38715570044056));
#49962=CARTESIAN_POINT('',(-21.,2.77045032493322,-9.08705700417233));
#49963=CARTESIAN_POINT('Origin',(-21.,0.,0.));
#49964=CARTESIAN_POINT('',(-21.,2.45543694297674,-6.75507110762463));
#49965=CARTESIAN_POINT('Ctrl Pts',(-21.,2.77045032493322,-9.08705700417233));
#49966=CARTESIAN_POINT('Ctrl Pts',(-21.,2.7754881363495,-9.06903282528875));
#49967=CARTESIAN_POINT('Ctrl Pts',(-21.,2.78706953240264,-9.02493884204925));
#49968=CARTESIAN_POINT('Ctrl Pts',(-21.,2.8022511505425,-8.95610999975804));
#49969=CARTESIAN_POINT('Ctrl Pts',(-21.,2.81671983020871,-8.86441786360011));
#49970=CARTESIAN_POINT('Ctrl Pts',(-21.,2.8281804649272,-8.7503085875302));
#49971=CARTESIAN_POINT('Ctrl Pts',(-21.,2.838231660712,-8.62789111098118));
#49972=CARTESIAN_POINT('Ctrl Pts',(-21.,2.84893087833482,-8.50318672326558));
#49973=CARTESIAN_POINT('Ctrl Pts',(-21.,2.85932311928695,-8.37659160589212));
#49974=CARTESIAN_POINT('Ctrl Pts',(-21.,2.8666442371861,-8.24955186700095));
#49975=CARTESIAN_POINT('Ctrl Pts',(-21.,2.86748815125169,-8.12392974416385));
#49976=CARTESIAN_POINT('Ctrl Pts',(-21.,2.85947913898695,-8.00108902987832));
#49977=CARTESIAN_POINT('Ctrl Pts',(-21.,2.84216119689693,-7.88140953422486));
#49978=CARTESIAN_POINT('Ctrl Pts',(-21.,2.81629364412744,-7.76466852264525));
#49979=CARTESIAN_POINT('Ctrl Pts',(-21.,2.78345892001629,-7.65025207826714));
#49980=CARTESIAN_POINT('Ctrl Pts',(-21.,2.74553095355499,-7.53744508591865));
#49981=CARTESIAN_POINT('Ctrl Pts',(-21.,2.70427297026251,-7.42564364342468));
#49982=CARTESIAN_POINT('Ctrl Pts',(-21.,2.66128382072048,-7.31434056822034));
#49983=CARTESIAN_POINT('Ctrl Pts',(-21.,2.61790620462629,-7.20313763732345));
#49984=CARTESIAN_POINT('Ctrl Pts',(-21.,2.57514309471485,-7.09174914908801));
#49985=CARTESIAN_POINT('Ctrl Pts',(-21.,2.53358368474749,-6.98000697278327));
#49986=CARTESIAN_POINT('Ctrl Pts',(-21.,2.50153193679118,-6.89026394714059));
#49987=CARTESIAN_POINT('Ctrl Pts',(-21.,2.47820711493347,-6.82274841734025));
#49988=CARTESIAN_POINT('Ctrl Pts',(-21.,2.46297417772978,-6.77764561818537));
#49989=CARTESIAN_POINT('Ctrl Pts',(-21.,2.45543694297674,-6.75507110762463));
#49990=CARTESIAN_POINT('',(-21.,3.75038736519794,-6.13145585166881));
#49991=CARTESIAN_POINT('Origin',(-21.,0.,0.));
#49992=CARTESIAN_POINT('',(-21.,5.38825861761966,-7.82410819644306));
#49993=CARTESIAN_POINT('Ctrl Pts',(-21.,3.75038736519793,-6.13145585166881));
#49994=CARTESIAN_POINT('Ctrl Pts',(-21.,3.7614973065729,-6.1481985134482));
#49995=CARTESIAN_POINT('Ctrl Pts',(-21.,3.78357651403939,-6.1817683663582));
#49996=CARTESIAN_POINT('Ctrl Pts',(-21.,3.81627329006595,-6.23237673886416));
#49997=CARTESIAN_POINT('Ctrl Pts',(-21.,3.859023878729,-6.30036238594766));
#49998=CARTESIAN_POINT('Ctrl Pts',(-21.,3.91110213900011,-6.38616193008433));
#49999=CARTESIAN_POINT('Ctrl Pts',(-21.,3.96197913233089,-6.47268455970493));
#50000=CARTESIAN_POINT('Ctrl Pts',(-21.,4.01197889710939,-6.55973735411151));
#50001=CARTESIAN_POINT('Ctrl Pts',(-21.,4.06165666819706,-6.64698999124062));
#50002=CARTESIAN_POINT('Ctrl Pts',(-21.,4.11183783259628,-6.73395053478792));
#50003=CARTESIAN_POINT('Ctrl Pts',(-21.,4.16348379256721,-6.82003644526658));
#50004=CARTESIAN_POINT('Ctrl Pts',(-21.,4.21757413484032,-6.90463617300865));
#50005=CARTESIAN_POINT('Ctrl Pts',(-21.,4.27498923356982,-6.98717136730191));
#50006=CARTESIAN_POINT('Ctrl Pts',(-21.,4.33637651734857,-7.06716577496009));
#50007=CARTESIAN_POINT('Ctrl Pts',(-21.,4.40207217433237,-7.14429034032177));
#50008=CARTESIAN_POINT('Ctrl Pts',(-21.,4.47217290162416,-7.21834255288981));
#50009=CARTESIAN_POINT('Ctrl Pts',(-21.,4.54657777868016,-7.28923990788708));
#50010=CARTESIAN_POINT('Ctrl Pts',(-21.,4.62503998887083,-7.35700721943171));
#50011=CARTESIAN_POINT('Ctrl Pts',(-21.,4.70721371156899,-7.42177134000892));
#50012=CARTESIAN_POINT('Ctrl Pts',(-21.,4.79269894740031,-7.48374039375355));
#50013=CARTESIAN_POINT('Ctrl Pts',(-21.,4.88107836846757,-7.54316218647348));
#50014=CARTESIAN_POINT('Ctrl Pts',(-21.,4.9719575030537,-7.60028648840776));
#50015=CARTESIAN_POINT('Ctrl Pts',(-21.,5.06499955030093,-7.65532943098672));
#50016=CARTESIAN_POINT('Ctrl Pts',(-21.,5.15997145275563,-7.70842918324715));
#50017=CARTESIAN_POINT('Ctrl Pts',(-21.,5.24371066241773,-7.75273391435114));
#50018=CARTESIAN_POINT('Ctrl Pts',(-21.,5.3090676378046,-7.78574460437678));
#50019=CARTESIAN_POINT('Ctrl Pts',(-21.,5.3552506895127,-7.80830658422591));
#50020=CARTESIAN_POINT('Ctrl Pts',(-21.,5.38173489786212,-7.82099713708327));
#50021=CARTESIAN_POINT('Ctrl Pts',(-21.,5.38825861761966,-7.82410819644306));
#50022=CARTESIAN_POINT('',(-21.,6.43881576337966,-6.98510211559242));
#50023=CARTESIAN_POINT('Origin',(-21.,0.,0.));
#50024=CARTESIAN_POINT('',(-21.,5.14318775290069,-5.02073460645076));
#50025=CARTESIAN_POINT('Ctrl Pts',(-21.,6.43881576337966,-6.98510211559242));
#50026=CARTESIAN_POINT('Ctrl Pts',(-21.,6.43553427649956,-6.96667706709454));
#50027=CARTESIAN_POINT('Ctrl Pts',(-21.,6.42683709146975,-6.9219247815102));
#50028=CARTESIAN_POINT('Ctrl Pts',(-21.,6.4106515413257,-6.85332508014768));
#50029=CARTESIAN_POINT('Ctrl Pts',(-21.,6.38390364438073,-6.76443559520424));
#50030=CARTESIAN_POINT('Ctrl Pts',(-21.,6.34471916009928,-6.65665410688205));
#50031=CARTESIAN_POINT('Ctrl Pts',(-21.,6.30066002212815,-6.5419987212145));
#50032=CARTESIAN_POINT('Ctrl Pts',(-21.,6.25619247809081,-6.42500173364409));
#50033=CARTESIAN_POINT('Ctrl Pts',(-21.,6.2106280007764,-6.30643444970003));
#50034=CARTESIAN_POINT('Ctrl Pts',(-21.,6.16210362315516,-6.18879908596403));
#50035=CARTESIAN_POINT('Ctrl Pts',(-21.,6.108358567083,-6.07525130357771));
#50036=CARTESIAN_POINT('Ctrl Pts',(-21.,6.04784410793973,-5.96805062448362));
#50037=CARTESIAN_POINT('Ctrl Pts',(-21.,5.98031419419066,-5.86773709824143));
#50038=CARTESIAN_POINT('Ctrl Pts',(-21.,5.906356307844,-5.77378059171821));
#50039=CARTESIAN_POINT('Ctrl Pts',(-21.,5.82712980893039,-5.68494139022769));
#50040=CARTESIAN_POINT('Ctrl Pts',(-21.,5.74401277228714,-5.59976212994534));
#50041=CARTESIAN_POINT('Ctrl Pts',(-21.,5.65833178588016,-5.51693367893109));
#50042=CARTESIAN_POINT('Ctrl Pts',(-21.,5.57130730604024,-5.43530536621495));
#50043=CARTESIAN_POINT('Ctrl Pts',(-21.,5.48397628091718,-5.35393582972231));
#50044=CARTESIAN_POINT('Ctrl Pts',(-21.,5.39711839642203,-5.27213248760413));
#50045=CARTESIAN_POINT('Ctrl Pts',(-21.,5.31119154860082,-5.18948821771405));
#50046=CARTESIAN_POINT('Ctrl Pts',(-21.,5.24337588200475,-5.12253927774717));
#50047=CARTESIAN_POINT('Ctrl Pts',(-21.,5.19306705314332,-5.071830148219));
#50048=CARTESIAN_POINT('Ctrl Pts',(-21.,5.1597732798141,-5.03780325407688));
#50049=CARTESIAN_POINT('Ctrl Pts',(-21.,5.14318775290069,-5.02073460645076));
#50050=CARTESIAN_POINT('',(-21.,6.03932124977422,-3.89701874412038));
#50051=CARTESIAN_POINT('Origin',(-21.,0.,0.));
#50052=CARTESIAN_POINT('',(-21.,8.24940658621529,-4.71140010775012));
#50053=CARTESIAN_POINT('Ctrl Pts',(-21.,6.03932124977421,-3.89701874412039));
#50054=CARTESIAN_POINT('Ctrl Pts',(-21.,6.0565953297729,-3.90728293824429));
#50055=CARTESIAN_POINT('Ctrl Pts',(-21.,6.09105342163039,-3.92794852152395));
#50056=CARTESIAN_POINT('Ctrl Pts',(-21.,6.14247034880463,-3.95935849016754));
#50057=CARTESIAN_POINT('Ctrl Pts',(-21.,6.21048516503746,-4.00206265639536));
#50058=CARTESIAN_POINT('Ctrl Pts',(-21.,6.29463308326085,-4.05676946424956));
#50059=CARTESIAN_POINT('Ctrl Pts',(-21.,6.37801243240243,-4.11264895980536));
#50060=CARTESIAN_POINT('Ctrl Pts',(-21.,6.46083145580807,-4.1693867325325));
#50061=CARTESIAN_POINT('Ctrl Pts',(-21.,6.54344708143028,-4.22644426515767));
#50062=CARTESIAN_POINT('Ctrl Pts',(-21.,6.62638951409907,-4.28302021638686));
#50063=CARTESIAN_POINT('Ctrl Pts',(-21.,6.71027219290963,-4.33817259947066));
#50064=CARTESIAN_POINT('Ctrl Pts',(-21.,6.79571235355295,-4.39092540044368));
#50065=CARTESIAN_POINT('Ctrl Pts',(-21.,6.88325224876452,-4.44037556328962));
#50066=CARTESIAN_POINT('Ctrl Pts',(-21.,6.9732685530375,-4.48581308997575));
#50067=CARTESIAN_POINT('Ctrl Pts',(-21.,7.06592138953324,-4.5267956450212));
#50068=CARTESIAN_POINT('Ctrl Pts',(-21.,7.16121001331941,-4.56309881747208));
#50069=CARTESIAN_POINT('Ctrl Pts',(-21.,7.25900770064673,-4.59469206087561));
#50070=CARTESIAN_POINT('Ctrl Pts',(-21.,7.35910284385827,-4.62170482170181));
#50071=CARTESIAN_POINT('Ctrl Pts',(-21.,7.46123890856565,-4.64440143603747));
#50072=CARTESIAN_POINT('Ctrl Pts',(-21.,7.56514580946327,-4.66314297047291));
#50073=CARTESIAN_POINT('Ctrl Pts',(-21.,7.6705550660185,-4.67833376211481));
#50074=CARTESIAN_POINT('Ctrl Pts',(-21.,7.77721964274024,-4.69037000103626));
#50075=CARTESIAN_POINT('Ctrl Pts',(-21.,7.8849298684541,-4.69959254734285));
#50076=CARTESIAN_POINT('Ctrl Pts',(-21.,7.99353571494822,-4.70622700687469));
#50077=CARTESIAN_POINT('Ctrl Pts',(-21.,8.08820523826852,-4.70981110890123));
#50078=CARTESIAN_POINT('Ctrl Pts',(-21.,8.16141264001154,-4.71119538406403));
#50079=CARTESIAN_POINT('Ctrl Pts',(-21.,8.2128114080041,-4.71148495034738));
#50080=CARTESIAN_POINT('Ctrl Pts',(-21.,8.24217907974318,-4.71142767604211));
#50081=CARTESIAN_POINT('Ctrl Pts',(-21.,8.24940658621529,-4.71140010775012));
#50082=CARTESIAN_POINT('Origin',(-21.,0.,0.));
#50083=CARTESIAN_POINT('Origin',(-65.85,0.,0.));
#50084=CARTESIAN_POINT('',(-66.,3.33,-4.07807384116069E-16));
#50085=CARTESIAN_POINT('Origin',(-66.,0.,0.));
#50086=CARTESIAN_POINT('',(-65.85,3.18,-3.89437682128858E-16));
#50087=CARTESIAN_POINT('Origin',(-66.,16.375,0.));
#50088=CARTESIAN_POINT('',(-66.,16.3612159786808,-0.671741541784789));
#50089=CARTESIAN_POINT('',(-66.,14.0217614511585,-1.06963173887292));
#50090=CARTESIAN_POINT('Ctrl Pts',(-66.,16.3612159786808,-0.671741541784789));
#50091=CARTESIAN_POINT('Ctrl Pts',(-66.,16.3519363129391,-0.675875939350101));
#50092=CARTESIAN_POINT('Ctrl Pts',(-66.,16.322986318803,-0.688711885022031));
#50093=CARTESIAN_POINT('Ctrl Pts',(-66.,16.2743241898497,-0.709958710092983));
#50094=CARTESIAN_POINT('Ctrl Pts',(-66.,16.2058743852262,-0.739044856835963));
#50095=CARTESIAN_POINT('Ctrl Pts',(-66.,16.1175336986507,-0.775065535573949));
#50096=CARTESIAN_POINT('Ctrl Pts',(-66.,16.018547775909,-0.813401076758624));
#50097=CARTESIAN_POINT('Ctrl Pts',(-66.,15.9193580975472,-0.849783012021725));
#50098=CARTESIAN_POINT('Ctrl Pts',(-66.,15.8199726227578,-0.884304144422378));
#50099=CARTESIAN_POINT('Ctrl Pts',(-66.,15.7203984586304,-0.917113393337539));
#50100=CARTESIAN_POINT('Ctrl Pts',(-66.,15.6206443917204,-0.948332278883351));
#50101=CARTESIAN_POINT('Ctrl Pts',(-66.,15.5207233107191,-0.977976807855906));
#50102=CARTESIAN_POINT('Ctrl Pts',(-66.,15.42065441025,-1.00588830882699));
#50103=CARTESIAN_POINT('Ctrl Pts',(-66.,15.3204663197849,-1.03163045186508));
#50104=CARTESIAN_POINT('Ctrl Pts',(-66.,15.2201951366894,-1.05457808085916));
#50105=CARTESIAN_POINT('Ctrl Pts',(-66.,15.1198807137451,-1.07407094658941));
#50106=CARTESIAN_POINT('Ctrl Pts',(-66.,15.0195634762927,-1.08955145679141));
#50107=CARTESIAN_POINT('Ctrl Pts',(-66.,14.9192812134642,-1.100697501046));
#50108=CARTESIAN_POINT('Ctrl Pts',(-66.,14.8190654065121,-1.10759084369408));
#50109=CARTESIAN_POINT('Ctrl Pts',(-66.,14.7189411465911,-1.11063958426619));
#50110=CARTESIAN_POINT('Ctrl Pts',(-66.,14.6189280002071,-1.11043751754959));
#50111=CARTESIAN_POINT('Ctrl Pts',(-66.,14.5190405063557,-1.10764458318629));
#50112=CARTESIAN_POINT('Ctrl Pts',(-66.,14.4192887981899,-1.10286394535002));
#50113=CARTESIAN_POINT('Ctrl Pts',(-66.,14.3196790995356,-1.09650878711472));
#50114=CARTESIAN_POINT('Ctrl Pts',(-66.,14.2202146396052,-1.08882773106131));
#50115=CARTESIAN_POINT('Ctrl Pts',(-66.,14.1407601934611,-1.08172501415579));
#50116=CARTESIAN_POINT('Ctrl Pts',(-66.,14.0812352370361,-1.07587965991017));
#50117=CARTESIAN_POINT('Ctrl Pts',(-66.,14.0415811730659,-1.0717527195609));
#50118=CARTESIAN_POINT('Ctrl Pts',(-66.,14.0217614511585,-1.06963173887291));
#50119=CARTESIAN_POINT('',(-66.,13.847248627403,-2.45104298226008));
#50120=CARTESIAN_POINT('Origin',(-66.,0.,0.));
#50121=CARTESIAN_POINT('',(-66.,16.017075735697,-3.40498309495744));
#50122=CARTESIAN_POINT('Ctrl Pts',(-66.,13.847248627403,-2.45104298226008));
#50123=CARTESIAN_POINT('Ctrl Pts',(-66.,13.8704109184829,-2.45416751351779));
#50124=CARTESIAN_POINT('Ctrl Pts',(-66.,13.9167144589915,-2.46064068498796));
#50125=CARTESIAN_POINT('Ctrl Pts',(-66.,13.9861066530346,-2.47102275853729));
#50126=CARTESIAN_POINT('Ctrl Pts',(-66.,14.0785031060049,-2.48621203480011));
#50127=CARTESIAN_POINT('Ctrl Pts',(-66.,14.1937640331043,-2.50749463728168));
#50128=CARTESIAN_POINT('Ctrl Pts',(-66.,14.3087190397278,-2.53121250086624));
#50129=CARTESIAN_POINT('Ctrl Pts',(-66.,14.423228955274,-2.55762788131115));
#50130=CARTESIAN_POINT('Ctrl Pts',(-66.,14.537056384215,-2.58717382256056));
#50131=CARTESIAN_POINT('Ctrl Pts',(-66.,14.6499173448672,-2.62041096375855));
#50132=CARTESIAN_POINT('Ctrl Pts',(-66.,14.7615516365331,-2.65797355871958));
#50133=CARTESIAN_POINT('Ctrl Pts',(-66.,14.8717795409674,-2.70050907188802));
#50134=CARTESIAN_POINT('Ctrl Pts',(-66.,14.9805825983482,-2.74864579544975));
#50135=CARTESIAN_POINT('Ctrl Pts',(-66.,15.0880810351184,-2.80279667637514));
#50136=CARTESIAN_POINT('Ctrl Pts',(-66.,15.1944599098748,-2.86283428974206));
#50137=CARTESIAN_POINT('Ctrl Pts',(-66.,15.299916309402,-2.9278833773088));
#50138=CARTESIAN_POINT('Ctrl Pts',(-66.,15.4045879562307,-2.99587287520288));
#50139=CARTESIAN_POINT('Ctrl Pts',(-66.,15.5085273245779,-3.06389197726713));
#50140=CARTESIAN_POINT('Ctrl Pts',(-66.,15.6117260024113,-3.1296030647124));
#50141=CARTESIAN_POINT('Ctrl Pts',(-66.,15.7141266693079,-3.19226978910788));
#50142=CARTESIAN_POINT('Ctrl Pts',(-66.,15.8156387361042,-3.25420659877988));
#50143=CARTESIAN_POINT('Ctrl Pts',(-66.,15.8964112622344,-3.30811417274226));
#50144=CARTESIAN_POINT('Ctrl Pts',(-66.,15.9565872333324,-3.35376990021665));
#50145=CARTESIAN_POINT('Ctrl Pts',(-66.,15.9965977364772,-3.38711758925191));
#50146=CARTESIAN_POINT('Ctrl Pts',(-66.,16.0167227315819,-3.40467488782123));
#50147=CARTESIAN_POINT('Ctrl Pts',(-66.,16.017075735697,-3.40498309495744));
#50148=CARTESIAN_POINT('',(-66.,15.6801429643085,-4.71950650162129));
#50149=CARTESIAN_POINT('Origin',(-66.,0.,0.));
#50150=CARTESIAN_POINT('',(-66.,13.3152354345065,-4.52309756402218));
#50151=CARTESIAN_POINT('Ctrl Pts',(-66.,15.6801429643085,-4.71950650162129));
#50152=CARTESIAN_POINT('Ctrl Pts',(-66.,15.6701266534662,-4.72120325045824));
#50153=CARTESIAN_POINT('Ctrl Pts',(-66.,15.6388940067504,-4.72643636051809));
#50154=CARTESIAN_POINT('Ctrl Pts',(-66.,15.586476817532,-4.73491389815065));
#50155=CARTESIAN_POINT('Ctrl Pts',(-66.,15.5129440588396,-4.74606347591976));
#50156=CARTESIAN_POINT('Ctrl Pts',(-66.,15.418420778849,-4.75898306342126));
#50157=CARTESIAN_POINT('Ctrl Pts',(-66.,15.3130110194811,-4.77149742512795));
#50158=CARTESIAN_POINT('Ctrl Pts',(-66.,15.2078897478867,-4.78206888507335));
#50159=CARTESIAN_POINT('Ctrl Pts',(-66.,15.1030415940234,-4.79078931010852));
#50160=CARTESIAN_POINT('Ctrl Pts',(-66.,14.9984364069554,-4.79780470849564));
#50161=CARTESIAN_POINT('Ctrl Pts',(-66.,14.8940524763685,-4.80323496770043));
#50162=CARTESIAN_POINT('Ctrl Pts',(-66.,14.7898983053036,-4.80709879692323));
#50163=CARTESIAN_POINT('Ctrl Pts',(-66.,14.6860319453295,-4.80924728319928));
#50164=CARTESIAN_POINT('Ctrl Pts',(-66.,14.5825896373118,-4.80926492456431));
#50165=CARTESIAN_POINT('Ctrl Pts',(-66.,14.4797618145538,-4.80655518238588));
#50166=CARTESIAN_POINT('Ctrl Pts',(-66.,14.3777512750926,-4.80048846137132));
#50167=CARTESIAN_POINT('Ctrl Pts',(-66.,14.27673584179,-4.79053474041595));
#50168=CARTESIAN_POINT('Ctrl Pts',(-66.,14.1768322221664,-4.77639142656668));
#50169=CARTESIAN_POINT('Ctrl Pts',(-66.,14.0780505744683,-4.75814554445644));
#50170=CARTESIAN_POINT('Ctrl Pts',(-66.,13.9803137113395,-4.73619861233502));
#50171=CARTESIAN_POINT('Ctrl Pts',(-66.,13.8834929138094,-4.71113063582666));
#50172=CARTESIAN_POINT('Ctrl Pts',(-66.,13.7874381437893,-4.68358443705714));
#50173=CARTESIAN_POINT('Ctrl Pts',(-66.,13.6920092152502,-4.65414675070122));
#50174=CARTESIAN_POINT('Ctrl Pts',(-66.,13.5971094020329,-4.62321932672933));
#50175=CARTESIAN_POINT('Ctrl Pts',(-66.,13.5026800019769,-4.59104377985933));
#50176=CARTESIAN_POINT('Ctrl Pts',(-66.,13.4274881372306,-4.56440469062003));
#50177=CARTESIAN_POINT('Ctrl Pts',(-66.,13.3712869472582,-4.54393972423008));
#50178=CARTESIAN_POINT('Ctrl Pts',(-66.,13.3339050169562,-4.53008087460641));
#50179=CARTESIAN_POINT('Ctrl Pts',(-66.,13.3152354345065,-4.52309756402217));
#50180=CARTESIAN_POINT('',(-66.,12.8026622457696,-5.81770965851216));
#50181=CARTESIAN_POINT('Origin',(-66.,0.,0.));
#50182=CARTESIAN_POINT('',(-66.,14.6670849864349,-7.28129404712486));
#50183=CARTESIAN_POINT('Ctrl Pts',(-66.,12.8026622457696,-5.81770965851216));
#50184=CARTESIAN_POINT('Ctrl Pts',(-66.,12.8243198115569,-5.82649625442995));
#50185=CARTESIAN_POINT('Ctrl Pts',(-66.,12.8675588289116,-5.84428128157946));
#50186=CARTESIAN_POINT('Ctrl Pts',(-66.,12.932189022876,-5.87159432010365));
#50187=CARTESIAN_POINT('Ctrl Pts',(-66.,13.0179052519711,-5.90928446078516));
#50188=CARTESIAN_POINT('Ctrl Pts',(-66.,13.124252277086,-5.95856265812867));
#50189=CARTESIAN_POINT('Ctrl Pts',(-66.,13.2296973679703,-6.01012352904084));
#50190=CARTESIAN_POINT('Ctrl Pts',(-66.,13.3340405059683,-6.06418647971103));
#50191=CARTESIAN_POINT('Ctrl Pts',(-66.,13.4369440601197,-6.12111191134452));
#50192=CARTESIAN_POINT('Ctrl Pts',(-66.,13.537993545262,-6.18137222620287));
#50193=CARTESIAN_POINT('Ctrl Pts',(-66.,13.6367792028716,-6.24551704256852));
#50194=CARTESIAN_POINT('Ctrl Pts',(-66.,13.7329659430228,-6.31412878948963));
#50195=CARTESIAN_POINT('Ctrl Pts',(-66.,13.8263796359301,-6.38781142942664));
#50196=CARTESIAN_POINT('Ctrl Pts',(-66.,13.9170340351662,-6.46699483496205));
#50197=CARTESIAN_POINT('Ctrl Pts',(-66.,14.0051400746611,-6.55160160666348));
#50198=CARTESIAN_POINT('Ctrl Pts',(-66.,14.0911063172293,-6.64083299762664));
#50199=CARTESIAN_POINT('Ctrl Pts',(-66.,14.1755812112355,-6.73271726045961));
#50200=CARTESIAN_POINT('Ctrl Pts',(-66.,14.2593394703776,-6.8244480871404));
#50201=CARTESIAN_POINT('Ctrl Pts',(-66.,14.3429542890555,-6.9137592074853));
#50202=CARTESIAN_POINT('Ctrl Pts',(-66.,14.426553270081,-6.99992315179396));
#50203=CARTESIAN_POINT('Ctrl Pts',(-66.,14.5094730904225,-7.08515912713373));
#50204=CARTESIAN_POINT('Ctrl Pts',(-66.,14.5743017306281,-7.15746040594034));
#50205=CARTESIAN_POINT('Ctrl Pts',(-66.,14.6212330452241,-7.21664693024351));
#50206=CARTESIAN_POINT('Ctrl Pts',(-66.,14.6516933118151,-7.2588971478181));
#50207=CARTESIAN_POINT('Ctrl Pts',(-66.,14.6668197205911,-7.28090773432903));
#50208=CARTESIAN_POINT('Ctrl Pts',(-66.,14.6670849864349,-7.28129404712486));
#50209=CARTESIAN_POINT('',(-66.,14.0138288999568,-8.47072751083015));
#50210=CARTESIAN_POINT('Origin',(-66.,0.,0.));
#50211=CARTESIAN_POINT('',(-66.,11.7720642054939,-7.6923605344347));
#50212=CARTESIAN_POINT('Ctrl Pts',(-66.,14.0138288999568,-8.47072751083015));
#50213=CARTESIAN_POINT('Ctrl Pts',(-66.,14.0037053056615,-8.4698799979691));
#50214=CARTESIAN_POINT('Ctrl Pts',(-66.,13.9721524684248,-8.46718145686578));
#50215=CARTESIAN_POINT('Ctrl Pts',(-66.,13.9192737837169,-8.4623570321923));
#50216=CARTESIAN_POINT('Ctrl Pts',(-66.,13.8452784046188,-8.45486947201102));
#50217=CARTESIAN_POINT('Ctrl Pts',(-66.,13.7505117765273,-8.44387618307839));
#50218=CARTESIAN_POINT('Ctrl Pts',(-66.,13.6453014633841,-8.42978304193647));
#50219=CARTESIAN_POINT('Ctrl Pts',(-66.,13.5408537546603,-8.41387978285669));
#50220=CARTESIAN_POINT('Ctrl Pts',(-66.,13.4371309168349,-8.39625156414993));
#50221=CARTESIAN_POINT('Ctrl Pts',(-66.,13.3340674354409,-8.37703230872753));
#50222=CARTESIAN_POINT('Ctrl Pts',(-66.,13.231612467433,-8.35633273843435));
#50223=CARTESIAN_POINT('Ctrl Pts',(-66.,13.1297695959248,-8.33417308930716));
#50224=CARTESIAN_POINT('Ctrl Pts',(-66.,13.0286320818366,-8.31042356359388));
#50225=CARTESIAN_POINT('Ctrl Pts',(-66.,12.9284352169133,-8.284715594814));
#50226=CARTESIAN_POINT('Ctrl Pts',(-66.,12.829511804771,-8.25651874452987));
#50227=CARTESIAN_POINT('Ctrl Pts',(-66.,12.7322148461558,-8.22527363116368));
#50228=CARTESIAN_POINT('Ctrl Pts',(-66.,12.636848388186,-8.19051110794578));
#50229=CARTESIAN_POINT('Ctrl Pts',(-66.,12.5436007236081,-8.15196711241727));
#50230=CARTESIAN_POINT('Ctrl Pts',(-66.,12.4524600493824,-8.10972846142537));
#50231=CARTESIAN_POINT('Ctrl Pts',(-66.,12.3632517496072,-8.06416486307078));
#50232=CARTESIAN_POINT('Ctrl Pts',(-66.,12.2757069077219,-8.01580608992824));
#50233=CARTESIAN_POINT('Ctrl Pts',(-66.,12.1895203359981,-7.96523745572904));
#50234=CARTESIAN_POINT('Ctrl Pts',(-66.,12.1044103376288,-7.91299239895144));
#50235=CARTESIAN_POINT('Ctrl Pts',(-66.,12.0201833141302,-7.85943599303422));
#50236=CARTESIAN_POINT('Ctrl Pts',(-66.,11.936722320441,-7.80478766329085));
#50237=CARTESIAN_POINT('Ctrl Pts',(-66.,11.870517618491,-7.7602860336664));
#50238=CARTESIAN_POINT('Ctrl Pts',(-66.,11.8211715224307,-7.72648734423527));
#50239=CARTESIAN_POINT('Ctrl Pts',(-66.,11.7884105699588,-7.70376738782835));
#50240=CARTESIAN_POINT('Ctrl Pts',(-66.,11.7720642054939,-7.69236053443469));
#50241=CARTESIAN_POINT('',(-66.,10.9536375103364,-8.81882824088046));
#50242=CARTESIAN_POINT('Origin',(-66.,0.,0.));
#50243=CARTESIAN_POINT('',(-66.,12.3955073457098,-10.7000945155851));
#50244=CARTESIAN_POINT('Ctrl Pts',(-66.,10.9536375103364,-8.81882824088046));
#50245=CARTESIAN_POINT('Ctrl Pts',(-66.,10.9724295263217,-8.83272480732197));
#50246=CARTESIAN_POINT('Ctrl Pts',(-66.,11.0098871540402,-8.86070419148627));
#50247=CARTESIAN_POINT('Ctrl Pts',(-66.,11.0656943951459,-8.90323201632451));
#50248=CARTESIAN_POINT('Ctrl Pts',(-66.,11.1393445344495,-8.96105481127105));
#50249=CARTESIAN_POINT('Ctrl Pts',(-66.,11.2300954828748,-9.03523227310488));
#50250=CARTESIAN_POINT('Ctrl Pts',(-66.,11.3194051551598,-9.11139639219764));
#50251=CARTESIAN_POINT('Ctrl Pts',(-66.,11.407025252502,-9.18970993907287));
#50252=CARTESIAN_POINT('Ctrl Pts',(-66.,11.4925391231036,-9.27043802686381));
#50253=CARTESIAN_POINT('Ctrl Pts',(-66.,11.5754278219505,-9.35393513817802));
#50254=CARTESIAN_POINT('Ctrl Pts',(-66.,11.655157779328,-9.44063172122792));
#50255=CARTESIAN_POINT('Ctrl Pts',(-66.,11.7312595885623,-9.53100857350628));
#50256=CARTESIAN_POINT('Ctrl Pts',(-66.,11.8034143911192,-9.62560737856555));
#50257=CARTESIAN_POINT('Ctrl Pts',(-66.,11.8715286035136,-9.724847924125));
#50258=CARTESIAN_POINT('Ctrl Pts',(-66.,11.9358257812543,-9.82870769953299));
#50259=CARTESIAN_POINT('Ctrl Pts',(-66.,11.9969002916812,-9.93651465742827));
#50260=CARTESIAN_POINT('Ctrl Pts',(-66.,12.0558705645975,-10.0465202590396));
#50261=CARTESIAN_POINT('Ctrl Pts',(-66.,12.1141848750712,-10.1561990251342));
#50262=CARTESIAN_POINT('Ctrl Pts',(-66.,12.1729620080223,-10.2634984322242));
#50263=CARTESIAN_POINT('Ctrl Pts',(-66.,12.2325064717433,-10.3677455989363));
#50264=CARTESIAN_POINT('Ctrl Pts',(-66.,12.2916238883603,-10.4709250501372));
#50265=CARTESIAN_POINT('Ctrl Pts',(-66.,12.336435220754,-10.5570770785351));
#50266=CARTESIAN_POINT('Ctrl Pts',(-66.,12.3671730117507,-10.6260754926723));
#50267=CARTESIAN_POINT('Ctrl Pts',(-66.,12.3861691112129,-10.6745735022306));
#50268=CARTESIAN_POINT('Ctrl Pts',(-66.,12.3953464857659,-10.6996543705834));
#50269=CARTESIAN_POINT('Ctrl Pts',(-66.,12.3955073457098,-10.7000945155851));
#50270=CARTESIAN_POINT('',(-66.,11.4669744265634,-11.689701557377));
#50271=CARTESIAN_POINT('Origin',(-66.,0.,0.));
#50272=CARTESIAN_POINT('',(-66.,9.48921088782657,-10.3782842019456));
#50273=CARTESIAN_POINT('Ctrl Pts',(-66.,11.4669744265634,-11.689701557377));
#50274=CARTESIAN_POINT('Ctrl Pts',(-66.,11.4573796514766,-11.6863630351679));
#50275=CARTESIAN_POINT('Ctrl Pts',(-66.,11.4274892045258,-11.6759024021635));
#50276=CARTESIAN_POINT('Ctrl Pts',(-66.,11.3774715865628,-11.6580791515292));
#50277=CARTESIAN_POINT('Ctrl Pts',(-66.,11.3076629888636,-11.632424924341));
#50278=CARTESIAN_POINT('Ctrl Pts',(-66.,11.2186075484415,-11.5982095077484));
#50279=CARTESIAN_POINT('Ctrl Pts',(-66.,11.1202074324343,-11.5583943876468));
#50280=CARTESIAN_POINT('Ctrl Pts',(-66.,11.0229961202521,-11.5170156697979));
#50281=CARTESIAN_POINT('Ctrl Pts',(-66.,10.926915885831,-11.4741464531626));
#50282=CARTESIAN_POINT('Ctrl Pts',(-66.,10.8318699676878,-11.4299001604323));
#50283=CARTESIAN_POINT('Ctrl Pts',(-66.,10.737781584702,-11.3843713907704));
#50284=CARTESIAN_POINT('Ctrl Pts',(-66.,10.6446491749193,-11.3375806355454));
#50285=CARTESIAN_POINT('Ctrl Pts',(-66.,10.5525953486849,-11.289425367888));
#50286=CARTESIAN_POINT('Ctrl Pts',(-66.,10.4619396643774,-11.2396071151889));
#50287=CARTESIAN_POINT('Ctrl Pts',(-66.,10.3731363846505,-11.1876948686032));
#50288=CARTESIAN_POINT('Ctrl Pts',(-66.,10.2866665326243,-11.1332346082697));
#50289=CARTESIAN_POINT('Ctrl Pts',(-66.,10.2029412752749,-11.0758475399707));
#50290=CARTESIAN_POINT('Ctrl Pts',(-66.,10.1222086594491,-11.0153247237569));
#50291=CARTESIAN_POINT('Ctrl Pts',(-66.,10.0444356624493,-10.951747313668));
#50292=CARTESIAN_POINT('Ctrl Pts',(-66.,9.9693612115878,-10.885429977536));
#50293=CARTESIAN_POINT('Ctrl Pts',(-66.,9.89659308973021,-10.816818967327));
#50294=CARTESIAN_POINT('Ctrl Pts',(-66.,9.82569013557624,-10.7464053109633));
#50295=CARTESIAN_POINT('Ctrl Pts',(-66.,9.75624684158698,-10.6746356328252));
#50296=CARTESIAN_POINT('Ctrl Pts',(-66.,9.68798490145875,-10.6018153909131));
#50297=CARTESIAN_POINT('Ctrl Pts',(-66.,9.62073647531797,-10.5281280338367));
#50298=CARTESIAN_POINT('Ctrl Pts',(-66.,9.56767882107163,-10.4685600648819));
#50299=CARTESIAN_POINT('Ctrl Pts',(-66.,9.52828841562115,-10.4235513483695));
#50300=CARTESIAN_POINT('Ctrl Pts',(-66.,9.50220693210954,-10.3933978635985));
#50301=CARTESIAN_POINT('Ctrl Pts',(-66.,9.48921088782658,-10.3782842019456));
#50302=CARTESIAN_POINT('',(-66.,8.41635544546801,-11.2658274114927));
#50303=CARTESIAN_POINT('Origin',(-66.,0.,0.));
#50304=CARTESIAN_POINT('',(-66.,9.34507439096662,-13.4465686934362));
#50305=CARTESIAN_POINT('Ctrl Pts',(-66.,8.41635544546801,-11.2658274114927));
#50306=CARTESIAN_POINT('Ctrl Pts',(-66.,8.43110114017464,-11.2839607760805));
#50307=CARTESIAN_POINT('Ctrl Pts',(-66.,8.46042377774785,-11.3203764696515));
#50308=CARTESIAN_POINT('Ctrl Pts',(-66.,8.50390149179148,-11.3754469011628));
#50309=CARTESIAN_POINT('Ctrl Pts',(-66.,8.56085783218497,-11.4497691315105));
#50310=CARTESIAN_POINT('Ctrl Pts',(-66.,8.63031048807256,-11.544185015102));
#50311=CARTESIAN_POINT('Ctrl Pts',(-66.,8.69787308659046,-11.6401667106607));
#50312=CARTESIAN_POINT('Ctrl Pts',(-66.,8.76326465031677,-11.7378101255738));
#50313=CARTESIAN_POINT('Ctrl Pts',(-66.,8.8260156863806,-11.8372684268691));
#50314=CARTESIAN_POINT('Ctrl Pts',(-66.,8.88553539714026,-11.9387559040544));
#50315=CARTESIAN_POINT('Ctrl Pts',(-66.,8.94119992783734,-12.0425567886278));
#50316=CARTESIAN_POINT('Ctrl Pts',(-66.,8.99243504959771,-12.149020036252));
#50317=CARTESIAN_POINT('Ctrl Pts',(-66.,9.03879721019277,-12.2585910156016));
#50318=CARTESIAN_POINT('Ctrl Pts',(-66.,9.08009136927418,-12.3716530527263));
#50319=CARTESIAN_POINT('Ctrl Pts',(-66.,9.11653965711474,-12.4882399401825));
#50320=CARTESIAN_POINT('Ctrl Pts',(-66.,9.14888489929381,-12.6078485573591));
#50321=CARTESIAN_POINT('Ctrl Pts',(-66.,9.17864523199547,-12.7290634412273));
#50322=CARTESIAN_POINT('Ctrl Pts',(-66.,9.20785149120868,-12.8497986264917));
#50323=CARTESIAN_POINT('Ctrl Pts',(-66.,9.23809775500251,-12.9683443039596));
#50324=CARTESIAN_POINT('Ctrl Pts',(-66.,9.26984630377419,-13.0841244601964));
#50325=CARTESIAN_POINT('Ctrl Pts',(-66.,9.30144675196197,-13.1987642428721));
#50326=CARTESIAN_POINT('Ctrl Pts',(-66.,9.32342511572492,-13.293353772072));
#50327=CARTESIAN_POINT('Ctrl Pts',(-66.,9.33603801466832,-13.3678286519246));
#50328=CARTESIAN_POINT('Ctrl Pts',(-66.,9.3423763522097,-13.4195271451628));
#50329=CARTESIAN_POINT('Ctrl Pts',(-66.,9.34502804434446,-13.4461023721578));
#50330=CARTESIAN_POINT('Ctrl Pts',(-66.,9.34507439096662,-13.4465686934362));
#50331=CARTESIAN_POINT('',(-66.,8.199607777367,-14.1741686633588));
#50332=CARTESIAN_POINT('Origin',(-66.,0.,0.));
#50333=CARTESIAN_POINT('',(-66.,6.61011555120063,-12.4121021043889));
#50334=CARTESIAN_POINT('Ctrl Pts',(-66.,8.199607777367,-14.1741686633588));
#50335=CARTESIAN_POINT('Ctrl Pts',(-66.,8.19114469649464,-14.1685489034304));
#50336=CARTESIAN_POINT('Ctrl Pts',(-66.,8.16479476654098,-14.150983458568));
#50337=CARTESIAN_POINT('Ctrl Pts',(-66.,8.1207810062114,-14.1212812823596));
#50338=CARTESIAN_POINT('Ctrl Pts',(-66.,8.05954552084273,-14.0790723376084));
#50339=CARTESIAN_POINT('Ctrl Pts',(-66.,7.98179694893469,-14.0237846738158));
#50340=CARTESIAN_POINT('Ctrl Pts',(-66.,7.89638987124254,-13.9607493051802));
#50341=CARTESIAN_POINT('Ctrl Pts',(-66.,7.81252309986449,-13.8964951055849));
#50342=CARTESIAN_POINT('Ctrl Pts',(-66.,7.7301225433348,-13.8310785215643));
#50343=CARTESIAN_POINT('Ctrl Pts',(-66.,7.6490662730339,-13.7645853488249));
#50344=CARTESIAN_POINT('Ctrl Pts',(-66.,7.56925639420599,-13.6970881198352));
#50345=CARTESIAN_POINT('Ctrl Pts',(-66.,7.49068629797234,-13.6286062937474));
#50346=CARTESIAN_POINT('Ctrl Pts',(-66.,7.41350024004436,-13.5590710567155));
#50347=CARTESIAN_POINT('Ctrl Pts',(-66.,7.33808196640605,-13.4882727841331));
#50348=CARTESIAN_POINT('Ctrl Pts',(-66.,7.26497865575545,-13.4159069786186));
#50349=CARTESIAN_POINT('Ctrl Pts',(-66.,7.19476912913493,-13.3416535097654));
#50350=CARTESIAN_POINT('Ctrl Pts',(-66.,7.12794583824513,-13.2652477369413));
#50351=CARTESIAN_POINT('Ctrl Pts',(-66.,7.06480099833745,-13.1865489711723));
#50352=CARTESIAN_POINT('Ctrl Pts',(-66.,7.00528244199424,-13.1056276044837));
#50353=CARTESIAN_POINT('Ctrl Pts',(-66.,6.94905904389849,-13.0227234927017));
#50354=CARTESIAN_POINT('Ctrl Pts',(-66.,6.89563993078743,-12.9381713275312));
#50355=CARTESIAN_POINT('Ctrl Pts',(-66.,6.84447568757558,-12.8523369979956));
#50356=CARTESIAN_POINT('Ctrl Pts',(-66.,6.79506247552229,-12.7655522513249));
#50357=CARTESIAN_POINT('Ctrl Pts',(-66.,6.74705476751256,-12.6780437370314));
#50358=CARTESIAN_POINT('Ctrl Pts',(-66.,6.70024437485702,-12.5899474002701));
#50359=CARTESIAN_POINT('Ctrl Pts',(-66.,6.66366757586302,-12.5190559665502));
#50360=CARTESIAN_POINT('Ctrl Pts',(-66.,6.63670790506457,-12.4656652861453));
#50361=CARTESIAN_POINT('Ctrl Pts',(-66.,6.6189446860433,-12.4299729273552));
#50362=CARTESIAN_POINT('Ctrl Pts',(-66.,6.61011555120064,-12.4121021043889));
#50363=CARTESIAN_POINT('',(-66.,5.35024281477071,-13.004953213026));
#50364=CARTESIAN_POINT('Origin',(-66.,0.,0.));
#50365=CARTESIAN_POINT('',(-66.,5.70745604345953,-15.3481455072584));
#50366=CARTESIAN_POINT('Ctrl Pts',(-66.,5.35024281477071,-13.004953213026));
#50367=CARTESIAN_POINT('Ctrl Pts',(-66.,5.36001566196946,-13.026183989773));
#50368=CARTESIAN_POINT('Ctrl Pts',(-66.,5.37936086023753,-13.0687478607962));
#50369=CARTESIAN_POINT('Ctrl Pts',(-66.,5.40777718254589,-13.1329006212338));
#50370=CARTESIAN_POINT('Ctrl Pts',(-66.,5.44446094769152,-13.2190523479119));
#50371=CARTESIAN_POINT('Ctrl Pts',(-66.,5.48825134524296,-13.3277741560577));
#50372=CARTESIAN_POINT('Ctrl Pts',(-66.,5.52982166345111,-13.4375425451545));
#50373=CARTESIAN_POINT('Ctrl Pts',(-66.,5.56887590111916,-13.548380533239));
#50374=CARTESIAN_POINT('Ctrl Pts',(-66.,5.60492122426722,-13.6603197171863));
#50375=CARTESIAN_POINT('Ctrl Pts',(-66.,5.63733210461441,-13.7734207288063));
#50376=CARTESIAN_POINT('Ctrl Pts',(-66.,5.66543360144756,-13.8878037235725));
#50377=CARTESIAN_POINT('Ctrl Pts',(-66.,5.68858274460417,-14.0036638891498));
#50378=CARTESIAN_POINT('Ctrl Pts',(-66.,5.7062391581791,-14.1213222951832));
#50379=CARTESIAN_POINT('Ctrl Pts',(-66.,5.71811860006313,-14.2411017202677));
#50380=CARTESIAN_POINT('Ctrl Pts',(-66.,5.7244278180311,-14.3630901368566));
#50381=CARTESIAN_POINT('Ctrl Pts',(-66.,5.72601142143879,-14.4869849640075));
#50382=CARTESIAN_POINT('Ctrl Pts',(-66.,5.72469186277131,-14.611792753182));
#50383=CARTESIAN_POINT('Ctrl Pts',(-66.,5.72295493404455,-14.7359981218931));
#50384=CARTESIAN_POINT('Ctrl Pts',(-66.,5.72276984468895,-14.8583414088431));
#50385=CARTESIAN_POINT('Ctrl Pts',(-66.,5.72472760042901,-14.9783796615786));
#50386=CARTESIAN_POINT('Ctrl Pts',(-66.,5.72682550780959,-15.0972765365679));
#50387=CARTESIAN_POINT('Ctrl Pts',(-66.,5.72458992151581,-15.1943601585744));
#50388=CARTESIAN_POINT('Ctrl Pts',(-66.,5.71828541357827,-15.2696319735416));
#50389=CARTESIAN_POINT('Ctrl Pts',(-66.,5.7115677281404,-15.3212825439959));
#50390=CARTESIAN_POINT('Ctrl Pts',(-66.,5.70752712228784,-15.3476823103842));
#50391=CARTESIAN_POINT('Ctrl Pts',(-66.,5.70745604345953,-15.3481455072584));
#50392=CARTESIAN_POINT('',(-66.,4.41702961547073,-15.7680206232759));
#50393=CARTESIAN_POINT('Origin',(-66.,0.,0.));
#50394=CARTESIAN_POINT('',(-66.,3.31568234418831,-13.6660219830951));
#50395=CARTESIAN_POINT('Ctrl Pts',(-66.,4.41702961547073,-15.7680206232759));
#50396=CARTESIAN_POINT('Ctrl Pts',(-66.,4.41022999530899,-15.7604727358124));
#50397=CARTESIAN_POINT('Ctrl Pts',(-66.,4.38907624535977,-15.7369061805941));
#50398=CARTESIAN_POINT('Ctrl Pts',(-66.,4.35383188909641,-15.6971913757796));
#50399=CARTESIAN_POINT('Ctrl Pts',(-66.,4.30501716681229,-15.6410798566978));
#50400=CARTESIAN_POINT('Ctrl Pts',(-66.,4.24346069213056,-15.5681938729551));
#50401=CARTESIAN_POINT('Ctrl Pts',(-66.,4.17641309355012,-15.4858989998248));
#50402=CARTESIAN_POINT('Ctrl Pts',(-66.,4.11116052066234,-15.4028066461541));
#50403=CARTESIAN_POINT('Ctrl Pts',(-66.,4.04761717203886,-15.3189530593075));
#50404=CARTESIAN_POINT('Ctrl Pts',(-66.,3.98564361314731,-15.2343910171469));
#50405=CARTESIAN_POINT('Ctrl Pts',(-66.,3.92512698668427,-15.1491664279643));
#50406=CARTESIAN_POINT('Ctrl Pts',(-66.,3.8660560521067,-15.0632964960055));
#50407=CARTESIAN_POINT('Ctrl Pts',(-66.,3.80858764637521,-14.9767504442745));
#50408=CARTESIAN_POINT('Ctrl Pts',(-66.,3.75314559090774,-14.8894206676529));
#50409=CARTESIAN_POINT('Ctrl Pts',(-66.,3.7003355991968,-14.801148312913));
#50410=CARTESIAN_POINT('Ctrl Pts',(-66.,3.65079792075207,-14.7117672540732));
#50411=CARTESIAN_POINT('Ctrl Pts',(-66.,3.60507534944737,-14.6211436324314));
#50412=CARTESIAN_POINT('Ctrl Pts',(-66.,3.56348590797974,-14.5292138499942));
#50413=CARTESIAN_POINT('Ctrl Pts',(-66.,3.52596156208203,-14.436033113783));
#50414=CARTESIAN_POINT('Ctrl Pts',(-66.,3.49212193962963,-14.3417513965941));
#50415=CARTESIAN_POINT('Ctrl Pts',(-66.,3.46140835460361,-14.246570799961));
#50416=CARTESIAN_POINT('Ctrl Pts',(-66.,3.43319765990381,-14.1507090838548));
#50417=CARTESIAN_POINT('Ctrl Pts',(-66.,3.40691934362888,-14.0543622734568));
#50418=CARTESIAN_POINT('Ctrl Pts',(-66.,3.38218236859189,-13.9576639685687));
#50419=CARTESIAN_POINT('Ctrl Pts',(-66.,3.35875127854871,-13.860694068957));
#50420=CARTESIAN_POINT('Ctrl Pts',(-66.,3.34095358960791,-13.7829335399729));
#50421=CARTESIAN_POINT('Ctrl Pts',(-66.,3.3281186287285,-13.7245156284827));
#50422=CARTESIAN_POINT('Ctrl Pts',(-66.,3.31978980257722,-13.6855270778435));
#50423=CARTESIAN_POINT('Ctrl Pts',(-66.,3.31568234418832,-13.6660219830951));
#50424=CARTESIAN_POINT('',(-66.,1.94795475120472,-13.9269299753125));
#50425=CARTESIAN_POINT('Origin',(-66.,0.,0.));
#50426=CARTESIAN_POINT('',(-66.,1.71121724218688,-16.2853418923289));
#50427=CARTESIAN_POINT('Ctrl Pts',(-66.,1.94795475120472,-13.9269299753125));
#50428=CARTESIAN_POINT('Ctrl Pts',(-66.,1.95214068696407,-13.9499241564345));
#50429=CARTESIAN_POINT('Ctrl Pts',(-66.,1.96029291597316,-13.9959617603545));
#50430=CARTESIAN_POINT('Ctrl Pts',(-66.,1.9718623445077,-14.0651658958429));
#50431=CARTESIAN_POINT('Ctrl Pts',(-66.,1.98596855852791,-14.1577338890203));
#50432=CARTESIAN_POINT('Ctrl Pts',(-66.,2.00134518601523,-14.2739302306637));
#50433=CARTESIAN_POINT('Ctrl Pts',(-66.,2.01431120793567,-14.3905881617116));
#50434=CARTESIAN_POINT('Ctrl Pts',(-66.,2.02457419816135,-14.5076563645426));
#50435=CARTESIAN_POINT('Ctrl Pts',(-66.,2.03164894817481,-14.625042880531));
#50436=CARTESIAN_POINT('Ctrl Pts',(-66.,2.03491450329845,-14.7426508740692));
#50437=CARTESIAN_POINT('Ctrl Pts',(-66.,2.03368724587156,-14.8604288747958));
#50438=CARTESIAN_POINT('Ctrl Pts',(-66.,2.02729586462329,-14.9784060380191));
#50439=CARTESIAN_POINT('Ctrl Pts',(-66.,2.01513711377743,-15.096758960368));
#50440=CARTESIAN_POINT('Ctrl Pts',(-66.,1.99685540944097,-15.2157295916163));
#50441=CARTESIAN_POINT('Ctrl Pts',(-66.,1.97262912616775,-15.3354545564815));
#50442=CARTESIAN_POINT('Ctrl Pts',(-66.,1.94335158717786,-15.4558508259636));
#50443=CARTESIAN_POINT('Ctrl Pts',(-66.,1.91103504986532,-15.5764093880396));
#50444=CARTESIAN_POINT('Ctrl Pts',(-66.,1.87846407081847,-15.6962806600859));
#50445=CARTESIAN_POINT('Ctrl Pts',(-66.,1.84785925815835,-15.8147342778518));
#50446=CARTESIAN_POINT('Ctrl Pts',(-66.,1.81990320787353,-15.9314881821968));
#50447=CARTESIAN_POINT('Ctrl Pts',(-66.,1.79236675521062,-16.047171421572));
#50448=CARTESIAN_POINT('Ctrl Pts',(-66.,1.76605768896888,-16.1406490153657));
#50449=CARTESIAN_POINT('Ctrl Pts',(-66.,1.74123190957046,-16.211988160483));
#50450=CARTESIAN_POINT('Ctrl Pts',(-66.,1.72188029803531,-16.2603454128541));
#50451=CARTESIAN_POINT('Ctrl Pts',(-66.,1.71140128032148,-16.284910924222));
#50452=CARTESIAN_POINT('Ctrl Pts',(-66.,1.71121724218688,-16.2853418923289));
#50453=CARTESIAN_POINT('',(-66.,0.356913238135829,-16.3711098567093));
#50454=CARTESIAN_POINT('Origin',(-66.,0.,0.));
#50455=CARTESIAN_POINT('',(-66.,-0.187087378736044,-14.0612554404903));
#50456=CARTESIAN_POINT('Ctrl Pts',(-66.,0.356913238135829,-16.3711098567093));
#50457=CARTESIAN_POINT('Ctrl Pts',(-66.,0.352204323826719,-16.3621081032393));
#50458=CARTESIAN_POINT('Ctrl Pts',(-66.,0.337575921789304,-16.3340212110009));
#50459=CARTESIAN_POINT('Ctrl Pts',(-66.,0.313315502115871,-16.2867892048278));
#50460=CARTESIAN_POINT('Ctrl Pts',(-66.,0.279988751445404,-16.220300804523));
#50461=CARTESIAN_POINT('Ctrl Pts',(-66.,0.238492193683111,-16.1343961952447));
#50462=CARTESIAN_POINT('Ctrl Pts',(-66.,0.194016921417006,-16.0380127071578));
#50463=CARTESIAN_POINT('Ctrl Pts',(-66.,0.151478606156202,-15.9413031975852));
#50464=CARTESIAN_POINT('Ctrl Pts',(-66.,0.110785127729046,-15.844281437166));
#50465=CARTESIAN_POINT('Ctrl Pts',(-66.,0.0717883068748032,-15.7469638696907));
#50466=CARTESIAN_POINT('Ctrl Pts',(-66.,0.0343674149818962,-15.6493668946876));
#50467=CARTESIAN_POINT('Ctrl Pts',(-66.,-0.00149271387238248,-15.5515043804903));
#50468=CARTESIAN_POINT('Ctrl Pts',(-66.,-0.0356325161212601,-15.4533855207845));
#50469=CARTESIAN_POINT('Ctrl Pts',(-66.,-0.0676147251712506,-15.3550114911653));
#50470=CARTESIAN_POINT('Ctrl Pts',(-66.,-0.0968131519417803,-15.2563790638913));
#50471=CARTESIAN_POINT('Ctrl Pts',(-66.,-0.122566347687195,-15.1574865557124));
#50472=CARTESIAN_POINT('Ctrl Pts',(-66.,-0.144315282095873,-15.058339300691));
#50473=CARTESIAN_POINT('Ctrl Pts',(-66.,-0.161736107560775,-14.9589547879103));
#50474=CARTESIAN_POINT('Ctrl Pts',(-66.,-0.174908450355344,-14.8593695705273));
#50475=CARTESIAN_POINT('Ctrl Pts',(-66.,-0.184238029232279,-14.7596343149665));
#50476=CARTESIAN_POINT('Ctrl Pts',(-66.,-0.190316238669402,-14.6598058338069));
#50477=CARTESIAN_POINT('Ctrl Pts',(-66.,-0.19380080315749,-14.5599400753078));
#50478=CARTESIAN_POINT('Ctrl Pts',(-66.,-0.195293060397626,-14.4600850256186));
#50479=CARTESIAN_POINT('Ctrl Pts',(-66.,-0.195204987344071,-14.3602728402636));
#50480=CARTESIAN_POINT('Ctrl Pts',(-66.,-0.193784513213942,-14.2605223532243));
#50481=CARTESIAN_POINT('Ctrl Pts',(-66.,-0.191684797850075,-14.1807787089954));
#50482=CARTESIAN_POINT('Ctrl Pts',(-66.,-0.189588581014708,-14.1210041786448));
#50483=CARTESIAN_POINT('Ctrl Pts',(-66.,-0.187959683517641,-14.0811692301831));
#50484=CARTESIAN_POINT('Ctrl Pts',(-66.,-0.187087378736032,-14.0612554404903));
#50485=CARTESIAN_POINT('',(-66.,-1.57673047345591,-13.9738265075847));
#50486=CARTESIAN_POINT('Origin',(-66.,0.,0.));
#50487=CARTESIAN_POINT('',(-66.,-2.39254363182917,-16.1992703530064));
#50488=CARTESIAN_POINT('Ctrl Pts',(-66.,-1.57673047345591,-13.9738265075847));
#50489=CARTESIAN_POINT('Ctrl Pts',(-66.,-1.57839446687451,-13.997139284115));
#50490=CARTESIAN_POINT('Ctrl Pts',(-66.,-1.58194744165485,-14.0437579089631));
#50491=CARTESIAN_POINT('Ctrl Pts',(-66.,-1.58795185663835,-14.1136650691543));
#50492=CARTESIAN_POINT('Ctrl Pts',(-66.,-1.59730953904946,-14.2068329413785));
#50493=CARTESIAN_POINT('Ctrl Pts',(-66.,-1.61131285168258,-14.3232027730338));
#50494=CARTESIAN_POINT('Ctrl Pts',(-66.,-1.6277658288928,-14.4394201991873));
#50495=CARTESIAN_POINT('Ctrl Pts',(-66.,-1.64693894753001,-14.5553627910342));
#50496=CARTESIAN_POINT('Ctrl Pts',(-66.,-1.6692793032136,-14.6708208125467));
#50497=CARTESIAN_POINT('Ctrl Pts',(-66.,-1.69536426015181,-14.7855460452371));
#50498=CARTESIAN_POINT('Ctrl Pts',(-66.,-1.72584315874106,-14.8993186269813));
#50499=CARTESIAN_POINT('Ctrl Pts',(-66.,-1.76137347040452,-15.0119998487957));
#50500=CARTESIAN_POINT('Ctrl Pts',(-66.,-1.80258340663877,-15.1236107380773));
#50501=CARTESIAN_POINT('Ctrl Pts',(-66.,-1.84987755047685,-15.2342972131845));
#50502=CARTESIAN_POINT('Ctrl Pts',(-66.,-1.90311710851519,-15.3442359664661));
#50503=CARTESIAN_POINT('Ctrl Pts',(-66.,-1.96141617445265,-15.4535687378813));
#50504=CARTESIAN_POINT('Ctrl Pts',(-66.,-2.02269912351901,-15.5623029350202));
#50505=CARTESIAN_POINT('Ctrl Pts',(-66.,-2.08405759848474,-15.6703081575233));
#50506=CARTESIAN_POINT('Ctrl Pts',(-66.,-2.14315912151332,-15.777429229659));
#50507=CARTESIAN_POINT('Ctrl Pts',(-66.,-2.19927239636847,-15.8835627084126));
#50508=CARTESIAN_POINT('Ctrl Pts',(-66.,-2.25471299248206,-15.9887635087906));
#50509=CARTESIAN_POINT('Ctrl Pts',(-66.,-2.30344244328183,-16.0727615333669));
#50510=CARTESIAN_POINT('Ctrl Pts',(-66.,-2.34522959911868,-16.1356855077795));
#50511=CARTESIAN_POINT('Ctrl Pts',(-66.,-2.3759992038281,-16.1777109780555));
#50512=CARTESIAN_POINT('Ctrl Pts',(-66.,-2.39225819818114,-16.1988986929781));
#50513=CARTESIAN_POINT('Ctrl Pts',(-66.,-2.39254363182917,-16.1992703530064));
#50514=CARTESIAN_POINT('',(-66.,-3.7256293105862,-15.9455420491152));
#50515=CARTESIAN_POINT('Origin',(-66.,0.,0.));
#50516=CARTESIAN_POINT('',(-66.,-3.67810171359515,-13.5729685048794));
#50517=CARTESIAN_POINT('Ctrl Pts',(-66.,-3.7256293105862,-15.9455420491152));
#50518=CARTESIAN_POINT('Ctrl Pts',(-66.,-3.72795164063846,-15.9356520429153));
#50519=CARTESIAN_POINT('Ctrl Pts',(-66.,-3.73513553846456,-15.9048096163928));
#50520=CARTESIAN_POINT('Ctrl Pts',(-66.,-3.74688765015641,-15.853028169516));
#50521=CARTESIAN_POINT('Ctrl Pts',(-66.,-3.76263238690138,-15.7803405987066));
#50522=CARTESIAN_POINT('Ctrl Pts',(-66.,-3.78146164640637,-15.6868150664286));
#50523=CARTESIAN_POINT('Ctrl Pts',(-66.,-3.80057004743305,-15.5823990924153));
#50524=CARTESIAN_POINT('Ctrl Pts',(-66.,-3.81772126627406,-15.4781490410999));
#50525=CARTESIAN_POINT('Ctrl Pts',(-66.,-3.83300795359517,-15.3740553411364));
#50526=CARTESIAN_POINT('Ctrl Pts',(-66.,-3.84657772273756,-15.2700970690198));
#50527=CARTESIAN_POINT('Ctrl Pts',(-66.,-3.85855158779829,-15.1662600850723));
#50528=CARTESIAN_POINT('Ctrl Pts',(-66.,-3.86894768714904,-15.0625540503165));
#50529=CARTESIAN_POINT('Ctrl Pts',(-66.,-3.87761375658259,-14.9590275514473));
#50530=CARTESIAN_POINT('Ctrl Pts',(-66.,-3.88412655939816,-14.8557904709058));
#50531=CARTESIAN_POINT('Ctrl Pts',(-66.,-3.88787877668998,-14.7529954092481));
#50532=CARTESIAN_POINT('Ctrl Pts',(-66.,-3.88822932173376,-14.6508052317201));
#50533=CARTESIAN_POINT('Ctrl Pts',(-66.,-3.88463805371054,-14.5493641299902));
#50534=CARTESIAN_POINT('Ctrl Pts',(-66.,-3.87679564863944,-14.4487695813147));
#50535=CARTESIAN_POINT('Ctrl Pts',(-66.,-3.86478832158859,-14.3490371882169));
#50536=CARTESIAN_POINT('Ctrl Pts',(-66.,-3.84902164513744,-14.2501151271916));
#50537=CARTESIAN_POINT('Ctrl Pts',(-66.,-3.83008256273264,-14.1519113521203));
#50538=CARTESIAN_POINT('Ctrl Pts',(-66.,-3.8086220490069,-14.0543164841154));
#50539=CARTESIAN_POINT('Ctrl Pts',(-66.,-3.7852344832017,-13.9572274551481));
#50540=CARTESIAN_POINT('Ctrl Pts',(-66.,-3.76032689601146,-13.8605729560155));
#50541=CARTESIAN_POINT('Ctrl Pts',(-66.,-3.73414411132176,-13.764309571506));
#50542=CARTESIAN_POINT('Ctrl Pts',(-66.,-3.71227892449176,-13.6875933984758));
#50543=CARTESIAN_POINT('Ctrl Pts',(-66.,-3.69538324295473,-13.6302181028421));
#50544=CARTESIAN_POINT('Ctrl Pts',(-66.,-3.68389897142971,-13.5920397328724));
#50545=CARTESIAN_POINT('Ctrl Pts',(-66.,-3.67810171359514,-13.5729685048794));
#50546=CARTESIAN_POINT('',(-66.,-5.00234392366024,-13.1426961282463));
#50547=CARTESIAN_POINT('Origin',(-66.,0.,0.));
#50548=CARTESIAN_POINT('',(-66.,-6.34597219029742,-15.0953390806557));
#50549=CARTESIAN_POINT('Ctrl Pts',(-66.,-5.00234392366024,-13.1426961282463));
#50550=CARTESIAN_POINT('Ctrl Pts',(-66.,-5.00975329143057,-13.1648626726972));
#50551=CARTESIAN_POINT('Ctrl Pts',(-66.,-5.02478822352796,-13.2091330988228));
#50552=CARTESIAN_POINT('Ctrl Pts',(-66.,-5.04798920255339,-13.2753507597416));
#50553=CARTESIAN_POINT('Ctrl Pts',(-66.,-5.08022280379478,-13.3632644309532));
#50554=CARTESIAN_POINT('Ctrl Pts',(-66.,-5.12272617691501,-13.4724958081193));
#50555=CARTESIAN_POINT('Ctrl Pts',(-66.,-5.16756435218796,-13.5809703610753));
#50556=CARTESIAN_POINT('Ctrl Pts',(-66.,-5.21496886213029,-13.6885022424853));
#50557=CARTESIAN_POINT('Ctrl Pts',(-66.,-5.26532059680125,-13.7947771174053));
#50558=CARTESIAN_POINT('Ctrl Pts',(-66.,-5.31911705202313,-13.8994109809482));
#50559=CARTESIAN_POINT('Ctrl Pts',(-66.,-5.37693249048282,-14.0020293939727));
#50560=CARTESIAN_POINT('Ctrl Pts',(-66.,-5.43936923240832,-14.102334498799));
#50561=CARTESIAN_POINT('Ctrl Pts',(-66.,-5.50704098217782,-14.2001904323636));
#50562=CARTESIAN_POINT('Ctrl Pts',(-66.,-5.58037590052447,-14.2956379130225));
#50563=CARTESIAN_POINT('Ctrl Pts',(-66.,-5.65928349609497,-14.3888825985252));
#50564=CARTESIAN_POINT('Ctrl Pts',(-66.,-5.7429409442582,-14.4802820917477));
#50565=CARTESIAN_POINT('Ctrl Pts',(-66.,-5.8293396720056,-14.5703597544468));
#50566=CARTESIAN_POINT('Ctrl Pts',(-66.,-5.91563026424745,-14.6597125620614));
#50567=CARTESIAN_POINT('Ctrl Pts',(-66.,-5.99951493159239,-14.7487702776409));
#50568=CARTESIAN_POINT('Ctrl Pts',(-66.,-6.08025962758854,-14.8376145740015));
#50569=CARTESIAN_POINT('Ctrl Pts',(-66.,-6.16012083060275,-14.925722782193));
#50570=CARTESIAN_POINT('Ctrl Pts',(-66.,-6.22820881535241,-14.9949633327447));
#50571=CARTESIAN_POINT('Ctrl Pts',(-66.,-6.28433170694406,-15.045518391722));
#50572=CARTESIAN_POINT('Ctrl Pts',(-66.,-6.32458593740117,-15.0785714650465));
#50573=CARTESIAN_POINT('Ctrl Pts',(-66.,-6.3456032959818,-15.0950500814723));
#50574=CARTESIAN_POINT('Ctrl Pts',(-66.,-6.34597219029742,-15.0953390806557));
#50575=CARTESIAN_POINT('',(-66.,-7.57407686781798,-14.5180571909737));
#50576=CARTESIAN_POINT('Origin',(-66.,0.,0.));
#50577=CARTESIAN_POINT('',(-66.,-6.93800739067722,-12.2318420402206));
#50578=CARTESIAN_POINT('Ctrl Pts',(-66.,-7.57407686781798,-14.5180571909737));
#50579=CARTESIAN_POINT('Ctrl Pts',(-66.,-7.57386669307527,-14.5079003575064));
#50580=CARTESIAN_POINT('Ctrl Pts',(-66.,-7.57315469596912,-14.4762403397886));
#50581=CARTESIAN_POINT('Ctrl Pts',(-66.,-7.57166007128053,-14.4231630709543));
#50582=CARTESIAN_POINT('Ctrl Pts',(-66.,-7.56883349438523,-14.3488435570404));
#50583=CARTESIAN_POINT('Ctrl Pts',(-66.,-7.56381234400904,-14.2535736549186));
#50584=CARTESIAN_POINT('Ctrl Pts',(-66.,-7.556353222684,-14.1476860346413));
#50585=CARTESIAN_POINT('Ctrl Pts',(-66.,-7.54703967094767,-14.0424458557121));
#50586=CARTESIAN_POINT('Ctrl Pts',(-66.,-7.53595904837785,-13.9378208062029));
#50587=CARTESIAN_POINT('Ctrl Pts',(-66.,-7.52324912730704,-13.8337539100138));
#50588=CARTESIAN_POINT('Ctrl Pts',(-66.,-7.50902360355704,-13.730201376709));
#50589=CARTESIAN_POINT('Ctrl Pts',(-66.,-7.49330244824787,-13.6271680529626));
#50590=CARTESIAN_POINT('Ctrl Pts',(-66.,-7.47595026385202,-13.5247388655977));
#50591=CARTESIAN_POINT('Ctrl Pts',(-66.,-7.45658443707985,-13.4231254995838));
#50592=CARTESIAN_POINT('Ctrl Pts',(-66.,-7.43465467928082,-13.32262679532));
#50593=CARTESIAN_POINT('Ctrl Pts',(-66.,-7.40958054758866,-13.2235599331263));
#50594=CARTESIAN_POINT('Ctrl Pts',(-66.,-7.38087472971119,-13.1261989021839));
#50595=CARTESIAN_POINT('Ctrl Pts',(-66.,-7.34826186125705,-13.0307150430677));
#50596=CARTESIAN_POINT('Ctrl Pts',(-66.,-7.31182932887926,-12.9371020273035));
#50597=CARTESIAN_POINT('Ctrl Pts',(-66.,-7.27195707536722,-12.8452087977179));
#50598=CARTESIAN_POINT('Ctrl Pts',(-66.,-7.22919071332107,-12.7548002330908));
#50599=CARTESIAN_POINT('Ctrl Pts',(-66.,-7.18413356438513,-12.6656085000656));
#50600=CARTESIAN_POINT('Ctrl Pts',(-66.,-7.13733570230759,-12.5773859525787));
#50601=CARTESIAN_POINT('Ctrl Pts',(-66.,-7.08917363628753,-12.4899622973194));
#50602=CARTESIAN_POINT('Ctrl Pts',(-66.,-7.03987370169386,-12.4032345978205));
#50603=CARTESIAN_POINT('Ctrl Pts',(-66.,-6.99961691350077,-12.3343662552827));
#50604=CARTESIAN_POINT('Ctrl Pts',(-66.,-6.96898338507103,-12.2829952952022));
#50605=CARTESIAN_POINT('Ctrl Pts',(-66.,-6.94836533853418,-12.24887239112));
#50606=CARTESIAN_POINT('Ctrl Pts',(-66.,-6.93800739067721,-12.2318420402206));
#50607=CARTESIAN_POINT('',(-66.,-8.11364170780698,-11.4857618157149));
#50608=CARTESIAN_POINT('Origin',(-66.,0.,0.));
#50609=CARTESIAN_POINT('',(-66.,-9.90065997719615,-13.0429121370937));
#50610=CARTESIAN_POINT('Ctrl Pts',(-66.,-8.11364170780698,-11.4857618157149));
#50611=CARTESIAN_POINT('Ctrl Pts',(-66.,-8.12633089210227,-11.5053893225758));
#50612=CARTESIAN_POINT('Ctrl Pts',(-66.,-8.15190308143842,-11.5445298762901));
#50613=CARTESIAN_POINT('Ctrl Pts',(-66.,-8.19084282166638,-11.6028973387695));
#50614=CARTESIAN_POINT('Ctrl Pts',(-66.,-8.24392698602517,-11.6800328696824));
#50615=CARTESIAN_POINT('Ctrl Pts',(-66.,-8.3122597763829,-11.775262383207));
#50616=CARTESIAN_POINT('Ctrl Pts',(-66.,-8.3826658022629,-11.8691782078618));
#50617=CARTESIAN_POINT('Ctrl Pts',(-66.,-8.45532310380908,-11.9615427552514));
#50618=CARTESIAN_POINT('Ctrl Pts',(-66.,-8.53052243279731,-12.0519568423361));
#50619=CARTESIAN_POINT('Ctrl Pts',(-66.,-8.60865015717173,-12.1399248062686));
#50620=CARTESIAN_POINT('Ctrl Pts',(-66.,-8.69016937887314,-12.2249411582788));
#50621=CARTESIAN_POINT('Ctrl Pts',(-66.,-8.77558942093922,-12.3065676074844));
#50622=CARTESIAN_POINT('Ctrl Pts',(-66.,-8.86547091932666,-12.3845199371372));
#50623=CARTESIAN_POINT('Ctrl Pts',(-66.,-8.96023870955522,-12.4587311071067));
#50624=CARTESIAN_POINT('Ctrl Pts',(-66.,-9.05985628822634,-12.5294228183105));
#50625=CARTESIAN_POINT('Ctrl Pts',(-66.,-9.16361561347667,-12.5971460670373));
#50626=CARTESIAN_POINT('Ctrl Pts',(-66.,-9.26970137008846,-12.6629072844668));
#50627=CARTESIAN_POINT('Ctrl Pts',(-66.,-9.37550212434126,-12.7279933116739));
#50628=CARTESIAN_POINT('Ctrl Pts',(-66.,-9.47889915384706,-12.7933918468958));
#50629=CARTESIAN_POINT('Ctrl Pts',(-66.,-9.57920178477654,-12.8593645469766));
#50630=CARTESIAN_POINT('Ctrl Pts',(-66.,-9.67846562159703,-12.9248440002217));
#50631=CARTESIAN_POINT('Ctrl Pts',(-66.,-9.76163392180467,-12.9749764383087));
#50632=CARTESIAN_POINT('Ctrl Pts',(-66.,-9.82856614146686,-13.0099860215666));
#50633=CARTESIAN_POINT('Ctrl Pts',(-66.,-9.87577567632734,-13.031989851782));
#50634=CARTESIAN_POINT('Ctrl Pts',(-66.,-9.9002308011995,-13.0427239576368));
#50635=CARTESIAN_POINT('Ctrl Pts',(-66.,-9.90065997719615,-13.0429121370937));
#50636=CARTESIAN_POINT('',(-66.,-10.9466173199386,-12.178349405844));
#50637=CARTESIAN_POINT('Origin',(-66.,0.,0.));
#50638=CARTESIAN_POINT('',(-66.,-9.76197254719673,-10.1221439546065));
#50639=CARTESIAN_POINT('Ctrl Pts',(-66.,-10.9466173199386,-12.178349405844));
#50640=CARTESIAN_POINT('Ctrl Pts',(-66.,-10.9438878464529,-12.1685639363102));
#50641=CARTESIAN_POINT('Ctrl Pts',(-66.,-10.9353246918112,-12.1380756427477));
#50642=CARTESIAN_POINT('Ctrl Pts',(-66.,-10.9206772435082,-12.0870375919612));
#50643=CARTESIAN_POINT('Ctrl Pts',(-66.,-10.8994569571944,-12.0157559033301));
#50644=CARTESIAN_POINT('Ctrl Pts',(-66.,-10.8709008942817,-11.9247277896931));
#50645=CARTESIAN_POINT('Ctrl Pts',(-66.,-10.8373429346305,-11.8240218317612));
#50646=CARTESIAN_POINT('Ctrl Pts',(-66.,-10.8021498170253,-11.7244041527066));
#50647=CARTESIAN_POINT('Ctrl Pts',(-66.,-10.7653981208323,-11.6258217302963));
#50648=CARTESIAN_POINT('Ctrl Pts',(-66.,-10.727207120633,-11.5281851158537));
#50649=CARTESIAN_POINT('Ctrl Pts',(-66.,-10.6876760500473,-11.4314236196986));
#50650=CARTESIAN_POINT('Ctrl Pts',(-66.,-10.6468254580846,-11.3355369696227));
#50651=CARTESIAN_POINT('Ctrl Pts',(-66.,-10.6045453214218,-11.2406410963124));
#50652=CARTESIAN_POINT('Ctrl Pts',(-66.,-10.5605176911805,-11.1470361863206));
#50653=CARTESIAN_POINT('Ctrl Pts',(-66.,-10.5142838856252,-11.055148542648));
#50654=CARTESIAN_POINT('Ctrl Pts',(-66.,-10.4653605771075,-10.9654297310826));
#50655=CARTESIAN_POINT('Ctrl Pts',(-66.,-10.4133439014856,-10.8782663225706));
#50656=CARTESIAN_POINT('Ctrl Pts',(-66.,-10.3580097561152,-10.7938927550471));
#50657=CARTESIAN_POINT('Ctrl Pts',(-66.,-10.2994412084092,-10.7122811666816));
#50658=CARTESIAN_POINT('Ctrl Pts',(-66.,-10.2379686981643,-10.6331907581101));
#50659=CARTESIAN_POINT('Ctrl Pts',(-66.,-10.1740622242879,-10.5562581065423));
#50660=CARTESIAN_POINT('Ctrl Pts',(-66.,-10.108239546518,-10.4810737531071));
#50661=CARTESIAN_POINT('Ctrl Pts',(-66.,-10.0409718699529,-10.4072610342189));
#50662=CARTESIAN_POINT('Ctrl Pts',(-66.,-9.97258152483879,-10.3345613726147));
#50663=CARTESIAN_POINT('Ctrl Pts',(-66.,-9.90326213654415,-10.2628187784479));
#50664=CARTESIAN_POINT('Ctrl Pts',(-66.,-9.84714322904426,-10.2061255176443));
#50665=CARTESIAN_POINT('Ctrl Pts',(-66.,-9.80469667097528,-10.163986719468));
#50666=CARTESIAN_POINT('Ctrl Pts',(-66.,-9.77624035711837,-10.1360633488319));
#50667=CARTESIAN_POINT('Ctrl Pts',(-66.,-9.76197254719672,-10.1221439546065));
#50668=CARTESIAN_POINT('',(-66.,-10.7151295435653,-9.10713484662511));
#50669=CARTESIAN_POINT('Origin',(-66.,0.,0.));
#50670=CARTESIAN_POINT('',(-66.,-12.8332528856473,-10.1709510554827));
#50671=CARTESIAN_POINT('Ctrl Pts',(-66.,-10.7151295435653,-9.10713484662511));
#50672=CARTESIAN_POINT('Ctrl Pts',(-66.,-10.7323012362688,-9.12299004745485));
#50673=CARTESIAN_POINT('Ctrl Pts',(-66.,-10.7668038881397,-9.15454138381928));
#50674=CARTESIAN_POINT('Ctrl Pts',(-66.,-10.8190356624814,-9.20139120553108));
#50675=CARTESIAN_POINT('Ctrl Pts',(-66.,-10.889634916681,-9.26290188705335));
#50676=CARTESIAN_POINT('Ctrl Pts',(-66.,-10.9795035237476,-9.33814591637203));
#50677=CARTESIAN_POINT('Ctrl Pts',(-66.,-11.0710535306934,-9.4116019360644));
#50678=CARTESIAN_POINT('Ctrl Pts',(-66.,-11.1643982983724,-9.48299554522798));
#50679=CARTESIAN_POINT('Ctrl Pts',(-66.,-11.2597201712738,-9.55186779486609));
#50680=CARTESIAN_POINT('Ctrl Pts',(-66.,-11.3572701125446,-9.61764250849074));
#50681=CARTESIAN_POINT('Ctrl Pts',(-66.,-11.4573709649815,-9.6797149094218));
#50682=CARTESIAN_POINT('Ctrl Pts',(-66.,-11.5604070517922,-9.73753381300202));
#50683=CARTESIAN_POINT('Ctrl Pts',(-66.,-11.6668507136929,-9.79068450718227));
#50684=CARTESIAN_POINT('Ctrl Pts',(-66.,-11.7770967670118,-9.83899640572359));
#50685=CARTESIAN_POINT('Ctrl Pts',(-66.,-11.8911649899478,-9.88269332242761));
#50686=CARTESIAN_POINT('Ctrl Pts',(-66.,-12.0085066122796,-9.9224850258725));
#50687=CARTESIAN_POINT('Ctrl Pts',(-66.,-12.1276136395118,-9.95979777888845));
#50688=CARTESIAN_POINT('Ctrl Pts',(-66.,-12.2462767052779,-9.99652743122885));
#50689=CARTESIAN_POINT('Ctrl Pts',(-66.,-12.362689281313,-10.0341575556064));
#50690=CARTESIAN_POINT('Ctrl Pts',(-66.,-12.4762474639872,-10.0731133520306));
#50691=CARTESIAN_POINT('Ctrl Pts',(-66.,-12.5886768226797,-10.1118497354652));
#50692=CARTESIAN_POINT('Ctrl Pts',(-66.,-12.6816996681717,-10.1397240556283));
#50693=CARTESIAN_POINT('Ctrl Pts',(-66.,-12.7552356183835,-10.1569883822946));
#50694=CARTESIAN_POINT('Ctrl Pts',(-66.,-12.8064341089476,-10.166560387824));
#50695=CARTESIAN_POINT('Ctrl Pts',(-66.,-12.8327903946759,-10.1708755197597));
#50696=CARTESIAN_POINT('Ctrl Pts',(-66.,-12.8332528856473,-10.1709510554827));
#50697=CARTESIAN_POINT('',(-66.,-13.631341547005,-9.07343113870903));
#50698=CARTESIAN_POINT('Origin',(-66.,0.,0.));
#50699=CARTESIAN_POINT('',(-66.,-11.9725570665522,-7.37643433768308));
#50700=CARTESIAN_POINT('Ctrl Pts',(-66.,-13.631341547005,-9.07343113870903));
#50701=CARTESIAN_POINT('Ctrl Pts',(-66.,-13.6262642776339,-9.06463189014802));
#50702=CARTESIAN_POINT('Ctrl Pts',(-66.,-13.6103880199559,-9.03723101235338));
#50703=CARTESIAN_POINT('Ctrl Pts',(-66.,-13.5835081010849,-8.99143908805054));
#50704=CARTESIAN_POINT('Ctrl Pts',(-66.,-13.5452274539844,-8.92767411535463));
#50705=CARTESIAN_POINT('Ctrl Pts',(-66.,-13.4949307609898,-8.84660742136017));
#50706=CARTESIAN_POINT('Ctrl Pts',(-66.,-13.4373825330349,-8.7574108514811));
#50707=CARTESIAN_POINT('Ctrl Pts',(-66.,-13.3785211625712,-8.66967501744431));
#50708=CARTESIAN_POINT('Ctrl Pts',(-66.,-13.3184076369901,-8.58332951829382));
#50709=CARTESIAN_POINT('Ctrl Pts',(-66.,-13.2571352386615,-8.49825805316535));
#50710=CARTESIAN_POINT('Ctrl Pts',(-66.,-13.1947825037901,-8.41436747482742));
#50711=CARTESIAN_POINT('Ctrl Pts',(-66.,-13.1313692681049,-8.3316524092927));
#50712=CARTESIAN_POINT('Ctrl Pts',(-66.,-13.0668177956572,-8.25025250675973));
#50713=CARTESIAN_POINT('Ctrl Pts',(-66.,-13.0008947798771,-8.17053759353955));
#50714=CARTESIAN_POINT('Ctrl Pts',(-66.,-12.9332619666045,-8.09303464904925));
#50715=CARTESIAN_POINT('Ctrl Pts',(-66.,-12.8635635126628,-8.01830125100551));
#50716=CARTESIAN_POINT('Ctrl Pts',(-66.,-12.7915043783298,-7.9468122624453));
#50717=CARTESIAN_POINT('Ctrl Pts',(-66.,-12.7169258039014,-7.87885048806616));
#50718=CARTESIAN_POINT('Ctrl Pts',(-66.,-12.6399013181197,-7.81436828334278));
#50719=CARTESIAN_POINT('Ctrl Pts',(-66.,-12.5606910950408,-7.75305023703025));
#50720=CARTESIAN_POINT('Ctrl Pts',(-66.,-12.4796599881192,-7.69442745995809));
#50721=CARTESIAN_POINT('Ctrl Pts',(-66.,-12.3972076624386,-7.63797459554787));
#50722=CARTESIAN_POINT('Ctrl Pts',(-66.,-12.3136968468978,-7.58320962985052));
#50723=CARTESIAN_POINT('Ctrl Pts',(-66.,-12.2293754395952,-7.5298019490105));
#50724=CARTESIAN_POINT('Ctrl Pts',(-66.,-12.144392189705,-7.47755231121817));
#50725=CARTESIAN_POINT('Ctrl Pts',(-66.,-12.0759373202474,-7.43659637822836));
#50726=CARTESIAN_POINT('Ctrl Pts',(-66.,-12.0243448058902,-7.40633747762124));
#50727=CARTESIAN_POINT('Ctrl Pts',(-66.,-11.9898382395678,-7.38636816850343));
#50728=CARTESIAN_POINT('Ctrl Pts',(-66.,-11.9725570665522,-7.37643433768309));
#50729=CARTESIAN_POINT('',(-66.,-12.6433463826116,-6.1562731014228));
#50730=CARTESIAN_POINT('Origin',(-66.,0.,0.));
#50731=CARTESIAN_POINT('',(-66.,-14.9594853178907,-6.65991171291435));
#50732=CARTESIAN_POINT('Ctrl Pts',(-66.,-12.6433463826116,-6.1562731014228));
#50733=CARTESIAN_POINT('Ctrl Pts',(-66.,-12.6639216231176,-6.16735975564195));
#50734=CARTESIAN_POINT('Ctrl Pts',(-66.,-12.7051868090144,-6.18933938815496));
#50735=CARTESIAN_POINT('Ctrl Pts',(-66.,-12.7674287029928,-6.22172782249946));
#50736=CARTESIAN_POINT('Ctrl Pts',(-66.,-12.851107036246,-6.26374871229064));
#50737=CARTESIAN_POINT('Ctrl Pts',(-66.,-12.9568646849259,-6.31427939831312));
#50738=CARTESIAN_POINT('Ctrl Pts',(-66.,-13.0638062493037,-6.3626601011734));
#50739=CARTESIAN_POINT('Ctrl Pts',(-66.,-13.1719732880642,-6.40859684907992));
#50740=CARTESIAN_POINT('Ctrl Pts',(-66.,-13.281428281035,-6.45159976453225));
#50741=CARTESIAN_POINT('Ctrl Pts',(-66.,-13.3922710176287,-6.49104836068956));
#50742=CARTESIAN_POINT('Ctrl Pts',(-66.,-13.5046637960973,-6.52627657330457));
#50743=CARTESIAN_POINT('Ctrl Pts',(-66.,-13.6188417913781,-6.55665495690443));
#50744=CARTESIAN_POINT('Ctrl Pts',(-66.,-13.7351593700424,-6.58166436202222));
#50745=CARTESIAN_POINT('Ctrl Pts',(-66.,-13.8539565214648,-6.60104137487127));
#50746=CARTESIAN_POINT('Ctrl Pts',(-66.,-13.9753080627051,-6.61499785909296));
#50747=CARTESIAN_POINT('Ctrl Pts',(-66.,-14.0988589764351,-6.62435775818486));
#50748=CARTESIAN_POINT('Ctrl Pts',(-66.,-14.2235033417215,-6.63087754928856));
#50749=CARTESIAN_POINT('Ctrl Pts',(-66.,-14.3475726821666,-6.63694296762358));
#50750=CARTESIAN_POINT('Ctrl Pts',(-66.,-14.4696861744433,-6.64444024204806));
#50751=CARTESIAN_POINT('Ctrl Pts',(-66.,-14.5893646306071,-6.65393139885702));
#50752=CARTESIAN_POINT('Ctrl Pts',(-66.,-14.7078951610787,-6.6634907630476));
#50753=CARTESIAN_POINT('Ctrl Pts',(-66.,-14.8049275843586,-6.66735551923628));
#50754=CARTESIAN_POINT('Ctrl Pts',(-66.,-14.880446730922,-6.66578980817273));
#50755=CARTESIAN_POINT('Ctrl Pts',(-66.,-14.9324171877326,-6.66232854470537));
#50756=CARTESIAN_POINT('Ctrl Pts',(-66.,-14.9590185719531,-6.65995356711245));
#50757=CARTESIAN_POINT('Ctrl Pts',(-66.,-14.9594853178907,-6.65991171291435));
#50758=CARTESIAN_POINT('',(-66.,-15.4595584521058,-5.39839582338346));
#50759=CARTESIAN_POINT('Origin',(-66.,0.,0.));
#50760=CARTESIAN_POINT('',(-66.,-13.4308617934315,-4.16723622269519));
#50761=CARTESIAN_POINT('Ctrl Pts',(-66.,-15.4595584521058,-5.39839582338346));
#50762=CARTESIAN_POINT('Ctrl Pts',(-66.,-15.4524524103566,-5.3911356849437));
#50763=CARTESIAN_POINT('Ctrl Pts',(-66.,-15.430260613301,-5.36854392084221));
#50764=CARTESIAN_POINT('Ctrl Pts',(-66.,-15.3928371880222,-5.33087539803783));
#50765=CARTESIAN_POINT('Ctrl Pts',(-66.,-15.3399014939787,-5.27863372902275));
#50766=CARTESIAN_POINT('Ctrl Pts',(-66.,-15.2710244971014,-5.21262217319695));
#50767=CARTESIAN_POINT('Ctrl Pts',(-66.,-15.1931019676527,-5.14053953989829));
#50768=CARTESIAN_POINT('Ctrl Pts',(-66.,-15.1142708207137,-5.07019831600168));
#50769=CARTESIAN_POINT('Ctrl Pts',(-66.,-15.0345726196388,-5.00151514537911));
#50770=CARTESIAN_POINT('Ctrl Pts',(-66.,-14.954068793312,-4.9343541825898));
#50771=CARTESIAN_POINT('Ctrl Pts',(-66.,-14.8728122458042,-4.86860567563393));
#50772=CARTESIAN_POINT('Ctrl Pts',(-66.,-14.7908208532122,-4.80425948641264));
#50773=CARTESIAN_POINT('Ctrl Pts',(-66.,-14.7080540513971,-4.74147020990105));
#50774=CARTESIAN_POINT('Ctrl Pts',(-66.,-14.6243778356077,-4.68065407462106));
#50775=CARTESIAN_POINT('Ctrl Pts',(-66.,-14.5395956330118,-4.62240562435127));
#50776=CARTESIAN_POINT('Ctrl Pts',(-66.,-14.4535014438403,-4.56735341407851));
#50777=CARTESIAN_POINT('Ctrl Pts',(-66.,-14.3659275912213,-4.51603076153944));
#50778=CARTESIAN_POINT('Ctrl Pts',(-66.,-14.2767906338471,-4.4687510685349));
#50779=CARTESIAN_POINT('Ctrl Pts',(-66.,-14.1861499417075,-4.42544990152536));
#50780=CARTESIAN_POINT('Ctrl Pts',(-66.,-14.0941790754254,-4.38575705583354));
#50781=CARTESIAN_POINT('Ctrl Pts',(-66.,-14.0011148179182,-4.34912763794002));
#50782=CARTESIAN_POINT('Ctrl Pts',(-66.,-13.9072136271877,-4.31495340364481));
#50783=CARTESIAN_POINT('Ctrl Pts',(-66.,-13.8127069643429,-4.28267727534445));
#50784=CARTESIAN_POINT('Ctrl Pts',(-66.,-13.717752718985,-4.25191737627554));
#50785=CARTESIAN_POINT('Ctrl Pts',(-66.,-13.6224454176364,-4.22244373176092));
#50786=CARTESIAN_POINT('Ctrl Pts',(-66.,-13.5459558574286,-4.19979853847996));
#50787=CARTESIAN_POINT('Ctrl Pts',(-66.,-13.4884591342042,-4.1833208134517));
#50788=CARTESIAN_POINT('Ctrl Pts',(-66.,-13.4500704898848,-4.17256031098595));
#50789=CARTESIAN_POINT('Ctrl Pts',(-66.,-13.4308617934315,-4.1672362226952));
#50790=CARTESIAN_POINT('',(-66.,-13.7771352694631,-2.8185900760694));
#50791=CARTESIAN_POINT('Origin',(-66.,0.,0.));
#50792=CARTESIAN_POINT('',(-66.,-16.1457582704724,-2.73040562398164));
#50793=CARTESIAN_POINT('Ctrl Pts',(-66.,-13.7771352694631,-2.8185900760694));
#50794=CARTESIAN_POINT('Ctrl Pts',(-66.,-13.7998212397401,-2.82421156841951));
#50795=CARTESIAN_POINT('Ctrl Pts',(-66.,-13.8452561162702,-2.83523843593487));
#50796=CARTESIAN_POINT('Ctrl Pts',(-66.,-13.913597242777,-2.85113039846586));
#50797=CARTESIAN_POINT('Ctrl Pts',(-66.,-14.0050968376581,-2.87102116947837));
#50798=CARTESIAN_POINT('Ctrl Pts',(-66.,-14.1200983859353,-2.89366348336299));
#50799=CARTESIAN_POINT('Ctrl Pts',(-66.,-14.2357119759516,-2.91392893189869));
#50800=CARTESIAN_POINT('Ctrl Pts',(-66.,-14.3519047529378,-2.93152244373364));
#50801=CARTESIAN_POINT('Ctrl Pts',(-66.,-14.4686154062224,-2.94595399366867));
#50802=CARTESIAN_POINT('Ctrl Pts',(-66.,-14.5857862813476,-2.95659777198027));
#50803=CARTESIAN_POINT('Ctrl Pts',(-66.,-14.703408934225,-2.96276827812033));
#50804=CARTESIAN_POINT('Ctrl Pts',(-66.,-14.8215546146151,-2.96379735617437));
#50805=CARTESIAN_POINT('Ctrl Pts',(-66.,-14.9404374487894,-2.959094039328));
#50806=CARTESIAN_POINT('Ctrl Pts',(-66.,-15.0603212363863,-2.9483186375038));
#50807=CARTESIAN_POINT('Ctrl Pts',(-66.,-15.181331132295,-2.93165775201116));
#50808=CARTESIAN_POINT('Ctrl Pts',(-66.,-15.3033281791249,-2.90999772986683));
#50809=CARTESIAN_POINT('Ctrl Pts',(-66.,-15.4256780185848,-2.88531489660512));
#50810=CARTESIAN_POINT('Ctrl Pts',(-66.,-15.5473579007536,-2.86033496839371));
#50811=CARTESIAN_POINT('Ctrl Pts',(-66.,-15.6674994694501,-2.83722831154002));
#50812=CARTESIAN_POINT('Ctrl Pts',(-66.,-15.7857783615561,-2.81665846444538));
#50813=CARTESIAN_POINT('Ctrl Pts',(-66.,-15.9029623546524,-2.7964401593829));
#50814=CARTESIAN_POINT('Ctrl Pts',(-66.,-15.9979074517054,-2.77605251475231));
#50815=CARTESIAN_POINT('Ctrl Pts',(-66.,-16.0706646489018,-2.75575514534332));
#50816=CARTESIAN_POINT('Ctrl Pts',(-66.,-16.1201415770235,-2.73947809679247));
#50817=CARTESIAN_POINT('Ctrl Pts',(-66.,-16.1453165969326,-2.73056223824769));
#50818=CARTESIAN_POINT('Ctrl Pts',(-66.,-16.1457582704724,-2.73040562398164));
#50819=CARTESIAN_POINT('',(-66.,-16.3163944433819,-1.38415944456368));
#50820=CARTESIAN_POINT('Origin',(-66.,0.,0.));
#50821=CARTESIAN_POINT('',(-66.,-14.045256078575,-0.696195329812616));
#50822=CARTESIAN_POINT('Ctrl Pts',(-66.,-16.3163944433819,-1.38415944456368));
#50823=CARTESIAN_POINT('Ctrl Pts',(-66.,-16.307706127992,-1.37889459744425));
#50824=CARTESIAN_POINT('Ctrl Pts',(-66.,-16.2805931837835,-1.36253147066111));
#50825=CARTESIAN_POINT('Ctrl Pts',(-66.,-16.2349777035408,-1.33535320117812));
#50826=CARTESIAN_POINT('Ctrl Pts',(-66.,-16.170713106895,-1.29791737203952));
#50827=CARTESIAN_POINT('Ctrl Pts',(-66.,-16.0875836011606,-1.25110870320843));
#50828=CARTESIAN_POINT('Ctrl Pts',(-66.,-15.9941829293225,-1.20066922344171));
#50829=CARTESIAN_POINT('Ctrl Pts',(-66.,-15.900335256791,-1.15214240747963));
#50830=CARTESIAN_POINT('Ctrl Pts',(-66.,-15.8060601113054,-1.10543718159424));
#50831=CARTESIAN_POINT('Ctrl Pts',(-66.,-15.7113832084608,-1.06040669143688));
#50832=CARTESIAN_POINT('Ctrl Pts',(-66.,-15.6163284960372,-1.01693147636119));
#50833=CARTESIAN_POINT('Ctrl Pts',(-66.,-15.5209107672782,-0.974997271170846));
#50834=CARTESIAN_POINT('Ctrl Pts',(-66.,-15.4251291786488,-0.934763901846662));
#50835=CARTESIAN_POINT('Ctrl Pts',(-66.,-15.3289574472276,-0.89666784595261));
#50836=CARTESIAN_POINT('Ctrl Pts',(-66.,-15.2323530329047,-0.861333854256595));
#50837=CARTESIAN_POINT('Ctrl Pts',(-66.,-15.1352727230412,-0.829421964594113));
#50838=CARTESIAN_POINT('Ctrl Pts',(-66.,-15.0376867393704,-0.801490439086723));
#50839=CARTESIAN_POINT('Ctrl Pts',(-66.,-14.939592201905,-0.777863584450799));
#50840=CARTESIAN_POINT('Ctrl Pts',(-66.,-14.8410305914479,-0.758464226728878));
#50841=CARTESIAN_POINT('Ctrl Pts',(-66.,-14.7420779497362,-0.742890629132665));
#50842=CARTESIAN_POINT('Ctrl Pts',(-66.,-14.6428281112089,-0.730556131457601));
#50843=CARTESIAN_POINT('Ctrl Pts',(-66.,-14.5433782125866,-0.72080782010221));
#50844=CARTESIAN_POINT('Ctrl Pts',(-66.,-14.4438139036356,-0.71304855704325));
#50845=CARTESIAN_POINT('Ctrl Pts',(-66.,-14.3441931446757,-0.706869197330954));
#50846=CARTESIAN_POINT('Ctrl Pts',(-66.,-14.2445503001281,-0.702023483575367));
#50847=CARTESIAN_POINT('Ctrl Pts',(-66.,-14.1648321695468,-0.699111910780302));
#50848=CARTESIAN_POINT('Ctrl Pts',(-66.,-14.1050439680336,-0.697450717395246));
#50849=CARTESIAN_POINT('Ctrl Pts',(-66.,-14.0651853454231,-0.696575143525857));
#50850=CARTESIAN_POINT('Ctrl Pts',(-66.,-14.045256078575,-0.696195329812629));
#50851=CARTESIAN_POINT('',(-66.,-14.045256078575,0.696195329812624));
#50852=CARTESIAN_POINT('Origin',(-66.,0.,0.));
#50853=CARTESIAN_POINT('',(-66.,-16.3175338509752,1.37066189203528));
#50854=CARTESIAN_POINT('Ctrl Pts',(-66.,-14.045256078575,0.696195329812624));
#50855=CARTESIAN_POINT('Ctrl Pts',(-66.,-14.0686273356774,0.696392218370307));
#50856=CARTESIAN_POINT('Ctrl Pts',(-66.,-14.1153770624506,0.697010974492569));
#50857=CARTESIAN_POINT('Ctrl Pts',(-66.,-14.1855232971663,0.698614034227448));
#50858=CARTESIAN_POINT('Ctrl Pts',(-66.,-14.279094897617,0.702103192289484));
#50859=CARTESIAN_POINT('Ctrl Pts',(-66.,-14.3961143752671,0.708771950396692));
#50860=CARTESIAN_POINT('Ctrl Pts',(-66.,-14.5131355638642,0.717895108848178));
#50861=CARTESIAN_POINT('Ctrl Pts',(-66.,-14.6300532595709,0.7297502981378));
#50862=CARTESIAN_POINT('Ctrl Pts',(-66.,-14.7466862135917,0.744796901078022));
#50863=CARTESIAN_POINT('Ctrl Pts',(-66.,-14.8628229502399,0.763626728348506));
#50864=CARTESIAN_POINT('Ctrl Pts',(-66.,-14.97828481366,0.786901644277719));
#50865=CARTESIAN_POINT('Ctrl Pts',(-66.,-15.0929746515511,0.81528653252832));
#50866=CARTESIAN_POINT('Ctrl Pts',(-66.,-15.2069528955437,0.849407044643804));
#50867=CARTESIAN_POINT('Ctrl Pts',(-66.,-15.3203905800386,0.889657803015486));
#50868=CARTESIAN_POINT('Ctrl Pts',(-66.,-15.4334553338124,0.935889193512498));
#50869=CARTESIAN_POINT('Ctrl Pts',(-66.,-15.5462329906162,0.987208158041752));
#50870=CARTESIAN_POINT('Ctrl Pts',(-66.,-15.6586006138651,1.04154270247793));
#50871=CARTESIAN_POINT('Ctrl Pts',(-66.,-15.7702454432537,1.09599839647648));
#50872=CARTESIAN_POINT('Ctrl Pts',(-66.,-15.8808661517589,1.14825710837788));
#50873=CARTESIAN_POINT('Ctrl Pts',(-66.,-15.9903135820168,1.19759548023257));
#50874=CARTESIAN_POINT('Ctrl Pts',(-66.,-16.0987879364791,1.2463210640833));
#50875=CARTESIAN_POINT('Ctrl Pts',(-66.,-16.1856799576735,1.28968007884051));
#50876=CARTESIAN_POINT('Ctrl Pts',(-66.,-16.2511036032208,1.32743374822648));
#50877=CARTESIAN_POINT('Ctrl Pts',(-66.,-16.2949781852964,1.35550383503756));
#50878=CARTESIAN_POINT('Ctrl Pts',(-66.,-16.317145001806,1.37040035835162));
#50879=CARTESIAN_POINT('Ctrl Pts',(-66.,-16.3175338509752,1.37066189203528));
#50880=CARTESIAN_POINT('',(-66.,-16.1480113642792,2.71704876274038));
#50881=CARTESIAN_POINT('Origin',(-66.,0.,0.));
#50882=CARTESIAN_POINT('',(-66.,-13.7771352694631,2.8185900760694));
#50883=CARTESIAN_POINT('Ctrl Pts',(-66.,-16.1480113642792,2.71704876274038));
#50884=CARTESIAN_POINT('Ctrl Pts',(-66.,-16.1382866940579,2.7199875088322));
#50885=CARTESIAN_POINT('Ctrl Pts',(-66.,-16.1079562086956,2.72909384286184));
#50886=CARTESIAN_POINT('Ctrl Pts',(-66.,-16.0570148618746,2.74407414839715));
#50887=CARTESIAN_POINT('Ctrl Pts',(-66.,-15.9854593435823,2.76435190683515));
#50888=CARTESIAN_POINT('Ctrl Pts',(-66.,-15.8933006615651,2.78901652785862));
#50889=CARTESIAN_POINT('Ctrl Pts',(-66.,-15.7902905550528,2.81464355607623));
#50890=CARTESIAN_POINT('Ctrl Pts',(-66.,-15.6873231513416,2.83830684578773));
#50891=CARTESIAN_POINT('Ctrl Pts',(-66.,-15.5843947155558,2.86009946582377));
#50892=CARTESIAN_POINT('Ctrl Pts',(-66.,-15.4814936341966,2.88017005204204));
#50893=CARTESIAN_POINT('Ctrl Pts',(-66.,-15.3786133940255,2.89864026758367));
#50894=CARTESIAN_POINT('Ctrl Pts',(-66.,-15.2757647759192,2.91552760840775));
#50895=CARTESIAN_POINT('Ctrl Pts',(-66.,-15.1729867099492,2.9306770599819));
#50896=CARTESIAN_POINT('Ctrl Pts',(-66.,-15.0703622864763,2.94365932119071));
#50897=CARTESIAN_POINT('Ctrl Pts',(-66.,-14.9680056710645,2.95385868966535));
#50898=CARTESIAN_POINT('Ctrl Pts',(-66.,-14.8660391534142,2.96062511732634));
#50899=CARTESIAN_POINT('Ctrl Pts',(-66.,-14.7645727249416,2.96341047532946));
#50900=CARTESIAN_POINT('Ctrl Pts',(-66.,-14.6636842479405,2.96189992942649));
#50901=CARTESIAN_POINT('Ctrl Pts',(-66.,-14.5633947076351,2.95617854486928));
#50902=CARTESIAN_POINT('Ctrl Pts',(-66.,-14.463677848895,2.94665434795724));
#50903=CARTESIAN_POINT('Ctrl Pts',(-66.,-14.3644786617177,2.93391890356181));
#50904=CARTESIAN_POINT('Ctrl Pts',(-66.,-14.2657288580852,2.91862876972314));
#50905=CARTESIAN_POINT('Ctrl Pts',(-66.,-14.1673628947312,2.90138362450613));
#50906=CARTESIAN_POINT('Ctrl Pts',(-66.,-14.0693351608341,2.882594172965));
#50907=CARTESIAN_POINT('Ctrl Pts',(-66.,-13.9716176994713,2.862507481945));
#50908=CARTESIAN_POINT('Ctrl Pts',(-66.,-13.8936799818437,2.84550248942744));
#50909=CARTESIAN_POINT('Ctrl Pts',(-66.,-13.8353570146283,2.83224277227946));
#50910=CARTESIAN_POINT('Ctrl Pts',(-66.,-13.7965328775753,2.82317840202614));
#50911=CARTESIAN_POINT('Ctrl Pts',(-66.,-13.7771352694631,2.81859007606939));
#50912=CARTESIAN_POINT('',(-66.,-13.4308617934315,4.1672362226952));
#50913=CARTESIAN_POINT('Origin',(-66.,0.,0.));
#50914=CARTESIAN_POINT('',(-66.,-15.4640187679296,5.38560568043381));
#50915=CARTESIAN_POINT('Ctrl Pts',(-66.,-13.4308617934315,4.1672362226952));
#50916=CARTESIAN_POINT('Ctrl Pts',(-66.,-13.4534498353221,4.1732391209285));
#50917=CARTESIAN_POINT('Ctrl Pts',(-66.,-13.4985769550718,4.18546462196559));
#50918=CARTESIAN_POINT('Ctrl Pts',(-66.,-13.5661207520894,4.20446197782756));
#50919=CARTESIAN_POINT('Ctrl Pts',(-66.,-13.655884910321,4.23111182833087));
#50920=CARTESIAN_POINT('Ctrl Pts',(-66.,-13.7675695531958,4.26667263583206));
#50921=CARTESIAN_POINT('Ctrl Pts',(-66.,-13.8786454687203,4.30461115967259));
#50922=CARTESIAN_POINT('Ctrl Pts',(-66.,-13.988941714333,4.34517014494338));
#50923=CARTESIAN_POINT('Ctrl Pts',(-66.,-14.0981684916428,4.38874946735859));
#50924=CARTESIAN_POINT('Ctrl Pts',(-66.,-14.2059737915295,4.4358697529125));
#50925=CARTESIAN_POINT('Ctrl Pts',(-66.,-14.3120199719745,4.48712764234399));
#50926=CARTESIAN_POINT('Ctrl Pts',(-66.,-14.4160475830522,4.54314296997813));
#50927=CARTESIAN_POINT('Ctrl Pts',(-66.,-14.5179595646104,4.60453676010005));
#50928=CARTESIAN_POINT('Ctrl Pts',(-66.,-14.6178234390918,4.67173377183878));
#50929=CARTESIAN_POINT('Ctrl Pts',(-66.,-14.7158387764281,4.74463077904808));
#50930=CARTESIAN_POINT('Ctrl Pts',(-66.,-14.8123108082616,4.82238412668293));
#50931=CARTESIAN_POINT('Ctrl Pts',(-66.,-14.9076357442716,4.90295634303817));
#50932=CARTESIAN_POINT('Ctrl Pts',(-66.,-15.0022304656484,4.98346615129592));
#50933=CARTESIAN_POINT('Ctrl Pts',(-66.,-15.0963796080126,5.06159331118216));
#50934=CARTESIAN_POINT('Ctrl Pts',(-66.,-15.1901185918597,5.13660009643943));
#50935=CARTESIAN_POINT('Ctrl Pts',(-66.,-15.2830674650563,5.2107713514449));
#50936=CARTESIAN_POINT('Ctrl Pts',(-66.,-15.3564466651341,5.27437732996824));
#50937=CARTESIAN_POINT('Ctrl Pts',(-66.,-15.4104259507712,5.32721509743538));
#50938=CARTESIAN_POINT('Ctrl Pts',(-66.,-15.4459413854495,5.3653144757178));
#50939=CARTESIAN_POINT('Ctrl Pts',(-66.,-15.4637071759544,5.38525566045572));
#50940=CARTESIAN_POINT('Ctrl Pts',(-66.,-15.4640187679296,5.38560568043381));
#50941=CARTESIAN_POINT('',(-66.,-14.9649893429273,6.64753480367511));
#50942=CARTESIAN_POINT('Origin',(-66.,0.,0.));
#50943=CARTESIAN_POINT('',(-66.,-12.6433463826116,6.15627310142281));
#50944=CARTESIAN_POINT('Ctrl Pts',(-66.,-14.9649893429273,6.64753480367511));
#50945=CARTESIAN_POINT('Ctrl Pts',(-66.,-14.9548393546694,6.64796279651443));
#50946=CARTESIAN_POINT('Ctrl Pts',(-66.,-14.9231971040963,6.64924015333274));
#50947=CARTESIAN_POINT('Ctrl Pts',(-66.,-14.870130722867,6.65108122722986));
#50948=CARTESIAN_POINT('Ctrl Pts',(-66.,-14.7957803793054,6.65292678882822));
#50949=CARTESIAN_POINT('Ctrl Pts',(-66.,-14.7003831899324,6.65389759319505));
#50950=CARTESIAN_POINT('Ctrl Pts',(-66.,-14.5942361525827,6.65310192943101));
#50951=CARTESIAN_POINT('Ctrl Pts',(-66.,-14.4886188383546,6.65041484137187));
#50952=CARTESIAN_POINT('Ctrl Pts',(-66.,-14.3835044844334,6.64592554509403));
#50953=CARTESIAN_POINT('Ctrl Pts',(-66.,-14.278844877945,6.63977511862666));
#50954=CARTESIAN_POINT('Ctrl Pts',(-66.,-14.1746034538834,6.63207978306306));
#50955=CARTESIAN_POINT('Ctrl Pts',(-66.,-14.0707863033563,6.6228591657896));
#50956=CARTESIAN_POINT('Ctrl Pts',(-66.,-13.9674696839217,6.61197280385553));
#50957=CARTESIAN_POINT('Ctrl Pts',(-66.,-13.8648408383502,6.59902554716193));
#50958=CARTESIAN_POINT('Ctrl Pts',(-66.,-13.7631634644371,6.58344942858329));
#50959=CARTESIAN_POINT('Ctrl Pts',(-66.,-13.6627176703106,6.56464523470766));
#50960=CARTESIAN_POINT('Ctrl Pts',(-66.,-13.5637463059047,6.54210941091933));
#50961=CARTESIAN_POINT('Ctrl Pts',(-66.,-13.4664030834197,6.51555637763196));
#50962=CARTESIAN_POINT('Ctrl Pts',(-66.,-13.3706871739224,6.48507374642914));
#50963=CARTESIAN_POINT('Ctrl Pts',(-66.,-13.2764716751216,6.45105019532836));
#50964=CARTESIAN_POINT('Ctrl Pts',(-66.,-13.1835561890537,6.41404502367149));
#50965=CARTESIAN_POINT('Ctrl Pts',(-66.,-13.0917112937495,6.37467717998103));
#50966=CARTESIAN_POINT('Ctrl Pts',(-66.,-13.0007243712348,6.33351120238525));
#50967=CARTESIAN_POINT('Ctrl Pts',(-66.,-12.9104491054422,6.29093354993378));
#50968=CARTESIAN_POINT('Ctrl Pts',(-66.,-12.8207969747412,6.24717657480866));
#50969=CARTESIAN_POINT('Ctrl Pts',(-66.,-12.7495367835008,6.21132350319834));
#50970=CARTESIAN_POINT('Ctrl Pts',(-66.,-12.6963436971102,6.18397603231157));
#50971=CARTESIAN_POINT('Ctrl Pts',(-66.,-12.6609935089309,6.16554126565498));
#50972=CARTESIAN_POINT('Ctrl Pts',(-66.,-12.6433463826116,6.1562731014228));
#50973=CARTESIAN_POINT('',(-66.,-11.9725570665522,7.37643433768309));
#50974=CARTESIAN_POINT('Origin',(-66.,0.,0.));
#50975=CARTESIAN_POINT('',(-66.,-13.6388425130122,9.0621520570585));
#50976=CARTESIAN_POINT('Ctrl Pts',(-66.,-11.9725570665522,7.37643433768309));
#50977=CARTESIAN_POINT('Ctrl Pts',(-66.,-11.9929426034861,7.38786606141889));
#50978=CARTESIAN_POINT('Ctrl Pts',(-66.,-12.0336116133124,7.4109301341784));
#50979=CARTESIAN_POINT('Ctrl Pts',(-66.,-12.0943089474566,7.44612811243127));
#50980=CARTESIAN_POINT('Ctrl Pts',(-66.,-12.174625451278,7.49426414725743));
#50981=CARTESIAN_POINT('Ctrl Pts',(-66.,-12.2739577025182,7.5564825878338));
#50982=CARTESIAN_POINT('Ctrl Pts',(-66.,-12.3721090366891,7.62085266008235));
#50983=CARTESIAN_POINT('Ctrl Pts',(-66.,-12.4688535134548,7.68756697112423));
#50984=CARTESIAN_POINT('Ctrl Pts',(-66.,-12.5638109939272,7.75694076391353));
#50985=CARTESIAN_POINT('Ctrl Pts',(-66.,-12.6565110535803,7.82939076691323));
#50986=CARTESIAN_POINT('Ctrl Pts',(-66.,-12.7464782795223,7.9054109081407));
#50987=CARTESIAN_POINT('Ctrl Pts',(-66.,-12.8333072263957,7.98553702611316));
#50988=CARTESIAN_POINT('Ctrl Pts',(-66.,-12.9167494409123,8.07034649661759));
#50989=CARTESIAN_POINT('Ctrl Pts',(-66.,-12.9967646908729,8.16026752634251));
#50990=CARTESIAN_POINT('Ctrl Pts',(-66.,-13.0735719476516,8.2552497632047));
#50991=CARTESIAN_POINT('Ctrl Pts',(-66.,-13.1476766619554,8.35455196515643));
#50992=CARTESIAN_POINT('Ctrl Pts',(-66.,-13.2199692944164,8.45629920475326));
#50993=CARTESIAN_POINT('Ctrl Pts',(-66.,-13.2915701735423,8.557804399923));
#50994=CARTESIAN_POINT('Ctrl Pts',(-66.,-13.3633320128944,8.65689099100683));
#50995=CARTESIAN_POINT('Ctrl Pts',(-66.,-13.4354725852278,8.7528532374933));
#50996=CARTESIAN_POINT('Ctrl Pts',(-66.,-13.5070556576137,8.84780971091874));
#50997=CARTESIAN_POINT('Ctrl Pts',(-66.,-13.5623113515642,8.92766605565115));
#50998=CARTESIAN_POINT('Ctrl Pts',(-66.,-13.6014545602526,8.99226792994578));
#50999=CARTESIAN_POINT('Ctrl Pts',(-66.,-13.626379282156,9.03800267564234));
#51000=CARTESIAN_POINT('Ctrl Pts',(-66.,-13.6386277567007,9.0617355438285));
#51001=CARTESIAN_POINT('Ctrl Pts',(-66.,-13.6388425130122,9.0621520570585));
#51002=CARTESIAN_POINT('',(-66.,-12.8416620037784,10.1603317849721));
#51003=CARTESIAN_POINT('Origin',(-66.,0.,0.));
#51004=CARTESIAN_POINT('',(-66.,-10.7151295435653,9.10713484662512));
#51005=CARTESIAN_POINT('Ctrl Pts',(-66.,-12.8416620037784,10.1603317849721));
#51006=CARTESIAN_POINT('Ctrl Pts',(-66.,-12.8317244585753,10.1582221321948));
#51007=CARTESIAN_POINT('Ctrl Pts',(-66.,-12.8007586417669,10.151590250775));
#51008=CARTESIAN_POINT('Ctrl Pts',(-66.,-12.7489015820264,10.14017641159));
#51009=CARTESIAN_POINT('Ctrl Pts',(-66.,-12.6764281187229,10.123473812926));
#51010=CARTESIAN_POINT('Ctrl Pts',(-66.,-12.5837865782488,10.1006898014275));
#51011=CARTESIAN_POINT('Ctrl Pts',(-66.,-12.4811722187999,10.0735214401623));
#51012=CARTESIAN_POINT('Ctrl Pts',(-66.,-12.3795413183411,10.0446528139577));
#51013=CARTESIAN_POINT('Ctrl Pts',(-66.,-12.2788457677249,10.0141636803616));
#51014=CARTESIAN_POINT('Ctrl Pts',(-66.,-12.179003784094,9.98217869512325));
#51015=CARTESIAN_POINT('Ctrl Pts',(-66.,-12.079951048189,9.94880133468933));
#51016=CARTESIAN_POINT('Ctrl Pts',(-66.,-11.9816885786214,9.91405212461268));
#51017=CARTESIAN_POINT('Ctrl Pts',(-66.,-11.8843251688933,9.87781397932795));
#51018=CARTESIAN_POINT('Ctrl Pts',(-66.,-11.7881404490329,9.83975072848667));
#51019=CARTESIAN_POINT('Ctrl Pts',(-66.,-11.6935310799647,9.79937782767));
#51020=CARTESIAN_POINT('Ctrl Pts',(-66.,-11.6009173880207,9.75618454891596));
#51021=CARTESIAN_POINT('Ctrl Pts',(-66.,-11.5106598224983,9.70974355202577));
#51022=CARTESIAN_POINT('Ctrl Pts',(-66.,-11.4229782872014,9.65981645609066));
#51023=CARTESIAN_POINT('Ctrl Pts',(-66.,-11.3378501911246,9.60648791406797));
#51024=CARTESIAN_POINT('Ctrl Pts',(-66.,-11.255055958553,9.55010283362399));
#51025=CARTESIAN_POINT('Ctrl Pts',(-66.,-11.1742623953034,9.49115310573639));
#51026=CARTESIAN_POINT('Ctrl Pts',(-66.,-11.0950933608815,9.43018117859799));
#51027=CARTESIAN_POINT('Ctrl Pts',(-66.,-11.0172025221741,9.36768097839366));
#51028=CARTESIAN_POINT('Ctrl Pts',(-66.,-10.9403520514449,9.30399043552504));
#51029=CARTESIAN_POINT('Ctrl Pts',(-66.,-10.8643984244951,9.23931258796881));
#51030=CARTESIAN_POINT('Ctrl Pts',(-66.,-10.8042932995341,9.18686421761339));
#51031=CARTESIAN_POINT('Ctrl Pts',(-66.,-10.7595724112169,9.14714733516059));
#51032=CARTESIAN_POINT('Ctrl Pts',(-66.,-10.7299173542433,9.1205004962881));
#51033=CARTESIAN_POINT('Ctrl Pts',(-66.,-10.7151295435653,9.10713484662511));
#51034=CARTESIAN_POINT('',(-66.,-9.76197254719673,10.1221439546065));
#51035=CARTESIAN_POINT('Origin',(-66.,0.,0.));
#51036=CARTESIAN_POINT('',(-66.,-10.9566876228483,12.1692900916743));
#51037=CARTESIAN_POINT('Ctrl Pts',(-66.,-9.76197254719673,10.1221439546065));
#51038=CARTESIAN_POINT('Ctrl Pts',(-66.,-9.77887468091545,10.1382862065996));
#51039=CARTESIAN_POINT('Ctrl Pts',(-66.,-9.8125301973609,10.1707396505663));
#51040=CARTESIAN_POINT('Ctrl Pts',(-66.,-9.86256723189823,10.2199266327873));
#51041=CARTESIAN_POINT('Ctrl Pts',(-66.,-9.92838949999087,10.2865242878363));
#51042=CARTESIAN_POINT('Ctrl Pts',(-66.,-10.0091279489326,10.371490948043));
#51043=CARTESIAN_POINT('Ctrl Pts',(-66.,-10.0881874924486,10.4582479603236));
#51044=CARTESIAN_POINT('Ctrl Pts',(-66.,-10.1653013890907,10.5469256916157));
#51045=CARTESIAN_POINT('Ctrl Pts',(-66.,-10.2400230449985,10.6377349442392));
#51046=CARTESIAN_POINT('Ctrl Pts',(-66.,-10.3117931787431,10.7309623645438));
#51047=CARTESIAN_POINT('Ctrl Pts',(-66.,-10.3800284784999,10.8269681325114));
#51048=CARTESIAN_POINT('Ctrl Pts',(-66.,-10.4442029791024,10.9261704221467));
#51049=CARTESIAN_POINT('Ctrl Pts',(-66.,-10.5039324453602,11.0290666820944));
#51050=CARTESIAN_POINT('Ctrl Pts',(-66.,-10.5590714183695,11.1360616608015));
#51051=CARTESIAN_POINT('Ctrl Pts',(-66.,-10.6098445121699,11.2471610440543));
#51052=CARTESIAN_POINT('Ctrl Pts',(-66.,-10.6569256372063,11.3617725777663));
#51053=CARTESIAN_POINT('Ctrl Pts',(-66.,-10.7016435541469,11.4783016873407));
#51054=CARTESIAN_POINT('Ctrl Pts',(-66.,-10.7457516444569,11.5944243246999));
#51055=CARTESIAN_POINT('Ctrl Pts',(-66.,-10.7906171205087,11.7082443720486));
#51056=CARTESIAN_POINT('Ctrl Pts',(-66.,-10.8366264238543,11.819132418893));
#51057=CARTESIAN_POINT('Ctrl Pts',(-66.,-10.8823458677273,11.9289076462876));
#51058=CARTESIAN_POINT('Ctrl Pts',(-66.,-10.9160061370834,12.0199966893985));
#51059=CARTESIAN_POINT('Ctrl Pts',(-66.,-10.9378537570625,12.0923034971696));
#51060=CARTESIAN_POINT('Ctrl Pts',(-66.,-10.9506216542472,12.1427999280076));
#51061=CARTESIAN_POINT('Ctrl Pts',(-66.,-10.9565831961294,12.1688332562504));
#51062=CARTESIAN_POINT('Ctrl Pts',(-66.,-10.9566876228483,12.1692900916743));
#51063=CARTESIAN_POINT('',(-66.,-9.91144581260293,13.0347177531328));
#51064=CARTESIAN_POINT('Origin',(-66.,0.,0.));
#51065=CARTESIAN_POINT('',(-66.,-8.11364170780697,11.4857618157149));
#51066=CARTESIAN_POINT('Ctrl Pts',(-66.,-9.91144581260293,13.0347177531328));
#51067=CARTESIAN_POINT('Ctrl Pts',(-66.,-9.90234512296736,13.0302030119816));
#51068=CARTESIAN_POINT('Ctrl Pts',(-66.,-9.87400143607814,13.0160785978238));
#51069=CARTESIAN_POINT('Ctrl Pts',(-66.,-9.82661206760692,12.9921270190498));
#51070=CARTESIAN_POINT('Ctrl Pts',(-66.,-9.76056925879954,12.9579257458254));
#51071=CARTESIAN_POINT('Ctrl Pts',(-66.,-9.67650437592402,12.9128185216976));
#51072=CARTESIAN_POINT('Ctrl Pts',(-66.,-9.58387033196931,12.8609845509879));
#51073=CARTESIAN_POINT('Ctrl Pts',(-66.,-9.49261168852801,12.8077483085937));
#51074=CARTESIAN_POINT('Ctrl Pts',(-66.,-9.40266201299437,12.7531750820743));
#51075=CARTESIAN_POINT('Ctrl Pts',(-66.,-9.31391109124575,12.69736527232));
#51076=CARTESIAN_POINT('Ctrl Pts',(-66.,-9.22627089118454,12.6404031093252));
#51077=CARTESIAN_POINT('Ctrl Pts',(-66.,-9.13973729492348,12.5823087271131));
#51078=CARTESIAN_POINT('Ctrl Pts',(-66.,-9.05444479601274,12.5229957744206));
#51079=CARTESIAN_POINT('Ctrl Pts',(-66.,-8.9707478415549,12.4622081834688));
#51080=CARTESIAN_POINT('Ctrl Pts',(-66.,-8.88915113193907,12.3995752782536));
#51081=CARTESIAN_POINT('Ctrl Pts',(-66.,-8.81018880105177,12.334706907179));
#51082=CARTESIAN_POINT('Ctrl Pts',(-66.,-8.73431624919877,12.2672787958196));
#51083=CARTESIAN_POINT('Ctrl Pts',(-66.,-8.66180575442286,12.1971147402934));
#51084=CARTESIAN_POINT('Ctrl Pts',(-66.,-8.59261438312223,12.1242911158748));
#51085=CARTESIAN_POINT('Ctrl Pts',(-66.,-8.52644368290816,12.0490873880617));
#51086=CARTESIAN_POINT('Ctrl Pts',(-66.,-8.46284859919381,11.9718971321485));
#51087=CARTESIAN_POINT('Ctrl Pts',(-66.,-8.40132990725019,11.8931522119833));
#51088=CARTESIAN_POINT('Ctrl Pts',(-66.,-8.34142932020866,11.8132449066089));
#51089=CARTESIAN_POINT('Ctrl Pts',(-66.,-8.28283244225497,11.732443384369));
#51090=CARTESIAN_POINT('Ctrl Pts',(-66.,-8.22534976477564,11.6509086114121));
#51091=CARTESIAN_POINT('Ctrl Pts',(-66.,-8.18017633214654,11.5851604663126));
#51092=CARTESIAN_POINT('Ctrl Pts',(-66.,-8.14673761978747,11.5355697300868));
#51093=CARTESIAN_POINT('Ctrl Pts',(-66.,-8.12464103031309,11.502385137885));
#51094=CARTESIAN_POINT('Ctrl Pts',(-66.,-8.11364170780698,11.4857618157149));
#51095=CARTESIAN_POINT('',(-66.,-6.93800739067721,12.2318420402206));
#51096=CARTESIAN_POINT('Origin',(-66.,0.,0.));
#51097=CARTESIAN_POINT('',(-66.,-7.58608375346252,14.5117868743119));
#51098=CARTESIAN_POINT('Ctrl Pts',(-66.,-6.93800739067721,12.2318420402206));
#51099=CARTESIAN_POINT('Ctrl Pts',(-66.,-6.95036409795758,12.2516805434111));
#51100=CARTESIAN_POINT('Ctrl Pts',(-66.,-6.97489142114752,12.2914841893452));
#51101=CARTESIAN_POINT('Ctrl Pts',(-66.,-7.01112414517467,12.3515695765444));
#51102=CARTESIAN_POINT('Ctrl Pts',(-66.,-7.05831632235693,12.4324442762203));
#51103=CARTESIAN_POINT('Ctrl Pts',(-66.,-7.11538787531798,12.5348203883111));
#51104=CARTESIAN_POINT('Ctrl Pts',(-66.,-7.17038802629925,12.6385130784722));
#51105=CARTESIAN_POINT('Ctrl Pts',(-66.,-7.22302599308674,12.7435822820237));
#51106=CARTESIAN_POINT('Ctrl Pts',(-66.,-7.27281678798223,12.8501211151659));
#51107=CARTESIAN_POINT('Ctrl Pts',(-66.,-7.31914741436296,12.9582681310911));
#51108=CARTESIAN_POINT('Ctrl Pts',(-66.,-7.36136331309888,13.0682271303129));
#51109=CARTESIAN_POINT('Ctrl Pts',(-66.,-7.39885104754049,13.1802723469128));
#51110=CARTESIAN_POINT('Ctrl Pts',(-66.,-7.43111474350486,13.2947900458654));
#51111=CARTESIAN_POINT('Ctrl Pts',(-66.,-7.45791285510172,13.4121360855424));
#51112=CARTESIAN_POINT('Ctrl Pts',(-66.,-7.47946152571002,13.5323718323411));
#51113=CARTESIAN_POINT('Ctrl Pts',(-66.,-7.49656078124055,13.6550912336386));
#51114=CARTESIAN_POINT('Ctrl Pts',(-66.,-7.51089419147856,13.7790802606718));
#51115=CARTESIAN_POINT('Ctrl Pts',(-66.,-7.52473801944021,13.9025239278461));
#51116=CARTESIAN_POINT('Ctrl Pts',(-66.,-7.53988806932779,14.0239256992838));
#51117=CARTESIAN_POINT('Ctrl Pts',(-66.,-7.55687516994583,14.1427720426853));
#51118=CARTESIAN_POINT('Ctrl Pts',(-66.,-7.5738582645032,14.2604684427868));
#51119=CARTESIAN_POINT('Ctrl Pts',(-66.,-7.5838081107473,14.3570667246954));
#51120=CARTESIAN_POINT('Ctrl Pts',(-66.,-7.58698737570401,14.4325351632849));
#51121=CARTESIAN_POINT('Ctrl Pts',(-66.,-7.58679619423276,14.4846204028018));
#51122=CARTESIAN_POINT('Ctrl Pts',(-66.,-7.58609621785102,14.511318421344));
#51123=CARTESIAN_POINT('Ctrl Pts',(-66.,-7.58608375346252,14.5117868743119));
#51124=CARTESIAN_POINT('',(-66.,-6.35845702927376,15.0900844665257));
#51125=CARTESIAN_POINT('Origin',(-66.,0.,0.));
#51126=CARTESIAN_POINT('',(-66.,-5.00234392366024,13.1426961282463));
#51127=CARTESIAN_POINT('Ctrl Pts',(-66.,-6.35845702927376,15.0900844665257));
#51128=CARTESIAN_POINT('Ctrl Pts',(-66.,-6.35076502500556,15.0834483147912));
#51129=CARTESIAN_POINT('Ctrl Pts',(-66.,-6.32682440612351,15.0627188567828));
#51130=CARTESIAN_POINT('Ctrl Pts',(-66.,-6.2868803772285,15.027734504202));
#51131=CARTESIAN_POINT('Ctrl Pts',(-66.,-6.23141793548312,14.9781835481972));
#51132=CARTESIAN_POINT('Ctrl Pts',(-66.,-6.16121181596629,14.913587364225));
#51133=CARTESIAN_POINT('Ctrl Pts',(-66.,-6.08437862517161,14.8403447030824));
#51134=CARTESIAN_POINT('Ctrl Pts',(-66.,-6.00922635494104,14.7660858733973));
#51135=CARTESIAN_POINT('Ctrl Pts',(-66.,-5.93567442341548,14.6908575904833));
#51136=CARTESIAN_POINT('Ctrl Pts',(-66.,-5.86359111036561,14.614729691814));
#51137=CARTESIAN_POINT('Ctrl Pts',(-66.,-5.79287020223623,14.5377618684515));
#51138=CARTESIAN_POINT('Ctrl Pts',(-66.,-5.72350270338309,14.4599725977946));
#51139=CARTESIAN_POINT('Ctrl Pts',(-66.,-5.6556403566801,14.3813116886496));
#51140=CARTESIAN_POINT('Ctrl Pts',(-66.,-5.5896901550893,14.301619265488));
#51141=CARTESIAN_POINT('Ctrl Pts',(-66.,-5.52623312628269,14.2206618116565));
#51142=CARTESIAN_POINT('Ctrl Pts',(-66.,-5.46588365010489,14.1381942665852));
#51143=CARTESIAN_POINT('Ctrl Pts',(-66.,-5.40916346339393,14.0540157969766));
#51144=CARTESIAN_POINT('Ctrl Pts',(-66.,-5.35638011020072,13.9680234475133));
#51145=CARTESIAN_POINT('Ctrl Pts',(-66.,-5.30747301200313,13.8802805168475));
#51146=CARTESIAN_POINT('Ctrl Pts',(-66.,-5.2620835925999,13.7909834684638));
#51147=CARTESIAN_POINT('Ctrl Pts',(-66.,-5.21968290141691,13.7004028321899));
#51148=CARTESIAN_POINT('Ctrl Pts',(-66.,-5.17967999761633,13.6088327519355));
#51149=CARTESIAN_POINT('Ctrl Pts',(-66.,-5.14153343642338,13.5165392112663));
#51150=CARTESIAN_POINT('Ctrl Pts',(-66.,-5.10487200859133,13.4237037664646));
#51151=CARTESIAN_POINT('Ctrl Pts',(-66.,-5.06947212861492,13.3304351977558));
#51152=CARTESIAN_POINT('Ctrl Pts',(-66.,-5.04206880122609,13.2555184756737));
#51153=CARTESIAN_POINT('Ctrl Pts',(-66.,-5.02201334210169,13.1991698540138));
#51154=CARTESIAN_POINT('Ctrl Pts',(-66.,-5.00886363010872,13.1615326184551));
#51155=CARTESIAN_POINT('Ctrl Pts',(-66.,-5.00234392366025,13.1426961282463));
#51156=CARTESIAN_POINT('',(-66.,-3.67810171359515,13.5729685048794));
#51157=CARTESIAN_POINT('Origin',(-66.,0.,0.));
#51158=CARTESIAN_POINT('',(-66.,-3.73881834218222,15.9424547170178));
#51159=CARTESIAN_POINT('Ctrl Pts',(-66.,-3.67810171359515,13.5729685048794));
#51160=CARTESIAN_POINT('Ctrl Pts',(-66.,-3.68513657707394,13.595256733151));
#51161=CARTESIAN_POINT('Ctrl Pts',(-66.,-3.69899456508718,13.6399095715909));
#51162=CARTESIAN_POINT('Ctrl Pts',(-66.,-3.71914634329887,13.7071179779119));
#51163=CARTESIAN_POINT('Ctrl Pts',(-66.,-3.7447431715177,13.7971880673979));
#51164=CARTESIAN_POINT('Ctrl Pts',(-66.,-3.77456181293102,13.910540963737));
#51165=CARTESIAN_POINT('Ctrl Pts',(-66.,-3.80204670961501,14.0246539387008));
#51166=CARTESIAN_POINT('Ctrl Pts',(-66.,-3.82690130950572,14.1395127300348));
#51167=CARTESIAN_POINT('Ctrl Pts',(-66.,-3.84863270462788,14.2550869169872));
#51168=CARTESIAN_POINT('Ctrl Pts',(-66.,-3.86661269999714,14.3713582537855));
#51169=CARTESIAN_POINT('Ctrl Pts',(-66.,-3.88015661753544,14.4883613559395));
#51170=CARTESIAN_POINT('Ctrl Pts',(-66.,-3.88860209359085,14.6062092864715));
#51171=CARTESIAN_POINT('Ctrl Pts',(-66.,-3.89137277258683,14.725152856237));
#51172=CARTESIAN_POINT('Ctrl Pts',(-66.,-3.88814619886307,14.8454766736426));
#51173=CARTESIAN_POINT('Ctrl Pts',(-66.,-3.87911646405442,14.9672939298197));
#51174=CARTESIAN_POINT('Ctrl Pts',(-66.,-3.86515944096752,15.0904102873887));
#51175=CARTESIAN_POINT('Ctrl Pts',(-66.,-3.84820772362302,15.2140685453126));
#51176=CARTESIAN_POINT('Ctrl Pts',(-66.,-3.83091743061146,15.3370768226993));
#51177=CARTESIAN_POINT('Ctrl Pts',(-66.,-3.81540012098238,15.4584321984421));
#51178=CARTESIAN_POINT('Ctrl Pts',(-66.,-3.80229765686693,15.5777692855585));
#51179=CARTESIAN_POINT('Ctrl Pts',(-66.,-3.7894772918181,15.6959915606914));
#51180=CARTESIAN_POINT('Ctrl Pts',(-66.,-3.77509152951778,15.7920294560818));
#51181=CARTESIAN_POINT('Ctrl Pts',(-66.,-3.75940267454228,15.8659175659396));
#51182=CARTESIAN_POINT('Ctrl Pts',(-66.,-3.74626442705009,15.9163189069806));
#51183=CARTESIAN_POINT('Ctrl Pts',(-66.,-3.73894691449476,15.9420040811287));
#51184=CARTESIAN_POINT('Ctrl Pts',(-66.,-3.73881834218222,15.9424547170178));
#51185=CARTESIAN_POINT('',(-66.,-2.40594300602614,16.1972856754382));
#51186=CARTESIAN_POINT('Origin',(-66.,0.,0.));
#51187=CARTESIAN_POINT('',(-66.,-1.57673047345589,13.9738265075847));
#51188=CARTESIAN_POINT('Ctrl Pts',(-66.,-2.40594300602614,16.1972856754382));
#51189=CARTESIAN_POINT('Ctrl Pts',(-66.,-2.40014300404269,16.1889450869399));
#51190=CARTESIAN_POINT('Ctrl Pts',(-66.,-2.38210973029964,16.1629130931652));
#51191=CARTESIAN_POINT('Ctrl Pts',(-66.,-2.35212087122016,16.1190941623136));
#51192=CARTESIAN_POINT('Ctrl Pts',(-66.,-2.31072370572823,16.0573069923301));
#51193=CARTESIAN_POINT('Ctrl Pts',(-66.,-2.25878765825938,15.9772806643205));
#51194=CARTESIAN_POINT('Ctrl Pts',(-66.,-2.20258303257508,15.8872314185123));
#51195=CARTESIAN_POINT('Ctrl Pts',(-66.,-2.14825922908453,15.7966159569104));
#51196=CARTESIAN_POINT('Ctrl Pts',(-66.,-2.09572657992989,15.7054594872874));
#51197=CARTESIAN_POINT('Ctrl Pts',(-66.,-2.04484013524158,15.6137968955554));
#51198=CARTESIAN_POINT('Ctrl Pts',(-66.,-1.99548217379509,15.5216595832348));
#51199=CARTESIAN_POINT('Ctrl Pts',(-66.,-1.94763938741864,15.4290632100973));
#51200=CARTESIAN_POINT('Ctrl Pts',(-66.,-1.901471233747,15.3359968987161));
#51201=CARTESIAN_POINT('Ctrl Pts',(-66.,-1.85741167873706,15.2424070113801));
#51202=CARTESIAN_POINT('Ctrl Pts',(-66.,-1.81608156923822,15.1482118634974));
#51203=CARTESIAN_POINT('Ctrl Pts',(-66.,-1.77813692730802,15.0533268835806));
#51204=CARTESIAN_POINT('Ctrl Pts',(-66.,-1.74413304367239,14.957687298555));
#51205=CARTESIAN_POINT('Ctrl Pts',(-66.,-1.71439340426661,14.8612698707291));
#51206=CARTESIAN_POINT('Ctrl Pts',(-66.,-1.68884359201954,14.7641208448459));
#51207=CARTESIAN_POINT('Ctrl Pts',(-66.,-1.66708743757887,14.6663413378531));
#51208=CARTESIAN_POINT('Ctrl Pts',(-66.,-1.64854533029309,14.5680618357278));
#51209=CARTESIAN_POINT('Ctrl Pts',(-66.,-1.63257174420173,14.4694202802978));
#51210=CARTESIAN_POINT('Ctrl Pts',(-66.,-1.61857609759037,14.3705396469258));
#51211=CARTESIAN_POINT('Ctrl Pts',(-66.,-1.60615369222193,14.2715034719842));
#51212=CARTESIAN_POINT('Ctrl Pts',(-66.,-1.59506091439902,14.1723615147133));
#51213=CARTESIAN_POINT('Ctrl Pts',(-66.,-1.58714954409268,14.0929835088213));
#51214=CARTESIAN_POINT('Ctrl Pts',(-66.,-1.58173749645856,14.0334175928621));
#51215=CARTESIAN_POINT('Ctrl Pts',(-66.,-1.57836090671277,13.9936925998767));
#51216=CARTESIAN_POINT('Ctrl Pts',(-66.,-1.57673047345591,13.9738265075847));
#51217=CARTESIAN_POINT('',(-66.,-0.187087378736033,14.0612554404903));
#51218=CARTESIAN_POINT('Origin',(-66.,0.,0.));
#51219=CARTESIAN_POINT('',(-66.,0.343370775949386,16.3713994976063));
#51220=CARTESIAN_POINT('Ctrl Pts',(-66.,-0.187087378736033,14.0612554404903));
#51221=CARTESIAN_POINT('Ctrl Pts',(-66.,-0.188358372068459,14.0845929424903));
#51222=CARTESIAN_POINT('Ctrl Pts',(-66.,-0.190676276552008,14.1312892713751));
#51223=CARTESIAN_POINT('Ctrl Pts',(-66.,-0.193480898610155,14.2013977454735));
#51224=CARTESIAN_POINT('Ctrl Pts',(-66.,-0.195874035010017,14.2950037897925));
#51225=CARTESIAN_POINT('Ctrl Pts',(-66.,-0.196566149970303,14.4122110910203));
#51226=CARTESIAN_POINT('Ctrl Pts',(-66.,-0.194808815215985,14.5295742128916));
#51227=CARTESIAN_POINT('Ctrl Pts',(-66.,-0.190318342289957,14.6470055917277));
#51228=CARTESIAN_POINT('Ctrl Pts',(-66.,-0.182624874160768,14.7643531812717));
#51229=CARTESIAN_POINT('Ctrl Pts',(-66.,-0.171124489283723,14.8814430832361));
#51230=CARTESIAN_POINT('Ctrl Pts',(-66.,-0.155145411474415,14.9981385531066));
#51231=CARTESIAN_POINT('Ctrl Pts',(-66.,-0.13401796882278,15.1143843786811));
#51232=CARTESIAN_POINT('Ctrl Pts',(-66.,-0.107121538899203,15.2302801573274));
#51233=CARTESIAN_POINT('Ctrl Pts',(-66.,-0.0740730173483893,15.3460213644938));
#51234=CARTESIAN_POINT('Ctrl Pts',(-66.,-0.035032248569878,15.4617659038311));
#51235=CARTESIAN_POINT('Ctrl Pts',(-66.,0.00910408204356977,15.5775433641354));
#51236=CARTESIAN_POINT('Ctrl Pts',(-66.,0.0562757882257695,15.6931009498213));
#51237=CARTESIAN_POINT('Ctrl Pts',(-66.,0.103613789511375,15.8079447749594));
#51238=CARTESIAN_POINT('Ctrl Pts',(-66.,0.148823449024451,15.9216285504355));
#51239=CARTESIAN_POINT('Ctrl Pts',(-66.,0.191192201865526,16.0339579931922));
#51240=CARTESIAN_POINT('Ctrl Pts',(-66.,0.233010475834533,16.1452778030188));
#51241=CARTESIAN_POINT('Ctrl Pts',(-66.,0.270827936326797,16.2347208977209));
#51242=CARTESIAN_POINT('Ctrl Pts',(-66.,0.304399122776818,16.3023860171632));
#51243=CARTESIAN_POINT('Ctrl Pts',(-66.,0.329658911880923,16.3479365581074));
#51244=CARTESIAN_POINT('Ctrl Pts',(-66.,0.343134174384058,16.3709949939062));
#51245=CARTESIAN_POINT('Ctrl Pts',(-66.,0.343370775949386,16.3713994976063));
#51246=CARTESIAN_POINT('',(-66.,1.69774526472951,16.2867518559131));
#51247=CARTESIAN_POINT('Origin',(-66.,0.,0.));
#51248=CARTESIAN_POINT('',(-66.,1.94795475120473,13.9269299753125));
#51249=CARTESIAN_POINT('Ctrl Pts',(-66.,1.69774526472951,16.2867518559131));
#51250=CARTESIAN_POINT('Ctrl Pts',(-66.,1.70128882897267,16.277230900501));
#51251=CARTESIAN_POINT('Ctrl Pts',(-66.,1.71228166066573,16.2475320568679));
#51252=CARTESIAN_POINT('Ctrl Pts',(-66.,1.73043103962239,16.1976318523256));
#51253=CARTESIAN_POINT('Ctrl Pts',(-66.,1.75516179270489,16.1274907834907));
#51254=CARTESIAN_POINT('Ctrl Pts',(-66.,1.78556443525587,16.0370626599488));
#51255=CARTESIAN_POINT('Ctrl Pts',(-66.,1.8176089524919,15.9358649547671));
#51256=CARTESIAN_POINT('Ctrl Pts',(-66.,1.84769092488014,15.8345865639611));
#51257=CARTESIAN_POINT('Ctrl Pts',(-66.,1.87590347211591,15.7332296038656));
#51258=CARTESIAN_POINT('Ctrl Pts',(-66.,1.90239566597564,15.6317918168208));
#51259=CARTESIAN_POINT('Ctrl Pts',(-66.,1.92728933849566,15.5302743417326));
#51260=CARTESIAN_POINT('Ctrl Pts',(-66.,1.95060127417394,15.4286890367845));
#51261=CARTESIAN_POINT('Ctrl Pts',(-66.,1.97217431992445,15.3270650217851));
#51262=CARTESIAN_POINT('Ctrl Pts',(-66.,1.99157480447254,15.2254582670956));
#51263=CARTESIAN_POINT('Ctrl Pts',(-66.,2.00818107188229,15.1239440527286));
#51264=CARTESIAN_POINT('Ctrl Pts',(-66.,2.02133667816179,15.022603610217));
#51265=CARTESIAN_POINT('Ctrl Pts',(-66.,2.03048766965571,14.9215122966393));
#51266=CARTESIAN_POINT('Ctrl Pts',(-66.,2.03531494435546,14.8207280520398));
#51267=CARTESIAN_POINT('Ctrl Pts',(-66.,2.03590208198289,14.7202771615244));
#51268=CARTESIAN_POINT('Ctrl Pts',(-66.,2.03265795226397,14.6201590419547));
#51269=CARTESIAN_POINT('Ctrl Pts',(-66.,2.02617640685866,14.5203559365434));
#51270=CARTESIAN_POINT('Ctrl Pts',(-66.,2.01711699607993,14.4208409176437));
#51271=CARTESIAN_POINT('Ctrl Pts',(-66.,2.00608233016073,14.3215862254212));
#51272=CARTESIAN_POINT('Ctrl Pts',(-66.,1.99348516764985,14.2225721274408));
#51273=CARTESIAN_POINT('Ctrl Pts',(-66.,1.97957384329226,14.1237862354018));
#51274=CARTESIAN_POINT('Ctrl Pts',(-66.,1.96749615602378,14.044934557742));
#51275=CARTESIAN_POINT('Ctrl Pts',(-66.,1.95792473331065,13.9858940930512));
#51276=CARTESIAN_POINT('Ctrl Pts',(-66.,1.9513160372573,13.9465774100468));
#51277=CARTESIAN_POINT('Ctrl Pts',(-66.,1.94795475120472,13.9269299753125));
#51278=CARTESIAN_POINT('',(-66.,3.31568234418832,13.6660219830951));
#51279=CARTESIAN_POINT('Origin',(-66.,0.,0.));
#51280=CARTESIAN_POINT('',(-66.,4.40398464539872,15.7716690379646));
#51281=CARTESIAN_POINT('Ctrl Pts',(-66.,3.31568234418832,13.6660219830951));
#51282=CARTESIAN_POINT('Ctrl Pts',(-66.,3.32025508218772,13.6889423777435));
#51283=CARTESIAN_POINT('Ctrl Pts',(-66.,3.32962290369722,13.7347480949923));
#51284=CARTESIAN_POINT('Ctrl Pts',(-66.,3.34434166251121,13.8033514635997));
#51285=CARTESIAN_POINT('Ctrl Pts',(-66.,3.36530258749166,13.8946118507282));
#51286=CARTESIAN_POINT('Ctrl Pts',(-66.,3.39378048711278,14.0083089910501));
#51287=CARTESIAN_POINT('Ctrl Pts',(-66.,3.42466963349977,14.1215479032503));
#51288=CARTESIAN_POINT('Ctrl Pts',(-66.,3.45822302631379,14.2341732241738));
#51289=CARTESIAN_POINT('Ctrl Pts',(-66.,3.49485794879717,14.3459208356842));
#51290=CARTESIAN_POINT('Ctrl Pts',(-66.,3.53511610244324,14.4564721136477));
#51291=CARTESIAN_POINT('Ctrl Pts',(-66.,3.57961415137445,14.5655275456869));
#51292=CARTESIAN_POINT('Ctrl Pts',(-66.,3.62898699781003,14.6728671135607));
#51293=CARTESIAN_POINT('Ctrl Pts',(-66.,3.68386053504292,14.7784329430806));
#51294=CARTESIAN_POINT('Ctrl Pts',(-66.,3.74465444426779,14.8823190942953));
#51295=CARTESIAN_POINT('Ctrl Pts',(-66.,3.81125317193191,14.9847182617076));
#51296=CARTESIAN_POINT('Ctrl Pts',(-66.,3.88279556209739,15.0858821011164));
#51297=CARTESIAN_POINT('Ctrl Pts',(-66.,3.95722328533246,15.1860781064647));
#51298=CARTESIAN_POINT('Ctrl Pts',(-66.,4.03163457417435,15.2855414194547));
#51299=CARTESIAN_POINT('Ctrl Pts',(-66.,4.10369589439471,15.3844104249513));
#51300=CARTESIAN_POINT('Ctrl Pts',(-66.,4.17266875139903,15.482674151341));
#51301=CARTESIAN_POINT('Ctrl Pts',(-66.,4.24085733833789,15.5800968628044));
#51302=CARTESIAN_POINT('Ctrl Pts',(-66.,4.29973028689649,15.6573251182294));
#51303=CARTESIAN_POINT('Ctrl Pts',(-66.,4.34907440371019,15.7145155989467));
#51304=CARTESIAN_POINT('Ctrl Pts',(-66.,4.38486856897779,15.7523532317835));
#51305=CARTESIAN_POINT('Ctrl Pts',(-66.,4.40365488112712,15.7713360829087));
#51306=CARTESIAN_POINT('Ctrl Pts',(-66.,4.40398464539872,15.7716690379646));
#51307=CARTESIAN_POINT('',(-66.,5.69475795663189,15.3528615187977));
#51308=CARTESIAN_POINT('Origin',(-66.,0.,0.));
#51309=CARTESIAN_POINT('',(-66.,5.35024281477072,13.004953213026));
#51310=CARTESIAN_POINT('Ctrl Pts',(-66.,5.69475795663189,15.3528615187977));
#51311=CARTESIAN_POINT('Ctrl Pts',(-66.,5.69582242796104,15.3427584331158));
#51312=CARTESIAN_POINT('Ctrl Pts',(-66.,5.69908409756002,15.3112588271944));
#51313=CARTESIAN_POINT('Ctrl Pts',(-66.,5.70425360416528,15.2584127623331));
#51314=CARTESIAN_POINT('Ctrl Pts',(-66.,5.71076402066882,15.1843250159624));
#51315=CARTESIAN_POINT('Ctrl Pts',(-66.,5.71772294845736,15.0891770284618));
#51316=CARTESIAN_POINT('Ctrl Pts',(-66.,5.72359388237569,14.9831894879022));
#51317=CARTESIAN_POINT('Ctrl Pts',(-66.,5.72754386270271,14.8776118616624));
#51318=CARTESIAN_POINT('Ctrl Pts',(-66.,5.72966360991829,14.772423041662));
#51319=CARTESIAN_POINT('Ctrl Pts',(-66.,5.73009695097776,14.6675837685266));
#51320=CARTESIAN_POINT('Ctrl Pts',(-66.,5.72896217357436,14.5630648469857));
#51321=CARTESIAN_POINT('Ctrl Pts',(-66.,5.72627848390049,14.4588735885414));
#51322=CARTESIAN_POINT('Ctrl Pts',(-66.,5.72190090792526,14.3550772805332));
#51323=CARTESIAN_POINT('Ctrl Pts',(-66.,5.71542331821735,14.2518379845708));
#51324=CARTESIAN_POINT('Ctrl Pts',(-66.,5.70626231068308,14.1493832151514));
#51325=CARTESIAN_POINT('Ctrl Pts',(-66.,5.6938022661864,14.0479549027521));
#51326=CARTESIAN_POINT('Ctrl Pts',(-66.,5.67752537508807,13.9477637996424));
#51327=CARTESIAN_POINT('Ctrl Pts',(-66.,5.65713696965892,13.8489453830157));
#51328=CARTESIAN_POINT('Ctrl Pts',(-66.,5.63272454065023,13.7515043267519));
#51329=CARTESIAN_POINT('Ctrl Pts',(-66.,5.60468396737303,13.6553383842666));
#51330=CARTESIAN_POINT('Ctrl Pts',(-66.,5.57358602861192,13.5602826717323));
#51331=CARTESIAN_POINT('Ctrl Pts',(-66.,5.54006285706051,13.466147083991));
#51332=CARTESIAN_POINT('Ctrl Pts',(-66.,5.50469122725311,13.3727548702637));
#51333=CARTESIAN_POINT('Ctrl Pts',(-66.,5.46786602291259,13.2799842691689));
#51334=CARTESIAN_POINT('Ctrl Pts',(-66.,5.42982469604617,13.1877615232676));
#51335=CARTESIAN_POINT('Ctrl Pts',(-66.,5.39851683671257,13.1143907147436));
#51336=CARTESIAN_POINT('Ctrl Pts',(-66.,5.37456335134248,13.0595854308535));
#51337=CARTESIAN_POINT('Ctrl Pts',(-66.,5.35838461816811,13.0231474696198));
#51338=CARTESIAN_POINT('Ctrl Pts',(-66.,5.35024281477071,13.004953213026));
#51339=CARTESIAN_POINT('',(-66.,6.61011555120064,12.4121021043889));
#51340=CARTESIAN_POINT('Origin',(-66.,0.,0.));
#51341=CARTESIAN_POINT('',(-66.,8.1878799628551,14.1809466085264));
#51342=CARTESIAN_POINT('Ctrl Pts',(-66.,6.61011555120064,12.4121021043889));
#51343=CARTESIAN_POINT('Ctrl Pts',(-66.,6.62024469858602,12.4331652189947));
#51344=CARTESIAN_POINT('Ctrl Pts',(-66.,6.64070963141069,12.4752021829311));
#51345=CARTESIAN_POINT('Ctrl Pts',(-66.,6.67202693734873,12.5379898440923));
#51346=CARTESIAN_POINT('Ctrl Pts',(-66.,6.71502487170408,12.6211703482748));
#51347=CARTESIAN_POINT('Ctrl Pts',(-66.,6.77088341473902,12.7242133182155));
#51348=CARTESIAN_POINT('Ctrl Pts',(-66.,6.82896349408885,12.8262128034276));
#51349=CARTESIAN_POINT('Ctrl Pts',(-66.,6.88947152371961,12.9269554033179));
#51350=CARTESIAN_POINT('Ctrl Pts',(-66.,6.95274599364373,13.0260815233846));
#51351=CARTESIAN_POINT('Ctrl Pts',(-66.,7.01923234820612,13.1231478339735));
#51352=CARTESIAN_POINT('Ctrl Pts',(-66.,7.08945339219251,13.2177108743086));
#51353=CARTESIAN_POINT('Ctrl Pts',(-66.,7.16396936488986,13.3093996446649));
#51354=CARTESIAN_POINT('Ctrl Pts',(-66.,7.24337210327696,13.3980024357456));
#51355=CARTESIAN_POINT('Ctrl Pts',(-66.,7.32809149527493,13.4835059820612));
#51356=CARTESIAN_POINT('Ctrl Pts',(-66.,7.41806353883254,13.5661256612623));
#51357=CARTESIAN_POINT('Ctrl Pts',(-66.,7.51251671706145,13.646319383691));
#51358=CARTESIAN_POINT('Ctrl Pts',(-66.,7.60952388977251,13.7248581251904));
#51359=CARTESIAN_POINT('Ctrl Pts',(-66.,7.70633293122716,13.8026912802767));
#51360=CARTESIAN_POINT('Ctrl Pts',(-66.,7.80071803438238,13.8805332125637));
#51361=CARTESIAN_POINT('Ctrl Pts',(-66.,7.89196117727994,13.9585569512687));
#51362=CARTESIAN_POINT('Ctrl Pts',(-66.,7.9822355374912,14.0359611371119));
#51363=CARTESIAN_POINT('Ctrl Pts',(-66.,8.05846477023863,14.0961220179458));
#51364=CARTESIAN_POINT('Ctrl Pts',(-66.,8.12048134508164,14.1392443717028));
#51365=CARTESIAN_POINT('Ctrl Pts',(-66.,8.16456080746724,14.1669916188038));
#51366=CARTESIAN_POINT('Ctrl Pts',(-66.,8.18747775617919,14.1807061229053));
#51367=CARTESIAN_POINT('Ctrl Pts',(-66.,8.1878799628551,14.1809466085264));
#51368=CARTESIAN_POINT('',(-66.,9.33394806226437,13.4542944285812));
#51369=CARTESIAN_POINT('Origin',(-66.,0.,0.));
#51370=CARTESIAN_POINT('',(-66.,8.41635544546802,11.2658274114927));
#51371=CARTESIAN_POINT('Ctrl Pts',(-66.,9.33394806226437,13.4542944285812));
#51372=CARTESIAN_POINT('Ctrl Pts',(-66.,9.33246655603105,13.4442440266596));
#51373=CARTESIAN_POINT('Ctrl Pts',(-66.,9.32779212083946,13.4129228945374));
#51374=CARTESIAN_POINT('Ctrl Pts',(-66.,9.3196569359812,13.3604514819665));
#51375=CARTESIAN_POINT('Ctrl Pts',(-66.,9.30753794249323,13.2870722636402));
#51376=CARTESIAN_POINT('Ctrl Pts',(-66.,9.29061590049322,13.1931829101653));
#51377=CARTESIAN_POINT('Ctrl Pts',(-66.,9.26994435872398,13.0890651211961));
#51378=CARTESIAN_POINT('Ctrl Pts',(-66.,9.24751415519882,12.9858220900665));
#51379=CARTESIAN_POINT('Ctrl Pts',(-66.,9.22340791088078,12.8834108105793));
#51380=CARTESIAN_POINT('Ctrl Pts',(-66.,9.19775517072751,12.7817574884561));
#51381=CARTESIAN_POINT('Ctrl Pts',(-66.,9.17066324563836,12.6808044286968));
#51382=CARTESIAN_POINT('Ctrl Pts',(-66.,9.14215255670447,12.580553936713));
#51383=CARTESIAN_POINT('Ctrl Pts',(-66.,9.11209941820162,12.4811072394643));
#51384=CARTESIAN_POINT('Ctrl Pts',(-66.,9.08015076502197,12.3827223068819));
#51385=CARTESIAN_POINT('Ctrl Pts',(-66.,9.04579810233888,12.2857645923749));
#51386=CARTESIAN_POINT('Ctrl Pts',(-66.,9.00850531748659,12.1906215239832));
#51387=CARTESIAN_POINT('Ctrl Pts',(-66.,8.96782328072592,12.0976260068268));
#51388=CARTESIAN_POINT('Ctrl Pts',(-66.,8.9235002736643,12.0069825427185));
#51389=CARTESIAN_POINT('Ctrl Pts',(-66.,8.87562220071675,11.9186739006343));
#51390=CARTESIAN_POINT('Ctrl Pts',(-66.,8.82454707622628,11.8325025950734));
#51391=CARTESIAN_POINT('Ctrl Pts',(-66.,8.77078674197194,11.7481669754252));
#51392=CARTESIAN_POINT('Ctrl Pts',(-66.,8.71490619380604,11.6653257040265));
#51393=CARTESIAN_POINT('Ctrl Pts',(-66.,8.657420129699,11.5836641450553));
#51394=CARTESIAN_POINT('Ctrl Pts',(-66.,8.59868074655117,11.5029661588994));
#51395=CARTESIAN_POINT('Ctrl Pts',(-66.,8.53889969364915,11.4231012534324));
#51396=CARTESIAN_POINT('Ctrl Pts',(-66.,8.49032885019461,11.3598214717827));
#51397=CARTESIAN_POINT('Ctrl Pts',(-66.,8.45349838774813,11.3126949862398));
#51398=CARTESIAN_POINT('Ctrl Pts',(-66.,8.4287661867593,11.2814252778905));
#51399=CARTESIAN_POINT('Ctrl Pts',(-66.,8.416355445468,11.2658274114927));
#51400=CARTESIAN_POINT('',(-66.,9.48921088782658,10.3782842019456));
#51401=CARTESIAN_POINT('Origin',(-66.,0.,0.));
#51402=CARTESIAN_POINT('',(-66.,11.4573006693292,11.699183149801));
#51403=CARTESIAN_POINT('Ctrl Pts',(-66.,9.48921088782658,10.3782842019456));
#51404=CARTESIAN_POINT('Ctrl Pts',(-66.,9.5042599930153,10.3961665635534));
#51405=CARTESIAN_POINT('Ctrl Pts',(-66.,9.53453615016101,10.4317934371322));
#51406=CARTESIAN_POINT('Ctrl Pts',(-66.,9.58048422171402,10.4848202111794));
#51407=CARTESIAN_POINT('Ctrl Pts',(-66.,9.64281744709338,10.5546942954216));
#51408=CARTESIAN_POINT('Ctrl Pts',(-66.,9.72254683584991,10.6406085262144));
#51409=CARTESIAN_POINT('Ctrl Pts',(-66.,9.80416846317344,10.7249595816546));
#51410=CARTESIAN_POINT('Ctrl Pts',(-66.,9.88782918758628,10.8074894324552));
#51411=CARTESIAN_POINT('Ctrl Pts',(-66.,9.97376743729857,10.8877656023939));
#51412=CARTESIAN_POINT('Ctrl Pts',(-66.,10.0623044106004,10.9652479123292));
#51413=CARTESIAN_POINT('Ctrl Pts',(-66.,10.1538362031934,11.0393768173572));
#51414=CARTESIAN_POINT('Ctrl Pts',(-66.,10.2488131895374,11.1096536475468));
#51415=CARTESIAN_POINT('Ctrl Pts',(-66.,10.347755963003,11.1757261609666));
#51416=CARTESIAN_POINT('Ctrl Pts',(-66.,10.4510776067987,11.237474600108));
#51417=CARTESIAN_POINT('Ctrl Pts',(-66.,10.558769691859,11.2951234927996));
#51418=CARTESIAN_POINT('Ctrl Pts',(-66.,10.6701988175887,11.3493082317362));
#51419=CARTESIAN_POINT('Ctrl Pts',(-66.,10.7836901223469,11.4012548314131));
#51420=CARTESIAN_POINT('Ctrl Pts',(-66.,10.896814048301,11.4525672852113));
#51421=CARTESIAN_POINT('Ctrl Pts',(-66.,11.0075923712357,11.5044910494005));
#51422=CARTESIAN_POINT('Ctrl Pts',(-66.,11.1153726577894,11.5573722819667));
#51423=CARTESIAN_POINT('Ctrl Pts',(-66.,11.2220605212152,11.6098943525204));
#51424=CARTESIAN_POINT('Ctrl Pts',(-66.,11.3108562751064,11.6492077293642));
#51425=CARTESIAN_POINT('Ctrl Pts',(-66.,11.3816485785003,11.6755524200814));
#51426=CARTESIAN_POINT('Ctrl Pts',(-66.,11.4312436632693,11.6914658198642));
#51427=CARTESIAN_POINT('Ctrl Pts',(-66.,11.4568512923737,11.6990502442108));
#51428=CARTESIAN_POINT('Ctrl Pts',(-66.,11.4573006693292,11.699183149801));
#51429=CARTESIAN_POINT('',(-66.,12.3866518832851,10.7103445379834));
#51430=CARTESIAN_POINT('Origin',(-66.,0.,0.));
#51431=CARTESIAN_POINT('',(-66.,10.9536375103364,8.81882824088046));
#51432=CARTESIAN_POINT('Ctrl Pts',(-66.,12.3866518832851,10.7103445379834));
#51433=CARTESIAN_POINT('Ctrl Pts',(-66.,12.3827174879745,10.7009783235375));
#51434=CARTESIAN_POINT('Ctrl Pts',(-66.,12.3704006599468,10.6718036871368));
#51435=CARTESIAN_POINT('Ctrl Pts',(-66.,12.3494719472088,10.6230038986845));
#51436=CARTESIAN_POINT('Ctrl Pts',(-66.,12.3194850246607,10.5549438945599));
#51437=CARTESIAN_POINT('Ctrl Pts',(-66.,12.2797452870059,10.4682125884904));
#51438=CARTESIAN_POINT('Ctrl Pts',(-66.,12.2338301385431,10.3725066547111));
#51439=CARTESIAN_POINT('Ctrl Pts',(-66.,12.1864291233458,10.2780853580389));
#51440=CARTESIAN_POINT('Ctrl Pts',(-66.,12.1376115714812,10.1848864963973));
#51441=CARTESIAN_POINT('Ctrl Pts',(-66.,12.0874846061232,10.0928063773702));
#51442=CARTESIAN_POINT('Ctrl Pts',(-66.,12.0361378186387,10.0017624314164));
#51443=CARTESIAN_POINT('Ctrl Pts',(-66.,11.9835915618855,9.91175181299999));
#51444=CARTESIAN_POINT('Ctrl Pts',(-66.,11.9297512100749,9.82290332823825));
#51445=CARTESIAN_POINT('Ctrl Pts',(-66.,11.8743389448017,9.73555464618448));
#51446=CARTESIAN_POINT('Ctrl Pts',(-66.,11.8169531311064,9.65018619637799));
#51447=CARTESIAN_POINT('Ctrl Pts',(-66.,11.7571708487241,9.56730656089267));
#51448=CARTESIAN_POINT('Ctrl Pts',(-66.,11.6946398682888,9.48734988004618));
#51449=CARTESIAN_POINT('Ctrl Pts',(-66.,11.629167237137,9.41057683066949));
#51450=CARTESIAN_POINT('Ctrl Pts',(-66.,11.5608318756571,9.3369493595236));
#51451=CARTESIAN_POINT('Ctrl Pts',(-66.,11.4899314378663,9.26618715093123));
#51452=CARTESIAN_POINT('Ctrl Pts',(-66.,11.4168866676366,9.19787074131628));
#51453=CARTESIAN_POINT('Ctrl Pts',(-66.,11.3421599232118,9.13152900801114));
#51454=CARTESIAN_POINT('Ctrl Pts',(-66.,11.2661714856319,9.06672919987649));
#51455=CARTESIAN_POINT('Ctrl Pts',(-66.,11.1892087351483,9.00317437991606));
#51456=CARTESIAN_POINT('Ctrl Pts',(-66.,11.1114442196238,8.9406855206164));
#51457=CARTESIAN_POINT('Ctrl Pts',(-66.,11.0486622767737,8.89147286724882));
#51458=CARTESIAN_POINT('Ctrl Pts',(-66.,11.0012690306593,8.85498631045878));
#51459=CARTESIAN_POINT('Ctrl Pts',(-66.,10.9695373770028,8.83084964577152));
#51460=CARTESIAN_POINT('Ctrl Pts',(-66.,10.9536375103364,8.81882824088047));
#51461=CARTESIAN_POINT('',(-66.,11.7720642054939,7.69236053443469));
#51462=CARTESIAN_POINT('Origin',(-66.,0.,0.));
#51463=CARTESIAN_POINT('',(-66.,14.0068170377451,8.48231698718778));
#51464=CARTESIAN_POINT('Ctrl Pts',(-66.,11.7720642054939,7.69236053443469));
#51465=CARTESIAN_POINT('Ctrl Pts',(-66.,11.7910876778603,7.70593852849788));
#51466=CARTESIAN_POINT('Ctrl Pts',(-66.,11.8292726970256,7.73291674422561));
#51467=CARTESIAN_POINT('Ctrl Pts',(-66.,11.8869644478727,7.77285076392682));
#51468=CARTESIAN_POINT('Ctrl Pts',(-66.,11.96471633848,7.82502798253687));
#51469=CARTESIAN_POINT('Ctrl Pts',(-66.,12.0633068822383,7.88841516709048));
#51470=CARTESIAN_POINT('Ctrl Pts',(-66.,12.1633414705075,7.94981770572398));
#51471=CARTESIAN_POINT('Ctrl Pts',(-66.,12.2648981787049,8.00894915338555));
#51472=CARTESIAN_POINT('Ctrl Pts',(-66.,12.3681003919172,8.06533132620399));
#51473=CARTESIAN_POINT('Ctrl Pts',(-66.,12.4731248803097,8.11836113699226));
#51474=CARTESIAN_POINT('Ctrl Pts',(-66.,12.5802161423503,8.16739811498339));
#51475=CARTESIAN_POINT('Ctrl Pts',(-66.,12.6896863889879,8.21184725330542));
#51476=CARTESIAN_POINT('Ctrl Pts',(-66.,12.8019522591891,8.25123791004828));
#51477=CARTESIAN_POINT('Ctrl Pts',(-66.,12.9173840759125,8.28535136048938));
#51478=CARTESIAN_POINT('Ctrl Pts',(-66.,13.0360295127074,8.31440717472604));
#51479=CARTESIAN_POINT('Ctrl Pts',(-66.,13.1574330841607,8.33917830374554));
#51480=CARTESIAN_POINT('Ctrl Pts',(-66.,13.2802774448963,8.36126876569594));
#51481=CARTESIAN_POINT('Ctrl Pts',(-66.,13.4026082630414,8.38283636801991));
#51482=CARTESIAN_POINT('Ctrl Pts',(-66.,13.5228191963114,8.40557940304509));
#51483=CARTESIAN_POINT('Ctrl Pts',(-66.,13.640364394729,8.42999540714673));
#51484=CARTESIAN_POINT('Ctrl Pts',(-66.,13.7567621705396,8.45433520755552));
#51485=CARTESIAN_POINT('Ctrl Pts',(-66.,13.8525450817897,8.47033087635756));
#51486=CARTESIAN_POINT('Ctrl Pts',(-66.,13.9276649729564,8.47824257022821));
#51487=CARTESIAN_POINT('Ctrl Pts',(-66.,13.9796594385348,8.481322225259));
#51488=CARTESIAN_POINT('Ctrl Pts',(-66.,14.0063487265167,8.48230001257543));
#51489=CARTESIAN_POINT('Ctrl Pts',(-66.,14.0068170377451,8.48231698718778));
#51490=CARTESIAN_POINT('',(-66.,14.66105681156,7.2934243101722));
#51491=CARTESIAN_POINT('Origin',(-66.,0.,0.));
#51492=CARTESIAN_POINT('',(-66.,12.8026622457696,5.81770965851215));
#51493=CARTESIAN_POINT('Ctrl Pts',(-66.,14.66105681156,7.2934243101722));
#51494=CARTESIAN_POINT('Ctrl Pts',(-66.,14.6549167396993,7.28533079690226));
#51495=CARTESIAN_POINT('Ctrl Pts',(-66.,14.6357314304385,7.26013580592497));
#51496=CARTESIAN_POINT('Ctrl Pts',(-66.,14.6033242178125,7.21807391177268));
#51497=CARTESIAN_POINT('Ctrl Pts',(-66.,14.5573535548322,7.15960958221619));
#51498=CARTESIAN_POINT('Ctrl Pts',(-66.,14.497293115392,7.08548597048793));
#51499=CARTESIAN_POINT('Ctrl Pts',(-66.,14.4290193778776,7.00420544769957));
#51500=CARTESIAN_POINT('Ctrl Pts',(-66.,14.3596259311217,6.92453872281182));
#51501=CARTESIAN_POINT('Ctrl Pts',(-66.,14.2891644580326,6.84640830625432));
#51502=CARTESIAN_POINT('Ctrl Pts',(-66.,14.2177129290574,6.76968712284877));
#51503=CARTESIAN_POINT('Ctrl Pts',(-66.,14.1453375866756,6.69427291666095));
#51504=CARTESIAN_POINT('Ctrl Pts',(-66.,14.0720574366665,6.62015787000295));
#51505=CARTESIAN_POINT('Ctrl Pts',(-66.,13.9978128588633,6.54749027478764));
#51506=CARTESIAN_POINT('Ctrl Pts',(-66.,13.9224187379158,6.47666628220192));
#51507=CARTESIAN_POINT('Ctrl Pts',(-66.,13.845605534933,6.40825111076043));
#51508=CARTESIAN_POINT('Ctrl Pts',(-66.,13.7670900956865,6.342842540489));
#51509=CARTESIAN_POINT('Ctrl Pts',(-66.,13.6866392230503,6.28094866827011));
#51510=CARTESIAN_POINT('Ctrl Pts',(-66.,13.6041308540151,6.22286996666888));
#51511=CARTESIAN_POINT('Ctrl Pts',(-66.,13.5196319660845,6.16854995125629));
#51512=CARTESIAN_POINT('Ctrl Pts',(-66.,13.4333611502533,6.11764308944358));
#51513=CARTESIAN_POINT('Ctrl Pts',(-66.,13.3456216156017,6.06963846112818));
#51514=CARTESIAN_POINT('Ctrl Pts',(-66.,13.2567440310958,6.02396476100794));
#51515=CARTESIAN_POINT('Ctrl Pts',(-66.,13.1670278530422,5.98009831397194));
#51516=CARTESIAN_POINT('Ctrl Pts',(-66.,13.0766775878848,5.93768004328337));
#51517=CARTESIAN_POINT('Ctrl Pts',(-66.,12.9858158402462,5.89649363499879));
#51518=CARTESIAN_POINT('Ctrl Pts',(-66.,12.9127676183656,5.86444032191588));
#51519=CARTESIAN_POINT('Ctrl Pts',(-66.,12.8577894805368,5.84088627843006));
#51520=CARTESIAN_POINT('Ctrl Pts',(-66.,12.8210521907127,5.82539925281556));
#51521=CARTESIAN_POINT('Ctrl Pts',(-66.,12.8026622457696,5.81770965851216));
#51522=CARTESIAN_POINT('',(-66.,13.3152354345065,4.52309756402217));
#51523=CARTESIAN_POINT('Origin',(-66.,0.,0.));
#51524=CARTESIAN_POINT('',(-66.,15.6762335782098,4.73247565248983));
#51525=CARTESIAN_POINT('Ctrl Pts',(-66.,13.3152354345065,4.52309756402217));
#51526=CARTESIAN_POINT('Ctrl Pts',(-66.,13.3370379593182,4.53151803523741));
#51527=CARTESIAN_POINT('Ctrl Pts',(-66.,13.3807325353144,4.54815245260096));
#51528=CARTESIAN_POINT('Ctrl Pts',(-66.,13.4465429805744,4.57248451663122));
#51529=CARTESIAN_POINT('Ctrl Pts',(-66.,13.5348280991712,4.60368638306948));
#51530=CARTESIAN_POINT('Ctrl Pts',(-66.,13.6460849914764,4.64056367145667));
#51531=CARTESIAN_POINT('Ctrl Pts',(-66.,13.7582469996088,4.67515954595839));
#51532=CARTESIAN_POINT('Ctrl Pts',(-66.,13.8713185101153,4.70717714415409));
#51533=CARTESIAN_POINT('Ctrl Pts',(-66.,13.9853001122203,4.73612262057495));
#51534=CARTESIAN_POINT('Ctrl Pts',(-66.,14.1002130408447,4.76136787417443));
#51535=CARTESIAN_POINT('Ctrl Pts',(-66.,14.2161348344847,4.78223175145606));
#51536=CARTESIAN_POINT('Ctrl Pts',(-66.,14.3332199232164,4.79806029507722));
#51537=CARTESIAN_POINT('Ctrl Pts',(-66.,14.4517548126435,4.80829403531135));
#51538=CARTESIAN_POINT('Ctrl Pts',(-66.,14.5720437967212,4.81262902350044));
#51539=CARTESIAN_POINT('Ctrl Pts',(-66.,14.6941876561096,4.81126607561379));
#51540=CARTESIAN_POINT('Ctrl Pts',(-66.,14.8179374404009,4.80506713357809));
#51541=CARTESIAN_POINT('Ctrl Pts',(-66.,14.9424160941388,4.79591343283465));
#51542=CARTESIAN_POINT('Ctrl Pts',(-66.,15.0662673092696,4.78638101191027));
#51543=CARTESIAN_POINT('Ctrl Pts',(-66.,15.1883575578327,4.77851428923771));
#51544=CARTESIAN_POINT('Ctrl Pts',(-66.,15.3082818709966,4.77293091754137));
#51545=CARTESIAN_POINT('Ctrl Pts',(-66.,15.4270758588568,4.76755908862997));
#51546=CARTESIAN_POINT('Ctrl Pts',(-66.,15.5238275348871,4.7592319826915));
#51547=CARTESIAN_POINT('Ctrl Pts',(-66.,15.598554954793,4.74821355889253));
#51548=CARTESIAN_POINT('Ctrl Pts',(-66.,15.6496817976862,4.73826596311956));
#51549=CARTESIAN_POINT('Ctrl Pts',(-66.,15.6757757584253,4.73257567543269));
#51550=CARTESIAN_POINT('Ctrl Pts',(-66.,15.6762335782098,4.73247565248983));
#51551=CARTESIAN_POINT('',(-66.,16.0142536207693,3.41823140961462));
#51552=CARTESIAN_POINT('Origin',(-66.,0.,0.));
#51553=CARTESIAN_POINT('',(-66.,13.847248627403,2.45104298226008));
#51554=CARTESIAN_POINT('Ctrl Pts',(-66.,16.0142536207693,3.41823140961462));
#51555=CARTESIAN_POINT('Ctrl Pts',(-66.,16.0062936756551,3.41191914272521));
#51556=CARTESIAN_POINT('Ctrl Pts',(-66.,15.9814453687008,3.39228689111509));
#51557=CARTESIAN_POINT('Ctrl Pts',(-66.,15.9395959205415,3.35960579476531));
#51558=CARTESIAN_POINT('Ctrl Pts',(-66.,15.8805300229522,3.31441066861968));
#51559=CARTESIAN_POINT('Ctrl Pts',(-66.,15.8039227000236,3.2575522103651));
#51560=CARTESIAN_POINT('Ctrl Pts',(-66.,15.7175802634788,3.19580425274334));
#51561=CARTESIAN_POINT('Ctrl Pts',(-66.,15.6305546306352,3.13589785295852));
#51562=CARTESIAN_POINT('Ctrl Pts',(-66.,15.542876589815,3.07774510290095));
#51563=CARTESIAN_POINT('Ctrl Pts',(-66.,15.4545900595684,3.02120352923108));
#51564=CARTESIAN_POINT('Ctrl Pts',(-66.,15.3657337712291,2.96615761473811));
#51565=CARTESIAN_POINT('Ctrl Pts',(-66.,15.2763241892947,2.9125950607961));
#51566=CARTESIAN_POINT('Ctrl Pts',(-66.,15.1863404453747,2.86067432738731));
#51567=CARTESIAN_POINT('Ctrl Pts',(-66.,15.0957017586521,2.81082515619622));
#51568=CARTESIAN_POINT('Ctrl Pts',(-66.,15.0042876224246,2.76366203995482));
#51569=CARTESIAN_POINT('Ctrl Pts',(-66.,14.9119724401214,2.71983439592332));
#51570=CARTESIAN_POINT('Ctrl Pts',(-66.,14.8186566994895,2.67989235195328));
#51571=CARTESIAN_POINT('Ctrl Pts',(-66.,14.7242968968419,2.64415729654763));
#51572=CARTESIAN_POINT('Ctrl Pts',(-66.,14.6289438583545,2.61255786321175));
#51573=CARTESIAN_POINT('Ctrl Pts',(-66.,14.5327233771235,2.58470501352874));
#51574=CARTESIAN_POINT('Ctrl Pts',(-66.,14.4358020756955,2.56002847385863));
#51575=CARTESIAN_POINT('Ctrl Pts',(-66.,14.338358156612,2.53789265347798));
#51576=CARTESIAN_POINT('Ctrl Pts',(-66.,14.2405514355047,2.51771585773738));
#51577=CARTESIAN_POINT('Ctrl Pts',(-66.,14.1424906951186,2.49909943227153));
#51578=CARTESIAN_POINT('Ctrl Pts',(-66.,14.0442408931361,2.48180336850756));
#51579=CARTESIAN_POINT('Ctrl Pts',(-66.,13.9655162806582,2.46892342325417));
#51580=CARTESIAN_POINT('Ctrl Pts',(-66.,13.9064077297103,2.45978188025048));
#51581=CARTESIAN_POINT('Ctrl Pts',(-66.,13.8669731427486,2.45391760048539));
#51582=CARTESIAN_POINT('Ctrl Pts',(-66.,13.847248627403,2.45104298226009));
#51583=CARTESIAN_POINT('',(-66.,14.0217614511585,1.06963173887291));
#51584=CARTESIAN_POINT('Origin',(-66.,0.,0.));
#51585=CARTESIAN_POINT('',(-66.,16.3606547098013,0.685275467717996));
#51586=CARTESIAN_POINT('Ctrl Pts',(-66.,14.0217614511585,1.06963173887291));
#51587=CARTESIAN_POINT('Ctrl Pts',(-66.,14.0449730955977,1.07236559806543));
#51588=CARTESIAN_POINT('Ctrl Pts',(-66.,14.0914317375174,1.07761101544474));
#51589=CARTESIAN_POINT('Ctrl Pts',(-66.,14.1612257648809,1.08481225073396));
#51590=CARTESIAN_POINT('Ctrl Pts',(-66.,14.2544968327758,1.09307823697967));
#51591=CARTESIAN_POINT('Ctrl Pts',(-66.,14.3714293939101,1.1011284935459));
#51592=CARTESIAN_POINT('Ctrl Pts',(-66.,14.4886712704316,1.10674391788617));
#51593=CARTESIAN_POINT('Ctrl Pts',(-66.,14.6061528843942,1.10963588316888));
#51594=CARTESIAN_POINT('Ctrl Pts',(-66.,14.7237519921366,1.10932591245462));
#51595=CARTESIAN_POINT('Ctrl Pts',(-66.,14.8413329590673,1.10520035673609));
#51596=CARTESIAN_POINT('Ctrl Pts',(-66.,14.9588014916819,1.09658017916666));
#51597=CARTESIAN_POINT('Ctrl Pts',(-66.,15.0761445357738,1.08279356247792));
#51598=CARTESIAN_POINT('Ctrl Pts',(-66.,15.1935004613832,1.06322736266735));
#51599=CARTESIAN_POINT('Ctrl Pts',(-66.,15.3110884135537,1.03751150535353));
#51600=CARTESIAN_POINT('Ctrl Pts',(-66.,15.4290559476364,1.00581543437186));
#51601=CARTESIAN_POINT('Ctrl Pts',(-66.,15.5473762906989,0.969035923607179));
#51602=CARTESIAN_POINT('Ctrl Pts',(-66.,15.6656677858244,0.929213220852553));
#51603=CARTESIAN_POINT('Ctrl Pts',(-66.,15.7832573706013,0.889179733744299));
#51604=CARTESIAN_POINT('Ctrl Pts',(-66.,15.8995555551237,0.851197548491309));
#51605=CARTESIAN_POINT('Ctrl Pts',(-66.,16.014323697387,0.815965624774873));
#51606=CARTESIAN_POINT('Ctrl Pts',(-66.,16.1280496341459,0.78121969830999));
#51607=CARTESIAN_POINT('Ctrl Pts',(-66.,16.2196908113235,0.749093040322084));
#51608=CARTESIAN_POINT('Ctrl Pts',(-66.,16.2893303613477,0.719836826943709));
#51609=CARTESIAN_POINT('Ctrl Pts',(-66.,16.3363770939854,0.697487024394078));
#51610=CARTESIAN_POINT('Ctrl Pts',(-66.,16.3602361479617,0.6854862034067));
#51611=CARTESIAN_POINT('Ctrl Pts',(-66.,16.3606547098013,0.685275467717996));
#51612=CARTESIAN_POINT('Origin',(-66.,0.,0.));
#51613=CARTESIAN_POINT('Ctrl Pts',(-50.,10.5997841913839,0.0676394565978705));
#51614=CARTESIAN_POINT('Ctrl Pts',(-21.,10.5997841913839,0.0676394565978705));
#51615=CARTESIAN_POINT('Ctrl Pts',(-50.,10.5813335008211,0.0524740444052774));
#51616=CARTESIAN_POINT('Ctrl Pts',(-21.,10.5813335008211,0.0524740444052774));
#51617=CARTESIAN_POINT('Ctrl Pts',(-50.,10.5443614263321,0.0223524300248218));
#51618=CARTESIAN_POINT('Ctrl Pts',(-21.,10.5443614263321,0.0223524300248218));
#51619=CARTESIAN_POINT('Ctrl Pts',(-50.,10.4886912348662,-0.0222023607441713));
#51620=CARTESIAN_POINT('Ctrl Pts',(-21.,10.4886912348662,-0.0222023607441713));
#51621=CARTESIAN_POINT('Ctrl Pts',(-50.,10.4140395862599,-0.0803518244312862));
#51622=CARTESIAN_POINT('Ctrl Pts',(-21.,10.4140395862599,-0.0803518244312862));
#51623=CARTESIAN_POINT('Ctrl Pts',(-50.,10.3200154257224,-0.150928577557962));
#51624=CARTESIAN_POINT('Ctrl Pts',(-21.,10.3200154257224,-0.150928577557962));
#51625=CARTESIAN_POINT('Ctrl Pts',(-50.,10.2252821497258,-0.21936662469166));
#51626=CARTESIAN_POINT('Ctrl Pts',(-21.,10.2252821497258,-0.21936662469166));
#51627=CARTESIAN_POINT('Ctrl Pts',(-50.,10.1298451744404,-0.285621225675487));
#51628=CARTESIAN_POINT('Ctrl Pts',(-21.,10.1298451744404,-0.285621225675487));
#51629=CARTESIAN_POINT('Ctrl Pts',(-50.,10.0337173245343,-0.349629916443317));
#51630=CARTESIAN_POINT('Ctrl Pts',(-21.,10.0337173245343,-0.349629916443317));
#51631=CARTESIAN_POINT('Ctrl Pts',(-50.,9.93692222450759,-0.411308601209036));
#51632=CARTESIAN_POINT('Ctrl Pts',(-21.,9.93692222450759,-0.411308601209036));
#51633=CARTESIAN_POINT('Ctrl Pts',(-50.,9.83949259364292,-0.470562407132084));
#51634=CARTESIAN_POINT('Ctrl Pts',(-21.,9.83949259364292,-0.470562407132084));
#51635=CARTESIAN_POINT('Ctrl Pts',(-50.,9.74146724538631,-0.527299895441833));
#51636=CARTESIAN_POINT('Ctrl Pts',(-21.,9.74146724538631,-0.527299895441833));
#51637=CARTESIAN_POINT('Ctrl Pts',(-50.,9.64288855622378,-0.581447879194613));
#51638=CARTESIAN_POINT('Ctrl Pts',(-21.,9.64288855622378,-0.581447879194613));
#51639=CARTESIAN_POINT('Ctrl Pts',(-50.,9.54380000381903,-0.632963053309266));
#51640=CARTESIAN_POINT('Ctrl Pts',(-21.,9.54380000381903,-0.632963053309266));
#51641=CARTESIAN_POINT('Ctrl Pts',(-50.,9.44424332627553,-0.681853728650741));
#51642=CARTESIAN_POINT('Ctrl Pts',(-21.,9.44424332627553,-0.681853728650741));
#51643=CARTESIAN_POINT('Ctrl Pts',(-50.,9.34425800352241,-0.728158030239757));
#51644=CARTESIAN_POINT('Ctrl Pts',(-21.,9.34425800352241,-0.728158030239757));
#51645=CARTESIAN_POINT('Ctrl Pts',(-50.,9.24388219451327,-0.771898853704204));
#51646=CARTESIAN_POINT('Ctrl Pts',(-21.,9.24388219451327,-0.771898853704204));
#51647=CARTESIAN_POINT('Ctrl Pts',(-50.,9.14315312384119,-0.813043722977556));
#51648=CARTESIAN_POINT('Ctrl Pts',(-21.,9.14315312384119,-0.813043722977556));
#51649=CARTESIAN_POINT('Ctrl Pts',(-50.,9.04210805084257,-0.851468211346448));
#51650=CARTESIAN_POINT('Ctrl Pts',(-21.,9.04210805084257,-0.851468211346448));
#51651=CARTESIAN_POINT('Ctrl Pts',(-50.,8.94078425956014,-0.886903960171006));
#51652=CARTESIAN_POINT('Ctrl Pts',(-21.,8.94078425956014,-0.886903960171006));
#51653=CARTESIAN_POINT('Ctrl Pts',(-50.,8.83922276353739,-0.91895289219465));
#51654=CARTESIAN_POINT('Ctrl Pts',(-21.,8.83922276353739,-0.91895289219465));
#51655=CARTESIAN_POINT('Ctrl Pts',(-50.,8.73747423363077,-0.947150867813171));
#51656=CARTESIAN_POINT('Ctrl Pts',(-21.,8.73747423363077,-0.947150867813171));
#51657=CARTESIAN_POINT('Ctrl Pts',(-50.,8.63560512714608,-0.971017102543952));
#51658=CARTESIAN_POINT('Ctrl Pts',(-21.,8.63560512714608,-0.971017102543952));
#51659=CARTESIAN_POINT('Ctrl Pts',(-50.,8.53370212161309,-0.990109101007578));
#51660=CARTESIAN_POINT('Ctrl Pts',(-21.,8.53370212161309,-0.990109101007578));
#51661=CARTESIAN_POINT('Ctrl Pts',(-50.,8.43188165539955,-1.00407739851957));
#51662=CARTESIAN_POINT('Ctrl Pts',(-21.,8.43188165539955,-1.00407739851957));
#51663=CARTESIAN_POINT('Ctrl Pts',(-50.,8.33027821569813,-1.01271355471894));
#51664=CARTESIAN_POINT('Ctrl Pts',(-21.,8.33027821569813,-1.01271355471894));
#51665=CARTESIAN_POINT('Ctrl Pts',(-50.,8.2290192302709,-1.01599010763451));
#51666=CARTESIAN_POINT('Ctrl Pts',(-21.,8.2290192302709,-1.01599010763451));
#51667=CARTESIAN_POINT('Ctrl Pts',(-50.,8.12820273854248,-1.01410892133532));
#51668=CARTESIAN_POINT('Ctrl Pts',(-21.,8.12820273854248,-1.01410892133532));
#51669=CARTESIAN_POINT('Ctrl Pts',(-50.,8.02787639670185,-1.00753800115478));
#51670=CARTESIAN_POINT('Ctrl Pts',(-21.,8.02787639670185,-1.00753800115478));
#51671=CARTESIAN_POINT('Ctrl Pts',(-50.,7.92800888935854,-0.997080466154163));
#51672=CARTESIAN_POINT('Ctrl Pts',(-21.,7.92800888935854,-0.997080466154163));
#51673=CARTESIAN_POINT('Ctrl Pts',(-50.,7.82850348500033,-0.983785216334556));
#51674=CARTESIAN_POINT('Ctrl Pts',(-21.,7.82850348500033,-0.983785216334556));
#51675=CARTESIAN_POINT('Ctrl Pts',(-50.,7.7292275500742,-0.968799418422936));
#51676=CARTESIAN_POINT('Ctrl Pts',(-21.,7.7292275500742,-0.968799418422936));
#51677=CARTESIAN_POINT('Ctrl Pts',(-50.,7.63003710778607,-0.953237934402832));
#51678=CARTESIAN_POINT('Ctrl Pts',(-21.,7.63003710778607,-0.953237934402832));
#51679=CARTESIAN_POINT('Ctrl Pts',(-50.,7.53080214904746,-0.938052795086853));
#51680=CARTESIAN_POINT('Ctrl Pts',(-21.,7.53080214904746,-0.938052795086853));
#51681=CARTESIAN_POINT('Ctrl Pts',(-50.,7.43143474677318,-0.923884053007732));
#51682=CARTESIAN_POINT('Ctrl Pts',(-21.,7.43143474677318,-0.923884053007732));
#51683=CARTESIAN_POINT('Ctrl Pts',(-50.,7.33188369780814,-0.9111053356665));
#51684=CARTESIAN_POINT('Ctrl Pts',(-21.,7.33188369780814,-0.9111053356665));
#51685=CARTESIAN_POINT('Ctrl Pts',(-50.,7.25207582250743,-0.902140734147995));
#51686=CARTESIAN_POINT('Ctrl Pts',(-21.,7.25207582250743,-0.902140734147995));
#51687=CARTESIAN_POINT('Ctrl Pts',(-50.,7.19212249719958,-0.896150298874621));
#51688=CARTESIAN_POINT('Ctrl Pts',(-21.,7.19212249719958,-0.896150298874621));
#51689=CARTESIAN_POINT('Ctrl Pts',(-50.,7.15211036864424,-0.892482057440589));
#51690=CARTESIAN_POINT('Ctrl Pts',(-21.,7.15211036864424,-0.892482057440589));
#51691=CARTESIAN_POINT('Ctrl Pts',(-50.,7.13209349341826,-0.890729280500493));
#51692=CARTESIAN_POINT('Ctrl Pts',(-21.,7.13209349341826,-0.890729280500493));
#51693=CARTESIAN_POINT('',(-21.5,9.99295703981581,-0.375246053138014));
#51694=CARTESIAN_POINT('Ctrl Pts',(-21.,9.47665840807863,-0.665541446186865));
#51695=CARTESIAN_POINT('Ctrl Pts',(-21.0648600646548,9.54397725881005,-0.632805485548985));
#51696=CARTESIAN_POINT('Ctrl Pts',(-21.1289204403021,9.61037774908651,-0.598586462588316));
#51697=CARTESIAN_POINT('Ctrl Pts',(-21.1924157855725,9.67606071178067,-0.562824879825102));
#51698=CARTESIAN_POINT('Ctrl Pts',(-21.2961101180279,9.78332764514829,-0.504422591651166));
#51699=CARTESIAN_POINT('Ctrl Pts',(-21.3982975032035,9.88867999737488,-0.441915547517655));
#51700=CARTESIAN_POINT('Ctrl Pts',(-21.5,9.99295703981581,-0.375246053138014));
#51701=CARTESIAN_POINT('',(-50.,7.13209349341826,-0.890729280500487));
#51702=CARTESIAN_POINT('',(-50.,7.13209349341826,-0.890729280500487));
#51703=CARTESIAN_POINT('',(-50.,9.99295703981581,-0.375246053138014));
#51704=CARTESIAN_POINT('Ctrl Pts',(-50.,7.13209349341826,-0.890729280500493));
#51705=CARTESIAN_POINT('Ctrl Pts',(-50.,7.15211036864424,-0.892482057440589));
#51706=CARTESIAN_POINT('Ctrl Pts',(-50.,7.19212249719958,-0.896150298874621));
#51707=CARTESIAN_POINT('Ctrl Pts',(-50.,7.25207582250743,-0.902140734147995));
#51708=CARTESIAN_POINT('Ctrl Pts',(-50.,7.33188369780814,-0.9111053356665));
#51709=CARTESIAN_POINT('Ctrl Pts',(-50.,7.43143474677318,-0.923884053007732));
#51710=CARTESIAN_POINT('Ctrl Pts',(-50.,7.53080214904746,-0.938052795086853));
#51711=CARTESIAN_POINT('Ctrl Pts',(-50.,7.63003710778607,-0.953237934402832));
#51712=CARTESIAN_POINT('Ctrl Pts',(-50.,7.7292275500742,-0.968799418422936));
#51713=CARTESIAN_POINT('Ctrl Pts',(-50.,7.82850348500033,-0.983785216334556));
#51714=CARTESIAN_POINT('Ctrl Pts',(-50.,7.92800888935854,-0.997080466154163));
#51715=CARTESIAN_POINT('Ctrl Pts',(-50.,8.02787639670185,-1.00753800115478));
#51716=CARTESIAN_POINT('Ctrl Pts',(-50.,8.12820273854248,-1.01410892133532));
#51717=CARTESIAN_POINT('Ctrl Pts',(-50.,8.2290192302709,-1.01599010763451));
#51718=CARTESIAN_POINT('Ctrl Pts',(-50.,8.33027821569813,-1.01271355471894));
#51719=CARTESIAN_POINT('Ctrl Pts',(-50.,8.43188165539955,-1.00407739851957));
#51720=CARTESIAN_POINT('Ctrl Pts',(-50.,8.53370212161309,-0.990109101007578));
#51721=CARTESIAN_POINT('Ctrl Pts',(-50.,8.63560512714608,-0.971017102543952));
#51722=CARTESIAN_POINT('Ctrl Pts',(-50.,8.73747423363077,-0.947150867813171));
#51723=CARTESIAN_POINT('Ctrl Pts',(-50.,8.83922276353739,-0.91895289219465));
#51724=CARTESIAN_POINT('Ctrl Pts',(-50.,8.94078425956014,-0.886903960171006));
#51725=CARTESIAN_POINT('Ctrl Pts',(-50.,9.04210805084257,-0.851468211346448));
#51726=CARTESIAN_POINT('Ctrl Pts',(-50.,9.14315312384119,-0.813043722977556));
#51727=CARTESIAN_POINT('Ctrl Pts',(-50.,9.24388219451327,-0.771898853704204));
#51728=CARTESIAN_POINT('Ctrl Pts',(-50.,9.34425800352241,-0.728158030239757));
#51729=CARTESIAN_POINT('Ctrl Pts',(-50.,9.44424332627553,-0.681853728650741));
#51730=CARTESIAN_POINT('Ctrl Pts',(-50.,9.54380000381903,-0.632963053309266));
#51731=CARTESIAN_POINT('Ctrl Pts',(-50.,9.64288855622378,-0.581447879194613));
#51732=CARTESIAN_POINT('Ctrl Pts',(-50.,9.74146724538631,-0.527299895441833));
#51733=CARTESIAN_POINT('Ctrl Pts',(-50.,9.83125393359042,-0.475330978595796));
#51734=CARTESIAN_POINT('Ctrl Pts',(-50.,9.9010538538092,-0.433097260939648));
#51735=CARTESIAN_POINT('Ctrl Pts',(-50.,9.95114599336045,-0.401850266969568));
#51736=CARTESIAN_POINT('Ctrl Pts',(-50.,9.98174010098887,-0.382417599458989));
#51737=CARTESIAN_POINT('Ctrl Pts',(-50.,9.99295703981614,-0.375246053137802));
#51738=CARTESIAN_POINT('Ctrl Pts',(-21.5,9.99295703981581,-0.375246053138015));
#51739=CARTESIAN_POINT('Ctrl Pts',(-26.3333333333333,9.99295703981581,-0.375246053138015));
#51740=CARTESIAN_POINT('Ctrl Pts',(-31.1666666666667,9.99295703981581,-0.375246053138015));
#51741=CARTESIAN_POINT('Ctrl Pts',(-40.6666666666667,9.99295703981581,-0.375246053138015));
#51742=CARTESIAN_POINT('Ctrl Pts',(-45.3333333333333,9.99295703981581,-0.375246053138014));
#51743=CARTESIAN_POINT('Ctrl Pts',(-50.,9.99295703981581,-0.375246053138014));
#51744=CARTESIAN_POINT('Origin',(-50.,0.,0.));
#51745=CARTESIAN_POINT('',(-50.,6.8122671513043,-2.29198004120026));
#51746=CARTESIAN_POINT('Origin',(-50.,0.,0.));
#51747=CARTESIAN_POINT('',(-50.,6.8122671513043,-2.29198004120026));
#51748=CARTESIAN_POINT('Ctrl Pts',(-50.,6.8122671513043,-2.29198004120026));
#51749=CARTESIAN_POINT('Ctrl Pts',(-21.,6.8122671513043,-2.29198004120026));
#51750=CARTESIAN_POINT('Ctrl Pts',(-50.,6.83461600336474,-2.30016217089616));
#51751=CARTESIAN_POINT('Ctrl Pts',(-21.,6.83461600336474,-2.30016217089616));
#51752=CARTESIAN_POINT('Ctrl Pts',(-50.,6.8793763726903,-2.31637371632821));
#51753=CARTESIAN_POINT('Ctrl Pts',(-21.,6.8793763726903,-2.31637371632821));
#51754=CARTESIAN_POINT('Ctrl Pts',(-50.,6.94670492800217,-2.3402328805745));
#51755=CARTESIAN_POINT('Ctrl Pts',(-21.,6.94670492800217,-2.3402328805745));
#51756=CARTESIAN_POINT('Ctrl Pts',(-50.,7.03685278876406,-2.37112767623027));
#51757=CARTESIAN_POINT('Ctrl Pts',(-21.,7.03685278876406,-2.37112767623027));
#51758=CARTESIAN_POINT('Ctrl Pts',(-50.,7.15012820840451,-2.4083053284885));
#51759=CARTESIAN_POINT('Ctrl Pts',(-21.,7.15012820840451,-2.4083053284885));
#51760=CARTESIAN_POINT('Ctrl Pts',(-50.,7.26387759821705,-2.44432136933076));
#51761=CARTESIAN_POINT('Ctrl Pts',(-21.,7.26387759821705,-2.44432136933076));
#51762=CARTESIAN_POINT('Ctrl Pts',(-50.,7.37786505179862,-2.47974127678492));
#51763=CARTESIAN_POINT('Ctrl Pts',(-21.,7.37786505179862,-2.47974127678492));
#51764=CARTESIAN_POINT('Ctrl Pts',(-50.,7.49168859641892,-2.51552733857386));
#51765=CARTESIAN_POINT('Ctrl Pts',(-21.,7.49168859641892,-2.51552733857386));
#51766=CARTESIAN_POINT('Ctrl Pts',(-50.,7.60482241577417,-2.55297760756074));
#51767=CARTESIAN_POINT('Ctrl Pts',(-21.,7.60482241577417,-2.55297760756074));
#51768=CARTESIAN_POINT('Ctrl Pts',(-50.,7.71666617412861,-2.59365833862295));
#51769=CARTESIAN_POINT('Ctrl Pts',(-21.,7.71666617412861,-2.59365833862295));
#51770=CARTESIAN_POINT('Ctrl Pts',(-50.,7.82659266808561,-2.63932460382938));
#51771=CARTESIAN_POINT('Ctrl Pts',(-21.,7.82659266808561,-2.63932460382938));
#51772=CARTESIAN_POINT('Ctrl Pts',(-50.,7.93399262158453,-2.69188736687836));
#51773=CARTESIAN_POINT('Ctrl Pts',(-21.,7.93399262158453,-2.69188736687836));
#51774=CARTESIAN_POINT('Ctrl Pts',(-50.,8.03835937937461,-2.75296659957235));
#51775=CARTESIAN_POINT('Ctrl Pts',(-21.,8.03835937937461,-2.75296659957235));
#51776=CARTESIAN_POINT('Ctrl Pts',(-50.,8.13939365460193,-2.82329483425037));
#51777=CARTESIAN_POINT('Ctrl Pts',(-21.,8.13939365460193,-2.82329483425037));
#51778=CARTESIAN_POINT('Ctrl Pts',(-50.,8.2370828133169,-2.90227874531213));
#51779=CARTESIAN_POINT('Ctrl Pts',(-21.,8.2370828133169,-2.90227874531213));
#51780=CARTESIAN_POINT('Ctrl Pts',(-50.,8.33184183835821,-2.98721060740199));
#51781=CARTESIAN_POINT('Ctrl Pts',(-21.,8.33184183835821,-2.98721060740199));
#51782=CARTESIAN_POINT('Ctrl Pts',(-50.,8.4243384303954,-3.07426635319921));
#51783=CARTESIAN_POINT('Ctrl Pts',(-21.,8.4243384303954,-3.07426635319921));
#51784=CARTESIAN_POINT('Ctrl Pts',(-50.,8.51516539363766,-3.16038325236223));
#51785=CARTESIAN_POINT('Ctrl Pts',(-21.,8.51516539363766,-3.16038325236223));
#51786=CARTESIAN_POINT('Ctrl Pts',(-50.,8.60460841273967,-3.24456764186082));
#51787=CARTESIAN_POINT('Ctrl Pts',(-21.,8.60460841273967,-3.24456764186082));
#51788=CARTESIAN_POINT('Ctrl Pts',(-50.,8.69226485417113,-3.33012809006974));
#51789=CARTESIAN_POINT('Ctrl Pts',(-21.,8.69226485417113,-3.33012809006974));
#51790=CARTESIAN_POINT('Ctrl Pts',(-50.,8.77716058006919,-3.42378642402312));
#51791=CARTESIAN_POINT('Ctrl Pts',(-21.,8.77716058006919,-3.42378642402312));
#51792=CARTESIAN_POINT('Ctrl Pts',(-50.,8.85834857876282,-3.53174964938136));
#51793=CARTESIAN_POINT('Ctrl Pts',(-21.,8.85834857876282,-3.53174964938136));
#51794=CARTESIAN_POINT('Ctrl Pts',(-50.,8.93534116084886,-3.65684682750522));
#51795=CARTESIAN_POINT('Ctrl Pts',(-21.,8.93534116084886,-3.65684682750522));
#51796=CARTESIAN_POINT('Ctrl Pts',(-50.,9.0086889241718,-3.79469796977264));
#51797=CARTESIAN_POINT('Ctrl Pts',(-21.,9.0086889241718,-3.79469796977264));
#51798=CARTESIAN_POINT('Ctrl Pts',(-50.,9.08026462895257,-3.93186755639596));
#51799=CARTESIAN_POINT('Ctrl Pts',(-21.,9.08026462895257,-3.93186755639596));
#51800=CARTESIAN_POINT('Ctrl Pts',(-50.,9.15270492381554,-4.04971509082727));
#51801=CARTESIAN_POINT('Ctrl Pts',(-21.,9.15270492381554,-4.04971509082727));
#51802=CARTESIAN_POINT('Ctrl Pts',(-50.,9.22899343053301,-4.12729029694314));
#51803=CARTESIAN_POINT('Ctrl Pts',(-21.,9.22899343053301,-4.12729029694314));
#51804=CARTESIAN_POINT('Ctrl Pts',(-50.,9.31200173345042,-4.1445121148068));
#51805=CARTESIAN_POINT('Ctrl Pts',(-21.,9.31200173345042,-4.1445121148068));
#51806=CARTESIAN_POINT('Ctrl Pts',(-50.,9.4040191976898,-4.08543198173291));
#51807=CARTESIAN_POINT('Ctrl Pts',(-21.,9.4040191976898,-4.08543198173291));
#51808=CARTESIAN_POINT('Ctrl Pts',(-50.,9.50679569557631,-3.93791789477537));
#51809=CARTESIAN_POINT('Ctrl Pts',(-21.,9.50679569557631,-3.93791789477537));
#51810=CARTESIAN_POINT('Ctrl Pts',(-50.,9.6216277792442,-3.69303758521427));
#51811=CARTESIAN_POINT('Ctrl Pts',(-21.,9.6216277792442,-3.69303758521427));
#51812=CARTESIAN_POINT('Ctrl Pts',(-50.,9.74942513377921,-3.34458014605708));
#51813=CARTESIAN_POINT('Ctrl Pts',(-21.,9.74942513377921,-3.34458014605708));
#51814=CARTESIAN_POINT('Ctrl Pts',(-50.,9.89078169235227,-2.88854649339194));
#51815=CARTESIAN_POINT('Ctrl Pts',(-21.,9.89078169235227,-2.88854649339194));
#51816=CARTESIAN_POINT('Ctrl Pts',(-50.,10.0460413192499,-2.32267878361756));
#51817=CARTESIAN_POINT('Ctrl Pts',(-21.,10.0460413192499,-2.32267878361756));
#51818=CARTESIAN_POINT('Ctrl Pts',(-50.,10.2153627041086,-1.64599643173284));
#51819=CARTESIAN_POINT('Ctrl Pts',(-21.,10.2153627041086,-1.64599643173284));
#51820=CARTESIAN_POINT('Ctrl Pts',(-50.,10.3620979683038,-1.01587958589522));
#51821=CARTESIAN_POINT('Ctrl Pts',(-21.,10.3620979683038,-1.01587958589522));
#51822=CARTESIAN_POINT('Ctrl Pts',(-50.,10.478481770919,-0.493469650218984));
#51823=CARTESIAN_POINT('Ctrl Pts',(-21.,10.478481770919,-0.493469650218984));
#51824=CARTESIAN_POINT('Ctrl Pts',(-50.,10.5588816113278,-0.123082548500186));
#51825=CARTESIAN_POINT('Ctrl Pts',(-21.,10.5588816113278,-0.123082548500186));
#51826=CARTESIAN_POINT('Ctrl Pts',(-50.,10.5997841913839,0.0676394565978705));
#51827=CARTESIAN_POINT('Ctrl Pts',(-21.,10.5997841913839,0.0676394565978705));
#51828=CARTESIAN_POINT('',(-21.5,9.14990386923577,-4.03475639707582));
#51829=CARTESIAN_POINT('Ctrl Pts',(-21.5,9.14990386923577,-4.03475639707581));
#51830=CARTESIAN_POINT('Ctrl Pts',(-21.4716714037531,9.13031726529337,-4.00896291438969));
#51831=CARTESIAN_POINT('Ctrl Pts',(-21.4424150110748,9.11133064989716,-3.97941274406063));
#51832=CARTESIAN_POINT('Ctrl Pts',(-21.2909879716453,9.01605057347099,-3.81864524910466));
#51833=CARTESIAN_POINT('Ctrl Pts',(-21.1630186724944,8.94508544457216,-3.65653131387786));
#51834=CARTESIAN_POINT('Ctrl Pts',(-21.,8.83189477299562,-3.49966208636385));
#51835=CARTESIAN_POINT('',(-50.,9.14990386923577,-4.03475639707582));
#51836=CARTESIAN_POINT('Ctrl Pts',(-50.,9.14990386923578,-4.03475639707582));
#51837=CARTESIAN_POINT('Ctrl Pts',(-45.1666666666667,9.14990386923578,-4.03475639707582));
#51838=CARTESIAN_POINT('Ctrl Pts',(-40.3333333333333,9.14990386923578,-4.03475639707582));
#51839=CARTESIAN_POINT('Ctrl Pts',(-30.8333333333333,9.14990386923578,-4.03475639707582));
#51840=CARTESIAN_POINT('Ctrl Pts',(-26.1666666666667,9.14990386923578,-4.03475639707582));
#51841=CARTESIAN_POINT('Ctrl Pts',(-21.5,9.14990386923578,-4.03475639707582));
#51842=CARTESIAN_POINT('Ctrl Pts',(-50.,9.14990386923577,-4.03475639707581));
#51843=CARTESIAN_POINT('Ctrl Pts',(-50.,9.13577160343033,-4.01614569996669));
#51844=CARTESIAN_POINT('Ctrl Pts',(-50.,9.10709633384263,-3.97431669461607));
#51845=CARTESIAN_POINT('Ctrl Pts',(-50.,9.06450371311672,-3.90166326358648));
#51846=CARTESIAN_POINT('Ctrl Pts',(-50.,9.00794825534563,-3.79330594308901));
#51847=CARTESIAN_POINT('Ctrl Pts',(-50.,8.93534116084886,-3.65684682750522));
#51848=CARTESIAN_POINT('Ctrl Pts',(-50.,8.85834857876282,-3.53174964938136));
#51849=CARTESIAN_POINT('Ctrl Pts',(-50.,8.77716058006919,-3.42378642402312));
#51850=CARTESIAN_POINT('Ctrl Pts',(-50.,8.69226485417113,-3.33012809006974));
#51851=CARTESIAN_POINT('Ctrl Pts',(-50.,8.60460841273967,-3.24456764186082));
#51852=CARTESIAN_POINT('Ctrl Pts',(-50.,8.51516539363766,-3.16038325236223));
#51853=CARTESIAN_POINT('Ctrl Pts',(-50.,8.4243384303954,-3.07426635319921));
#51854=CARTESIAN_POINT('Ctrl Pts',(-50.,8.33184183835821,-2.98721060740199));
#51855=CARTESIAN_POINT('Ctrl Pts',(-50.,8.2370828133169,-2.90227874531213));
#51856=CARTESIAN_POINT('Ctrl Pts',(-50.,8.13939365460193,-2.82329483425037));
#51857=CARTESIAN_POINT('Ctrl Pts',(-50.,8.03835937937461,-2.75296659957235));
#51858=CARTESIAN_POINT('Ctrl Pts',(-50.,7.93399262158453,-2.69188736687836));
#51859=CARTESIAN_POINT('Ctrl Pts',(-50.,7.82659266808561,-2.63932460382938));
#51860=CARTESIAN_POINT('Ctrl Pts',(-50.,7.71666617412861,-2.59365833862295));
#51861=CARTESIAN_POINT('Ctrl Pts',(-50.,7.60482241577417,-2.55297760756074));
#51862=CARTESIAN_POINT('Ctrl Pts',(-50.,7.49168859641892,-2.51552733857386));
#51863=CARTESIAN_POINT('Ctrl Pts',(-50.,7.37786505179862,-2.47974127678492));
#51864=CARTESIAN_POINT('Ctrl Pts',(-50.,7.26387759821705,-2.44432136933076));
#51865=CARTESIAN_POINT('Ctrl Pts',(-50.,7.15012820840451,-2.4083053284885));
#51866=CARTESIAN_POINT('Ctrl Pts',(-50.,7.03685278876406,-2.37112767623027));
#51867=CARTESIAN_POINT('Ctrl Pts',(-50.,6.94670492800217,-2.3402328805745));
#51868=CARTESIAN_POINT('Ctrl Pts',(-50.,6.8793763726903,-2.31637371632821));
#51869=CARTESIAN_POINT('Ctrl Pts',(-50.,6.83461600336474,-2.30016217089616));
#51870=CARTESIAN_POINT('Ctrl Pts',(-50.,6.8122671513043,-2.29198004120026));
#51871=CARTESIAN_POINT('Origin',(-21.25,0.,0.));
#51872=CARTESIAN_POINT('',(-21.5,9.99439372247306,0.334804600014791));
#51873=CARTESIAN_POINT('Origin',(-21.5,0.,0.));
#51874=CARTESIAN_POINT('Ctrl Pts',(-21.5,9.99439372247306,0.334804600014791));
#51875=CARTESIAN_POINT('Ctrl Pts',(-21.4716714037526,9.96555542937976,0.349545415954904));
#51876=CARTESIAN_POINT('Ctrl Pts',(-21.4424150110737,9.93562774160641,0.367931215781723));
#51877=CARTESIAN_POINT('Ctrl Pts',(-21.2909879716438,9.78002895717459,0.471437247885104));
#51878=CARTESIAN_POINT('Ctrl Pts',(-21.1630186724941,9.64575298495204,0.586706241102918));
#51879=CARTESIAN_POINT('Ctrl Pts',(-21.,9.47570870673866,0.678928939607903));
#51880=CARTESIAN_POINT('Origin',(-35.75,0.,0.));
#51881=CARTESIAN_POINT('',(-50.,9.99439372247306,0.334804600014791));
#51882=CARTESIAN_POINT('Origin',(-50.,0.,0.));
#51883=CARTESIAN_POINT('Ctrl Pts',(-50.,9.99439372247306,0.334804600014792));
#51884=CARTESIAN_POINT('Ctrl Pts',(-45.1666666666667,9.99439372247306,0.334804600014792));
#51885=CARTESIAN_POINT('Ctrl Pts',(-40.3333333333333,9.99439372247306,0.334804600014792));
#51886=CARTESIAN_POINT('Ctrl Pts',(-30.8333333333333,9.99439372247306,0.334804600014792));
#51887=CARTESIAN_POINT('Ctrl Pts',(-26.1666666666667,9.99439372247306,0.334804600014792));
#51888=CARTESIAN_POINT('Ctrl Pts',(-21.5,9.99439372247306,0.334804600014792));
#51889=CARTESIAN_POINT('Ctrl Pts',(-50.,5.14318775290069,-5.02073460645076));
#51890=CARTESIAN_POINT('Ctrl Pts',(-21.,5.14318775290069,-5.02073460645076));
#51891=CARTESIAN_POINT('Ctrl Pts',(-50.,5.1597732798141,-5.03780325407688));
#51892=CARTESIAN_POINT('Ctrl Pts',(-21.,5.1597732798141,-5.03780325407688));
#51893=CARTESIAN_POINT('Ctrl Pts',(-50.,5.19306705314332,-5.071830148219));
#51894=CARTESIAN_POINT('Ctrl Pts',(-21.,5.19306705314332,-5.071830148219));
#51895=CARTESIAN_POINT('Ctrl Pts',(-50.,5.24337588200475,-5.12253927774717));
#51896=CARTESIAN_POINT('Ctrl Pts',(-21.,5.24337588200475,-5.12253927774717));
#51897=CARTESIAN_POINT('Ctrl Pts',(-50.,5.31119154860082,-5.18948821771405));
#51898=CARTESIAN_POINT('Ctrl Pts',(-21.,5.31119154860082,-5.18948821771405));
#51899=CARTESIAN_POINT('Ctrl Pts',(-50.,5.39711839642203,-5.27213248760413));
#51900=CARTESIAN_POINT('Ctrl Pts',(-21.,5.39711839642203,-5.27213248760413));
#51901=CARTESIAN_POINT('Ctrl Pts',(-50.,5.48397628091718,-5.35393582972231));
#51902=CARTESIAN_POINT('Ctrl Pts',(-21.,5.48397628091718,-5.35393582972231));
#51903=CARTESIAN_POINT('Ctrl Pts',(-50.,5.57130730604024,-5.43530536621495));
#51904=CARTESIAN_POINT('Ctrl Pts',(-21.,5.57130730604024,-5.43530536621495));
#51905=CARTESIAN_POINT('Ctrl Pts',(-50.,5.65833178588016,-5.51693367893109));
#51906=CARTESIAN_POINT('Ctrl Pts',(-21.,5.65833178588016,-5.51693367893109));
#51907=CARTESIAN_POINT('Ctrl Pts',(-50.,5.74401277228714,-5.59976212994534));
#51908=CARTESIAN_POINT('Ctrl Pts',(-21.,5.74401277228714,-5.59976212994534));
#51909=CARTESIAN_POINT('Ctrl Pts',(-50.,5.82712980893039,-5.68494139022769));
#51910=CARTESIAN_POINT('Ctrl Pts',(-21.,5.82712980893039,-5.68494139022769));
#51911=CARTESIAN_POINT('Ctrl Pts',(-50.,5.906356307844,-5.77378059171821));
#51912=CARTESIAN_POINT('Ctrl Pts',(-21.,5.906356307844,-5.77378059171821));
#51913=CARTESIAN_POINT('Ctrl Pts',(-50.,5.98031419419066,-5.86773709824143));
#51914=CARTESIAN_POINT('Ctrl Pts',(-21.,5.98031419419066,-5.86773709824143));
#51915=CARTESIAN_POINT('Ctrl Pts',(-50.,6.04784410793973,-5.96805062448362));
#51916=CARTESIAN_POINT('Ctrl Pts',(-21.,6.04784410793973,-5.96805062448362));
#51917=CARTESIAN_POINT('Ctrl Pts',(-50.,6.108358567083,-6.07525130357771));
#51918=CARTESIAN_POINT('Ctrl Pts',(-21.,6.108358567083,-6.07525130357771));
#51919=CARTESIAN_POINT('Ctrl Pts',(-50.,6.16210362315516,-6.18879908596403));
#51920=CARTESIAN_POINT('Ctrl Pts',(-21.,6.16210362315516,-6.18879908596403));
#51921=CARTESIAN_POINT('Ctrl Pts',(-50.,6.2106280007764,-6.30643444970003));
#51922=CARTESIAN_POINT('Ctrl Pts',(-21.,6.2106280007764,-6.30643444970003));
#51923=CARTESIAN_POINT('Ctrl Pts',(-50.,6.25619247809081,-6.42500173364409));
#51924=CARTESIAN_POINT('Ctrl Pts',(-21.,6.25619247809081,-6.42500173364409));
#51925=CARTESIAN_POINT('Ctrl Pts',(-50.,6.30066002212815,-6.5419987212145));
#51926=CARTESIAN_POINT('Ctrl Pts',(-21.,6.30066002212815,-6.5419987212145));
#51927=CARTESIAN_POINT('Ctrl Pts',(-50.,6.34471916009928,-6.65665410688205));
#51928=CARTESIAN_POINT('Ctrl Pts',(-21.,6.34471916009928,-6.65665410688205));
#51929=CARTESIAN_POINT('Ctrl Pts',(-50.,6.38657159771068,-6.77177411160809));
#51930=CARTESIAN_POINT('Ctrl Pts',(-21.,6.38657159771068,-6.77177411160809));
#51931=CARTESIAN_POINT('Ctrl Pts',(-50.,6.42242317562759,-6.89299222970744));
#51932=CARTESIAN_POINT('Ctrl Pts',(-21.,6.42242317562759,-6.89299222970744));
#51933=CARTESIAN_POINT('Ctrl Pts',(-50.,6.44872754699223,-7.02548988707821));
#51934=CARTESIAN_POINT('Ctrl Pts',(-21.,6.44872754699223,-7.02548988707821));
#51935=CARTESIAN_POINT('Ctrl Pts',(-50.,6.46381783511374,-7.17160437943005));
#51936=CARTESIAN_POINT('Ctrl Pts',(-21.,6.46381783511374,-7.17160437943005));
#51937=CARTESIAN_POINT('Ctrl Pts',(-50.,6.47009051734937,-7.32762836882426));
#51938=CARTESIAN_POINT('Ctrl Pts',(-21.,6.47009051734937,-7.32762836882426));
#51939=CARTESIAN_POINT('Ctrl Pts',(-50.,6.47506234591768,-7.48226943041517));
#51940=CARTESIAN_POINT('Ctrl Pts',(-21.,6.47506234591768,-7.48226943041517));
#51941=CARTESIAN_POINT('Ctrl Pts',(-50.,6.48919666748604,-7.61987705609476));
#51942=CARTESIAN_POINT('Ctrl Pts',(-21.,6.48919666748604,-7.61987705609476));
#51943=CARTESIAN_POINT('Ctrl Pts',(-50.,6.52427161652488,-7.72287024427254));
#51944=CARTESIAN_POINT('Ctrl Pts',(-21.,6.52427161652488,-7.72287024427254));
#51945=CARTESIAN_POINT('Ctrl Pts',(-50.,6.59158724650179,-7.774402518864));
#51946=CARTESIAN_POINT('Ctrl Pts',(-21.,6.59158724650179,-7.774402518864));
#51947=CARTESIAN_POINT('Ctrl Pts',(-50.,6.70012602613047,-7.76109803970118));
#51948=CARTESIAN_POINT('Ctrl Pts',(-21.,6.70012602613047,-7.76109803970118));
#51949=CARTESIAN_POINT('Ctrl Pts',(-50.,6.8567284146999,-7.67278549097179));
#51950=CARTESIAN_POINT('Ctrl Pts',(-21.,6.8567284146999,-7.67278549097179));
#51951=CARTESIAN_POINT('Ctrl Pts',(-50.,7.06643813146967,-7.50197972952742));
#51952=CARTESIAN_POINT('Ctrl Pts',(-21.,7.06643813146967,-7.50197972952742));
#51953=CARTESIAN_POINT('Ctrl Pts',(-50.,7.33276958593085,-7.24347961909277));
#51954=CARTESIAN_POINT('Ctrl Pts',(-21.,7.33276958593085,-7.24347961909277));
#51955=CARTESIAN_POINT('Ctrl Pts',(-50.,7.65799303086079,-6.89393980750813));
#51956=CARTESIAN_POINT('Ctrl Pts',(-21.,7.65799303086079,-6.89393980750813));
#51957=CARTESIAN_POINT('Ctrl Pts',(-50.,8.04339791890053,-6.45147524510253));
#51958=CARTESIAN_POINT('Ctrl Pts',(-21.,8.04339791890053,-6.45147524510253));
#51959=CARTESIAN_POINT('Ctrl Pts',(-50.,8.48955268435888,-5.91527130817043));
#51960=CARTESIAN_POINT('Ctrl Pts',(-21.,8.48955268435888,-5.91527130817043));
#51961=CARTESIAN_POINT('Ctrl Pts',(-50.,8.89515404237518,-5.41122169201928));
#51962=CARTESIAN_POINT('Ctrl Pts',(-21.,8.89515404237518,-5.41122169201928));
#51963=CARTESIAN_POINT('Ctrl Pts',(-50.,9.22667740150299,-4.99104364314351));
#51964=CARTESIAN_POINT('Ctrl Pts',(-21.,9.22667740150299,-4.99104364314351));
#51965=CARTESIAN_POINT('Ctrl Pts',(-50.,9.45982009531033,-4.69222057880331));
#51966=CARTESIAN_POINT('Ctrl Pts',(-21.,9.45982009531033,-4.69222057880331));
#51967=CARTESIAN_POINT('Ctrl Pts',(-50.,9.57942322326164,-4.53813295416029));
#51968=CARTESIAN_POINT('Ctrl Pts',(-21.,9.57942322326164,-4.53813295416029));
#51969=CARTESIAN_POINT('',(-50.,6.49316333848958,-7.60518440668567));
#51970=CARTESIAN_POINT('',(-21.5,6.49316333848958,-7.60518440668567));
#51971=CARTESIAN_POINT('Ctrl Pts',(-50.,6.49316333848958,-7.60518440668567));
#51972=CARTESIAN_POINT('Ctrl Pts',(-45.1666666666667,6.49316333848958,-7.60518440668567));
#51973=CARTESIAN_POINT('Ctrl Pts',(-40.3333333333333,6.49316333848958,-7.60518440668567));
#51974=CARTESIAN_POINT('Ctrl Pts',(-30.8333333333333,6.49316333848958,-7.60518440668567));
#51975=CARTESIAN_POINT('Ctrl Pts',(-26.1666666666667,6.49316333848958,-7.60518440668567));
#51976=CARTESIAN_POINT('Ctrl Pts',(-21.5,6.49316333848958,-7.60518440668567));
#51977=CARTESIAN_POINT('',(-50.,5.14318775290069,-5.02073460645076));
#51978=CARTESIAN_POINT('Ctrl Pts',(-50.,6.49316333848958,-7.60518440668567));
#51979=CARTESIAN_POINT('Ctrl Pts',(-50.,6.48850548581524,-7.58228498765052));
#51980=CARTESIAN_POINT('Ctrl Pts',(-50.,6.48081888588311,-7.53215662286537));
#51981=CARTESIAN_POINT('Ctrl Pts',(-50.,6.47396740292153,-7.44821789782204));
#51982=CARTESIAN_POINT('Ctrl Pts',(-50.,6.47002717553801,-7.32605283195927));
#51983=CARTESIAN_POINT('Ctrl Pts',(-50.,6.46381783511374,-7.17160437943005));
#51984=CARTESIAN_POINT('Ctrl Pts',(-50.,6.44872754699223,-7.02548988707821));
#51985=CARTESIAN_POINT('Ctrl Pts',(-50.,6.42242317562759,-6.89299222970744));
#51986=CARTESIAN_POINT('Ctrl Pts',(-50.,6.38657159771068,-6.77177411160809));
#51987=CARTESIAN_POINT('Ctrl Pts',(-50.,6.34471916009928,-6.65665410688205));
#51988=CARTESIAN_POINT('Ctrl Pts',(-50.,6.30066002212815,-6.5419987212145));
#51989=CARTESIAN_POINT('Ctrl Pts',(-50.,6.25619247809081,-6.42500173364409));
#51990=CARTESIAN_POINT('Ctrl Pts',(-50.,6.2106280007764,-6.30643444970003));
#51991=CARTESIAN_POINT('Ctrl Pts',(-50.,6.16210362315516,-6.18879908596403));
#51992=CARTESIAN_POINT('Ctrl Pts',(-50.,6.108358567083,-6.07525130357771));
#51993=CARTESIAN_POINT('Ctrl Pts',(-50.,6.04784410793973,-5.96805062448362));
#51994=CARTESIAN_POINT('Ctrl Pts',(-50.,5.98031419419066,-5.86773709824143));
#51995=CARTESIAN_POINT('Ctrl Pts',(-50.,5.906356307844,-5.77378059171821));
#51996=CARTESIAN_POINT('Ctrl Pts',(-50.,5.82712980893039,-5.68494139022769));
#51997=CARTESIAN_POINT('Ctrl Pts',(-50.,5.74401277228714,-5.59976212994534));
#51998=CARTESIAN_POINT('Ctrl Pts',(-50.,5.65833178588016,-5.51693367893109));
#51999=CARTESIAN_POINT('Ctrl Pts',(-50.,5.57130730604024,-5.43530536621495));
#52000=CARTESIAN_POINT('Ctrl Pts',(-50.,5.48397628091718,-5.35393582972231));
#52001=CARTESIAN_POINT('Ctrl Pts',(-50.,5.39711839642203,-5.27213248760413));
#52002=CARTESIAN_POINT('Ctrl Pts',(-50.,5.31119154860082,-5.18948821771405));
#52003=CARTESIAN_POINT('Ctrl Pts',(-50.,5.24337588200475,-5.12253927774717));
#52004=CARTESIAN_POINT('Ctrl Pts',(-50.,5.19306705314332,-5.071830148219));
#52005=CARTESIAN_POINT('Ctrl Pts',(-50.,5.1597732798141,-5.03780325407688));
#52006=CARTESIAN_POINT('Ctrl Pts',(-50.,5.14318775290069,-5.02073460645076));
#52007=CARTESIAN_POINT('',(-50.,5.14318775290069,-5.02073460645076));
#52008=CARTESIAN_POINT('Ctrl Pts',(-21.5,6.49316333848958,-7.60518440668567));
#52009=CARTESIAN_POINT('Ctrl Pts',(-21.4716714037525,6.4867077908221,-7.57344697283478));
#52010=CARTESIAN_POINT('Ctrl Pts',(-21.4424150110734,6.48242277983716,-7.53858520564487));
#52011=CARTESIAN_POINT('Ctrl Pts',(-21.2909879716434,6.46633279908612,-7.35239822189483));
#52012=CARTESIAN_POINT('Ctrl Pts',(-21.1630186724938,6.47273402762071,-7.17554799773058));
#52013=CARTESIAN_POINT('Ctrl Pts',(-21.,6.43881576337965,-6.98510211559241));
#52014=CARTESIAN_POINT('Origin',(-50.,0.,0.));
#52015=CARTESIAN_POINT('',(-50.,6.03932124977422,-3.89701874412038));
#52016=CARTESIAN_POINT('Origin',(-50.,0.,0.));
#52017=CARTESIAN_POINT('',(-50.,6.03932124977422,-3.89701874412038));
#52018=CARTESIAN_POINT('Ctrl Pts',(-50.,9.57942322326164,-4.53813295416029));
#52019=CARTESIAN_POINT('Ctrl Pts',(-21.,9.57942322326164,-4.53813295416029));
#52020=CARTESIAN_POINT('Ctrl Pts',(-50.,9.55621969972587,-4.54379106380403));
#52021=CARTESIAN_POINT('Ctrl Pts',(-21.,9.55621969972587,-4.54379106380403));
#52022=CARTESIAN_POINT('Ctrl Pts',(-50.,9.50983973295391,-4.55488811868959));
#52023=CARTESIAN_POINT('Ctrl Pts',(-21.,9.50983973295391,-4.55488811868959));
#52024=CARTESIAN_POINT('Ctrl Pts',(-50.,9.44035102435851,-4.57087620725774));
#52025=CARTESIAN_POINT('Ctrl Pts',(-21.,9.44035102435851,-4.57087620725774));
#52026=CARTESIAN_POINT('Ctrl Pts',(-50.,9.34786210629442,-4.59087692729648));
#52027=CARTESIAN_POINT('Ctrl Pts',(-21.,9.34786210629442,-4.59087692729648));
#52028=CARTESIAN_POINT('Ctrl Pts',(-50.,9.23252715927802,-4.61366883031981));
#52029=CARTESIAN_POINT('Ctrl Pts',(-21.,9.23252715927802,-4.61366883031981));
#52030=CARTESIAN_POINT('Ctrl Pts',(-50.,9.11748127106242,-4.63422615215906));
#52031=CARTESIAN_POINT('Ctrl Pts',(-21.,9.11748127106242,-4.63422615215906));
#52032=CARTESIAN_POINT('Ctrl Pts',(-50.,9.00274873347492,-4.65251093331389));
#52033=CARTESIAN_POINT('Ctrl Pts',(-21.,9.00274873347492,-4.65251093331389));
#52034=CARTESIAN_POINT('Ctrl Pts',(-50.,8.8883682032848,-4.66847246002033));
#52035=CARTESIAN_POINT('Ctrl Pts',(-21.,8.8883682032848,-4.66847246002033));
#52036=CARTESIAN_POINT('Ctrl Pts',(-50.,8.7743974532252,-4.68204521487955));
#52037=CARTESIAN_POINT('Ctrl Pts',(-21.,8.7743974532252,-4.68204521487955));
#52038=CARTESIAN_POINT('Ctrl Pts',(-50.,8.66090712613407,-4.69315791678054));
#52039=CARTESIAN_POINT('Ctrl Pts',(-21.,8.66090712613407,-4.69315791678054));
#52040=CARTESIAN_POINT('Ctrl Pts',(-50.,8.5479718655136,-4.70174502276072));
#52041=CARTESIAN_POINT('Ctrl Pts',(-21.,8.5479718655136,-4.70174502276072));
#52042=CARTESIAN_POINT('Ctrl Pts',(-50.,8.4356616058832,-4.70775898013052));
#52043=CARTESIAN_POINT('Ctrl Pts',(-21.,8.4356616058832,-4.70775898013052));
#52044=CARTESIAN_POINT('Ctrl Pts',(-50.,8.32403430863484,-4.71117963661127));
#52045=CARTESIAN_POINT('Ctrl Pts',(-21.,8.32403430863484,-4.71117963661127));
#52046=CARTESIAN_POINT('Ctrl Pts',(-50.,8.21312397255121,-4.71203258951797));
#52047=CARTESIAN_POINT('Ctrl Pts',(-21.,8.21312397255121,-4.71203258951797));
#52048=CARTESIAN_POINT('Ctrl Pts',(-50.,8.1029496259928,-4.71036931800664));
#52049=CARTESIAN_POINT('Ctrl Pts',(-21.,8.1029496259928,-4.71036931800664));
#52050=CARTESIAN_POINT('Ctrl Pts',(-50.,7.99353571494822,-4.70622700687469));
#52051=CARTESIAN_POINT('Ctrl Pts',(-21.,7.99353571494822,-4.70622700687469));
#52052=CARTESIAN_POINT('Ctrl Pts',(-50.,7.8849298684541,-4.69959254734285));
#52053=CARTESIAN_POINT('Ctrl Pts',(-21.,7.8849298684541,-4.69959254734285));
#52054=CARTESIAN_POINT('Ctrl Pts',(-50.,7.77721964274024,-4.69037000103626));
#52055=CARTESIAN_POINT('Ctrl Pts',(-21.,7.77721964274024,-4.69037000103626));
#52056=CARTESIAN_POINT('Ctrl Pts',(-50.,7.6705550660185,-4.67833376211481));
#52057=CARTESIAN_POINT('Ctrl Pts',(-21.,7.6705550660185,-4.67833376211481));
#52058=CARTESIAN_POINT('Ctrl Pts',(-50.,7.56514580946327,-4.66314297047291));
#52059=CARTESIAN_POINT('Ctrl Pts',(-21.,7.56514580946327,-4.66314297047291));
#52060=CARTESIAN_POINT('Ctrl Pts',(-50.,7.46123890856565,-4.64440143603747));
#52061=CARTESIAN_POINT('Ctrl Pts',(-21.,7.46123890856565,-4.64440143603747));
#52062=CARTESIAN_POINT('Ctrl Pts',(-50.,7.35910284385827,-4.62170482170181));
#52063=CARTESIAN_POINT('Ctrl Pts',(-21.,7.35910284385827,-4.62170482170181));
#52064=CARTESIAN_POINT('Ctrl Pts',(-50.,7.25900770064673,-4.59469206087561));
#52065=CARTESIAN_POINT('Ctrl Pts',(-21.,7.25900770064673,-4.59469206087561));
#52066=CARTESIAN_POINT('Ctrl Pts',(-50.,7.16121001331941,-4.56309881747208));
#52067=CARTESIAN_POINT('Ctrl Pts',(-21.,7.16121001331941,-4.56309881747208));
#52068=CARTESIAN_POINT('Ctrl Pts',(-50.,7.06592138953324,-4.5267956450212));
#52069=CARTESIAN_POINT('Ctrl Pts',(-21.,7.06592138953324,-4.5267956450212));
#52070=CARTESIAN_POINT('Ctrl Pts',(-50.,6.9732685530375,-4.48581308997575));
#52071=CARTESIAN_POINT('Ctrl Pts',(-21.,6.9732685530375,-4.48581308997575));
#52072=CARTESIAN_POINT('Ctrl Pts',(-50.,6.88325224876452,-4.44037556328962));
#52073=CARTESIAN_POINT('Ctrl Pts',(-21.,6.88325224876452,-4.44037556328962));
#52074=CARTESIAN_POINT('Ctrl Pts',(-50.,6.79571235355295,-4.39092540044368));
#52075=CARTESIAN_POINT('Ctrl Pts',(-21.,6.79571235355295,-4.39092540044368));
#52076=CARTESIAN_POINT('Ctrl Pts',(-50.,6.71027219290963,-4.33817259947066));
#52077=CARTESIAN_POINT('Ctrl Pts',(-21.,6.71027219290963,-4.33817259947066));
#52078=CARTESIAN_POINT('Ctrl Pts',(-50.,6.62638951409907,-4.28302021638686));
#52079=CARTESIAN_POINT('Ctrl Pts',(-21.,6.62638951409907,-4.28302021638686));
#52080=CARTESIAN_POINT('Ctrl Pts',(-50.,6.54344708143028,-4.22644426515767));
#52081=CARTESIAN_POINT('Ctrl Pts',(-21.,6.54344708143028,-4.22644426515767));
#52082=CARTESIAN_POINT('Ctrl Pts',(-50.,6.46083145580807,-4.1693867325325));
#52083=CARTESIAN_POINT('Ctrl Pts',(-21.,6.46083145580807,-4.1693867325325));
#52084=CARTESIAN_POINT('Ctrl Pts',(-50.,6.37801243240243,-4.11264895980536));
#52085=CARTESIAN_POINT('Ctrl Pts',(-21.,6.37801243240243,-4.11264895980536));
#52086=CARTESIAN_POINT('Ctrl Pts',(-50.,6.29463308326085,-4.05676946424956));
#52087=CARTESIAN_POINT('Ctrl Pts',(-21.,6.29463308326085,-4.05676946424956));
#52088=CARTESIAN_POINT('Ctrl Pts',(-50.,6.21048516503746,-4.00206265639536));
#52089=CARTESIAN_POINT('Ctrl Pts',(-21.,6.21048516503746,-4.00206265639536));
#52090=CARTESIAN_POINT('Ctrl Pts',(-50.,6.14247034880463,-3.95935849016754));
#52091=CARTESIAN_POINT('Ctrl Pts',(-21.,6.14247034880463,-3.95935849016754));
#52092=CARTESIAN_POINT('Ctrl Pts',(-50.,6.09105342163039,-3.92794852152395));
#52093=CARTESIAN_POINT('Ctrl Pts',(-21.,6.09105342163039,-3.92794852152395));
#52094=CARTESIAN_POINT('Ctrl Pts',(-50.,6.0565953297729,-3.90728293824429));
#52095=CARTESIAN_POINT('Ctrl Pts',(-21.,6.0565953297729,-3.90728293824429));
#52096=CARTESIAN_POINT('Ctrl Pts',(-50.,6.03932124977421,-3.89701874412039));
#52097=CARTESIAN_POINT('Ctrl Pts',(-21.,6.03932124977421,-3.89701874412039));
#52098=CARTESIAN_POINT('',(-21.5,8.84053003053573,-4.67386657695702));
#52099=CARTESIAN_POINT('',(-50.,8.84053003053573,-4.67386657695701));
#52100=CARTESIAN_POINT('Ctrl Pts',(-21.5,8.84053003053573,-4.67386657695702));
#52101=CARTESIAN_POINT('Ctrl Pts',(-26.3333333333333,8.84053003053573,-4.67386657695702));
#52102=CARTESIAN_POINT('Ctrl Pts',(-31.1666666666667,8.84053003053573,-4.67386657695702));
#52103=CARTESIAN_POINT('Ctrl Pts',(-40.6666666666667,8.84053003053573,-4.67386657695702));
#52104=CARTESIAN_POINT('Ctrl Pts',(-45.3333333333333,8.84053003053573,-4.67386657695702));
#52105=CARTESIAN_POINT('Ctrl Pts',(-50.,8.84053003053573,-4.67386657695702));
#52106=CARTESIAN_POINT('Ctrl Pts',(-21.,8.24940658621528,-4.71140010775012));
#52107=CARTESIAN_POINT('Ctrl Pts',(-21.1171767611032,8.38464171183386,-4.71088427266306));
#52108=CARTESIAN_POINT('Ctrl Pts',(-21.2874825276494,8.58376433439636,-4.70484095794145));
#52109=CARTESIAN_POINT('Ctrl Pts',(-21.5,8.84053003053573,-4.67386657695702));
#52110=CARTESIAN_POINT('Ctrl Pts',(-50.,6.03932124977421,-3.89701874412039));
#52111=CARTESIAN_POINT('Ctrl Pts',(-50.,6.0565953297729,-3.90728293824429));
#52112=CARTESIAN_POINT('Ctrl Pts',(-50.,6.09105342163039,-3.92794852152395));
#52113=CARTESIAN_POINT('Ctrl Pts',(-50.,6.14247034880463,-3.95935849016754));
#52114=CARTESIAN_POINT('Ctrl Pts',(-50.,6.21048516503746,-4.00206265639536));
#52115=CARTESIAN_POINT('Ctrl Pts',(-50.,6.29463308326085,-4.05676946424956));
#52116=CARTESIAN_POINT('Ctrl Pts',(-50.,6.37801243240243,-4.11264895980536));
#52117=CARTESIAN_POINT('Ctrl Pts',(-50.,6.46083145580807,-4.1693867325325));
#52118=CARTESIAN_POINT('Ctrl Pts',(-50.,6.54344708143028,-4.22644426515767));
#52119=CARTESIAN_POINT('Ctrl Pts',(-50.,6.62638951409907,-4.28302021638686));
#52120=CARTESIAN_POINT('Ctrl Pts',(-50.,6.71027219290963,-4.33817259947066));
#52121=CARTESIAN_POINT('Ctrl Pts',(-50.,6.79571235355295,-4.39092540044368));
#52122=CARTESIAN_POINT('Ctrl Pts',(-50.,6.88325224876452,-4.44037556328962));
#52123=CARTESIAN_POINT('Ctrl Pts',(-50.,6.9732685530375,-4.48581308997575));
#52124=CARTESIAN_POINT('Ctrl Pts',(-50.,7.06592138953324,-4.5267956450212));
#52125=CARTESIAN_POINT('Ctrl Pts',(-50.,7.16121001331941,-4.56309881747208));
#52126=CARTESIAN_POINT('Ctrl Pts',(-50.,7.25900770064673,-4.59469206087561));
#52127=CARTESIAN_POINT('Ctrl Pts',(-50.,7.35910284385827,-4.62170482170181));
#52128=CARTESIAN_POINT('Ctrl Pts',(-50.,7.46123890856565,-4.64440143603747));
#52129=CARTESIAN_POINT('Ctrl Pts',(-50.,7.56514580946327,-4.66314297047291));
#52130=CARTESIAN_POINT('Ctrl Pts',(-50.,7.6705550660185,-4.67833376211481));
#52131=CARTESIAN_POINT('Ctrl Pts',(-50.,7.77721964274024,-4.69037000103626));
#52132=CARTESIAN_POINT('Ctrl Pts',(-50.,7.8849298684541,-4.69959254734285));
#52133=CARTESIAN_POINT('Ctrl Pts',(-50.,7.99353571494822,-4.70622700687469));
#52134=CARTESIAN_POINT('Ctrl Pts',(-50.,8.1029496259928,-4.71036931800664));
#52135=CARTESIAN_POINT('Ctrl Pts',(-50.,8.21312397255121,-4.71203258951797));
#52136=CARTESIAN_POINT('Ctrl Pts',(-50.,8.32403430863484,-4.71117963661127));
#52137=CARTESIAN_POINT('Ctrl Pts',(-50.,8.4356616058832,-4.70775898013052));
#52138=CARTESIAN_POINT('Ctrl Pts',(-50.,8.5479718655136,-4.70174502276072));
#52139=CARTESIAN_POINT('Ctrl Pts',(-50.,8.65141534429653,-4.69387963058482));
#52140=CARTESIAN_POINT('Ctrl Pts',(-50.,8.73262742272914,-4.68611341617549));
#52141=CARTESIAN_POINT('Ctrl Pts',(-50.,8.79131644357128,-4.67969501220182));
#52142=CARTESIAN_POINT('Ctrl Pts',(-50.,8.82731230052618,-4.67546106956729));
#52143=CARTESIAN_POINT('Ctrl Pts',(-50.,8.84053003053573,-4.67386657695701));
#52144=CARTESIAN_POINT('Origin',(-50.,10.,0.));
#52145=CARTESIAN_POINT('',(-50.,14.0217614511585,-1.06963173887292));
#52146=CARTESIAN_POINT('',(-50.,16.3612159786808,-0.671741541784792));
#52147=CARTESIAN_POINT('Ctrl Pts',(-50.,14.0217614511585,-1.06963173887291));
#52148=CARTESIAN_POINT('Ctrl Pts',(-50.,14.0415811730659,-1.0717527195609));
#52149=CARTESIAN_POINT('Ctrl Pts',(-50.,14.0812352370361,-1.07587965991017));
#52150=CARTESIAN_POINT('Ctrl Pts',(-50.,14.1407601934611,-1.08172501415579));
#52151=CARTESIAN_POINT('Ctrl Pts',(-50.,14.2202146396052,-1.08882773106131));
#52152=CARTESIAN_POINT('Ctrl Pts',(-50.,14.3196790995356,-1.09650878711472));
#52153=CARTESIAN_POINT('Ctrl Pts',(-50.,14.4192887981899,-1.10286394535002));
#52154=CARTESIAN_POINT('Ctrl Pts',(-50.,14.5190405063557,-1.10764458318629));
#52155=CARTESIAN_POINT('Ctrl Pts',(-50.,14.6189280002071,-1.11043751754959));
#52156=CARTESIAN_POINT('Ctrl Pts',(-50.,14.7189411465911,-1.11063958426619));
#52157=CARTESIAN_POINT('Ctrl Pts',(-50.,14.8190654065121,-1.10759084369408));
#52158=CARTESIAN_POINT('Ctrl Pts',(-50.,14.9192812134642,-1.100697501046));
#52159=CARTESIAN_POINT('Ctrl Pts',(-50.,15.0195634762927,-1.08955145679141));
#52160=CARTESIAN_POINT('Ctrl Pts',(-50.,15.1198807137451,-1.07407094658941));
#52161=CARTESIAN_POINT('Ctrl Pts',(-50.,15.2201951366894,-1.05457808085916));
#52162=CARTESIAN_POINT('Ctrl Pts',(-50.,15.3204663197849,-1.03163045186508));
#52163=CARTESIAN_POINT('Ctrl Pts',(-50.,15.42065441025,-1.00588830882699));
#52164=CARTESIAN_POINT('Ctrl Pts',(-50.,15.5207233107191,-0.977976807855906));
#52165=CARTESIAN_POINT('Ctrl Pts',(-50.,15.6206443917204,-0.948332278883351));
#52166=CARTESIAN_POINT('Ctrl Pts',(-50.,15.7203984586304,-0.917113393337539));
#52167=CARTESIAN_POINT('Ctrl Pts',(-50.,15.8199726227578,-0.884304144422378));
#52168=CARTESIAN_POINT('Ctrl Pts',(-50.,15.9193580975472,-0.849783012021725));
#52169=CARTESIAN_POINT('Ctrl Pts',(-50.,16.018547775909,-0.813401076758624));
#52170=CARTESIAN_POINT('Ctrl Pts',(-50.,16.1175336986507,-0.775065535573949));
#52171=CARTESIAN_POINT('Ctrl Pts',(-50.,16.2058743852262,-0.739044856835963));
#52172=CARTESIAN_POINT('Ctrl Pts',(-50.,16.2743241898497,-0.709958710092983));
#52173=CARTESIAN_POINT('Ctrl Pts',(-50.,16.322986318803,-0.688711885022031));
#52174=CARTESIAN_POINT('Ctrl Pts',(-50.,16.3519363129391,-0.675875939350104));
#52175=CARTESIAN_POINT('Ctrl Pts',(-50.,16.3612159786808,-0.671741541784792));
#52176=CARTESIAN_POINT('',(-50.,16.3606547098013,0.685275467717997));
#52177=CARTESIAN_POINT('Origin',(-50.,0.,0.));
#52178=CARTESIAN_POINT('',(-50.,14.0217614511585,1.06963173887291));
#52179=CARTESIAN_POINT('Ctrl Pts',(-50.,16.3606547098013,0.685275467717997));
#52180=CARTESIAN_POINT('Ctrl Pts',(-50.,16.3602361479617,0.685486203406702));
#52181=CARTESIAN_POINT('Ctrl Pts',(-50.,16.3363770939854,0.697487024394078));
#52182=CARTESIAN_POINT('Ctrl Pts',(-50.,16.2893303613477,0.719836826943709));
#52183=CARTESIAN_POINT('Ctrl Pts',(-50.,16.2196908113235,0.749093040322084));
#52184=CARTESIAN_POINT('Ctrl Pts',(-50.,16.1280496341459,0.78121969830999));
#52185=CARTESIAN_POINT('Ctrl Pts',(-50.,16.014323697387,0.815965624774873));
#52186=CARTESIAN_POINT('Ctrl Pts',(-50.,15.8995555551237,0.851197548491309));
#52187=CARTESIAN_POINT('Ctrl Pts',(-50.,15.7832573706013,0.889179733744299));
#52188=CARTESIAN_POINT('Ctrl Pts',(-50.,15.6656677858244,0.929213220852553));
#52189=CARTESIAN_POINT('Ctrl Pts',(-50.,15.5473762906989,0.969035923607179));
#52190=CARTESIAN_POINT('Ctrl Pts',(-50.,15.4290559476364,1.00581543437186));
#52191=CARTESIAN_POINT('Ctrl Pts',(-50.,15.3110884135537,1.03751150535353));
#52192=CARTESIAN_POINT('Ctrl Pts',(-50.,15.1935004613832,1.06322736266735));
#52193=CARTESIAN_POINT('Ctrl Pts',(-50.,15.0761445357738,1.08279356247792));
#52194=CARTESIAN_POINT('Ctrl Pts',(-50.,14.9588014916819,1.09658017916666));
#52195=CARTESIAN_POINT('Ctrl Pts',(-50.,14.8413329590673,1.10520035673609));
#52196=CARTESIAN_POINT('Ctrl Pts',(-50.,14.7237519921366,1.10932591245462));
#52197=CARTESIAN_POINT('Ctrl Pts',(-50.,14.6061528843942,1.10963588316888));
#52198=CARTESIAN_POINT('Ctrl Pts',(-50.,14.4886712704316,1.10674391788617));
#52199=CARTESIAN_POINT('Ctrl Pts',(-50.,14.3714293939101,1.1011284935459));
#52200=CARTESIAN_POINT('Ctrl Pts',(-50.,14.2544968327758,1.09307823697967));
#52201=CARTESIAN_POINT('Ctrl Pts',(-50.,14.1612257648809,1.08481225073396));
#52202=CARTESIAN_POINT('Ctrl Pts',(-50.,14.0914317375174,1.07761101544474));
#52203=CARTESIAN_POINT('Ctrl Pts',(-50.,14.0449730955977,1.07236559806543));
#52204=CARTESIAN_POINT('Ctrl Pts',(-50.,14.0217614511585,1.06963173887291));
#52205=CARTESIAN_POINT('',(-50.,13.847248627403,2.45104298226008));
#52206=CARTESIAN_POINT('Origin',(-50.,0.,0.));
#52207=CARTESIAN_POINT('',(-50.,16.0142536207693,3.41823140961461));
#52208=CARTESIAN_POINT('Ctrl Pts',(-50.,13.847248627403,2.45104298226009));
#52209=CARTESIAN_POINT('Ctrl Pts',(-50.,13.8669731427486,2.45391760048539));
#52210=CARTESIAN_POINT('Ctrl Pts',(-50.,13.9064077297103,2.45978188025048));
#52211=CARTESIAN_POINT('Ctrl Pts',(-50.,13.9655162806582,2.46892342325417));
#52212=CARTESIAN_POINT('Ctrl Pts',(-50.,14.0442408931361,2.48180336850756));
#52213=CARTESIAN_POINT('Ctrl Pts',(-50.,14.1424906951186,2.49909943227153));
#52214=CARTESIAN_POINT('Ctrl Pts',(-50.,14.2405514355047,2.51771585773738));
#52215=CARTESIAN_POINT('Ctrl Pts',(-50.,14.338358156612,2.53789265347798));
#52216=CARTESIAN_POINT('Ctrl Pts',(-50.,14.4358020756955,2.56002847385863));
#52217=CARTESIAN_POINT('Ctrl Pts',(-50.,14.5327233771235,2.58470501352874));
#52218=CARTESIAN_POINT('Ctrl Pts',(-50.,14.6289438583545,2.61255786321175));
#52219=CARTESIAN_POINT('Ctrl Pts',(-50.,14.7242968968419,2.64415729654763));
#52220=CARTESIAN_POINT('Ctrl Pts',(-50.,14.8186566994895,2.67989235195328));
#52221=CARTESIAN_POINT('Ctrl Pts',(-50.,14.9119724401214,2.71983439592332));
#52222=CARTESIAN_POINT('Ctrl Pts',(-50.,15.0042876224246,2.76366203995482));
#52223=CARTESIAN_POINT('Ctrl Pts',(-50.,15.0957017586521,2.81082515619622));
#52224=CARTESIAN_POINT('Ctrl Pts',(-50.,15.1863404453747,2.86067432738731));
#52225=CARTESIAN_POINT('Ctrl Pts',(-50.,15.2763241892947,2.9125950607961));
#52226=CARTESIAN_POINT('Ctrl Pts',(-50.,15.3657337712291,2.96615761473811));
#52227=CARTESIAN_POINT('Ctrl Pts',(-50.,15.4545900595684,3.02120352923108));
#52228=CARTESIAN_POINT('Ctrl Pts',(-50.,15.542876589815,3.07774510290095));
#52229=CARTESIAN_POINT('Ctrl Pts',(-50.,15.6305546306352,3.13589785295852));
#52230=CARTESIAN_POINT('Ctrl Pts',(-50.,15.7175802634788,3.19580425274334));
#52231=CARTESIAN_POINT('Ctrl Pts',(-50.,15.8039227000236,3.2575522103651));
#52232=CARTESIAN_POINT('Ctrl Pts',(-50.,15.8805300229522,3.31441066861968));
#52233=CARTESIAN_POINT('Ctrl Pts',(-50.,15.9395959205415,3.35960579476531));
#52234=CARTESIAN_POINT('Ctrl Pts',(-50.,15.9814453687008,3.39228689111509));
#52235=CARTESIAN_POINT('Ctrl Pts',(-50.,16.0062936756551,3.41191914272521));
#52236=CARTESIAN_POINT('Ctrl Pts',(-50.,16.0142536207693,3.41823140961461));
#52237=CARTESIAN_POINT('',(-50.,15.6762335782097,4.73247565248984));
#52238=CARTESIAN_POINT('Origin',(-50.,0.,0.));
#52239=CARTESIAN_POINT('',(-50.,13.3152354345065,4.52309756402217));
#52240=CARTESIAN_POINT('Ctrl Pts',(-50.,15.6762335782097,4.73247565248984));
#52241=CARTESIAN_POINT('Ctrl Pts',(-50.,15.6757757584253,4.73257567543269));
#52242=CARTESIAN_POINT('Ctrl Pts',(-50.,15.6496817976862,4.73826596311956));
#52243=CARTESIAN_POINT('Ctrl Pts',(-50.,15.598554954793,4.74821355889253));
#52244=CARTESIAN_POINT('Ctrl Pts',(-50.,15.5238275348871,4.7592319826915));
#52245=CARTESIAN_POINT('Ctrl Pts',(-50.,15.4270758588568,4.76755908862997));
#52246=CARTESIAN_POINT('Ctrl Pts',(-50.,15.3082818709966,4.77293091754137));
#52247=CARTESIAN_POINT('Ctrl Pts',(-50.,15.1883575578327,4.77851428923771));
#52248=CARTESIAN_POINT('Ctrl Pts',(-50.,15.0662673092696,4.78638101191027));
#52249=CARTESIAN_POINT('Ctrl Pts',(-50.,14.9424160941388,4.79591343283465));
#52250=CARTESIAN_POINT('Ctrl Pts',(-50.,14.8179374404009,4.80506713357809));
#52251=CARTESIAN_POINT('Ctrl Pts',(-50.,14.6941876561096,4.81126607561379));
#52252=CARTESIAN_POINT('Ctrl Pts',(-50.,14.5720437967212,4.81262902350044));
#52253=CARTESIAN_POINT('Ctrl Pts',(-50.,14.4517548126435,4.80829403531135));
#52254=CARTESIAN_POINT('Ctrl Pts',(-50.,14.3332199232164,4.79806029507722));
#52255=CARTESIAN_POINT('Ctrl Pts',(-50.,14.2161348344847,4.78223175145606));
#52256=CARTESIAN_POINT('Ctrl Pts',(-50.,14.1002130408447,4.76136787417443));
#52257=CARTESIAN_POINT('Ctrl Pts',(-50.,13.9853001122203,4.73612262057495));
#52258=CARTESIAN_POINT('Ctrl Pts',(-50.,13.8713185101153,4.70717714415409));
#52259=CARTESIAN_POINT('Ctrl Pts',(-50.,13.7582469996088,4.67515954595839));
#52260=CARTESIAN_POINT('Ctrl Pts',(-50.,13.6460849914764,4.64056367145667));
#52261=CARTESIAN_POINT('Ctrl Pts',(-50.,13.5348280991712,4.60368638306948));
#52262=CARTESIAN_POINT('Ctrl Pts',(-50.,13.4465429805744,4.57248451663122));
#52263=CARTESIAN_POINT('Ctrl Pts',(-50.,13.3807325353144,4.54815245260096));
#52264=CARTESIAN_POINT('Ctrl Pts',(-50.,13.3370379593182,4.53151803523741));
#52265=CARTESIAN_POINT('Ctrl Pts',(-50.,13.3152354345065,4.52309756402217));
#52266=CARTESIAN_POINT('',(-50.,12.8026622457696,5.81770965851215));
#52267=CARTESIAN_POINT('Origin',(-50.,0.,0.));
#52268=CARTESIAN_POINT('',(-50.,14.66105681156,7.29342431017219));
#52269=CARTESIAN_POINT('Ctrl Pts',(-50.,12.8026622457696,5.81770965851216));
#52270=CARTESIAN_POINT('Ctrl Pts',(-50.,12.8210521907127,5.82539925281556));
#52271=CARTESIAN_POINT('Ctrl Pts',(-50.,12.8577894805368,5.84088627843006));
#52272=CARTESIAN_POINT('Ctrl Pts',(-50.,12.9127676183656,5.86444032191588));
#52273=CARTESIAN_POINT('Ctrl Pts',(-50.,12.9858158402462,5.89649363499879));
#52274=CARTESIAN_POINT('Ctrl Pts',(-50.,13.0766775878848,5.93768004328337));
#52275=CARTESIAN_POINT('Ctrl Pts',(-50.,13.1670278530422,5.98009831397194));
#52276=CARTESIAN_POINT('Ctrl Pts',(-50.,13.2567440310958,6.02396476100794));
#52277=CARTESIAN_POINT('Ctrl Pts',(-50.,13.3456216156017,6.06963846112818));
#52278=CARTESIAN_POINT('Ctrl Pts',(-50.,13.4333611502533,6.11764308944358));
#52279=CARTESIAN_POINT('Ctrl Pts',(-50.,13.5196319660845,6.16854995125629));
#52280=CARTESIAN_POINT('Ctrl Pts',(-50.,13.6041308540151,6.22286996666888));
#52281=CARTESIAN_POINT('Ctrl Pts',(-50.,13.6866392230503,6.28094866827011));
#52282=CARTESIAN_POINT('Ctrl Pts',(-50.,13.7670900956865,6.342842540489));
#52283=CARTESIAN_POINT('Ctrl Pts',(-50.,13.845605534933,6.40825111076043));
#52284=CARTESIAN_POINT('Ctrl Pts',(-50.,13.9224187379158,6.47666628220192));
#52285=CARTESIAN_POINT('Ctrl Pts',(-50.,13.9978128588633,6.54749027478764));
#52286=CARTESIAN_POINT('Ctrl Pts',(-50.,14.0720574366665,6.62015787000295));
#52287=CARTESIAN_POINT('Ctrl Pts',(-50.,14.1453375866756,6.69427291666095));
#52288=CARTESIAN_POINT('Ctrl Pts',(-50.,14.2177129290574,6.76968712284877));
#52289=CARTESIAN_POINT('Ctrl Pts',(-50.,14.2891644580326,6.84640830625432));
#52290=CARTESIAN_POINT('Ctrl Pts',(-50.,14.3596259311217,6.92453872281182));
#52291=CARTESIAN_POINT('Ctrl Pts',(-50.,14.4290193778776,7.00420544769957));
#52292=CARTESIAN_POINT('Ctrl Pts',(-50.,14.497293115392,7.08548597048793));
#52293=CARTESIAN_POINT('Ctrl Pts',(-50.,14.5573535548322,7.15960958221619));
#52294=CARTESIAN_POINT('Ctrl Pts',(-50.,14.6033242178125,7.21807391177268));
#52295=CARTESIAN_POINT('Ctrl Pts',(-50.,14.6357314304385,7.26013580592497));
#52296=CARTESIAN_POINT('Ctrl Pts',(-50.,14.6549167396993,7.28533079690226));
#52297=CARTESIAN_POINT('Ctrl Pts',(-50.,14.66105681156,7.29342431017219));
#52298=CARTESIAN_POINT('',(-50.,14.0068170377451,8.48231698718778));
#52299=CARTESIAN_POINT('Origin',(-50.,0.,0.));
#52300=CARTESIAN_POINT('',(-50.,11.7720642054939,7.69236053443469));
#52301=CARTESIAN_POINT('Ctrl Pts',(-50.,14.0068170377451,8.48231698718778));
#52302=CARTESIAN_POINT('Ctrl Pts',(-50.,14.0063487265167,8.48230001257543));
#52303=CARTESIAN_POINT('Ctrl Pts',(-50.,13.9796594385348,8.481322225259));
#52304=CARTESIAN_POINT('Ctrl Pts',(-50.,13.9276649729564,8.47824257022821));
#52305=CARTESIAN_POINT('Ctrl Pts',(-50.,13.8525450817897,8.47033087635756));
#52306=CARTESIAN_POINT('Ctrl Pts',(-50.,13.7567621705396,8.45433520755552));
#52307=CARTESIAN_POINT('Ctrl Pts',(-50.,13.640364394729,8.42999540714673));
#52308=CARTESIAN_POINT('Ctrl Pts',(-50.,13.5228191963114,8.40557940304509));
#52309=CARTESIAN_POINT('Ctrl Pts',(-50.,13.4026082630414,8.38283636801991));
#52310=CARTESIAN_POINT('Ctrl Pts',(-50.,13.2802774448963,8.36126876569594));
#52311=CARTESIAN_POINT('Ctrl Pts',(-50.,13.1574330841607,8.33917830374554));
#52312=CARTESIAN_POINT('Ctrl Pts',(-50.,13.0360295127074,8.31440717472604));
#52313=CARTESIAN_POINT('Ctrl Pts',(-50.,12.9173840759125,8.28535136048938));
#52314=CARTESIAN_POINT('Ctrl Pts',(-50.,12.8019522591891,8.25123791004828));
#52315=CARTESIAN_POINT('Ctrl Pts',(-50.,12.6896863889879,8.21184725330542));
#52316=CARTESIAN_POINT('Ctrl Pts',(-50.,12.5802161423503,8.16739811498339));
#52317=CARTESIAN_POINT('Ctrl Pts',(-50.,12.4731248803097,8.11836113699226));
#52318=CARTESIAN_POINT('Ctrl Pts',(-50.,12.3681003919172,8.06533132620399));
#52319=CARTESIAN_POINT('Ctrl Pts',(-50.,12.2648981787049,8.00894915338555));
#52320=CARTESIAN_POINT('Ctrl Pts',(-50.,12.1633414705075,7.94981770572398));
#52321=CARTESIAN_POINT('Ctrl Pts',(-50.,12.0633068822383,7.88841516709048));
#52322=CARTESIAN_POINT('Ctrl Pts',(-50.,11.96471633848,7.82502798253687));
#52323=CARTESIAN_POINT('Ctrl Pts',(-50.,11.8869644478727,7.77285076392682));
#52324=CARTESIAN_POINT('Ctrl Pts',(-50.,11.8292726970256,7.73291674422561));
#52325=CARTESIAN_POINT('Ctrl Pts',(-50.,11.7910876778603,7.70593852849788));
#52326=CARTESIAN_POINT('Ctrl Pts',(-50.,11.7720642054939,7.69236053443469));
#52327=CARTESIAN_POINT('',(-50.,10.9536375103364,8.81882824088046));
#52328=CARTESIAN_POINT('Origin',(-50.,0.,0.));
#52329=CARTESIAN_POINT('',(-50.,12.3866518832851,10.7103445379834));
#52330=CARTESIAN_POINT('Ctrl Pts',(-50.,10.9536375103364,8.81882824088047));
#52331=CARTESIAN_POINT('Ctrl Pts',(-50.,10.9695373770028,8.83084964577152));
#52332=CARTESIAN_POINT('Ctrl Pts',(-50.,11.0012690306593,8.85498631045878));
#52333=CARTESIAN_POINT('Ctrl Pts',(-50.,11.0486622767737,8.89147286724882));
#52334=CARTESIAN_POINT('Ctrl Pts',(-50.,11.1114442196238,8.9406855206164));
#52335=CARTESIAN_POINT('Ctrl Pts',(-50.,11.1892087351483,9.00317437991606));
#52336=CARTESIAN_POINT('Ctrl Pts',(-50.,11.2661714856319,9.06672919987649));
#52337=CARTESIAN_POINT('Ctrl Pts',(-50.,11.3421599232118,9.13152900801114));
#52338=CARTESIAN_POINT('Ctrl Pts',(-50.,11.4168866676366,9.19787074131628));
#52339=CARTESIAN_POINT('Ctrl Pts',(-50.,11.4899314378663,9.26618715093123));
#52340=CARTESIAN_POINT('Ctrl Pts',(-50.,11.5608318756571,9.3369493595236));
#52341=CARTESIAN_POINT('Ctrl Pts',(-50.,11.629167237137,9.41057683066949));
#52342=CARTESIAN_POINT('Ctrl Pts',(-50.,11.6946398682888,9.48734988004618));
#52343=CARTESIAN_POINT('Ctrl Pts',(-50.,11.7571708487241,9.56730656089267));
#52344=CARTESIAN_POINT('Ctrl Pts',(-50.,11.8169531311064,9.65018619637799));
#52345=CARTESIAN_POINT('Ctrl Pts',(-50.,11.8743389448017,9.73555464618448));
#52346=CARTESIAN_POINT('Ctrl Pts',(-50.,11.9297512100749,9.82290332823825));
#52347=CARTESIAN_POINT('Ctrl Pts',(-50.,11.9835915618855,9.91175181299999));
#52348=CARTESIAN_POINT('Ctrl Pts',(-50.,12.0361378186387,10.0017624314164));
#52349=CARTESIAN_POINT('Ctrl Pts',(-50.,12.0874846061232,10.0928063773702));
#52350=CARTESIAN_POINT('Ctrl Pts',(-50.,12.1376115714812,10.1848864963973));
#52351=CARTESIAN_POINT('Ctrl Pts',(-50.,12.1864291233458,10.2780853580389));
#52352=CARTESIAN_POINT('Ctrl Pts',(-50.,12.2338301385431,10.3725066547111));
#52353=CARTESIAN_POINT('Ctrl Pts',(-50.,12.2797452870059,10.4682125884904));
#52354=CARTESIAN_POINT('Ctrl Pts',(-50.,12.3194850246607,10.5549438945599));
#52355=CARTESIAN_POINT('Ctrl Pts',(-50.,12.3494719472088,10.6230038986845));
#52356=CARTESIAN_POINT('Ctrl Pts',(-50.,12.3704006599468,10.6718036871368));
#52357=CARTESIAN_POINT('Ctrl Pts',(-50.,12.3827174879745,10.7009783235375));
#52358=CARTESIAN_POINT('Ctrl Pts',(-50.,12.3866518832851,10.7103445379834));
#52359=CARTESIAN_POINT('',(-50.,11.4573006693292,11.699183149801));
#52360=CARTESIAN_POINT('Origin',(-50.,0.,0.));
#52361=CARTESIAN_POINT('',(-50.,9.48921088782658,10.3782842019456));
#52362=CARTESIAN_POINT('Ctrl Pts',(-50.,11.4573006693292,11.699183149801));
#52363=CARTESIAN_POINT('Ctrl Pts',(-50.,11.4568512923737,11.6990502442108));
#52364=CARTESIAN_POINT('Ctrl Pts',(-50.,11.4312436632693,11.6914658198642));
#52365=CARTESIAN_POINT('Ctrl Pts',(-50.,11.3816485785003,11.6755524200814));
#52366=CARTESIAN_POINT('Ctrl Pts',(-50.,11.3108562751064,11.6492077293642));
#52367=CARTESIAN_POINT('Ctrl Pts',(-50.,11.2220605212152,11.6098943525204));
#52368=CARTESIAN_POINT('Ctrl Pts',(-50.,11.1153726577894,11.5573722819667));
#52369=CARTESIAN_POINT('Ctrl Pts',(-50.,11.0075923712357,11.5044910494005));
#52370=CARTESIAN_POINT('Ctrl Pts',(-50.,10.896814048301,11.4525672852113));
#52371=CARTESIAN_POINT('Ctrl Pts',(-50.,10.7836901223469,11.4012548314131));
#52372=CARTESIAN_POINT('Ctrl Pts',(-50.,10.6701988175887,11.3493082317362));
#52373=CARTESIAN_POINT('Ctrl Pts',(-50.,10.558769691859,11.2951234927996));
#52374=CARTESIAN_POINT('Ctrl Pts',(-50.,10.4510776067987,11.237474600108));
#52375=CARTESIAN_POINT('Ctrl Pts',(-50.,10.347755963003,11.1757261609666));
#52376=CARTESIAN_POINT('Ctrl Pts',(-50.,10.2488131895374,11.1096536475468));
#52377=CARTESIAN_POINT('Ctrl Pts',(-50.,10.1538362031934,11.0393768173572));
#52378=CARTESIAN_POINT('Ctrl Pts',(-50.,10.0623044106004,10.9652479123292));
#52379=CARTESIAN_POINT('Ctrl Pts',(-50.,9.97376743729857,10.8877656023939));
#52380=CARTESIAN_POINT('Ctrl Pts',(-50.,9.88782918758628,10.8074894324552));
#52381=CARTESIAN_POINT('Ctrl Pts',(-50.,9.80416846317344,10.7249595816546));
#52382=CARTESIAN_POINT('Ctrl Pts',(-50.,9.72254683584991,10.6406085262144));
#52383=CARTESIAN_POINT('Ctrl Pts',(-50.,9.64281744709338,10.5546942954216));
#52384=CARTESIAN_POINT('Ctrl Pts',(-50.,9.58048422171402,10.4848202111794));
#52385=CARTESIAN_POINT('Ctrl Pts',(-50.,9.53453615016101,10.4317934371322));
#52386=CARTESIAN_POINT('Ctrl Pts',(-50.,9.5042599930153,10.3961665635534));
#52387=CARTESIAN_POINT('Ctrl Pts',(-50.,9.48921088782658,10.3782842019456));
#52388=CARTESIAN_POINT('',(-50.,8.41635544546802,11.2658274114927));
#52389=CARTESIAN_POINT('Origin',(-50.,0.,0.));
#52390=CARTESIAN_POINT('',(-50.,9.33394806226437,13.4542944285812));
#52391=CARTESIAN_POINT('Ctrl Pts',(-50.,8.416355445468,11.2658274114927));
#52392=CARTESIAN_POINT('Ctrl Pts',(-50.,8.4287661867593,11.2814252778905));
#52393=CARTESIAN_POINT('Ctrl Pts',(-50.,8.45349838774813,11.3126949862398));
#52394=CARTESIAN_POINT('Ctrl Pts',(-50.,8.49032885019461,11.3598214717827));
#52395=CARTESIAN_POINT('Ctrl Pts',(-50.,8.53889969364915,11.4231012534324));
#52396=CARTESIAN_POINT('Ctrl Pts',(-50.,8.59868074655117,11.5029661588994));
#52397=CARTESIAN_POINT('Ctrl Pts',(-50.,8.657420129699,11.5836641450553));
#52398=CARTESIAN_POINT('Ctrl Pts',(-50.,8.71490619380604,11.6653257040265));
#52399=CARTESIAN_POINT('Ctrl Pts',(-50.,8.77078674197194,11.7481669754252));
#52400=CARTESIAN_POINT('Ctrl Pts',(-50.,8.82454707622628,11.8325025950734));
#52401=CARTESIAN_POINT('Ctrl Pts',(-50.,8.87562220071675,11.9186739006343));
#52402=CARTESIAN_POINT('Ctrl Pts',(-50.,8.9235002736643,12.0069825427185));
#52403=CARTESIAN_POINT('Ctrl Pts',(-50.,8.96782328072592,12.0976260068268));
#52404=CARTESIAN_POINT('Ctrl Pts',(-50.,9.00850531748659,12.1906215239832));
#52405=CARTESIAN_POINT('Ctrl Pts',(-50.,9.04579810233888,12.2857645923749));
#52406=CARTESIAN_POINT('Ctrl Pts',(-50.,9.08015076502197,12.3827223068819));
#52407=CARTESIAN_POINT('Ctrl Pts',(-50.,9.11209941820162,12.4811072394643));
#52408=CARTESIAN_POINT('Ctrl Pts',(-50.,9.14215255670447,12.580553936713));
#52409=CARTESIAN_POINT('Ctrl Pts',(-50.,9.17066324563836,12.6808044286968));
#52410=CARTESIAN_POINT('Ctrl Pts',(-50.,9.19775517072751,12.7817574884561));
#52411=CARTESIAN_POINT('Ctrl Pts',(-50.,9.22340791088078,12.8834108105793));
#52412=CARTESIAN_POINT('Ctrl Pts',(-50.,9.24751415519882,12.9858220900665));
#52413=CARTESIAN_POINT('Ctrl Pts',(-50.,9.26994435872398,13.0890651211961));
#52414=CARTESIAN_POINT('Ctrl Pts',(-50.,9.29061590049322,13.1931829101653));
#52415=CARTESIAN_POINT('Ctrl Pts',(-50.,9.30753794249323,13.2870722636402));
#52416=CARTESIAN_POINT('Ctrl Pts',(-50.,9.3196569359812,13.3604514819665));
#52417=CARTESIAN_POINT('Ctrl Pts',(-50.,9.32779212083946,13.4129228945374));
#52418=CARTESIAN_POINT('Ctrl Pts',(-50.,9.33246655603105,13.4442440266596));
#52419=CARTESIAN_POINT('Ctrl Pts',(-50.,9.33394806226437,13.4542944285812));
#52420=CARTESIAN_POINT('',(-50.,8.1878799628551,14.1809466085264));
#52421=CARTESIAN_POINT('Origin',(-50.,0.,0.));
#52422=CARTESIAN_POINT('',(-50.,6.61011555120064,12.4121021043889));
#52423=CARTESIAN_POINT('Ctrl Pts',(-50.,8.1878799628551,14.1809466085264));
#52424=CARTESIAN_POINT('Ctrl Pts',(-50.,8.18747775617919,14.1807061229053));
#52425=CARTESIAN_POINT('Ctrl Pts',(-50.,8.16456080746724,14.1669916188038));
#52426=CARTESIAN_POINT('Ctrl Pts',(-50.,8.12048134508164,14.1392443717028));
#52427=CARTESIAN_POINT('Ctrl Pts',(-50.,8.05846477023863,14.0961220179458));
#52428=CARTESIAN_POINT('Ctrl Pts',(-50.,7.9822355374912,14.0359611371119));
#52429=CARTESIAN_POINT('Ctrl Pts',(-50.,7.89196117727994,13.9585569512687));
#52430=CARTESIAN_POINT('Ctrl Pts',(-50.,7.80071803438238,13.8805332125637));
#52431=CARTESIAN_POINT('Ctrl Pts',(-50.,7.70633293122716,13.8026912802767));
#52432=CARTESIAN_POINT('Ctrl Pts',(-50.,7.60952388977251,13.7248581251904));
#52433=CARTESIAN_POINT('Ctrl Pts',(-50.,7.51251671706145,13.646319383691));
#52434=CARTESIAN_POINT('Ctrl Pts',(-50.,7.41806353883254,13.5661256612623));
#52435=CARTESIAN_POINT('Ctrl Pts',(-50.,7.32809149527493,13.4835059820612));
#52436=CARTESIAN_POINT('Ctrl Pts',(-50.,7.24337210327696,13.3980024357456));
#52437=CARTESIAN_POINT('Ctrl Pts',(-50.,7.16396936488986,13.3093996446649));
#52438=CARTESIAN_POINT('Ctrl Pts',(-50.,7.08945339219251,13.2177108743086));
#52439=CARTESIAN_POINT('Ctrl Pts',(-50.,7.01923234820612,13.1231478339735));
#52440=CARTESIAN_POINT('Ctrl Pts',(-50.,6.95274599364373,13.0260815233846));
#52441=CARTESIAN_POINT('Ctrl Pts',(-50.,6.88947152371961,12.9269554033179));
#52442=CARTESIAN_POINT('Ctrl Pts',(-50.,6.82896349408885,12.8262128034276));
#52443=CARTESIAN_POINT('Ctrl Pts',(-50.,6.77088341473902,12.7242133182155));
#52444=CARTESIAN_POINT('Ctrl Pts',(-50.,6.71502487170408,12.6211703482748));
#52445=CARTESIAN_POINT('Ctrl Pts',(-50.,6.67202693734873,12.5379898440923));
#52446=CARTESIAN_POINT('Ctrl Pts',(-50.,6.64070963141069,12.4752021829311));
#52447=CARTESIAN_POINT('Ctrl Pts',(-50.,6.62024469858602,12.4331652189947));
#52448=CARTESIAN_POINT('Ctrl Pts',(-50.,6.61011555120064,12.4121021043889));
#52449=CARTESIAN_POINT('',(-50.,5.35024281477072,13.004953213026));
#52450=CARTESIAN_POINT('Origin',(-50.,0.,0.));
#52451=CARTESIAN_POINT('',(-50.,5.69475795663189,15.3528615187976));
#52452=CARTESIAN_POINT('Ctrl Pts',(-50.,5.35024281477071,13.004953213026));
#52453=CARTESIAN_POINT('Ctrl Pts',(-50.,5.35838461816811,13.0231474696198));
#52454=CARTESIAN_POINT('Ctrl Pts',(-50.,5.37456335134248,13.0595854308535));
#52455=CARTESIAN_POINT('Ctrl Pts',(-50.,5.39851683671257,13.1143907147436));
#52456=CARTESIAN_POINT('Ctrl Pts',(-50.,5.42982469604617,13.1877615232676));
#52457=CARTESIAN_POINT('Ctrl Pts',(-50.,5.46786602291259,13.2799842691689));
#52458=CARTESIAN_POINT('Ctrl Pts',(-50.,5.50469122725311,13.3727548702637));
#52459=CARTESIAN_POINT('Ctrl Pts',(-50.,5.54006285706051,13.466147083991));
#52460=CARTESIAN_POINT('Ctrl Pts',(-50.,5.57358602861192,13.5602826717323));
#52461=CARTESIAN_POINT('Ctrl Pts',(-50.,5.60468396737303,13.6553383842666));
#52462=CARTESIAN_POINT('Ctrl Pts',(-50.,5.63272454065023,13.7515043267519));
#52463=CARTESIAN_POINT('Ctrl Pts',(-50.,5.65713696965892,13.8489453830157));
#52464=CARTESIAN_POINT('Ctrl Pts',(-50.,5.67752537508807,13.9477637996424));
#52465=CARTESIAN_POINT('Ctrl Pts',(-50.,5.6938022661864,14.0479549027521));
#52466=CARTESIAN_POINT('Ctrl Pts',(-50.,5.70626231068308,14.1493832151514));
#52467=CARTESIAN_POINT('Ctrl Pts',(-50.,5.71542331821735,14.2518379845708));
#52468=CARTESIAN_POINT('Ctrl Pts',(-50.,5.72190090792526,14.3550772805332));
#52469=CARTESIAN_POINT('Ctrl Pts',(-50.,5.72627848390049,14.4588735885414));
#52470=CARTESIAN_POINT('Ctrl Pts',(-50.,5.72896217357436,14.5630648469857));
#52471=CARTESIAN_POINT('Ctrl Pts',(-50.,5.73009695097776,14.6675837685266));
#52472=CARTESIAN_POINT('Ctrl Pts',(-50.,5.72966360991829,14.772423041662));
#52473=CARTESIAN_POINT('Ctrl Pts',(-50.,5.72754386270271,14.8776118616624));
#52474=CARTESIAN_POINT('Ctrl Pts',(-50.,5.72359388237569,14.9831894879022));
#52475=CARTESIAN_POINT('Ctrl Pts',(-50.,5.71772294845736,15.0891770284618));
#52476=CARTESIAN_POINT('Ctrl Pts',(-50.,5.71076402066882,15.1843250159624));
#52477=CARTESIAN_POINT('Ctrl Pts',(-50.,5.70425360416528,15.2584127623331));
#52478=CARTESIAN_POINT('Ctrl Pts',(-50.,5.69908409756002,15.3112588271944));
#52479=CARTESIAN_POINT('Ctrl Pts',(-50.,5.69582242796104,15.3427584331158));
#52480=CARTESIAN_POINT('Ctrl Pts',(-50.,5.69475795663189,15.3528615187976));
#52481=CARTESIAN_POINT('',(-50.,4.40398464539872,15.7716690379646));
#52482=CARTESIAN_POINT('Origin',(-50.,0.,0.));
#52483=CARTESIAN_POINT('',(-50.,3.31568234418832,13.6660219830951));
#52484=CARTESIAN_POINT('Ctrl Pts',(-50.,4.40398464539872,15.7716690379646));
#52485=CARTESIAN_POINT('Ctrl Pts',(-50.,4.40365488112711,15.7713360829087));
#52486=CARTESIAN_POINT('Ctrl Pts',(-50.,4.38486856897779,15.7523532317834));
#52487=CARTESIAN_POINT('Ctrl Pts',(-50.,4.34907440371019,15.7145155989467));
#52488=CARTESIAN_POINT('Ctrl Pts',(-50.,4.29973028689649,15.6573251182294));
#52489=CARTESIAN_POINT('Ctrl Pts',(-50.,4.24085733833789,15.5800968628044));
#52490=CARTESIAN_POINT('Ctrl Pts',(-50.,4.17266875139903,15.482674151341));
#52491=CARTESIAN_POINT('Ctrl Pts',(-50.,4.10369589439471,15.3844104249513));
#52492=CARTESIAN_POINT('Ctrl Pts',(-50.,4.03163457417435,15.2855414194547));
#52493=CARTESIAN_POINT('Ctrl Pts',(-50.,3.95722328533246,15.1860781064647));
#52494=CARTESIAN_POINT('Ctrl Pts',(-50.,3.88279556209739,15.0858821011164));
#52495=CARTESIAN_POINT('Ctrl Pts',(-50.,3.81125317193191,14.9847182617076));
#52496=CARTESIAN_POINT('Ctrl Pts',(-50.,3.74465444426779,14.8823190942953));
#52497=CARTESIAN_POINT('Ctrl Pts',(-50.,3.68386053504292,14.7784329430806));
#52498=CARTESIAN_POINT('Ctrl Pts',(-50.,3.62898699781003,14.6728671135607));
#52499=CARTESIAN_POINT('Ctrl Pts',(-50.,3.57961415137445,14.5655275456869));
#52500=CARTESIAN_POINT('Ctrl Pts',(-50.,3.53511610244324,14.4564721136477));
#52501=CARTESIAN_POINT('Ctrl Pts',(-50.,3.49485794879717,14.3459208356842));
#52502=CARTESIAN_POINT('Ctrl Pts',(-50.,3.45822302631379,14.2341732241738));
#52503=CARTESIAN_POINT('Ctrl Pts',(-50.,3.42466963349977,14.1215479032503));
#52504=CARTESIAN_POINT('Ctrl Pts',(-50.,3.39378048711278,14.0083089910501));
#52505=CARTESIAN_POINT('Ctrl Pts',(-50.,3.36530258749166,13.8946118507282));
#52506=CARTESIAN_POINT('Ctrl Pts',(-50.,3.34434166251121,13.8033514635997));
#52507=CARTESIAN_POINT('Ctrl Pts',(-50.,3.32962290369722,13.7347480949923));
#52508=CARTESIAN_POINT('Ctrl Pts',(-50.,3.32025508218772,13.6889423777435));
#52509=CARTESIAN_POINT('Ctrl Pts',(-50.,3.31568234418832,13.6660219830951));
#52510=CARTESIAN_POINT('',(-50.,1.94795475120473,13.9269299753125));
#52511=CARTESIAN_POINT('Origin',(-50.,0.,0.));
#52512=CARTESIAN_POINT('',(-50.,1.69774526472952,16.2867518559131));
#52513=CARTESIAN_POINT('Ctrl Pts',(-50.,1.94795475120472,13.9269299753125));
#52514=CARTESIAN_POINT('Ctrl Pts',(-50.,1.9513160372573,13.9465774100468));
#52515=CARTESIAN_POINT('Ctrl Pts',(-50.,1.95792473331065,13.9858940930512));
#52516=CARTESIAN_POINT('Ctrl Pts',(-50.,1.96749615602378,14.044934557742));
#52517=CARTESIAN_POINT('Ctrl Pts',(-50.,1.97957384329226,14.1237862354018));
#52518=CARTESIAN_POINT('Ctrl Pts',(-50.,1.99348516764985,14.2225721274408));
#52519=CARTESIAN_POINT('Ctrl Pts',(-50.,2.00608233016073,14.3215862254212));
#52520=CARTESIAN_POINT('Ctrl Pts',(-50.,2.01711699607993,14.4208409176437));
#52521=CARTESIAN_POINT('Ctrl Pts',(-50.,2.02617640685866,14.5203559365434));
#52522=CARTESIAN_POINT('Ctrl Pts',(-50.,2.03265795226397,14.6201590419547));
#52523=CARTESIAN_POINT('Ctrl Pts',(-50.,2.03590208198289,14.7202771615244));
#52524=CARTESIAN_POINT('Ctrl Pts',(-50.,2.03531494435546,14.8207280520398));
#52525=CARTESIAN_POINT('Ctrl Pts',(-50.,2.03048766965571,14.9215122966393));
#52526=CARTESIAN_POINT('Ctrl Pts',(-50.,2.02133667816179,15.022603610217));
#52527=CARTESIAN_POINT('Ctrl Pts',(-50.,2.00818107188229,15.1239440527286));
#52528=CARTESIAN_POINT('Ctrl Pts',(-50.,1.99157480447254,15.2254582670956));
#52529=CARTESIAN_POINT('Ctrl Pts',(-50.,1.97217431992445,15.3270650217851));
#52530=CARTESIAN_POINT('Ctrl Pts',(-50.,1.95060127417394,15.4286890367845));
#52531=CARTESIAN_POINT('Ctrl Pts',(-50.,1.92728933849566,15.5302743417326));
#52532=CARTESIAN_POINT('Ctrl Pts',(-50.,1.90239566597564,15.6317918168208));
#52533=CARTESIAN_POINT('Ctrl Pts',(-50.,1.87590347211591,15.7332296038656));
#52534=CARTESIAN_POINT('Ctrl Pts',(-50.,1.84769092488014,15.8345865639611));
#52535=CARTESIAN_POINT('Ctrl Pts',(-50.,1.8176089524919,15.9358649547671));
#52536=CARTESIAN_POINT('Ctrl Pts',(-50.,1.78556443525587,16.0370626599488));
#52537=CARTESIAN_POINT('Ctrl Pts',(-50.,1.75516179270489,16.1274907834907));
#52538=CARTESIAN_POINT('Ctrl Pts',(-50.,1.73043103962239,16.1976318523256));
#52539=CARTESIAN_POINT('Ctrl Pts',(-50.,1.71228166066573,16.2475320568679));
#52540=CARTESIAN_POINT('Ctrl Pts',(-50.,1.70128882897267,16.2772309005009));
#52541=CARTESIAN_POINT('Ctrl Pts',(-50.,1.69774526472952,16.2867518559131));
#52542=CARTESIAN_POINT('',(-50.,0.343370775949385,16.3713994976063));
#52543=CARTESIAN_POINT('Origin',(-50.,0.,0.));
#52544=CARTESIAN_POINT('',(-50.,-0.187087378736033,14.0612554404903));
#52545=CARTESIAN_POINT('Ctrl Pts',(-50.,0.343370775949385,16.3713994976063));
#52546=CARTESIAN_POINT('Ctrl Pts',(-50.,0.343134174384057,16.3709949939062));
#52547=CARTESIAN_POINT('Ctrl Pts',(-50.,0.329658911880923,16.3479365581074));
#52548=CARTESIAN_POINT('Ctrl Pts',(-50.,0.304399122776818,16.3023860171632));
#52549=CARTESIAN_POINT('Ctrl Pts',(-50.,0.270827936326797,16.2347208977209));
#52550=CARTESIAN_POINT('Ctrl Pts',(-50.,0.233010475834533,16.1452778030188));
#52551=CARTESIAN_POINT('Ctrl Pts',(-50.,0.191192201865526,16.0339579931922));
#52552=CARTESIAN_POINT('Ctrl Pts',(-50.,0.148823449024451,15.9216285504355));
#52553=CARTESIAN_POINT('Ctrl Pts',(-50.,0.103613789511375,15.8079447749594));
#52554=CARTESIAN_POINT('Ctrl Pts',(-50.,0.0562757882257695,15.6931009498213));
#52555=CARTESIAN_POINT('Ctrl Pts',(-50.,0.00910408204356977,15.5775433641354));
#52556=CARTESIAN_POINT('Ctrl Pts',(-50.,-0.035032248569878,15.4617659038311));
#52557=CARTESIAN_POINT('Ctrl Pts',(-50.,-0.0740730173483893,15.3460213644938));
#52558=CARTESIAN_POINT('Ctrl Pts',(-50.,-0.107121538899203,15.2302801573274));
#52559=CARTESIAN_POINT('Ctrl Pts',(-50.,-0.13401796882278,15.1143843786811));
#52560=CARTESIAN_POINT('Ctrl Pts',(-50.,-0.155145411474415,14.9981385531066));
#52561=CARTESIAN_POINT('Ctrl Pts',(-50.,-0.171124489283723,14.8814430832361));
#52562=CARTESIAN_POINT('Ctrl Pts',(-50.,-0.182624874160768,14.7643531812717));
#52563=CARTESIAN_POINT('Ctrl Pts',(-50.,-0.190318342289957,14.6470055917277));
#52564=CARTESIAN_POINT('Ctrl Pts',(-50.,-0.194808815215985,14.5295742128916));
#52565=CARTESIAN_POINT('Ctrl Pts',(-50.,-0.196566149970303,14.4122110910203));
#52566=CARTESIAN_POINT('Ctrl Pts',(-50.,-0.195874035010017,14.2950037897925));
#52567=CARTESIAN_POINT('Ctrl Pts',(-50.,-0.193480898610155,14.2013977454735));
#52568=CARTESIAN_POINT('Ctrl Pts',(-50.,-0.190676276552008,14.1312892713751));
#52569=CARTESIAN_POINT('Ctrl Pts',(-50.,-0.188358372068459,14.0845929424903));
#52570=CARTESIAN_POINT('Ctrl Pts',(-50.,-0.187087378736033,14.0612554404903));
#52571=CARTESIAN_POINT('',(-50.,-1.57673047345589,13.9738265075847));
#52572=CARTESIAN_POINT('Origin',(-50.,0.,0.));
#52573=CARTESIAN_POINT('',(-50.,-2.40594300602614,16.1972856754381));
#52574=CARTESIAN_POINT('Ctrl Pts',(-50.,-1.57673047345591,13.9738265075847));
#52575=CARTESIAN_POINT('Ctrl Pts',(-50.,-1.57836090671277,13.9936925998767));
#52576=CARTESIAN_POINT('Ctrl Pts',(-50.,-1.58173749645856,14.0334175928621));
#52577=CARTESIAN_POINT('Ctrl Pts',(-50.,-1.58714954409268,14.0929835088213));
#52578=CARTESIAN_POINT('Ctrl Pts',(-50.,-1.59506091439902,14.1723615147133));
#52579=CARTESIAN_POINT('Ctrl Pts',(-50.,-1.60615369222193,14.2715034719842));
#52580=CARTESIAN_POINT('Ctrl Pts',(-50.,-1.61857609759037,14.3705396469258));
#52581=CARTESIAN_POINT('Ctrl Pts',(-50.,-1.63257174420173,14.4694202802978));
#52582=CARTESIAN_POINT('Ctrl Pts',(-50.,-1.64854533029309,14.5680618357278));
#52583=CARTESIAN_POINT('Ctrl Pts',(-50.,-1.66708743757887,14.6663413378531));
#52584=CARTESIAN_POINT('Ctrl Pts',(-50.,-1.68884359201954,14.7641208448459));
#52585=CARTESIAN_POINT('Ctrl Pts',(-50.,-1.71439340426661,14.8612698707291));
#52586=CARTESIAN_POINT('Ctrl Pts',(-50.,-1.74413304367239,14.957687298555));
#52587=CARTESIAN_POINT('Ctrl Pts',(-50.,-1.77813692730802,15.0533268835806));
#52588=CARTESIAN_POINT('Ctrl Pts',(-50.,-1.81608156923822,15.1482118634974));
#52589=CARTESIAN_POINT('Ctrl Pts',(-50.,-1.85741167873706,15.2424070113801));
#52590=CARTESIAN_POINT('Ctrl Pts',(-50.,-1.901471233747,15.3359968987161));
#52591=CARTESIAN_POINT('Ctrl Pts',(-50.,-1.94763938741864,15.4290632100973));
#52592=CARTESIAN_POINT('Ctrl Pts',(-50.,-1.99548217379509,15.5216595832348));
#52593=CARTESIAN_POINT('Ctrl Pts',(-50.,-2.04484013524158,15.6137968955554));
#52594=CARTESIAN_POINT('Ctrl Pts',(-50.,-2.09572657992989,15.7054594872874));
#52595=CARTESIAN_POINT('Ctrl Pts',(-50.,-2.14825922908453,15.7966159569104));
#52596=CARTESIAN_POINT('Ctrl Pts',(-50.,-2.20258303257508,15.8872314185123));
#52597=CARTESIAN_POINT('Ctrl Pts',(-50.,-2.25878765825938,15.9772806643205));
#52598=CARTESIAN_POINT('Ctrl Pts',(-50.,-2.31072370572823,16.0573069923301));
#52599=CARTESIAN_POINT('Ctrl Pts',(-50.,-2.35212087122016,16.1190941623136));
#52600=CARTESIAN_POINT('Ctrl Pts',(-50.,-2.38210973029964,16.1629130931652));
#52601=CARTESIAN_POINT('Ctrl Pts',(-50.,-2.40014300404269,16.1889450869399));
#52602=CARTESIAN_POINT('Ctrl Pts',(-50.,-2.40594300602614,16.1972856754381));
#52603=CARTESIAN_POINT('',(-50.,-3.73881834218223,15.9424547170177));
#52604=CARTESIAN_POINT('Origin',(-50.,0.,0.));
#52605=CARTESIAN_POINT('',(-50.,-3.67810171359515,13.5729685048794));
#52606=CARTESIAN_POINT('Ctrl Pts',(-50.,-3.73881834218223,15.9424547170177));
#52607=CARTESIAN_POINT('Ctrl Pts',(-50.,-3.73894691449477,15.9420040811286));
#52608=CARTESIAN_POINT('Ctrl Pts',(-50.,-3.74626442705009,15.9163189069806));
#52609=CARTESIAN_POINT('Ctrl Pts',(-50.,-3.75940267454228,15.8659175659396));
#52610=CARTESIAN_POINT('Ctrl Pts',(-50.,-3.77509152951778,15.7920294560818));
#52611=CARTESIAN_POINT('Ctrl Pts',(-50.,-3.7894772918181,15.6959915606914));
#52612=CARTESIAN_POINT('Ctrl Pts',(-50.,-3.80229765686693,15.5777692855585));
#52613=CARTESIAN_POINT('Ctrl Pts',(-50.,-3.81540012098238,15.4584321984421));
#52614=CARTESIAN_POINT('Ctrl Pts',(-50.,-3.83091743061146,15.3370768226993));
#52615=CARTESIAN_POINT('Ctrl Pts',(-50.,-3.84820772362302,15.2140685453126));
#52616=CARTESIAN_POINT('Ctrl Pts',(-50.,-3.86515944096752,15.0904102873887));
#52617=CARTESIAN_POINT('Ctrl Pts',(-50.,-3.87911646405442,14.9672939298197));
#52618=CARTESIAN_POINT('Ctrl Pts',(-50.,-3.88814619886307,14.8454766736426));
#52619=CARTESIAN_POINT('Ctrl Pts',(-50.,-3.89137277258683,14.725152856237));
#52620=CARTESIAN_POINT('Ctrl Pts',(-50.,-3.88860209359085,14.6062092864715));
#52621=CARTESIAN_POINT('Ctrl Pts',(-50.,-3.88015661753544,14.4883613559395));
#52622=CARTESIAN_POINT('Ctrl Pts',(-50.,-3.86661269999714,14.3713582537855));
#52623=CARTESIAN_POINT('Ctrl Pts',(-50.,-3.84863270462788,14.2550869169872));
#52624=CARTESIAN_POINT('Ctrl Pts',(-50.,-3.82690130950572,14.1395127300348));
#52625=CARTESIAN_POINT('Ctrl Pts',(-50.,-3.80204670961501,14.0246539387008));
#52626=CARTESIAN_POINT('Ctrl Pts',(-50.,-3.77456181293102,13.910540963737));
#52627=CARTESIAN_POINT('Ctrl Pts',(-50.,-3.7447431715177,13.7971880673979));
#52628=CARTESIAN_POINT('Ctrl Pts',(-50.,-3.71914634329887,13.7071179779119));
#52629=CARTESIAN_POINT('Ctrl Pts',(-50.,-3.69899456508718,13.6399095715909));
#52630=CARTESIAN_POINT('Ctrl Pts',(-50.,-3.68513657707394,13.595256733151));
#52631=CARTESIAN_POINT('Ctrl Pts',(-50.,-3.67810171359515,13.5729685048794));
#52632=CARTESIAN_POINT('',(-50.,-5.00234392366024,13.1426961282463));
#52633=CARTESIAN_POINT('Origin',(-50.,0.,0.));
#52634=CARTESIAN_POINT('',(-50.,-6.35845702927375,15.0900844665257));
#52635=CARTESIAN_POINT('Ctrl Pts',(-50.,-5.00234392366025,13.1426961282463));
#52636=CARTESIAN_POINT('Ctrl Pts',(-50.,-5.00886363010872,13.1615326184551));
#52637=CARTESIAN_POINT('Ctrl Pts',(-50.,-5.02201334210169,13.1991698540138));
#52638=CARTESIAN_POINT('Ctrl Pts',(-50.,-5.04206880122609,13.2555184756737));
#52639=CARTESIAN_POINT('Ctrl Pts',(-50.,-5.06947212861492,13.3304351977558));
#52640=CARTESIAN_POINT('Ctrl Pts',(-50.,-5.10487200859133,13.4237037664646));
#52641=CARTESIAN_POINT('Ctrl Pts',(-50.,-5.14153343642338,13.5165392112663));
#52642=CARTESIAN_POINT('Ctrl Pts',(-50.,-5.17967999761633,13.6088327519355));
#52643=CARTESIAN_POINT('Ctrl Pts',(-50.,-5.21968290141691,13.7004028321899));
#52644=CARTESIAN_POINT('Ctrl Pts',(-50.,-5.2620835925999,13.7909834684638));
#52645=CARTESIAN_POINT('Ctrl Pts',(-50.,-5.30747301200313,13.8802805168475));
#52646=CARTESIAN_POINT('Ctrl Pts',(-50.,-5.35638011020072,13.9680234475133));
#52647=CARTESIAN_POINT('Ctrl Pts',(-50.,-5.40916346339393,14.0540157969766));
#52648=CARTESIAN_POINT('Ctrl Pts',(-50.,-5.46588365010489,14.1381942665852));
#52649=CARTESIAN_POINT('Ctrl Pts',(-50.,-5.52623312628269,14.2206618116565));
#52650=CARTESIAN_POINT('Ctrl Pts',(-50.,-5.5896901550893,14.301619265488));
#52651=CARTESIAN_POINT('Ctrl Pts',(-50.,-5.6556403566801,14.3813116886496));
#52652=CARTESIAN_POINT('Ctrl Pts',(-50.,-5.72350270338309,14.4599725977946));
#52653=CARTESIAN_POINT('Ctrl Pts',(-50.,-5.79287020223623,14.5377618684515));
#52654=CARTESIAN_POINT('Ctrl Pts',(-50.,-5.86359111036561,14.614729691814));
#52655=CARTESIAN_POINT('Ctrl Pts',(-50.,-5.93567442341548,14.6908575904833));
#52656=CARTESIAN_POINT('Ctrl Pts',(-50.,-6.00922635494104,14.7660858733973));
#52657=CARTESIAN_POINT('Ctrl Pts',(-50.,-6.08437862517161,14.8403447030824));
#52658=CARTESIAN_POINT('Ctrl Pts',(-50.,-6.16121181596629,14.913587364225));
#52659=CARTESIAN_POINT('Ctrl Pts',(-50.,-6.23141793548312,14.9781835481972));
#52660=CARTESIAN_POINT('Ctrl Pts',(-50.,-6.2868803772285,15.027734504202));
#52661=CARTESIAN_POINT('Ctrl Pts',(-50.,-6.32682440612351,15.0627188567828));
#52662=CARTESIAN_POINT('Ctrl Pts',(-50.,-6.35076502500555,15.0834483147912));
#52663=CARTESIAN_POINT('Ctrl Pts',(-50.,-6.35845702927375,15.0900844665257));
#52664=CARTESIAN_POINT('',(-50.,-7.58608375346252,14.5117868743119));
#52665=CARTESIAN_POINT('Origin',(-50.,0.,0.));
#52666=CARTESIAN_POINT('',(-50.,-6.93800739067721,12.2318420402206));
#52667=CARTESIAN_POINT('Ctrl Pts',(-50.,-7.58608375346252,14.5117868743119));
#52668=CARTESIAN_POINT('Ctrl Pts',(-50.,-7.58609621785102,14.511318421344));
#52669=CARTESIAN_POINT('Ctrl Pts',(-50.,-7.58679619423276,14.4846204028018));
#52670=CARTESIAN_POINT('Ctrl Pts',(-50.,-7.58698737570401,14.4325351632849));
#52671=CARTESIAN_POINT('Ctrl Pts',(-50.,-7.5838081107473,14.3570667246954));
#52672=CARTESIAN_POINT('Ctrl Pts',(-50.,-7.5738582645032,14.2604684427868));
#52673=CARTESIAN_POINT('Ctrl Pts',(-50.,-7.55687516994583,14.1427720426853));
#52674=CARTESIAN_POINT('Ctrl Pts',(-50.,-7.53988806932779,14.0239256992838));
#52675=CARTESIAN_POINT('Ctrl Pts',(-50.,-7.52473801944021,13.9025239278461));
#52676=CARTESIAN_POINT('Ctrl Pts',(-50.,-7.51089419147856,13.7790802606718));
#52677=CARTESIAN_POINT('Ctrl Pts',(-50.,-7.49656078124055,13.6550912336386));
#52678=CARTESIAN_POINT('Ctrl Pts',(-50.,-7.47946152571002,13.5323718323411));
#52679=CARTESIAN_POINT('Ctrl Pts',(-50.,-7.45791285510172,13.4121360855424));
#52680=CARTESIAN_POINT('Ctrl Pts',(-50.,-7.43111474350486,13.2947900458654));
#52681=CARTESIAN_POINT('Ctrl Pts',(-50.,-7.39885104754049,13.1802723469128));
#52682=CARTESIAN_POINT('Ctrl Pts',(-50.,-7.36136331309888,13.0682271303129));
#52683=CARTESIAN_POINT('Ctrl Pts',(-50.,-7.31914741436296,12.9582681310911));
#52684=CARTESIAN_POINT('Ctrl Pts',(-50.,-7.27281678798223,12.8501211151659));
#52685=CARTESIAN_POINT('Ctrl Pts',(-50.,-7.22302599308674,12.7435822820237));
#52686=CARTESIAN_POINT('Ctrl Pts',(-50.,-7.17038802629925,12.6385130784722));
#52687=CARTESIAN_POINT('Ctrl Pts',(-50.,-7.11538787531798,12.5348203883111));
#52688=CARTESIAN_POINT('Ctrl Pts',(-50.,-7.05831632235693,12.4324442762203));
#52689=CARTESIAN_POINT('Ctrl Pts',(-50.,-7.01112414517467,12.3515695765444));
#52690=CARTESIAN_POINT('Ctrl Pts',(-50.,-6.97489142114752,12.2914841893452));
#52691=CARTESIAN_POINT('Ctrl Pts',(-50.,-6.95036409795758,12.2516805434111));
#52692=CARTESIAN_POINT('Ctrl Pts',(-50.,-6.93800739067721,12.2318420402206));
#52693=CARTESIAN_POINT('',(-50.,-8.11364170780697,11.4857618157149));
#52694=CARTESIAN_POINT('Origin',(-50.,0.,0.));
#52695=CARTESIAN_POINT('',(-50.,-9.91144581260293,13.0347177531328));
#52696=CARTESIAN_POINT('Ctrl Pts',(-50.,-8.11364170780698,11.4857618157149));
#52697=CARTESIAN_POINT('Ctrl Pts',(-50.,-8.12464103031309,11.502385137885));
#52698=CARTESIAN_POINT('Ctrl Pts',(-50.,-8.14673761978747,11.5355697300868));
#52699=CARTESIAN_POINT('Ctrl Pts',(-50.,-8.18017633214654,11.5851604663126));
#52700=CARTESIAN_POINT('Ctrl Pts',(-50.,-8.22534976477564,11.6509086114121));
#52701=CARTESIAN_POINT('Ctrl Pts',(-50.,-8.28283244225497,11.732443384369));
#52702=CARTESIAN_POINT('Ctrl Pts',(-50.,-8.34142932020866,11.8132449066089));
#52703=CARTESIAN_POINT('Ctrl Pts',(-50.,-8.40132990725019,11.8931522119833));
#52704=CARTESIAN_POINT('Ctrl Pts',(-50.,-8.46284859919381,11.9718971321485));
#52705=CARTESIAN_POINT('Ctrl Pts',(-50.,-8.52644368290816,12.0490873880617));
#52706=CARTESIAN_POINT('Ctrl Pts',(-50.,-8.59261438312223,12.1242911158748));
#52707=CARTESIAN_POINT('Ctrl Pts',(-50.,-8.66180575442286,12.1971147402934));
#52708=CARTESIAN_POINT('Ctrl Pts',(-50.,-8.73431624919877,12.2672787958196));
#52709=CARTESIAN_POINT('Ctrl Pts',(-50.,-8.81018880105177,12.334706907179));
#52710=CARTESIAN_POINT('Ctrl Pts',(-50.,-8.88915113193907,12.3995752782536));
#52711=CARTESIAN_POINT('Ctrl Pts',(-50.,-8.9707478415549,12.4622081834688));
#52712=CARTESIAN_POINT('Ctrl Pts',(-50.,-9.05444479601274,12.5229957744206));
#52713=CARTESIAN_POINT('Ctrl Pts',(-50.,-9.13973729492348,12.5823087271131));
#52714=CARTESIAN_POINT('Ctrl Pts',(-50.,-9.22627089118454,12.6404031093252));
#52715=CARTESIAN_POINT('Ctrl Pts',(-50.,-9.31391109124575,12.69736527232));
#52716=CARTESIAN_POINT('Ctrl Pts',(-50.,-9.40266201299437,12.7531750820743));
#52717=CARTESIAN_POINT('Ctrl Pts',(-50.,-9.49261168852801,12.8077483085937));
#52718=CARTESIAN_POINT('Ctrl Pts',(-50.,-9.58387033196931,12.8609845509879));
#52719=CARTESIAN_POINT('Ctrl Pts',(-50.,-9.67650437592402,12.9128185216976));
#52720=CARTESIAN_POINT('Ctrl Pts',(-50.,-9.76056925879954,12.9579257458254));
#52721=CARTESIAN_POINT('Ctrl Pts',(-50.,-9.82661206760692,12.9921270190498));
#52722=CARTESIAN_POINT('Ctrl Pts',(-50.,-9.87400143607813,13.0160785978238));
#52723=CARTESIAN_POINT('Ctrl Pts',(-50.,-9.90234512296736,13.0302030119816));
#52724=CARTESIAN_POINT('Ctrl Pts',(-50.,-9.91144581260293,13.0347177531328));
#52725=CARTESIAN_POINT('',(-50.,-10.9566876228483,12.1692900916743));
#52726=CARTESIAN_POINT('Origin',(-50.,0.,0.));
#52727=CARTESIAN_POINT('',(-50.,-9.76197254719673,10.1221439546065));
#52728=CARTESIAN_POINT('Ctrl Pts',(-50.,-10.9566876228483,12.1692900916743));
#52729=CARTESIAN_POINT('Ctrl Pts',(-50.,-10.9565831961294,12.1688332562504));
#52730=CARTESIAN_POINT('Ctrl Pts',(-50.,-10.9506216542472,12.1427999280076));
#52731=CARTESIAN_POINT('Ctrl Pts',(-50.,-10.9378537570625,12.0923034971696));
#52732=CARTESIAN_POINT('Ctrl Pts',(-50.,-10.9160061370834,12.0199966893985));
#52733=CARTESIAN_POINT('Ctrl Pts',(-50.,-10.8823458677273,11.9289076462876));
#52734=CARTESIAN_POINT('Ctrl Pts',(-50.,-10.8366264238543,11.819132418893));
#52735=CARTESIAN_POINT('Ctrl Pts',(-50.,-10.7906171205087,11.7082443720486));
#52736=CARTESIAN_POINT('Ctrl Pts',(-50.,-10.7457516444569,11.5944243246999));
#52737=CARTESIAN_POINT('Ctrl Pts',(-50.,-10.7016435541469,11.4783016873407));
#52738=CARTESIAN_POINT('Ctrl Pts',(-50.,-10.6569256372063,11.3617725777663));
#52739=CARTESIAN_POINT('Ctrl Pts',(-50.,-10.6098445121699,11.2471610440543));
#52740=CARTESIAN_POINT('Ctrl Pts',(-50.,-10.5590714183695,11.1360616608015));
#52741=CARTESIAN_POINT('Ctrl Pts',(-50.,-10.5039324453602,11.0290666820944));
#52742=CARTESIAN_POINT('Ctrl Pts',(-50.,-10.4442029791024,10.9261704221467));
#52743=CARTESIAN_POINT('Ctrl Pts',(-50.,-10.3800284784999,10.8269681325114));
#52744=CARTESIAN_POINT('Ctrl Pts',(-50.,-10.3117931787431,10.7309623645438));
#52745=CARTESIAN_POINT('Ctrl Pts',(-50.,-10.2400230449985,10.6377349442392));
#52746=CARTESIAN_POINT('Ctrl Pts',(-50.,-10.1653013890907,10.5469256916157));
#52747=CARTESIAN_POINT('Ctrl Pts',(-50.,-10.0881874924486,10.4582479603236));
#52748=CARTESIAN_POINT('Ctrl Pts',(-50.,-10.0091279489326,10.371490948043));
#52749=CARTESIAN_POINT('Ctrl Pts',(-50.,-9.92838949999087,10.2865242878363));
#52750=CARTESIAN_POINT('Ctrl Pts',(-50.,-9.86256723189823,10.2199266327873));
#52751=CARTESIAN_POINT('Ctrl Pts',(-50.,-9.8125301973609,10.1707396505663));
#52752=CARTESIAN_POINT('Ctrl Pts',(-50.,-9.77887468091545,10.1382862065996));
#52753=CARTESIAN_POINT('Ctrl Pts',(-50.,-9.76197254719673,10.1221439546065));
#52754=CARTESIAN_POINT('',(-50.,-10.7151295435653,9.10713484662512));
#52755=CARTESIAN_POINT('Origin',(-50.,0.,0.));
#52756=CARTESIAN_POINT('',(-50.,-12.8416620037784,10.1603317849721));
#52757=CARTESIAN_POINT('Ctrl Pts',(-50.,-10.7151295435653,9.10713484662511));
#52758=CARTESIAN_POINT('Ctrl Pts',(-50.,-10.7299173542433,9.1205004962881));
#52759=CARTESIAN_POINT('Ctrl Pts',(-50.,-10.7595724112169,9.14714733516059));
#52760=CARTESIAN_POINT('Ctrl Pts',(-50.,-10.8042932995341,9.18686421761339));
#52761=CARTESIAN_POINT('Ctrl Pts',(-50.,-10.8643984244951,9.23931258796881));
#52762=CARTESIAN_POINT('Ctrl Pts',(-50.,-10.9403520514449,9.30399043552504));
#52763=CARTESIAN_POINT('Ctrl Pts',(-50.,-11.0172025221741,9.36768097839366));
#52764=CARTESIAN_POINT('Ctrl Pts',(-50.,-11.0950933608815,9.43018117859799));
#52765=CARTESIAN_POINT('Ctrl Pts',(-50.,-11.1742623953034,9.49115310573639));
#52766=CARTESIAN_POINT('Ctrl Pts',(-50.,-11.255055958553,9.55010283362399));
#52767=CARTESIAN_POINT('Ctrl Pts',(-50.,-11.3378501911246,9.60648791406797));
#52768=CARTESIAN_POINT('Ctrl Pts',(-50.,-11.4229782872014,9.65981645609066));
#52769=CARTESIAN_POINT('Ctrl Pts',(-50.,-11.5106598224983,9.70974355202577));
#52770=CARTESIAN_POINT('Ctrl Pts',(-50.,-11.6009173880207,9.75618454891596));
#52771=CARTESIAN_POINT('Ctrl Pts',(-50.,-11.6935310799647,9.79937782767));
#52772=CARTESIAN_POINT('Ctrl Pts',(-50.,-11.7881404490329,9.83975072848667));
#52773=CARTESIAN_POINT('Ctrl Pts',(-50.,-11.8843251688933,9.87781397932795));
#52774=CARTESIAN_POINT('Ctrl Pts',(-50.,-11.9816885786214,9.91405212461268));
#52775=CARTESIAN_POINT('Ctrl Pts',(-50.,-12.079951048189,9.94880133468933));
#52776=CARTESIAN_POINT('Ctrl Pts',(-50.,-12.179003784094,9.98217869512325));
#52777=CARTESIAN_POINT('Ctrl Pts',(-50.,-12.2788457677249,10.0141636803616));
#52778=CARTESIAN_POINT('Ctrl Pts',(-50.,-12.3795413183411,10.0446528139577));
#52779=CARTESIAN_POINT('Ctrl Pts',(-50.,-12.4811722187999,10.0735214401623));
#52780=CARTESIAN_POINT('Ctrl Pts',(-50.,-12.5837865782488,10.1006898014275));
#52781=CARTESIAN_POINT('Ctrl Pts',(-50.,-12.6764281187229,10.123473812926));
#52782=CARTESIAN_POINT('Ctrl Pts',(-50.,-12.7489015820264,10.14017641159));
#52783=CARTESIAN_POINT('Ctrl Pts',(-50.,-12.8007586417669,10.151590250775));
#52784=CARTESIAN_POINT('Ctrl Pts',(-50.,-12.8317244585753,10.1582221321948));
#52785=CARTESIAN_POINT('Ctrl Pts',(-50.,-12.8416620037784,10.1603317849721));
#52786=CARTESIAN_POINT('',(-50.,-13.6388425130122,9.0621520570585));
#52787=CARTESIAN_POINT('Origin',(-50.,0.,0.));
#52788=CARTESIAN_POINT('',(-50.,-11.9725570665522,7.37643433768309));
#52789=CARTESIAN_POINT('Ctrl Pts',(-50.,-13.6388425130122,9.0621520570585));
#52790=CARTESIAN_POINT('Ctrl Pts',(-50.,-13.6386277567007,9.0617355438285));
#52791=CARTESIAN_POINT('Ctrl Pts',(-50.,-13.626379282156,9.03800267564235));
#52792=CARTESIAN_POINT('Ctrl Pts',(-50.,-13.6014545602526,8.99226792994578));
#52793=CARTESIAN_POINT('Ctrl Pts',(-50.,-13.5623113515642,8.92766605565115));
#52794=CARTESIAN_POINT('Ctrl Pts',(-50.,-13.5070556576137,8.84780971091874));
#52795=CARTESIAN_POINT('Ctrl Pts',(-50.,-13.4354725852278,8.7528532374933));
#52796=CARTESIAN_POINT('Ctrl Pts',(-50.,-13.3633320128944,8.65689099100683));
#52797=CARTESIAN_POINT('Ctrl Pts',(-50.,-13.2915701735423,8.557804399923));
#52798=CARTESIAN_POINT('Ctrl Pts',(-50.,-13.2199692944164,8.45629920475326));
#52799=CARTESIAN_POINT('Ctrl Pts',(-50.,-13.1476766619554,8.35455196515643));
#52800=CARTESIAN_POINT('Ctrl Pts',(-50.,-13.0735719476516,8.2552497632047));
#52801=CARTESIAN_POINT('Ctrl Pts',(-50.,-12.9967646908729,8.16026752634251));
#52802=CARTESIAN_POINT('Ctrl Pts',(-50.,-12.9167494409123,8.07034649661759));
#52803=CARTESIAN_POINT('Ctrl Pts',(-50.,-12.8333072263957,7.98553702611316));
#52804=CARTESIAN_POINT('Ctrl Pts',(-50.,-12.7464782795223,7.9054109081407));
#52805=CARTESIAN_POINT('Ctrl Pts',(-50.,-12.6565110535803,7.82939076691323));
#52806=CARTESIAN_POINT('Ctrl Pts',(-50.,-12.5638109939272,7.75694076391353));
#52807=CARTESIAN_POINT('Ctrl Pts',(-50.,-12.4688535134548,7.68756697112423));
#52808=CARTESIAN_POINT('Ctrl Pts',(-50.,-12.3721090366891,7.62085266008235));
#52809=CARTESIAN_POINT('Ctrl Pts',(-50.,-12.2739577025182,7.5564825878338));
#52810=CARTESIAN_POINT('Ctrl Pts',(-50.,-12.174625451278,7.49426414725743));
#52811=CARTESIAN_POINT('Ctrl Pts',(-50.,-12.0943089474566,7.44612811243127));
#52812=CARTESIAN_POINT('Ctrl Pts',(-50.,-12.0336116133124,7.4109301341784));
#52813=CARTESIAN_POINT('Ctrl Pts',(-50.,-11.9929426034861,7.38786606141889));
#52814=CARTESIAN_POINT('Ctrl Pts',(-50.,-11.9725570665522,7.37643433768309));
#52815=CARTESIAN_POINT('',(-50.,-12.6433463826116,6.15627310142281));
#52816=CARTESIAN_POINT('Origin',(-50.,0.,0.));
#52817=CARTESIAN_POINT('',(-50.,-14.9649893429273,6.64753480367511));
#52818=CARTESIAN_POINT('Ctrl Pts',(-50.,-12.6433463826116,6.1562731014228));
#52819=CARTESIAN_POINT('Ctrl Pts',(-50.,-12.6609935089309,6.16554126565498));
#52820=CARTESIAN_POINT('Ctrl Pts',(-50.,-12.6963436971102,6.18397603231157));
#52821=CARTESIAN_POINT('Ctrl Pts',(-50.,-12.7495367835008,6.21132350319834));
#52822=CARTESIAN_POINT('Ctrl Pts',(-50.,-12.8207969747412,6.24717657480866));
#52823=CARTESIAN_POINT('Ctrl Pts',(-50.,-12.9104491054422,6.29093354993378));
#52824=CARTESIAN_POINT('Ctrl Pts',(-50.,-13.0007243712348,6.33351120238525));
#52825=CARTESIAN_POINT('Ctrl Pts',(-50.,-13.0917112937495,6.37467717998103));
#52826=CARTESIAN_POINT('Ctrl Pts',(-50.,-13.1835561890537,6.41404502367149));
#52827=CARTESIAN_POINT('Ctrl Pts',(-50.,-13.2764716751216,6.45105019532836));
#52828=CARTESIAN_POINT('Ctrl Pts',(-50.,-13.3706871739224,6.48507374642914));
#52829=CARTESIAN_POINT('Ctrl Pts',(-50.,-13.4664030834197,6.51555637763196));
#52830=CARTESIAN_POINT('Ctrl Pts',(-50.,-13.5637463059047,6.54210941091933));
#52831=CARTESIAN_POINT('Ctrl Pts',(-50.,-13.6627176703106,6.56464523470766));
#52832=CARTESIAN_POINT('Ctrl Pts',(-50.,-13.7631634644371,6.58344942858329));
#52833=CARTESIAN_POINT('Ctrl Pts',(-50.,-13.8648408383502,6.59902554716193));
#52834=CARTESIAN_POINT('Ctrl Pts',(-50.,-13.9674696839217,6.61197280385553));
#52835=CARTESIAN_POINT('Ctrl Pts',(-50.,-14.0707863033563,6.6228591657896));
#52836=CARTESIAN_POINT('Ctrl Pts',(-50.,-14.1746034538834,6.63207978306306));
#52837=CARTESIAN_POINT('Ctrl Pts',(-50.,-14.278844877945,6.63977511862666));
#52838=CARTESIAN_POINT('Ctrl Pts',(-50.,-14.3835044844334,6.64592554509403));
#52839=CARTESIAN_POINT('Ctrl Pts',(-50.,-14.4886188383546,6.65041484137187));
#52840=CARTESIAN_POINT('Ctrl Pts',(-50.,-14.5942361525827,6.65310192943101));
#52841=CARTESIAN_POINT('Ctrl Pts',(-50.,-14.7003831899324,6.65389759319505));
#52842=CARTESIAN_POINT('Ctrl Pts',(-50.,-14.7957803793054,6.65292678882822));
#52843=CARTESIAN_POINT('Ctrl Pts',(-50.,-14.870130722867,6.65108122722986));
#52844=CARTESIAN_POINT('Ctrl Pts',(-50.,-14.9231971040963,6.64924015333274));
#52845=CARTESIAN_POINT('Ctrl Pts',(-50.,-14.9548393546694,6.64796279651443));
#52846=CARTESIAN_POINT('Ctrl Pts',(-50.,-14.9649893429273,6.64753480367511));
#52847=CARTESIAN_POINT('',(-50.,-15.4640187679296,5.38560568043381));
#52848=CARTESIAN_POINT('Origin',(-50.,0.,0.));
#52849=CARTESIAN_POINT('',(-50.,-13.4308617934315,4.1672362226952));
#52850=CARTESIAN_POINT('Ctrl Pts',(-50.,-15.4640187679296,5.38560568043381));
#52851=CARTESIAN_POINT('Ctrl Pts',(-50.,-15.4637071759544,5.38525566045572));
#52852=CARTESIAN_POINT('Ctrl Pts',(-50.,-15.4459413854495,5.3653144757178));
#52853=CARTESIAN_POINT('Ctrl Pts',(-50.,-15.4104259507712,5.32721509743538));
#52854=CARTESIAN_POINT('Ctrl Pts',(-50.,-15.3564466651341,5.27437732996824));
#52855=CARTESIAN_POINT('Ctrl Pts',(-50.,-15.2830674650563,5.2107713514449));
#52856=CARTESIAN_POINT('Ctrl Pts',(-50.,-15.1901185918597,5.13660009643943));
#52857=CARTESIAN_POINT('Ctrl Pts',(-50.,-15.0963796080126,5.06159331118216));
#52858=CARTESIAN_POINT('Ctrl Pts',(-50.,-15.0022304656484,4.98346615129592));
#52859=CARTESIAN_POINT('Ctrl Pts',(-50.,-14.9076357442716,4.90295634303817));
#52860=CARTESIAN_POINT('Ctrl Pts',(-50.,-14.8123108082616,4.82238412668293));
#52861=CARTESIAN_POINT('Ctrl Pts',(-50.,-14.7158387764281,4.74463077904808));
#52862=CARTESIAN_POINT('Ctrl Pts',(-50.,-14.6178234390918,4.67173377183878));
#52863=CARTESIAN_POINT('Ctrl Pts',(-50.,-14.5179595646104,4.60453676010005));
#52864=CARTESIAN_POINT('Ctrl Pts',(-50.,-14.4160475830522,4.54314296997813));
#52865=CARTESIAN_POINT('Ctrl Pts',(-50.,-14.3120199719745,4.48712764234399));
#52866=CARTESIAN_POINT('Ctrl Pts',(-50.,-14.2059737915295,4.4358697529125));
#52867=CARTESIAN_POINT('Ctrl Pts',(-50.,-14.0981684916428,4.38874946735859));
#52868=CARTESIAN_POINT('Ctrl Pts',(-50.,-13.988941714333,4.34517014494338));
#52869=CARTESIAN_POINT('Ctrl Pts',(-50.,-13.8786454687203,4.30461115967259));
#52870=CARTESIAN_POINT('Ctrl Pts',(-50.,-13.7675695531958,4.26667263583206));
#52871=CARTESIAN_POINT('Ctrl Pts',(-50.,-13.655884910321,4.23111182833087));
#52872=CARTESIAN_POINT('Ctrl Pts',(-50.,-13.5661207520894,4.20446197782756));
#52873=CARTESIAN_POINT('Ctrl Pts',(-50.,-13.4985769550718,4.18546462196559));
#52874=CARTESIAN_POINT('Ctrl Pts',(-50.,-13.4534498353221,4.1732391209285));
#52875=CARTESIAN_POINT('Ctrl Pts',(-50.,-13.4308617934315,4.1672362226952));
#52876=CARTESIAN_POINT('',(-50.,-13.7771352694631,2.8185900760694));
#52877=CARTESIAN_POINT('Origin',(-50.,0.,0.));
#52878=CARTESIAN_POINT('',(-50.,-16.1480113642792,2.71704876274038));
#52879=CARTESIAN_POINT('Ctrl Pts',(-50.,-13.7771352694631,2.81859007606939));
#52880=CARTESIAN_POINT('Ctrl Pts',(-50.,-13.7965328775753,2.82317840202614));
#52881=CARTESIAN_POINT('Ctrl Pts',(-50.,-13.8353570146283,2.83224277227946));
#52882=CARTESIAN_POINT('Ctrl Pts',(-50.,-13.8936799818437,2.84550248942744));
#52883=CARTESIAN_POINT('Ctrl Pts',(-50.,-13.9716176994713,2.862507481945));
#52884=CARTESIAN_POINT('Ctrl Pts',(-50.,-14.0693351608341,2.882594172965));
#52885=CARTESIAN_POINT('Ctrl Pts',(-50.,-14.1673628947312,2.90138362450613));
#52886=CARTESIAN_POINT('Ctrl Pts',(-50.,-14.2657288580852,2.91862876972314));
#52887=CARTESIAN_POINT('Ctrl Pts',(-50.,-14.3644786617177,2.93391890356181));
#52888=CARTESIAN_POINT('Ctrl Pts',(-50.,-14.463677848895,2.94665434795724));
#52889=CARTESIAN_POINT('Ctrl Pts',(-50.,-14.5633947076351,2.95617854486928));
#52890=CARTESIAN_POINT('Ctrl Pts',(-50.,-14.6636842479405,2.96189992942649));
#52891=CARTESIAN_POINT('Ctrl Pts',(-50.,-14.7645727249416,2.96341047532946));
#52892=CARTESIAN_POINT('Ctrl Pts',(-50.,-14.8660391534142,2.96062511732634));
#52893=CARTESIAN_POINT('Ctrl Pts',(-50.,-14.9680056710645,2.95385868966535));
#52894=CARTESIAN_POINT('Ctrl Pts',(-50.,-15.0703622864763,2.94365932119071));
#52895=CARTESIAN_POINT('Ctrl Pts',(-50.,-15.1729867099492,2.9306770599819));
#52896=CARTESIAN_POINT('Ctrl Pts',(-50.,-15.2757647759192,2.91552760840775));
#52897=CARTESIAN_POINT('Ctrl Pts',(-50.,-15.3786133940255,2.89864026758367));
#52898=CARTESIAN_POINT('Ctrl Pts',(-50.,-15.4814936341966,2.88017005204204));
#52899=CARTESIAN_POINT('Ctrl Pts',(-50.,-15.5843947155558,2.86009946582377));
#52900=CARTESIAN_POINT('Ctrl Pts',(-50.,-15.6873231513416,2.83830684578773));
#52901=CARTESIAN_POINT('Ctrl Pts',(-50.,-15.7902905550528,2.81464355607623));
#52902=CARTESIAN_POINT('Ctrl Pts',(-50.,-15.8933006615651,2.78901652785862));
#52903=CARTESIAN_POINT('Ctrl Pts',(-50.,-15.9854593435823,2.76435190683515));
#52904=CARTESIAN_POINT('Ctrl Pts',(-50.,-16.0570148618746,2.74407414839715));
#52905=CARTESIAN_POINT('Ctrl Pts',(-50.,-16.1079562086956,2.72909384286184));
#52906=CARTESIAN_POINT('Ctrl Pts',(-50.,-16.1382866940579,2.7199875088322));
#52907=CARTESIAN_POINT('Ctrl Pts',(-50.,-16.1480113642792,2.71704876274038));
#52908=CARTESIAN_POINT('',(-50.,-16.3175338509752,1.37066189203528));
#52909=CARTESIAN_POINT('Origin',(-50.,0.,0.));
#52910=CARTESIAN_POINT('',(-50.,-14.045256078575,0.696195329812624));
#52911=CARTESIAN_POINT('Ctrl Pts',(-50.,-16.3175338509752,1.37066189203528));
#52912=CARTESIAN_POINT('Ctrl Pts',(-50.,-16.317145001806,1.37040035835161));
#52913=CARTESIAN_POINT('Ctrl Pts',(-50.,-16.2949781852964,1.35550383503756));
#52914=CARTESIAN_POINT('Ctrl Pts',(-50.,-16.2511036032208,1.32743374822648));
#52915=CARTESIAN_POINT('Ctrl Pts',(-50.,-16.1856799576735,1.28968007884051));
#52916=CARTESIAN_POINT('Ctrl Pts',(-50.,-16.0987879364791,1.2463210640833));
#52917=CARTESIAN_POINT('Ctrl Pts',(-50.,-15.9903135820168,1.19759548023257));
#52918=CARTESIAN_POINT('Ctrl Pts',(-50.,-15.8808661517589,1.14825710837788));
#52919=CARTESIAN_POINT('Ctrl Pts',(-50.,-15.7702454432537,1.09599839647648));
#52920=CARTESIAN_POINT('Ctrl Pts',(-50.,-15.6586006138651,1.04154270247793));
#52921=CARTESIAN_POINT('Ctrl Pts',(-50.,-15.5462329906162,0.987208158041752));
#52922=CARTESIAN_POINT('Ctrl Pts',(-50.,-15.4334553338124,0.935889193512498));
#52923=CARTESIAN_POINT('Ctrl Pts',(-50.,-15.3203905800386,0.889657803015486));
#52924=CARTESIAN_POINT('Ctrl Pts',(-50.,-15.2069528955437,0.849407044643804));
#52925=CARTESIAN_POINT('Ctrl Pts',(-50.,-15.0929746515511,0.81528653252832));
#52926=CARTESIAN_POINT('Ctrl Pts',(-50.,-14.97828481366,0.786901644277719));
#52927=CARTESIAN_POINT('Ctrl Pts',(-50.,-14.8628229502399,0.763626728348506));
#52928=CARTESIAN_POINT('Ctrl Pts',(-50.,-14.7466862135917,0.744796901078022));
#52929=CARTESIAN_POINT('Ctrl Pts',(-50.,-14.6300532595709,0.7297502981378));
#52930=CARTESIAN_POINT('Ctrl Pts',(-50.,-14.5131355638642,0.717895108848178));
#52931=CARTESIAN_POINT('Ctrl Pts',(-50.,-14.3961143752671,0.708771950396692));
#52932=CARTESIAN_POINT('Ctrl Pts',(-50.,-14.279094897617,0.702103192289484));
#52933=CARTESIAN_POINT('Ctrl Pts',(-50.,-14.1855232971663,0.698614034227448));
#52934=CARTESIAN_POINT('Ctrl Pts',(-50.,-14.1153770624506,0.697010974492569));
#52935=CARTESIAN_POINT('Ctrl Pts',(-50.,-14.0686273356774,0.696392218370307));
#52936=CARTESIAN_POINT('Ctrl Pts',(-50.,-14.045256078575,0.696195329812624));
#52937=CARTESIAN_POINT('',(-50.,-14.045256078575,-0.696195329812616));
#52938=CARTESIAN_POINT('Origin',(-50.,0.,0.));
#52939=CARTESIAN_POINT('',(-50.,-16.3163944433819,-1.38415944456368));
#52940=CARTESIAN_POINT('Ctrl Pts',(-50.,-14.045256078575,-0.696195329812629));
#52941=CARTESIAN_POINT('Ctrl Pts',(-50.,-14.0651853454231,-0.696575143525857));
#52942=CARTESIAN_POINT('Ctrl Pts',(-50.,-14.1050439680336,-0.697450717395246));
#52943=CARTESIAN_POINT('Ctrl Pts',(-50.,-14.1648321695468,-0.699111910780302));
#52944=CARTESIAN_POINT('Ctrl Pts',(-50.,-14.2445503001281,-0.702023483575367));
#52945=CARTESIAN_POINT('Ctrl Pts',(-50.,-14.3441931446757,-0.706869197330954));
#52946=CARTESIAN_POINT('Ctrl Pts',(-50.,-14.4438139036356,-0.71304855704325));
#52947=CARTESIAN_POINT('Ctrl Pts',(-50.,-14.5433782125866,-0.72080782010221));
#52948=CARTESIAN_POINT('Ctrl Pts',(-50.,-14.6428281112089,-0.730556131457601));
#52949=CARTESIAN_POINT('Ctrl Pts',(-50.,-14.7420779497362,-0.742890629132665));
#52950=CARTESIAN_POINT('Ctrl Pts',(-50.,-14.8410305914479,-0.758464226728878));
#52951=CARTESIAN_POINT('Ctrl Pts',(-50.,-14.939592201905,-0.777863584450799));
#52952=CARTESIAN_POINT('Ctrl Pts',(-50.,-15.0376867393704,-0.801490439086723));
#52953=CARTESIAN_POINT('Ctrl Pts',(-50.,-15.1352727230412,-0.829421964594113));
#52954=CARTESIAN_POINT('Ctrl Pts',(-50.,-15.2323530329047,-0.861333854256595));
#52955=CARTESIAN_POINT('Ctrl Pts',(-50.,-15.3289574472276,-0.89666784595261));
#52956=CARTESIAN_POINT('Ctrl Pts',(-50.,-15.4251291786488,-0.934763901846662));
#52957=CARTESIAN_POINT('Ctrl Pts',(-50.,-15.5209107672782,-0.974997271170846));
#52958=CARTESIAN_POINT('Ctrl Pts',(-50.,-15.6163284960372,-1.01693147636119));
#52959=CARTESIAN_POINT('Ctrl Pts',(-50.,-15.7113832084608,-1.06040669143688));
#52960=CARTESIAN_POINT('Ctrl Pts',(-50.,-15.8060601113054,-1.10543718159424));
#52961=CARTESIAN_POINT('Ctrl Pts',(-50.,-15.900335256791,-1.15214240747963));
#52962=CARTESIAN_POINT('Ctrl Pts',(-50.,-15.9941829293225,-1.20066922344171));
#52963=CARTESIAN_POINT('Ctrl Pts',(-50.,-16.0875836011606,-1.25110870320843));
#52964=CARTESIAN_POINT('Ctrl Pts',(-50.,-16.170713106895,-1.29791737203952));
#52965=CARTESIAN_POINT('Ctrl Pts',(-50.,-16.2349777035408,-1.33535320117812));
#52966=CARTESIAN_POINT('Ctrl Pts',(-50.,-16.2805931837835,-1.36253147066111));
#52967=CARTESIAN_POINT('Ctrl Pts',(-50.,-16.307706127992,-1.37889459744425));
#52968=CARTESIAN_POINT('Ctrl Pts',(-50.,-16.3163944433819,-1.38415944456368));
#52969=CARTESIAN_POINT('',(-50.,-16.1457582704724,-2.73040562398164));
#52970=CARTESIAN_POINT('Origin',(-50.,0.,0.));
#52971=CARTESIAN_POINT('',(-50.,-13.7771352694631,-2.8185900760694));
#52972=CARTESIAN_POINT('Ctrl Pts',(-50.,-16.1457582704724,-2.73040562398164));
#52973=CARTESIAN_POINT('Ctrl Pts',(-50.,-16.1453165969326,-2.73056223824769));
#52974=CARTESIAN_POINT('Ctrl Pts',(-50.,-16.1201415770235,-2.73947809679247));
#52975=CARTESIAN_POINT('Ctrl Pts',(-50.,-16.0706646489018,-2.75575514534332));
#52976=CARTESIAN_POINT('Ctrl Pts',(-50.,-15.9979074517054,-2.77605251475231));
#52977=CARTESIAN_POINT('Ctrl Pts',(-50.,-15.9029623546524,-2.7964401593829));
#52978=CARTESIAN_POINT('Ctrl Pts',(-50.,-15.7857783615561,-2.81665846444538));
#52979=CARTESIAN_POINT('Ctrl Pts',(-50.,-15.6674994694501,-2.83722831154002));
#52980=CARTESIAN_POINT('Ctrl Pts',(-50.,-15.5473579007536,-2.86033496839371));
#52981=CARTESIAN_POINT('Ctrl Pts',(-50.,-15.4256780185848,-2.88531489660512));
#52982=CARTESIAN_POINT('Ctrl Pts',(-50.,-15.3033281791249,-2.90999772986683));
#52983=CARTESIAN_POINT('Ctrl Pts',(-50.,-15.181331132295,-2.93165775201116));
#52984=CARTESIAN_POINT('Ctrl Pts',(-50.,-15.0603212363863,-2.9483186375038));
#52985=CARTESIAN_POINT('Ctrl Pts',(-50.,-14.9404374487894,-2.959094039328));
#52986=CARTESIAN_POINT('Ctrl Pts',(-50.,-14.8215546146151,-2.96379735617437));
#52987=CARTESIAN_POINT('Ctrl Pts',(-50.,-14.703408934225,-2.96276827812033));
#52988=CARTESIAN_POINT('Ctrl Pts',(-50.,-14.5857862813476,-2.95659777198027));
#52989=CARTESIAN_POINT('Ctrl Pts',(-50.,-14.4686154062224,-2.94595399366867));
#52990=CARTESIAN_POINT('Ctrl Pts',(-50.,-14.3519047529378,-2.93152244373364));
#52991=CARTESIAN_POINT('Ctrl Pts',(-50.,-14.2357119759516,-2.91392893189869));
#52992=CARTESIAN_POINT('Ctrl Pts',(-50.,-14.1200983859353,-2.89366348336299));
#52993=CARTESIAN_POINT('Ctrl Pts',(-50.,-14.0050968376581,-2.87102116947837));
#52994=CARTESIAN_POINT('Ctrl Pts',(-50.,-13.913597242777,-2.85113039846586));
#52995=CARTESIAN_POINT('Ctrl Pts',(-50.,-13.8452561162702,-2.83523843593487));
#52996=CARTESIAN_POINT('Ctrl Pts',(-50.,-13.7998212397401,-2.82421156841951));
#52997=CARTESIAN_POINT('Ctrl Pts',(-50.,-13.7771352694631,-2.8185900760694));
#52998=CARTESIAN_POINT('',(-50.,-13.4308617934315,-4.16723622269519));
#52999=CARTESIAN_POINT('Origin',(-50.,0.,0.));
#53000=CARTESIAN_POINT('',(-50.,-15.4595584521058,-5.39839582338345));
#53001=CARTESIAN_POINT('Ctrl Pts',(-50.,-13.4308617934315,-4.1672362226952));
#53002=CARTESIAN_POINT('Ctrl Pts',(-50.,-13.4500704898848,-4.17256031098595));
#53003=CARTESIAN_POINT('Ctrl Pts',(-50.,-13.4884591342042,-4.1833208134517));
#53004=CARTESIAN_POINT('Ctrl Pts',(-50.,-13.5459558574286,-4.19979853847996));
#53005=CARTESIAN_POINT('Ctrl Pts',(-50.,-13.6224454176364,-4.22244373176092));
#53006=CARTESIAN_POINT('Ctrl Pts',(-50.,-13.717752718985,-4.25191737627554));
#53007=CARTESIAN_POINT('Ctrl Pts',(-50.,-13.8127069643429,-4.28267727534445));
#53008=CARTESIAN_POINT('Ctrl Pts',(-50.,-13.9072136271877,-4.31495340364481));
#53009=CARTESIAN_POINT('Ctrl Pts',(-50.,-14.0011148179182,-4.34912763794002));
#53010=CARTESIAN_POINT('Ctrl Pts',(-50.,-14.0941790754254,-4.38575705583354));
#53011=CARTESIAN_POINT('Ctrl Pts',(-50.,-14.1861499417075,-4.42544990152536));
#53012=CARTESIAN_POINT('Ctrl Pts',(-50.,-14.2767906338471,-4.4687510685349));
#53013=CARTESIAN_POINT('Ctrl Pts',(-50.,-14.3659275912213,-4.51603076153944));
#53014=CARTESIAN_POINT('Ctrl Pts',(-50.,-14.4535014438403,-4.56735341407851));
#53015=CARTESIAN_POINT('Ctrl Pts',(-50.,-14.5395956330118,-4.62240562435127));
#53016=CARTESIAN_POINT('Ctrl Pts',(-50.,-14.6243778356077,-4.68065407462106));
#53017=CARTESIAN_POINT('Ctrl Pts',(-50.,-14.7080540513971,-4.74147020990105));
#53018=CARTESIAN_POINT('Ctrl Pts',(-50.,-14.7908208532122,-4.80425948641264));
#53019=CARTESIAN_POINT('Ctrl Pts',(-50.,-14.8728122458042,-4.86860567563393));
#53020=CARTESIAN_POINT('Ctrl Pts',(-50.,-14.954068793312,-4.9343541825898));
#53021=CARTESIAN_POINT('Ctrl Pts',(-50.,-15.0345726196388,-5.00151514537911));
#53022=CARTESIAN_POINT('Ctrl Pts',(-50.,-15.1142708207137,-5.07019831600168));
#53023=CARTESIAN_POINT('Ctrl Pts',(-50.,-15.1931019676527,-5.14053953989829));
#53024=CARTESIAN_POINT('Ctrl Pts',(-50.,-15.2710244971014,-5.21262217319695));
#53025=CARTESIAN_POINT('Ctrl Pts',(-50.,-15.3399014939787,-5.27863372902275));
#53026=CARTESIAN_POINT('Ctrl Pts',(-50.,-15.3928371880222,-5.33087539803783));
#53027=CARTESIAN_POINT('Ctrl Pts',(-50.,-15.430260613301,-5.36854392084221));
#53028=CARTESIAN_POINT('Ctrl Pts',(-50.,-15.4524524103566,-5.39113568494369));
#53029=CARTESIAN_POINT('Ctrl Pts',(-50.,-15.4595584521058,-5.39839582338345));
#53030=CARTESIAN_POINT('',(-50.,-14.9594853178907,-6.65991171291435));
#53031=CARTESIAN_POINT('Origin',(-50.,0.,0.));
#53032=CARTESIAN_POINT('',(-50.,-12.6433463826116,-6.1562731014228));
#53033=CARTESIAN_POINT('Ctrl Pts',(-50.,-14.9594853178907,-6.65991171291435));
#53034=CARTESIAN_POINT('Ctrl Pts',(-50.,-14.9590185719531,-6.65995356711246));
#53035=CARTESIAN_POINT('Ctrl Pts',(-50.,-14.9324171877326,-6.66232854470537));
#53036=CARTESIAN_POINT('Ctrl Pts',(-50.,-14.880446730922,-6.66578980817273));
#53037=CARTESIAN_POINT('Ctrl Pts',(-50.,-14.8049275843586,-6.66735551923628));
#53038=CARTESIAN_POINT('Ctrl Pts',(-50.,-14.7078951610787,-6.6634907630476));
#53039=CARTESIAN_POINT('Ctrl Pts',(-50.,-14.5893646306071,-6.65393139885702));
#53040=CARTESIAN_POINT('Ctrl Pts',(-50.,-14.4696861744433,-6.64444024204806));
#53041=CARTESIAN_POINT('Ctrl Pts',(-50.,-14.3475726821666,-6.63694296762358));
#53042=CARTESIAN_POINT('Ctrl Pts',(-50.,-14.2235033417215,-6.63087754928856));
#53043=CARTESIAN_POINT('Ctrl Pts',(-50.,-14.0988589764351,-6.62435775818486));
#53044=CARTESIAN_POINT('Ctrl Pts',(-50.,-13.9753080627051,-6.61499785909296));
#53045=CARTESIAN_POINT('Ctrl Pts',(-50.,-13.8539565214648,-6.60104137487127));
#53046=CARTESIAN_POINT('Ctrl Pts',(-50.,-13.7351593700424,-6.58166436202222));
#53047=CARTESIAN_POINT('Ctrl Pts',(-50.,-13.6188417913781,-6.55665495690443));
#53048=CARTESIAN_POINT('Ctrl Pts',(-50.,-13.5046637960973,-6.52627657330457));
#53049=CARTESIAN_POINT('Ctrl Pts',(-50.,-13.3922710176287,-6.49104836068956));
#53050=CARTESIAN_POINT('Ctrl Pts',(-50.,-13.281428281035,-6.45159976453225));
#53051=CARTESIAN_POINT('Ctrl Pts',(-50.,-13.1719732880642,-6.40859684907992));
#53052=CARTESIAN_POINT('Ctrl Pts',(-50.,-13.0638062493037,-6.3626601011734));
#53053=CARTESIAN_POINT('Ctrl Pts',(-50.,-12.9568646849259,-6.31427939831312));
#53054=CARTESIAN_POINT('Ctrl Pts',(-50.,-12.851107036246,-6.26374871229064));
#53055=CARTESIAN_POINT('Ctrl Pts',(-50.,-12.7674287029928,-6.22172782249946));
#53056=CARTESIAN_POINT('Ctrl Pts',(-50.,-12.7051868090144,-6.18933938815496));
#53057=CARTESIAN_POINT('Ctrl Pts',(-50.,-12.6639216231176,-6.16735975564195));
#53058=CARTESIAN_POINT('Ctrl Pts',(-50.,-12.6433463826116,-6.1562731014228));
#53059=CARTESIAN_POINT('',(-50.,-11.9725570665522,-7.37643433768308));
#53060=CARTESIAN_POINT('Origin',(-50.,0.,0.));
#53061=CARTESIAN_POINT('',(-50.,-13.631341547005,-9.07343113870902));
#53062=CARTESIAN_POINT('Ctrl Pts',(-50.,-11.9725570665522,-7.37643433768309));
#53063=CARTESIAN_POINT('Ctrl Pts',(-50.,-11.9898382395678,-7.38636816850343));
#53064=CARTESIAN_POINT('Ctrl Pts',(-50.,-12.0243448058902,-7.40633747762124));
#53065=CARTESIAN_POINT('Ctrl Pts',(-50.,-12.0759373202474,-7.43659637822836));
#53066=CARTESIAN_POINT('Ctrl Pts',(-50.,-12.144392189705,-7.47755231121817));
#53067=CARTESIAN_POINT('Ctrl Pts',(-50.,-12.2293754395952,-7.5298019490105));
#53068=CARTESIAN_POINT('Ctrl Pts',(-50.,-12.3136968468978,-7.58320962985052));
#53069=CARTESIAN_POINT('Ctrl Pts',(-50.,-12.3972076624386,-7.63797459554787));
#53070=CARTESIAN_POINT('Ctrl Pts',(-50.,-12.4796599881192,-7.69442745995809));
#53071=CARTESIAN_POINT('Ctrl Pts',(-50.,-12.5606910950408,-7.75305023703025));
#53072=CARTESIAN_POINT('Ctrl Pts',(-50.,-12.6399013181197,-7.81436828334278));
#53073=CARTESIAN_POINT('Ctrl Pts',(-50.,-12.7169258039014,-7.87885048806616));
#53074=CARTESIAN_POINT('Ctrl Pts',(-50.,-12.7915043783298,-7.9468122624453));
#53075=CARTESIAN_POINT('Ctrl Pts',(-50.,-12.8635635126628,-8.01830125100551));
#53076=CARTESIAN_POINT('Ctrl Pts',(-50.,-12.9332619666045,-8.09303464904925));
#53077=CARTESIAN_POINT('Ctrl Pts',(-50.,-13.0008947798771,-8.17053759353955));
#53078=CARTESIAN_POINT('Ctrl Pts',(-50.,-13.0668177956572,-8.25025250675973));
#53079=CARTESIAN_POINT('Ctrl Pts',(-50.,-13.1313692681049,-8.3316524092927));
#53080=CARTESIAN_POINT('Ctrl Pts',(-50.,-13.1947825037901,-8.41436747482742));
#53081=CARTESIAN_POINT('Ctrl Pts',(-50.,-13.2571352386615,-8.49825805316535));
#53082=CARTESIAN_POINT('Ctrl Pts',(-50.,-13.3184076369901,-8.58332951829382));
#53083=CARTESIAN_POINT('Ctrl Pts',(-50.,-13.3785211625712,-8.66967501744431));
#53084=CARTESIAN_POINT('Ctrl Pts',(-50.,-13.4373825330349,-8.7574108514811));
#53085=CARTESIAN_POINT('Ctrl Pts',(-50.,-13.4949307609898,-8.84660742136017));
#53086=CARTESIAN_POINT('Ctrl Pts',(-50.,-13.5452274539844,-8.92767411535463));
#53087=CARTESIAN_POINT('Ctrl Pts',(-50.,-13.5835081010849,-8.99143908805054));
#53088=CARTESIAN_POINT('Ctrl Pts',(-50.,-13.6103880199559,-9.03723101235338));
#53089=CARTESIAN_POINT('Ctrl Pts',(-50.,-13.6262642776339,-9.06463189014802));
#53090=CARTESIAN_POINT('Ctrl Pts',(-50.,-13.631341547005,-9.07343113870902));
#53091=CARTESIAN_POINT('',(-50.,-12.8332528856473,-10.1709510554827));
#53092=CARTESIAN_POINT('Origin',(-50.,0.,0.));
#53093=CARTESIAN_POINT('',(-50.,-10.7151295435653,-9.10713484662511));
#53094=CARTESIAN_POINT('Ctrl Pts',(-50.,-12.8332528856473,-10.1709510554827));
#53095=CARTESIAN_POINT('Ctrl Pts',(-50.,-12.8327903946759,-10.1708755197597));
#53096=CARTESIAN_POINT('Ctrl Pts',(-50.,-12.8064341089476,-10.166560387824));
#53097=CARTESIAN_POINT('Ctrl Pts',(-50.,-12.7552356183835,-10.1569883822946));
#53098=CARTESIAN_POINT('Ctrl Pts',(-50.,-12.6816996681717,-10.1397240556283));
#53099=CARTESIAN_POINT('Ctrl Pts',(-50.,-12.5886768226797,-10.1118497354652));
#53100=CARTESIAN_POINT('Ctrl Pts',(-50.,-12.4762474639872,-10.0731133520306));
#53101=CARTESIAN_POINT('Ctrl Pts',(-50.,-12.362689281313,-10.0341575556064));
#53102=CARTESIAN_POINT('Ctrl Pts',(-50.,-12.2462767052779,-9.99652743122885));
#53103=CARTESIAN_POINT('Ctrl Pts',(-50.,-12.1276136395118,-9.95979777888845));
#53104=CARTESIAN_POINT('Ctrl Pts',(-50.,-12.0085066122796,-9.9224850258725));
#53105=CARTESIAN_POINT('Ctrl Pts',(-50.,-11.8911649899478,-9.88269332242761));
#53106=CARTESIAN_POINT('Ctrl Pts',(-50.,-11.7770967670118,-9.83899640572359));
#53107=CARTESIAN_POINT('Ctrl Pts',(-50.,-11.6668507136929,-9.79068450718227));
#53108=CARTESIAN_POINT('Ctrl Pts',(-50.,-11.5604070517922,-9.73753381300202));
#53109=CARTESIAN_POINT('Ctrl Pts',(-50.,-11.4573709649815,-9.6797149094218));
#53110=CARTESIAN_POINT('Ctrl Pts',(-50.,-11.3572701125446,-9.61764250849074));
#53111=CARTESIAN_POINT('Ctrl Pts',(-50.,-11.2597201712738,-9.55186779486609));
#53112=CARTESIAN_POINT('Ctrl Pts',(-50.,-11.1643982983724,-9.48299554522798));
#53113=CARTESIAN_POINT('Ctrl Pts',(-50.,-11.0710535306934,-9.4116019360644));
#53114=CARTESIAN_POINT('Ctrl Pts',(-50.,-10.9795035237476,-9.33814591637203));
#53115=CARTESIAN_POINT('Ctrl Pts',(-50.,-10.889634916681,-9.26290188705335));
#53116=CARTESIAN_POINT('Ctrl Pts',(-50.,-10.8190356624814,-9.20139120553108));
#53117=CARTESIAN_POINT('Ctrl Pts',(-50.,-10.7668038881397,-9.15454138381928));
#53118=CARTESIAN_POINT('Ctrl Pts',(-50.,-10.7323012362688,-9.12299004745485));
#53119=CARTESIAN_POINT('Ctrl Pts',(-50.,-10.7151295435653,-9.10713484662511));
#53120=CARTESIAN_POINT('',(-50.,-9.76197254719673,-10.1221439546065));
#53121=CARTESIAN_POINT('Origin',(-50.,0.,0.));
#53122=CARTESIAN_POINT('',(-50.,-10.9466173199385,-12.178349405844));
#53123=CARTESIAN_POINT('Ctrl Pts',(-50.,-9.76197254719672,-10.1221439546065));
#53124=CARTESIAN_POINT('Ctrl Pts',(-50.,-9.77624035711837,-10.1360633488319));
#53125=CARTESIAN_POINT('Ctrl Pts',(-50.,-9.80469667097528,-10.163986719468));
#53126=CARTESIAN_POINT('Ctrl Pts',(-50.,-9.84714322904426,-10.2061255176443));
#53127=CARTESIAN_POINT('Ctrl Pts',(-50.,-9.90326213654415,-10.2628187784479));
#53128=CARTESIAN_POINT('Ctrl Pts',(-50.,-9.97258152483879,-10.3345613726147));
#53129=CARTESIAN_POINT('Ctrl Pts',(-50.,-10.0409718699529,-10.4072610342189));
#53130=CARTESIAN_POINT('Ctrl Pts',(-50.,-10.108239546518,-10.4810737531071));
#53131=CARTESIAN_POINT('Ctrl Pts',(-50.,-10.1740622242879,-10.5562581065423));
#53132=CARTESIAN_POINT('Ctrl Pts',(-50.,-10.2379686981643,-10.6331907581101));
#53133=CARTESIAN_POINT('Ctrl Pts',(-50.,-10.2994412084092,-10.7122811666816));
#53134=CARTESIAN_POINT('Ctrl Pts',(-50.,-10.3580097561152,-10.7938927550471));
#53135=CARTESIAN_POINT('Ctrl Pts',(-50.,-10.4133439014856,-10.8782663225706));
#53136=CARTESIAN_POINT('Ctrl Pts',(-50.,-10.4653605771075,-10.9654297310826));
#53137=CARTESIAN_POINT('Ctrl Pts',(-50.,-10.5142838856252,-11.055148542648));
#53138=CARTESIAN_POINT('Ctrl Pts',(-50.,-10.5605176911805,-11.1470361863206));
#53139=CARTESIAN_POINT('Ctrl Pts',(-50.,-10.6045453214218,-11.2406410963124));
#53140=CARTESIAN_POINT('Ctrl Pts',(-50.,-10.6468254580846,-11.3355369696227));
#53141=CARTESIAN_POINT('Ctrl Pts',(-50.,-10.6876760500473,-11.4314236196986));
#53142=CARTESIAN_POINT('Ctrl Pts',(-50.,-10.727207120633,-11.5281851158537));
#53143=CARTESIAN_POINT('Ctrl Pts',(-50.,-10.7653981208323,-11.6258217302963));
#53144=CARTESIAN_POINT('Ctrl Pts',(-50.,-10.8021498170253,-11.7244041527066));
#53145=CARTESIAN_POINT('Ctrl Pts',(-50.,-10.8373429346305,-11.8240218317612));
#53146=CARTESIAN_POINT('Ctrl Pts',(-50.,-10.8709008942817,-11.9247277896931));
#53147=CARTESIAN_POINT('Ctrl Pts',(-50.,-10.8994569571944,-12.0157559033301));
#53148=CARTESIAN_POINT('Ctrl Pts',(-50.,-10.9206772435082,-12.0870375919612));
#53149=CARTESIAN_POINT('Ctrl Pts',(-50.,-10.9353246918112,-12.1380756427477));
#53150=CARTESIAN_POINT('Ctrl Pts',(-50.,-10.9438878464529,-12.1685639363102));
#53151=CARTESIAN_POINT('Ctrl Pts',(-50.,-10.9466173199385,-12.178349405844));
#53152=CARTESIAN_POINT('',(-50.,-9.90065997719615,-13.0429121370937));
#53153=CARTESIAN_POINT('Origin',(-50.,0.,0.));
#53154=CARTESIAN_POINT('',(-50.,-8.11364170780698,-11.4857618157149));
#53155=CARTESIAN_POINT('Ctrl Pts',(-50.,-9.90065997719615,-13.0429121370937));
#53156=CARTESIAN_POINT('Ctrl Pts',(-50.,-9.90023080119949,-13.0427239576368));
#53157=CARTESIAN_POINT('Ctrl Pts',(-50.,-9.87577567632734,-13.031989851782));
#53158=CARTESIAN_POINT('Ctrl Pts',(-50.,-9.82856614146686,-13.0099860215666));
#53159=CARTESIAN_POINT('Ctrl Pts',(-50.,-9.76163392180467,-12.9749764383087));
#53160=CARTESIAN_POINT('Ctrl Pts',(-50.,-9.67846562159703,-12.9248440002217));
#53161=CARTESIAN_POINT('Ctrl Pts',(-50.,-9.57920178477654,-12.8593645469766));
#53162=CARTESIAN_POINT('Ctrl Pts',(-50.,-9.47889915384706,-12.7933918468958));
#53163=CARTESIAN_POINT('Ctrl Pts',(-50.,-9.37550212434126,-12.7279933116739));
#53164=CARTESIAN_POINT('Ctrl Pts',(-50.,-9.26970137008846,-12.6629072844668));
#53165=CARTESIAN_POINT('Ctrl Pts',(-50.,-9.16361561347667,-12.5971460670373));
#53166=CARTESIAN_POINT('Ctrl Pts',(-50.,-9.05985628822634,-12.5294228183105));
#53167=CARTESIAN_POINT('Ctrl Pts',(-50.,-8.96023870955522,-12.4587311071067));
#53168=CARTESIAN_POINT('Ctrl Pts',(-50.,-8.86547091932666,-12.3845199371372));
#53169=CARTESIAN_POINT('Ctrl Pts',(-50.,-8.77558942093922,-12.3065676074844));
#53170=CARTESIAN_POINT('Ctrl Pts',(-50.,-8.69016937887314,-12.2249411582788));
#53171=CARTESIAN_POINT('Ctrl Pts',(-50.,-8.60865015717173,-12.1399248062686));
#53172=CARTESIAN_POINT('Ctrl Pts',(-50.,-8.53052243279731,-12.0519568423361));
#53173=CARTESIAN_POINT('Ctrl Pts',(-50.,-8.45532310380908,-11.9615427552514));
#53174=CARTESIAN_POINT('Ctrl Pts',(-50.,-8.3826658022629,-11.8691782078618));
#53175=CARTESIAN_POINT('Ctrl Pts',(-50.,-8.3122597763829,-11.775262383207));
#53176=CARTESIAN_POINT('Ctrl Pts',(-50.,-8.24392698602517,-11.6800328696824));
#53177=CARTESIAN_POINT('Ctrl Pts',(-50.,-8.19084282166638,-11.6028973387695));
#53178=CARTESIAN_POINT('Ctrl Pts',(-50.,-8.15190308143842,-11.5445298762901));
#53179=CARTESIAN_POINT('Ctrl Pts',(-50.,-8.12633089210227,-11.5053893225758));
#53180=CARTESIAN_POINT('Ctrl Pts',(-50.,-8.11364170780698,-11.4857618157149));
#53181=CARTESIAN_POINT('',(-50.,-6.93800739067722,-12.2318420402206));
#53182=CARTESIAN_POINT('Origin',(-50.,0.,0.));
#53183=CARTESIAN_POINT('',(-50.,-7.57407686781798,-14.5180571909737));
#53184=CARTESIAN_POINT('Ctrl Pts',(-50.,-6.93800739067721,-12.2318420402206));
#53185=CARTESIAN_POINT('Ctrl Pts',(-50.,-6.94836533853418,-12.24887239112));
#53186=CARTESIAN_POINT('Ctrl Pts',(-50.,-6.96898338507103,-12.2829952952022));
#53187=CARTESIAN_POINT('Ctrl Pts',(-50.,-6.99961691350077,-12.3343662552827));
#53188=CARTESIAN_POINT('Ctrl Pts',(-50.,-7.03987370169386,-12.4032345978205));
#53189=CARTESIAN_POINT('Ctrl Pts',(-50.,-7.08917363628753,-12.4899622973194));
#53190=CARTESIAN_POINT('Ctrl Pts',(-50.,-7.13733570230759,-12.5773859525787));
#53191=CARTESIAN_POINT('Ctrl Pts',(-50.,-7.18413356438513,-12.6656085000656));
#53192=CARTESIAN_POINT('Ctrl Pts',(-50.,-7.22919071332107,-12.7548002330908));
#53193=CARTESIAN_POINT('Ctrl Pts',(-50.,-7.27195707536722,-12.8452087977179));
#53194=CARTESIAN_POINT('Ctrl Pts',(-50.,-7.31182932887926,-12.9371020273035));
#53195=CARTESIAN_POINT('Ctrl Pts',(-50.,-7.34826186125705,-13.0307150430677));
#53196=CARTESIAN_POINT('Ctrl Pts',(-50.,-7.38087472971119,-13.1261989021839));
#53197=CARTESIAN_POINT('Ctrl Pts',(-50.,-7.40958054758866,-13.2235599331263));
#53198=CARTESIAN_POINT('Ctrl Pts',(-50.,-7.43465467928082,-13.32262679532));
#53199=CARTESIAN_POINT('Ctrl Pts',(-50.,-7.45658443707985,-13.4231254995838));
#53200=CARTESIAN_POINT('Ctrl Pts',(-50.,-7.47595026385202,-13.5247388655977));
#53201=CARTESIAN_POINT('Ctrl Pts',(-50.,-7.49330244824787,-13.6271680529626));
#53202=CARTESIAN_POINT('Ctrl Pts',(-50.,-7.50902360355704,-13.730201376709));
#53203=CARTESIAN_POINT('Ctrl Pts',(-50.,-7.52324912730704,-13.8337539100138));
#53204=CARTESIAN_POINT('Ctrl Pts',(-50.,-7.53595904837785,-13.9378208062029));
#53205=CARTESIAN_POINT('Ctrl Pts',(-50.,-7.54703967094767,-14.0424458557121));
#53206=CARTESIAN_POINT('Ctrl Pts',(-50.,-7.556353222684,-14.1476860346413));
#53207=CARTESIAN_POINT('Ctrl Pts',(-50.,-7.56381234400904,-14.2535736549186));
#53208=CARTESIAN_POINT('Ctrl Pts',(-50.,-7.56883349438523,-14.3488435570404));
#53209=CARTESIAN_POINT('Ctrl Pts',(-50.,-7.57166007128053,-14.4231630709543));
#53210=CARTESIAN_POINT('Ctrl Pts',(-50.,-7.57315469596912,-14.4762403397886));
#53211=CARTESIAN_POINT('Ctrl Pts',(-50.,-7.57386669307527,-14.5079003575064));
#53212=CARTESIAN_POINT('Ctrl Pts',(-50.,-7.57407686781798,-14.5180571909737));
#53213=CARTESIAN_POINT('',(-50.,-6.34597219029741,-15.0953390806557));
#53214=CARTESIAN_POINT('Origin',(-50.,0.,0.));
#53215=CARTESIAN_POINT('',(-50.,-5.00234392366024,-13.1426961282463));
#53216=CARTESIAN_POINT('Ctrl Pts',(-50.,-6.34597219029741,-15.0953390806557));
#53217=CARTESIAN_POINT('Ctrl Pts',(-50.,-6.34560329598179,-15.0950500814723));
#53218=CARTESIAN_POINT('Ctrl Pts',(-50.,-6.32458593740117,-15.0785714650465));
#53219=CARTESIAN_POINT('Ctrl Pts',(-50.,-6.28433170694406,-15.045518391722));
#53220=CARTESIAN_POINT('Ctrl Pts',(-50.,-6.22820881535241,-14.9949633327447));
#53221=CARTESIAN_POINT('Ctrl Pts',(-50.,-6.16012083060275,-14.925722782193));
#53222=CARTESIAN_POINT('Ctrl Pts',(-50.,-6.08025962758854,-14.8376145740015));
#53223=CARTESIAN_POINT('Ctrl Pts',(-50.,-5.99951493159239,-14.7487702776409));
#53224=CARTESIAN_POINT('Ctrl Pts',(-50.,-5.91563026424745,-14.6597125620614));
#53225=CARTESIAN_POINT('Ctrl Pts',(-50.,-5.8293396720056,-14.5703597544468));
#53226=CARTESIAN_POINT('Ctrl Pts',(-50.,-5.7429409442582,-14.4802820917477));
#53227=CARTESIAN_POINT('Ctrl Pts',(-50.,-5.65928349609497,-14.3888825985252));
#53228=CARTESIAN_POINT('Ctrl Pts',(-50.,-5.58037590052447,-14.2956379130225));
#53229=CARTESIAN_POINT('Ctrl Pts',(-50.,-5.50704098217782,-14.2001904323636));
#53230=CARTESIAN_POINT('Ctrl Pts',(-50.,-5.43936923240832,-14.102334498799));
#53231=CARTESIAN_POINT('Ctrl Pts',(-50.,-5.37693249048282,-14.0020293939727));
#53232=CARTESIAN_POINT('Ctrl Pts',(-50.,-5.31911705202313,-13.8994109809482));
#53233=CARTESIAN_POINT('Ctrl Pts',(-50.,-5.26532059680125,-13.7947771174053));
#53234=CARTESIAN_POINT('Ctrl Pts',(-50.,-5.21496886213029,-13.6885022424853));
#53235=CARTESIAN_POINT('Ctrl Pts',(-50.,-5.16756435218796,-13.5809703610753));
#53236=CARTESIAN_POINT('Ctrl Pts',(-50.,-5.12272617691501,-13.4724958081193));
#53237=CARTESIAN_POINT('Ctrl Pts',(-50.,-5.08022280379478,-13.3632644309532));
#53238=CARTESIAN_POINT('Ctrl Pts',(-50.,-5.04798920255339,-13.2753507597416));
#53239=CARTESIAN_POINT('Ctrl Pts',(-50.,-5.02478822352796,-13.2091330988228));
#53240=CARTESIAN_POINT('Ctrl Pts',(-50.,-5.00975329143057,-13.1648626726972));
#53241=CARTESIAN_POINT('Ctrl Pts',(-50.,-5.00234392366024,-13.1426961282463));
#53242=CARTESIAN_POINT('',(-50.,-3.67810171359515,-13.5729685048794));
#53243=CARTESIAN_POINT('Origin',(-50.,0.,0.));
#53244=CARTESIAN_POINT('',(-50.,-3.7256293105862,-15.9455420491152));
#53245=CARTESIAN_POINT('Ctrl Pts',(-50.,-3.67810171359514,-13.5729685048794));
#53246=CARTESIAN_POINT('Ctrl Pts',(-50.,-3.68389897142971,-13.5920397328724));
#53247=CARTESIAN_POINT('Ctrl Pts',(-50.,-3.69538324295473,-13.6302181028421));
#53248=CARTESIAN_POINT('Ctrl Pts',(-50.,-3.71227892449176,-13.6875933984758));
#53249=CARTESIAN_POINT('Ctrl Pts',(-50.,-3.73414411132176,-13.764309571506));
#53250=CARTESIAN_POINT('Ctrl Pts',(-50.,-3.76032689601146,-13.8605729560155));
#53251=CARTESIAN_POINT('Ctrl Pts',(-50.,-3.7852344832017,-13.9572274551481));
#53252=CARTESIAN_POINT('Ctrl Pts',(-50.,-3.8086220490069,-14.0543164841154));
#53253=CARTESIAN_POINT('Ctrl Pts',(-50.,-3.83008256273264,-14.1519113521203));
#53254=CARTESIAN_POINT('Ctrl Pts',(-50.,-3.84902164513744,-14.2501151271916));
#53255=CARTESIAN_POINT('Ctrl Pts',(-50.,-3.86478832158859,-14.3490371882169));
#53256=CARTESIAN_POINT('Ctrl Pts',(-50.,-3.87679564863944,-14.4487695813147));
#53257=CARTESIAN_POINT('Ctrl Pts',(-50.,-3.88463805371054,-14.5493641299902));
#53258=CARTESIAN_POINT('Ctrl Pts',(-50.,-3.88822932173376,-14.6508052317201));
#53259=CARTESIAN_POINT('Ctrl Pts',(-50.,-3.88787877668998,-14.7529954092481));
#53260=CARTESIAN_POINT('Ctrl Pts',(-50.,-3.88412655939816,-14.8557904709058));
#53261=CARTESIAN_POINT('Ctrl Pts',(-50.,-3.87761375658259,-14.9590275514473));
#53262=CARTESIAN_POINT('Ctrl Pts',(-50.,-3.86894768714904,-15.0625540503165));
#53263=CARTESIAN_POINT('Ctrl Pts',(-50.,-3.85855158779829,-15.1662600850723));
#53264=CARTESIAN_POINT('Ctrl Pts',(-50.,-3.84657772273756,-15.2700970690198));
#53265=CARTESIAN_POINT('Ctrl Pts',(-50.,-3.83300795359517,-15.3740553411364));
#53266=CARTESIAN_POINT('Ctrl Pts',(-50.,-3.81772126627406,-15.4781490410999));
#53267=CARTESIAN_POINT('Ctrl Pts',(-50.,-3.80057004743305,-15.5823990924153));
#53268=CARTESIAN_POINT('Ctrl Pts',(-50.,-3.78146164640637,-15.6868150664286));
#53269=CARTESIAN_POINT('Ctrl Pts',(-50.,-3.76263238690138,-15.7803405987066));
#53270=CARTESIAN_POINT('Ctrl Pts',(-50.,-3.74688765015641,-15.853028169516));
#53271=CARTESIAN_POINT('Ctrl Pts',(-50.,-3.73513553846456,-15.9048096163928));
#53272=CARTESIAN_POINT('Ctrl Pts',(-50.,-3.72795164063846,-15.9356520429153));
#53273=CARTESIAN_POINT('Ctrl Pts',(-50.,-3.7256293105862,-15.9455420491152));
#53274=CARTESIAN_POINT('',(-50.,-2.39254363182917,-16.1992703530064));
#53275=CARTESIAN_POINT('Origin',(-50.,0.,0.));
#53276=CARTESIAN_POINT('',(-50.,-1.57673047345591,-13.9738265075847));
#53277=CARTESIAN_POINT('Ctrl Pts',(-50.,-2.39254363182917,-16.1992703530064));
#53278=CARTESIAN_POINT('Ctrl Pts',(-50.,-2.39225819818113,-16.1988986929781));
#53279=CARTESIAN_POINT('Ctrl Pts',(-50.,-2.37599920382811,-16.1777109780555));
#53280=CARTESIAN_POINT('Ctrl Pts',(-50.,-2.34522959911868,-16.1356855077795));
#53281=CARTESIAN_POINT('Ctrl Pts',(-50.,-2.30344244328183,-16.0727615333669));
#53282=CARTESIAN_POINT('Ctrl Pts',(-50.,-2.25471299248206,-15.9887635087906));
#53283=CARTESIAN_POINT('Ctrl Pts',(-50.,-2.19927239636847,-15.8835627084126));
#53284=CARTESIAN_POINT('Ctrl Pts',(-50.,-2.14315912151332,-15.777429229659));
#53285=CARTESIAN_POINT('Ctrl Pts',(-50.,-2.08405759848474,-15.6703081575233));
#53286=CARTESIAN_POINT('Ctrl Pts',(-50.,-2.02269912351901,-15.5623029350202));
#53287=CARTESIAN_POINT('Ctrl Pts',(-50.,-1.96141617445265,-15.4535687378813));
#53288=CARTESIAN_POINT('Ctrl Pts',(-50.,-1.90311710851519,-15.3442359664661));
#53289=CARTESIAN_POINT('Ctrl Pts',(-50.,-1.84987755047685,-15.2342972131845));
#53290=CARTESIAN_POINT('Ctrl Pts',(-50.,-1.80258340663877,-15.1236107380773));
#53291=CARTESIAN_POINT('Ctrl Pts',(-50.,-1.76137347040452,-15.0119998487957));
#53292=CARTESIAN_POINT('Ctrl Pts',(-50.,-1.72584315874106,-14.8993186269813));
#53293=CARTESIAN_POINT('Ctrl Pts',(-50.,-1.69536426015181,-14.7855460452371));
#53294=CARTESIAN_POINT('Ctrl Pts',(-50.,-1.6692793032136,-14.6708208125467));
#53295=CARTESIAN_POINT('Ctrl Pts',(-50.,-1.64693894753001,-14.5553627910342));
#53296=CARTESIAN_POINT('Ctrl Pts',(-50.,-1.6277658288928,-14.4394201991873));
#53297=CARTESIAN_POINT('Ctrl Pts',(-50.,-1.61131285168258,-14.3232027730338));
#53298=CARTESIAN_POINT('Ctrl Pts',(-50.,-1.59730953904946,-14.2068329413785));
#53299=CARTESIAN_POINT('Ctrl Pts',(-50.,-1.58795185663835,-14.1136650691543));
#53300=CARTESIAN_POINT('Ctrl Pts',(-50.,-1.58194744165485,-14.0437579089631));
#53301=CARTESIAN_POINT('Ctrl Pts',(-50.,-1.57839446687451,-13.997139284115));
#53302=CARTESIAN_POINT('Ctrl Pts',(-50.,-1.57673047345591,-13.9738265075847));
#53303=CARTESIAN_POINT('',(-50.,-0.187087378736044,-14.0612554404903));
#53304=CARTESIAN_POINT('Origin',(-50.,0.,0.));
#53305=CARTESIAN_POINT('',(-50.,0.356913238135828,-16.3711098567093));
#53306=CARTESIAN_POINT('Ctrl Pts',(-50.,-0.187087378736032,-14.0612554404903));
#53307=CARTESIAN_POINT('Ctrl Pts',(-50.,-0.187959683517641,-14.0811692301831));
#53308=CARTESIAN_POINT('Ctrl Pts',(-50.,-0.189588581014708,-14.1210041786448));
#53309=CARTESIAN_POINT('Ctrl Pts',(-50.,-0.191684797850075,-14.1807787089954));
#53310=CARTESIAN_POINT('Ctrl Pts',(-50.,-0.193784513213942,-14.2605223532243));
#53311=CARTESIAN_POINT('Ctrl Pts',(-50.,-0.195204987344071,-14.3602728402636));
#53312=CARTESIAN_POINT('Ctrl Pts',(-50.,-0.195293060397626,-14.4600850256186));
#53313=CARTESIAN_POINT('Ctrl Pts',(-50.,-0.19380080315749,-14.5599400753078));
#53314=CARTESIAN_POINT('Ctrl Pts',(-50.,-0.190316238669402,-14.6598058338069));
#53315=CARTESIAN_POINT('Ctrl Pts',(-50.,-0.184238029232279,-14.7596343149665));
#53316=CARTESIAN_POINT('Ctrl Pts',(-50.,-0.174908450355344,-14.8593695705273));
#53317=CARTESIAN_POINT('Ctrl Pts',(-50.,-0.161736107560775,-14.9589547879103));
#53318=CARTESIAN_POINT('Ctrl Pts',(-50.,-0.144315282095873,-15.058339300691));
#53319=CARTESIAN_POINT('Ctrl Pts',(-50.,-0.122566347687195,-15.1574865557124));
#53320=CARTESIAN_POINT('Ctrl Pts',(-50.,-0.0968131519417803,-15.2563790638913));
#53321=CARTESIAN_POINT('Ctrl Pts',(-50.,-0.0676147251712506,-15.3550114911653));
#53322=CARTESIAN_POINT('Ctrl Pts',(-50.,-0.0356325161212601,-15.4533855207845));
#53323=CARTESIAN_POINT('Ctrl Pts',(-50.,-0.00149271387238248,-15.5515043804903));
#53324=CARTESIAN_POINT('Ctrl Pts',(-50.,0.0343674149818962,-15.6493668946876));
#53325=CARTESIAN_POINT('Ctrl Pts',(-50.,0.0717883068748032,-15.7469638696907));
#53326=CARTESIAN_POINT('Ctrl Pts',(-50.,0.110785127729046,-15.844281437166));
#53327=CARTESIAN_POINT('Ctrl Pts',(-50.,0.151478606156202,-15.9413031975852));
#53328=CARTESIAN_POINT('Ctrl Pts',(-50.,0.194016921417006,-16.0380127071578));
#53329=CARTESIAN_POINT('Ctrl Pts',(-50.,0.238492193683111,-16.1343961952447));
#53330=CARTESIAN_POINT('Ctrl Pts',(-50.,0.279988751445404,-16.220300804523));
#53331=CARTESIAN_POINT('Ctrl Pts',(-50.,0.313315502115871,-16.2867892048278));
#53332=CARTESIAN_POINT('Ctrl Pts',(-50.,0.337575921789304,-16.3340212110009));
#53333=CARTESIAN_POINT('Ctrl Pts',(-50.,0.352204323826718,-16.3621081032393));
#53334=CARTESIAN_POINT('Ctrl Pts',(-50.,0.356913238135828,-16.3711098567093));
#53335=CARTESIAN_POINT('',(-50.,1.71121724218688,-16.2853418923289));
#53336=CARTESIAN_POINT('Origin',(-50.,0.,0.));
#53337=CARTESIAN_POINT('',(-50.,1.94795475120472,-13.9269299753125));
#53338=CARTESIAN_POINT('Ctrl Pts',(-50.,1.71121724218688,-16.2853418923289));
#53339=CARTESIAN_POINT('Ctrl Pts',(-50.,1.71140128032148,-16.284910924222));
#53340=CARTESIAN_POINT('Ctrl Pts',(-50.,1.72188029803531,-16.2603454128541));
#53341=CARTESIAN_POINT('Ctrl Pts',(-50.,1.74123190957046,-16.211988160483));
#53342=CARTESIAN_POINT('Ctrl Pts',(-50.,1.76605768896888,-16.1406490153657));
#53343=CARTESIAN_POINT('Ctrl Pts',(-50.,1.79236675521062,-16.047171421572));
#53344=CARTESIAN_POINT('Ctrl Pts',(-50.,1.81990320787353,-15.9314881821968));
#53345=CARTESIAN_POINT('Ctrl Pts',(-50.,1.84785925815835,-15.8147342778518));
#53346=CARTESIAN_POINT('Ctrl Pts',(-50.,1.87846407081847,-15.6962806600859));
#53347=CARTESIAN_POINT('Ctrl Pts',(-50.,1.91103504986532,-15.5764093880396));
#53348=CARTESIAN_POINT('Ctrl Pts',(-50.,1.94335158717786,-15.4558508259636));
#53349=CARTESIAN_POINT('Ctrl Pts',(-50.,1.97262912616775,-15.3354545564815));
#53350=CARTESIAN_POINT('Ctrl Pts',(-50.,1.99685540944097,-15.2157295916163));
#53351=CARTESIAN_POINT('Ctrl Pts',(-50.,2.01513711377743,-15.096758960368));
#53352=CARTESIAN_POINT('Ctrl Pts',(-50.,2.02729586462329,-14.9784060380191));
#53353=CARTESIAN_POINT('Ctrl Pts',(-50.,2.03368724587156,-14.8604288747958));
#53354=CARTESIAN_POINT('Ctrl Pts',(-50.,2.03491450329845,-14.7426508740692));
#53355=CARTESIAN_POINT('Ctrl Pts',(-50.,2.03164894817481,-14.625042880531));
#53356=CARTESIAN_POINT('Ctrl Pts',(-50.,2.02457419816135,-14.5076563645426));
#53357=CARTESIAN_POINT('Ctrl Pts',(-50.,2.01431120793567,-14.3905881617116));
#53358=CARTESIAN_POINT('Ctrl Pts',(-50.,2.00134518601523,-14.2739302306637));
#53359=CARTESIAN_POINT('Ctrl Pts',(-50.,1.98596855852791,-14.1577338890203));
#53360=CARTESIAN_POINT('Ctrl Pts',(-50.,1.9718623445077,-14.0651658958429));
#53361=CARTESIAN_POINT('Ctrl Pts',(-50.,1.96029291597316,-13.9959617603545));
#53362=CARTESIAN_POINT('Ctrl Pts',(-50.,1.95214068696407,-13.9499241564345));
#53363=CARTESIAN_POINT('Ctrl Pts',(-50.,1.94795475120472,-13.9269299753125));
#53364=CARTESIAN_POINT('',(-50.,3.31568234418831,-13.6660219830951));
#53365=CARTESIAN_POINT('Origin',(-50.,0.,0.));
#53366=CARTESIAN_POINT('',(-50.,4.41702961547073,-15.7680206232759));
#53367=CARTESIAN_POINT('Ctrl Pts',(-50.,3.31568234418832,-13.6660219830951));
#53368=CARTESIAN_POINT('Ctrl Pts',(-50.,3.31978980257722,-13.6855270778435));
#53369=CARTESIAN_POINT('Ctrl Pts',(-50.,3.3281186287285,-13.7245156284827));
#53370=CARTESIAN_POINT('Ctrl Pts',(-50.,3.34095358960791,-13.7829335399729));
#53371=CARTESIAN_POINT('Ctrl Pts',(-50.,3.35875127854871,-13.860694068957));
#53372=CARTESIAN_POINT('Ctrl Pts',(-50.,3.38218236859189,-13.9576639685687));
#53373=CARTESIAN_POINT('Ctrl Pts',(-50.,3.40691934362888,-14.0543622734568));
#53374=CARTESIAN_POINT('Ctrl Pts',(-50.,3.43319765990381,-14.1507090838548));
#53375=CARTESIAN_POINT('Ctrl Pts',(-50.,3.46140835460361,-14.246570799961));
#53376=CARTESIAN_POINT('Ctrl Pts',(-50.,3.49212193962963,-14.3417513965941));
#53377=CARTESIAN_POINT('Ctrl Pts',(-50.,3.52596156208203,-14.436033113783));
#53378=CARTESIAN_POINT('Ctrl Pts',(-50.,3.56348590797974,-14.5292138499942));
#53379=CARTESIAN_POINT('Ctrl Pts',(-50.,3.60507534944737,-14.6211436324314));
#53380=CARTESIAN_POINT('Ctrl Pts',(-50.,3.65079792075207,-14.7117672540732));
#53381=CARTESIAN_POINT('Ctrl Pts',(-50.,3.7003355991968,-14.801148312913));
#53382=CARTESIAN_POINT('Ctrl Pts',(-50.,3.75314559090774,-14.8894206676529));
#53383=CARTESIAN_POINT('Ctrl Pts',(-50.,3.80858764637521,-14.9767504442745));
#53384=CARTESIAN_POINT('Ctrl Pts',(-50.,3.8660560521067,-15.0632964960055));
#53385=CARTESIAN_POINT('Ctrl Pts',(-50.,3.92512698668427,-15.1491664279643));
#53386=CARTESIAN_POINT('Ctrl Pts',(-50.,3.98564361314731,-15.2343910171469));
#53387=CARTESIAN_POINT('Ctrl Pts',(-50.,4.04761717203886,-15.3189530593075));
#53388=CARTESIAN_POINT('Ctrl Pts',(-50.,4.11116052066234,-15.4028066461541));
#53389=CARTESIAN_POINT('Ctrl Pts',(-50.,4.17641309355012,-15.4858989998248));
#53390=CARTESIAN_POINT('Ctrl Pts',(-50.,4.24346069213056,-15.5681938729551));
#53391=CARTESIAN_POINT('Ctrl Pts',(-50.,4.30501716681229,-15.6410798566978));
#53392=CARTESIAN_POINT('Ctrl Pts',(-50.,4.35383188909641,-15.6971913757796));
#53393=CARTESIAN_POINT('Ctrl Pts',(-50.,4.38907624535977,-15.736906180594));
#53394=CARTESIAN_POINT('Ctrl Pts',(-50.,4.41022999530898,-15.7604727358124));
#53395=CARTESIAN_POINT('Ctrl Pts',(-50.,4.41702961547073,-15.7680206232759));
#53396=CARTESIAN_POINT('',(-50.,5.70745604345954,-15.3481455072584));
#53397=CARTESIAN_POINT('Origin',(-50.,0.,0.));
#53398=CARTESIAN_POINT('',(-50.,5.35024281477071,-13.004953213026));
#53399=CARTESIAN_POINT('Ctrl Pts',(-50.,5.70745604345954,-15.3481455072584));
#53400=CARTESIAN_POINT('Ctrl Pts',(-50.,5.70752712228785,-15.3476823103842));
#53401=CARTESIAN_POINT('Ctrl Pts',(-50.,5.7115677281404,-15.3212825439959));
#53402=CARTESIAN_POINT('Ctrl Pts',(-50.,5.71828541357827,-15.2696319735416));
#53403=CARTESIAN_POINT('Ctrl Pts',(-50.,5.72458992151582,-15.1943601585744));
#53404=CARTESIAN_POINT('Ctrl Pts',(-50.,5.72682550780959,-15.0972765365679));
#53405=CARTESIAN_POINT('Ctrl Pts',(-50.,5.72472760042901,-14.9783796615786));
#53406=CARTESIAN_POINT('Ctrl Pts',(-50.,5.72276984468895,-14.8583414088431));
#53407=CARTESIAN_POINT('Ctrl Pts',(-50.,5.72295493404455,-14.7359981218931));
#53408=CARTESIAN_POINT('Ctrl Pts',(-50.,5.72469186277131,-14.611792753182));
#53409=CARTESIAN_POINT('Ctrl Pts',(-50.,5.72601142143879,-14.4869849640075));
#53410=CARTESIAN_POINT('Ctrl Pts',(-50.,5.7244278180311,-14.3630901368566));
#53411=CARTESIAN_POINT('Ctrl Pts',(-50.,5.71811860006313,-14.2411017202677));
#53412=CARTESIAN_POINT('Ctrl Pts',(-50.,5.7062391581791,-14.1213222951832));
#53413=CARTESIAN_POINT('Ctrl Pts',(-50.,5.68858274460417,-14.0036638891498));
#53414=CARTESIAN_POINT('Ctrl Pts',(-50.,5.66543360144756,-13.8878037235725));
#53415=CARTESIAN_POINT('Ctrl Pts',(-50.,5.63733210461441,-13.7734207288063));
#53416=CARTESIAN_POINT('Ctrl Pts',(-50.,5.60492122426722,-13.6603197171863));
#53417=CARTESIAN_POINT('Ctrl Pts',(-50.,5.56887590111916,-13.548380533239));
#53418=CARTESIAN_POINT('Ctrl Pts',(-50.,5.52982166345111,-13.4375425451545));
#53419=CARTESIAN_POINT('Ctrl Pts',(-50.,5.48825134524296,-13.3277741560577));
#53420=CARTESIAN_POINT('Ctrl Pts',(-50.,5.44446094769152,-13.2190523479119));
#53421=CARTESIAN_POINT('Ctrl Pts',(-50.,5.40777718254589,-13.1329006212338));
#53422=CARTESIAN_POINT('Ctrl Pts',(-50.,5.37936086023753,-13.0687478607962));
#53423=CARTESIAN_POINT('Ctrl Pts',(-50.,5.36001566196946,-13.026183989773));
#53424=CARTESIAN_POINT('Ctrl Pts',(-50.,5.35024281477071,-13.004953213026));
#53425=CARTESIAN_POINT('',(-50.,6.61011555120063,-12.4121021043889));
#53426=CARTESIAN_POINT('Origin',(-50.,0.,0.));
#53427=CARTESIAN_POINT('',(-50.,8.199607777367,-14.1741686633588));
#53428=CARTESIAN_POINT('Ctrl Pts',(-50.,6.61011555120064,-12.4121021043889));
#53429=CARTESIAN_POINT('Ctrl Pts',(-50.,6.6189446860433,-12.4299729273552));
#53430=CARTESIAN_POINT('Ctrl Pts',(-50.,6.63670790506457,-12.4656652861453));
#53431=CARTESIAN_POINT('Ctrl Pts',(-50.,6.66366757586302,-12.5190559665502));
#53432=CARTESIAN_POINT('Ctrl Pts',(-50.,6.70024437485702,-12.5899474002701));
#53433=CARTESIAN_POINT('Ctrl Pts',(-50.,6.74705476751256,-12.6780437370314));
#53434=CARTESIAN_POINT('Ctrl Pts',(-50.,6.79506247552229,-12.7655522513249));
#53435=CARTESIAN_POINT('Ctrl Pts',(-50.,6.84447568757558,-12.8523369979956));
#53436=CARTESIAN_POINT('Ctrl Pts',(-50.,6.89563993078743,-12.9381713275312));
#53437=CARTESIAN_POINT('Ctrl Pts',(-50.,6.94905904389849,-13.0227234927017));
#53438=CARTESIAN_POINT('Ctrl Pts',(-50.,7.00528244199424,-13.1056276044837));
#53439=CARTESIAN_POINT('Ctrl Pts',(-50.,7.06480099833745,-13.1865489711723));
#53440=CARTESIAN_POINT('Ctrl Pts',(-50.,7.12794583824513,-13.2652477369413));
#53441=CARTESIAN_POINT('Ctrl Pts',(-50.,7.19476912913493,-13.3416535097654));
#53442=CARTESIAN_POINT('Ctrl Pts',(-50.,7.26497865575545,-13.4159069786186));
#53443=CARTESIAN_POINT('Ctrl Pts',(-50.,7.33808196640605,-13.4882727841331));
#53444=CARTESIAN_POINT('Ctrl Pts',(-50.,7.41350024004436,-13.5590710567155));
#53445=CARTESIAN_POINT('Ctrl Pts',(-50.,7.49068629797234,-13.6286062937474));
#53446=CARTESIAN_POINT('Ctrl Pts',(-50.,7.56925639420599,-13.6970881198352));
#53447=CARTESIAN_POINT('Ctrl Pts',(-50.,7.6490662730339,-13.7645853488249));
#53448=CARTESIAN_POINT('Ctrl Pts',(-50.,7.7301225433348,-13.8310785215643));
#53449=CARTESIAN_POINT('Ctrl Pts',(-50.,7.81252309986449,-13.8964951055849));
#53450=CARTESIAN_POINT('Ctrl Pts',(-50.,7.89638987124254,-13.9607493051802));
#53451=CARTESIAN_POINT('Ctrl Pts',(-50.,7.98179694893469,-14.0237846738158));
#53452=CARTESIAN_POINT('Ctrl Pts',(-50.,8.05954552084273,-14.0790723376084));
#53453=CARTESIAN_POINT('Ctrl Pts',(-50.,8.1207810062114,-14.1212812823596));
#53454=CARTESIAN_POINT('Ctrl Pts',(-50.,8.16479476654098,-14.150983458568));
#53455=CARTESIAN_POINT('Ctrl Pts',(-50.,8.19114469649464,-14.1685489034304));
#53456=CARTESIAN_POINT('Ctrl Pts',(-50.,8.199607777367,-14.1741686633588));
#53457=CARTESIAN_POINT('',(-50.,9.34507439096662,-13.4465686934362));
#53458=CARTESIAN_POINT('Origin',(-50.,0.,0.));
#53459=CARTESIAN_POINT('',(-50.,8.41635544546801,-11.2658274114927));
#53460=CARTESIAN_POINT('Ctrl Pts',(-50.,9.34507439096662,-13.4465686934362));
#53461=CARTESIAN_POINT('Ctrl Pts',(-50.,9.34502804434446,-13.4461023721578));
#53462=CARTESIAN_POINT('Ctrl Pts',(-50.,9.3423763522097,-13.4195271451628));
#53463=CARTESIAN_POINT('Ctrl Pts',(-50.,9.33603801466832,-13.3678286519246));
#53464=CARTESIAN_POINT('Ctrl Pts',(-50.,9.32342511572492,-13.293353772072));
#53465=CARTESIAN_POINT('Ctrl Pts',(-50.,9.30144675196197,-13.1987642428721));
#53466=CARTESIAN_POINT('Ctrl Pts',(-50.,9.26984630377419,-13.0841244601964));
#53467=CARTESIAN_POINT('Ctrl Pts',(-50.,9.23809775500251,-12.9683443039596));
#53468=CARTESIAN_POINT('Ctrl Pts',(-50.,9.20785149120868,-12.8497986264917));
#53469=CARTESIAN_POINT('Ctrl Pts',(-50.,9.17864523199547,-12.7290634412273));
#53470=CARTESIAN_POINT('Ctrl Pts',(-50.,9.14888489929381,-12.6078485573591));
#53471=CARTESIAN_POINT('Ctrl Pts',(-50.,9.11653965711474,-12.4882399401825));
#53472=CARTESIAN_POINT('Ctrl Pts',(-50.,9.08009136927418,-12.3716530527263));
#53473=CARTESIAN_POINT('Ctrl Pts',(-50.,9.03879721019277,-12.2585910156016));
#53474=CARTESIAN_POINT('Ctrl Pts',(-50.,8.99243504959771,-12.149020036252));
#53475=CARTESIAN_POINT('Ctrl Pts',(-50.,8.94119992783734,-12.0425567886278));
#53476=CARTESIAN_POINT('Ctrl Pts',(-50.,8.88553539714026,-11.9387559040544));
#53477=CARTESIAN_POINT('Ctrl Pts',(-50.,8.8260156863806,-11.8372684268691));
#53478=CARTESIAN_POINT('Ctrl Pts',(-50.,8.76326465031677,-11.7378101255738));
#53479=CARTESIAN_POINT('Ctrl Pts',(-50.,8.69787308659046,-11.6401667106607));
#53480=CARTESIAN_POINT('Ctrl Pts',(-50.,8.63031048807256,-11.544185015102));
#53481=CARTESIAN_POINT('Ctrl Pts',(-50.,8.56085783218497,-11.4497691315105));
#53482=CARTESIAN_POINT('Ctrl Pts',(-50.,8.50390149179148,-11.3754469011628));
#53483=CARTESIAN_POINT('Ctrl Pts',(-50.,8.46042377774785,-11.3203764696515));
#53484=CARTESIAN_POINT('Ctrl Pts',(-50.,8.43110114017464,-11.2839607760805));
#53485=CARTESIAN_POINT('Ctrl Pts',(-50.,8.41635544546801,-11.2658274114927));
#53486=CARTESIAN_POINT('',(-50.,9.48921088782657,-10.3782842019456));
#53487=CARTESIAN_POINT('Origin',(-50.,0.,0.));
#53488=CARTESIAN_POINT('',(-50.,11.4669744265634,-11.689701557377));
#53489=CARTESIAN_POINT('Ctrl Pts',(-50.,9.48921088782658,-10.3782842019456));
#53490=CARTESIAN_POINT('Ctrl Pts',(-50.,9.50220693210954,-10.3933978635985));
#53491=CARTESIAN_POINT('Ctrl Pts',(-50.,9.52828841562115,-10.4235513483695));
#53492=CARTESIAN_POINT('Ctrl Pts',(-50.,9.56767882107163,-10.4685600648819));
#53493=CARTESIAN_POINT('Ctrl Pts',(-50.,9.62073647531797,-10.5281280338367));
#53494=CARTESIAN_POINT('Ctrl Pts',(-50.,9.68798490145875,-10.6018153909131));
#53495=CARTESIAN_POINT('Ctrl Pts',(-50.,9.75624684158698,-10.6746356328252));
#53496=CARTESIAN_POINT('Ctrl Pts',(-50.,9.82569013557624,-10.7464053109633));
#53497=CARTESIAN_POINT('Ctrl Pts',(-50.,9.89659308973021,-10.816818967327));
#53498=CARTESIAN_POINT('Ctrl Pts',(-50.,9.9693612115878,-10.885429977536));
#53499=CARTESIAN_POINT('Ctrl Pts',(-50.,10.0444356624493,-10.951747313668));
#53500=CARTESIAN_POINT('Ctrl Pts',(-50.,10.1222086594491,-11.0153247237569));
#53501=CARTESIAN_POINT('Ctrl Pts',(-50.,10.2029412752749,-11.0758475399707));
#53502=CARTESIAN_POINT('Ctrl Pts',(-50.,10.2866665326243,-11.1332346082697));
#53503=CARTESIAN_POINT('Ctrl Pts',(-50.,10.3731363846505,-11.1876948686032));
#53504=CARTESIAN_POINT('Ctrl Pts',(-50.,10.4619396643774,-11.2396071151889));
#53505=CARTESIAN_POINT('Ctrl Pts',(-50.,10.5525953486849,-11.289425367888));
#53506=CARTESIAN_POINT('Ctrl Pts',(-50.,10.6446491749193,-11.3375806355454));
#53507=CARTESIAN_POINT('Ctrl Pts',(-50.,10.737781584702,-11.3843713907704));
#53508=CARTESIAN_POINT('Ctrl Pts',(-50.,10.8318699676878,-11.4299001604323));
#53509=CARTESIAN_POINT('Ctrl Pts',(-50.,10.926915885831,-11.4741464531626));
#53510=CARTESIAN_POINT('Ctrl Pts',(-50.,11.0229961202521,-11.5170156697979));
#53511=CARTESIAN_POINT('Ctrl Pts',(-50.,11.1202074324343,-11.5583943876468));
#53512=CARTESIAN_POINT('Ctrl Pts',(-50.,11.2186075484415,-11.5982095077484));
#53513=CARTESIAN_POINT('Ctrl Pts',(-50.,11.3076629888636,-11.632424924341));
#53514=CARTESIAN_POINT('Ctrl Pts',(-50.,11.3774715865628,-11.6580791515292));
#53515=CARTESIAN_POINT('Ctrl Pts',(-50.,11.4274892045258,-11.6759024021635));
#53516=CARTESIAN_POINT('Ctrl Pts',(-50.,11.4573796514766,-11.6863630351679));
#53517=CARTESIAN_POINT('Ctrl Pts',(-50.,11.4669744265634,-11.689701557377));
#53518=CARTESIAN_POINT('',(-50.,12.3955073457098,-10.7000945155851));
#53519=CARTESIAN_POINT('Origin',(-50.,0.,0.));
#53520=CARTESIAN_POINT('',(-50.,10.9536375103364,-8.81882824088046));
#53521=CARTESIAN_POINT('Ctrl Pts',(-50.,12.3955073457098,-10.7000945155851));
#53522=CARTESIAN_POINT('Ctrl Pts',(-50.,12.3953464857659,-10.6996543705834));
#53523=CARTESIAN_POINT('Ctrl Pts',(-50.,12.3861691112129,-10.6745735022306));
#53524=CARTESIAN_POINT('Ctrl Pts',(-50.,12.3671730117507,-10.6260754926723));
#53525=CARTESIAN_POINT('Ctrl Pts',(-50.,12.336435220754,-10.5570770785351));
#53526=CARTESIAN_POINT('Ctrl Pts',(-50.,12.2916238883603,-10.4709250501372));
#53527=CARTESIAN_POINT('Ctrl Pts',(-50.,12.2325064717433,-10.3677455989363));
#53528=CARTESIAN_POINT('Ctrl Pts',(-50.,12.1729620080223,-10.2634984322242));
#53529=CARTESIAN_POINT('Ctrl Pts',(-50.,12.1141848750712,-10.1561990251342));
#53530=CARTESIAN_POINT('Ctrl Pts',(-50.,12.0558705645975,-10.0465202590396));
#53531=CARTESIAN_POINT('Ctrl Pts',(-50.,11.9969002916812,-9.93651465742827));
#53532=CARTESIAN_POINT('Ctrl Pts',(-50.,11.9358257812543,-9.82870769953299));
#53533=CARTESIAN_POINT('Ctrl Pts',(-50.,11.8715286035136,-9.724847924125));
#53534=CARTESIAN_POINT('Ctrl Pts',(-50.,11.8034143911192,-9.62560737856555));
#53535=CARTESIAN_POINT('Ctrl Pts',(-50.,11.7312595885623,-9.53100857350628));
#53536=CARTESIAN_POINT('Ctrl Pts',(-50.,11.655157779328,-9.44063172122792));
#53537=CARTESIAN_POINT('Ctrl Pts',(-50.,11.5754278219505,-9.35393513817802));
#53538=CARTESIAN_POINT('Ctrl Pts',(-50.,11.4925391231036,-9.27043802686381));
#53539=CARTESIAN_POINT('Ctrl Pts',(-50.,11.407025252502,-9.18970993907287));
#53540=CARTESIAN_POINT('Ctrl Pts',(-50.,11.3194051551598,-9.11139639219764));
#53541=CARTESIAN_POINT('Ctrl Pts',(-50.,11.2300954828748,-9.03523227310488));
#53542=CARTESIAN_POINT('Ctrl Pts',(-50.,11.1393445344495,-8.96105481127105));
#53543=CARTESIAN_POINT('Ctrl Pts',(-50.,11.0656943951459,-8.90323201632451));
#53544=CARTESIAN_POINT('Ctrl Pts',(-50.,11.0098871540402,-8.86070419148627));
#53545=CARTESIAN_POINT('Ctrl Pts',(-50.,10.9724295263217,-8.83272480732197));
#53546=CARTESIAN_POINT('Ctrl Pts',(-50.,10.9536375103364,-8.81882824088046));
#53547=CARTESIAN_POINT('',(-50.,11.7720642054939,-7.6923605344347));
#53548=CARTESIAN_POINT('Origin',(-50.,0.,0.));
#53549=CARTESIAN_POINT('',(-50.,14.0138288999568,-8.47072751083015));
#53550=CARTESIAN_POINT('Ctrl Pts',(-50.,11.7720642054939,-7.69236053443469));
#53551=CARTESIAN_POINT('Ctrl Pts',(-50.,11.7884105699588,-7.70376738782835));
#53552=CARTESIAN_POINT('Ctrl Pts',(-50.,11.8211715224307,-7.72648734423527));
#53553=CARTESIAN_POINT('Ctrl Pts',(-50.,11.870517618491,-7.7602860336664));
#53554=CARTESIAN_POINT('Ctrl Pts',(-50.,11.936722320441,-7.80478766329085));
#53555=CARTESIAN_POINT('Ctrl Pts',(-50.,12.0201833141302,-7.85943599303422));
#53556=CARTESIAN_POINT('Ctrl Pts',(-50.,12.1044103376288,-7.91299239895144));
#53557=CARTESIAN_POINT('Ctrl Pts',(-50.,12.1895203359981,-7.96523745572904));
#53558=CARTESIAN_POINT('Ctrl Pts',(-50.,12.2757069077219,-8.01580608992824));
#53559=CARTESIAN_POINT('Ctrl Pts',(-50.,12.3632517496072,-8.06416486307078));
#53560=CARTESIAN_POINT('Ctrl Pts',(-50.,12.4524600493824,-8.10972846142537));
#53561=CARTESIAN_POINT('Ctrl Pts',(-50.,12.5436007236081,-8.15196711241727));
#53562=CARTESIAN_POINT('Ctrl Pts',(-50.,12.636848388186,-8.19051110794578));
#53563=CARTESIAN_POINT('Ctrl Pts',(-50.,12.7322148461558,-8.22527363116368));
#53564=CARTESIAN_POINT('Ctrl Pts',(-50.,12.829511804771,-8.25651874452987));
#53565=CARTESIAN_POINT('Ctrl Pts',(-50.,12.9284352169133,-8.284715594814));
#53566=CARTESIAN_POINT('Ctrl Pts',(-50.,13.0286320818366,-8.31042356359388));
#53567=CARTESIAN_POINT('Ctrl Pts',(-50.,13.1297695959248,-8.33417308930716));
#53568=CARTESIAN_POINT('Ctrl Pts',(-50.,13.231612467433,-8.35633273843435));
#53569=CARTESIAN_POINT('Ctrl Pts',(-50.,13.3340674354409,-8.37703230872753));
#53570=CARTESIAN_POINT('Ctrl Pts',(-50.,13.4371309168349,-8.39625156414993));
#53571=CARTESIAN_POINT('Ctrl Pts',(-50.,13.5408537546603,-8.41387978285669));
#53572=CARTESIAN_POINT('Ctrl Pts',(-50.,13.6453014633841,-8.42978304193647));
#53573=CARTESIAN_POINT('Ctrl Pts',(-50.,13.7505117765273,-8.44387618307839));
#53574=CARTESIAN_POINT('Ctrl Pts',(-50.,13.8452784046188,-8.45486947201102));
#53575=CARTESIAN_POINT('Ctrl Pts',(-50.,13.9192737837169,-8.4623570321923));
#53576=CARTESIAN_POINT('Ctrl Pts',(-50.,13.9721524684248,-8.46718145686578));
#53577=CARTESIAN_POINT('Ctrl Pts',(-50.,14.0037053056615,-8.4698799979691));
#53578=CARTESIAN_POINT('Ctrl Pts',(-50.,14.0138288999568,-8.47072751083015));
#53579=CARTESIAN_POINT('',(-50.,14.6670849864349,-7.28129404712485));
#53580=CARTESIAN_POINT('Origin',(-50.,0.,0.));
#53581=CARTESIAN_POINT('',(-50.,12.8026622457696,-5.81770965851216));
#53582=CARTESIAN_POINT('Ctrl Pts',(-50.,14.6670849864349,-7.28129404712485));
#53583=CARTESIAN_POINT('Ctrl Pts',(-50.,14.6668197205911,-7.28090773432903));
#53584=CARTESIAN_POINT('Ctrl Pts',(-50.,14.6516933118151,-7.2588971478181));
#53585=CARTESIAN_POINT('Ctrl Pts',(-50.,14.6212330452241,-7.21664693024351));
#53586=CARTESIAN_POINT('Ctrl Pts',(-50.,14.5743017306281,-7.15746040594034));
#53587=CARTESIAN_POINT('Ctrl Pts',(-50.,14.5094730904225,-7.08515912713373));
#53588=CARTESIAN_POINT('Ctrl Pts',(-50.,14.426553270081,-6.99992315179396));
#53589=CARTESIAN_POINT('Ctrl Pts',(-50.,14.3429542890555,-6.9137592074853));
#53590=CARTESIAN_POINT('Ctrl Pts',(-50.,14.2593394703776,-6.8244480871404));
#53591=CARTESIAN_POINT('Ctrl Pts',(-50.,14.1755812112355,-6.73271726045961));
#53592=CARTESIAN_POINT('Ctrl Pts',(-50.,14.0911063172293,-6.64083299762664));
#53593=CARTESIAN_POINT('Ctrl Pts',(-50.,14.0051400746611,-6.55160160666348));
#53594=CARTESIAN_POINT('Ctrl Pts',(-50.,13.9170340351662,-6.46699483496205));
#53595=CARTESIAN_POINT('Ctrl Pts',(-50.,13.8263796359301,-6.38781142942664));
#53596=CARTESIAN_POINT('Ctrl Pts',(-50.,13.7329659430228,-6.31412878948963));
#53597=CARTESIAN_POINT('Ctrl Pts',(-50.,13.6367792028716,-6.24551704256852));
#53598=CARTESIAN_POINT('Ctrl Pts',(-50.,13.537993545262,-6.18137222620287));
#53599=CARTESIAN_POINT('Ctrl Pts',(-50.,13.4369440601197,-6.12111191134452));
#53600=CARTESIAN_POINT('Ctrl Pts',(-50.,13.3340405059683,-6.06418647971103));
#53601=CARTESIAN_POINT('Ctrl Pts',(-50.,13.2296973679703,-6.01012352904084));
#53602=CARTESIAN_POINT('Ctrl Pts',(-50.,13.124252277086,-5.95856265812867));
#53603=CARTESIAN_POINT('Ctrl Pts',(-50.,13.0179052519711,-5.90928446078516));
#53604=CARTESIAN_POINT('Ctrl Pts',(-50.,12.932189022876,-5.87159432010365));
#53605=CARTESIAN_POINT('Ctrl Pts',(-50.,12.8675588289116,-5.84428128157946));
#53606=CARTESIAN_POINT('Ctrl Pts',(-50.,12.8243198115569,-5.82649625442995));
#53607=CARTESIAN_POINT('Ctrl Pts',(-50.,12.8026622457696,-5.81770965851216));
#53608=CARTESIAN_POINT('',(-50.,13.3152354345065,-4.52309756402218));
#53609=CARTESIAN_POINT('Origin',(-50.,0.,0.));
#53610=CARTESIAN_POINT('',(-50.,15.6801429643085,-4.71950650162129));
#53611=CARTESIAN_POINT('Ctrl Pts',(-50.,13.3152354345065,-4.52309756402217));
#53612=CARTESIAN_POINT('Ctrl Pts',(-50.,13.3339050169562,-4.53008087460641));
#53613=CARTESIAN_POINT('Ctrl Pts',(-50.,13.3712869472582,-4.54393972423008));
#53614=CARTESIAN_POINT('Ctrl Pts',(-50.,13.4274881372306,-4.56440469062003));
#53615=CARTESIAN_POINT('Ctrl Pts',(-50.,13.5026800019769,-4.59104377985933));
#53616=CARTESIAN_POINT('Ctrl Pts',(-50.,13.5971094020329,-4.62321932672933));
#53617=CARTESIAN_POINT('Ctrl Pts',(-50.,13.6920092152502,-4.65414675070122));
#53618=CARTESIAN_POINT('Ctrl Pts',(-50.,13.7874381437893,-4.68358443705714));
#53619=CARTESIAN_POINT('Ctrl Pts',(-50.,13.8834929138094,-4.71113063582666));
#53620=CARTESIAN_POINT('Ctrl Pts',(-50.,13.9803137113395,-4.73619861233502));
#53621=CARTESIAN_POINT('Ctrl Pts',(-50.,14.0780505744683,-4.75814554445644));
#53622=CARTESIAN_POINT('Ctrl Pts',(-50.,14.1768322221664,-4.77639142656668));
#53623=CARTESIAN_POINT('Ctrl Pts',(-50.,14.27673584179,-4.79053474041595));
#53624=CARTESIAN_POINT('Ctrl Pts',(-50.,14.3777512750926,-4.80048846137132));
#53625=CARTESIAN_POINT('Ctrl Pts',(-50.,14.4797618145538,-4.80655518238588));
#53626=CARTESIAN_POINT('Ctrl Pts',(-50.,14.5825896373118,-4.80926492456431));
#53627=CARTESIAN_POINT('Ctrl Pts',(-50.,14.6860319453295,-4.80924728319928));
#53628=CARTESIAN_POINT('Ctrl Pts',(-50.,14.7898983053036,-4.80709879692323));
#53629=CARTESIAN_POINT('Ctrl Pts',(-50.,14.8940524763685,-4.80323496770043));
#53630=CARTESIAN_POINT('Ctrl Pts',(-50.,14.9984364069554,-4.79780470849564));
#53631=CARTESIAN_POINT('Ctrl Pts',(-50.,15.1030415940234,-4.79078931010852));
#53632=CARTESIAN_POINT('Ctrl Pts',(-50.,15.2078897478867,-4.78206888507335));
#53633=CARTESIAN_POINT('Ctrl Pts',(-50.,15.3130110194811,-4.77149742512795));
#53634=CARTESIAN_POINT('Ctrl Pts',(-50.,15.418420778849,-4.75898306342126));
#53635=CARTESIAN_POINT('Ctrl Pts',(-50.,15.5129440588396,-4.74606347591976));
#53636=CARTESIAN_POINT('Ctrl Pts',(-50.,15.586476817532,-4.73491389815065));
#53637=CARTESIAN_POINT('Ctrl Pts',(-50.,15.6388940067504,-4.72643636051809));
#53638=CARTESIAN_POINT('Ctrl Pts',(-50.,15.6701266534662,-4.72120325045824));
#53639=CARTESIAN_POINT('Ctrl Pts',(-50.,15.6801429643085,-4.71950650162129));
#53640=CARTESIAN_POINT('',(-50.,16.017075735697,-3.40498309495743));
#53641=CARTESIAN_POINT('Origin',(-50.,0.,0.));
#53642=CARTESIAN_POINT('',(-50.,13.847248627403,-2.45104298226008));
#53643=CARTESIAN_POINT('Ctrl Pts',(-50.,16.017075735697,-3.40498309495743));
#53644=CARTESIAN_POINT('Ctrl Pts',(-50.,16.0167227315819,-3.40467488782123));
#53645=CARTESIAN_POINT('Ctrl Pts',(-50.,15.9965977364772,-3.38711758925191));
#53646=CARTESIAN_POINT('Ctrl Pts',(-50.,15.9565872333324,-3.35376990021665));
#53647=CARTESIAN_POINT('Ctrl Pts',(-50.,15.8964112622344,-3.30811417274226));
#53648=CARTESIAN_POINT('Ctrl Pts',(-50.,15.8156387361042,-3.25420659877988));
#53649=CARTESIAN_POINT('Ctrl Pts',(-50.,15.7141266693079,-3.19226978910788));
#53650=CARTESIAN_POINT('Ctrl Pts',(-50.,15.6117260024113,-3.1296030647124));
#53651=CARTESIAN_POINT('Ctrl Pts',(-50.,15.5085273245779,-3.06389197726713));
#53652=CARTESIAN_POINT('Ctrl Pts',(-50.,15.4045879562307,-2.99587287520288));
#53653=CARTESIAN_POINT('Ctrl Pts',(-50.,15.299916309402,-2.9278833773088));
#53654=CARTESIAN_POINT('Ctrl Pts',(-50.,15.1944599098748,-2.86283428974206));
#53655=CARTESIAN_POINT('Ctrl Pts',(-50.,15.0880810351184,-2.80279667637514));
#53656=CARTESIAN_POINT('Ctrl Pts',(-50.,14.9805825983482,-2.74864579544975));
#53657=CARTESIAN_POINT('Ctrl Pts',(-50.,14.8717795409674,-2.70050907188802));
#53658=CARTESIAN_POINT('Ctrl Pts',(-50.,14.7615516365331,-2.65797355871958));
#53659=CARTESIAN_POINT('Ctrl Pts',(-50.,14.6499173448672,-2.62041096375855));
#53660=CARTESIAN_POINT('Ctrl Pts',(-50.,14.537056384215,-2.58717382256056));
#53661=CARTESIAN_POINT('Ctrl Pts',(-50.,14.423228955274,-2.55762788131115));
#53662=CARTESIAN_POINT('Ctrl Pts',(-50.,14.3087190397278,-2.53121250086624));
#53663=CARTESIAN_POINT('Ctrl Pts',(-50.,14.1937640331043,-2.50749463728168));
#53664=CARTESIAN_POINT('Ctrl Pts',(-50.,14.0785031060049,-2.48621203480011));
#53665=CARTESIAN_POINT('Ctrl Pts',(-50.,13.9861066530346,-2.47102275853729));
#53666=CARTESIAN_POINT('Ctrl Pts',(-50.,13.9167144589915,-2.46064068498796));
#53667=CARTESIAN_POINT('Ctrl Pts',(-50.,13.8704109184829,-2.45416751351779));
#53668=CARTESIAN_POINT('Ctrl Pts',(-50.,13.847248627403,-2.45104298226008));
#53669=CARTESIAN_POINT('Origin',(-50.,0.,0.));
#53670=CARTESIAN_POINT('Origin',(-50.,0.,0.));
#53671=CARTESIAN_POINT('',(-50.,5.93712762672243,-8.04677050399782));
#53672=CARTESIAN_POINT('Origin',(-50.,0.,0.));
#53673=CARTESIAN_POINT('',(-50.,3.75038736519794,-6.13145585166881));
#53674=CARTESIAN_POINT('Ctrl Pts',(-50.,3.75038736519793,-6.13145585166881));
#53675=CARTESIAN_POINT('Ctrl Pts',(-50.,3.7614973065729,-6.1481985134482));
#53676=CARTESIAN_POINT('Ctrl Pts',(-50.,3.78357651403939,-6.1817683663582));
#53677=CARTESIAN_POINT('Ctrl Pts',(-50.,3.81627329006595,-6.23237673886416));
#53678=CARTESIAN_POINT('Ctrl Pts',(-50.,3.859023878729,-6.30036238594766));
#53679=CARTESIAN_POINT('Ctrl Pts',(-50.,3.91110213900011,-6.38616193008433));
#53680=CARTESIAN_POINT('Ctrl Pts',(-50.,3.96197913233089,-6.47268455970493));
#53681=CARTESIAN_POINT('Ctrl Pts',(-50.,4.01197889710939,-6.55973735411151));
#53682=CARTESIAN_POINT('Ctrl Pts',(-50.,4.06165666819706,-6.64698999124062));
#53683=CARTESIAN_POINT('Ctrl Pts',(-50.,4.11183783259628,-6.73395053478792));
#53684=CARTESIAN_POINT('Ctrl Pts',(-50.,4.16348379256721,-6.82003644526658));
#53685=CARTESIAN_POINT('Ctrl Pts',(-50.,4.21757413484032,-6.90463617300865));
#53686=CARTESIAN_POINT('Ctrl Pts',(-50.,4.27498923356982,-6.98717136730191));
#53687=CARTESIAN_POINT('Ctrl Pts',(-50.,4.33637651734857,-7.06716577496009));
#53688=CARTESIAN_POINT('Ctrl Pts',(-50.,4.40207217433237,-7.14429034032177));
#53689=CARTESIAN_POINT('Ctrl Pts',(-50.,4.47217290162416,-7.21834255288981));
#53690=CARTESIAN_POINT('Ctrl Pts',(-50.,4.54657777868016,-7.28923990788708));
#53691=CARTESIAN_POINT('Ctrl Pts',(-50.,4.62503998887083,-7.35700721943171));
#53692=CARTESIAN_POINT('Ctrl Pts',(-50.,4.70721371156899,-7.42177134000892));
#53693=CARTESIAN_POINT('Ctrl Pts',(-50.,4.79269894740031,-7.48374039375355));
#53694=CARTESIAN_POINT('Ctrl Pts',(-50.,4.88107836846757,-7.54316218647348));
#53695=CARTESIAN_POINT('Ctrl Pts',(-50.,4.9719575030537,-7.60028648840776));
#53696=CARTESIAN_POINT('Ctrl Pts',(-50.,5.06499955030093,-7.65532943098672));
#53697=CARTESIAN_POINT('Ctrl Pts',(-50.,5.15997145275563,-7.70842918324715));
#53698=CARTESIAN_POINT('Ctrl Pts',(-50.,5.25675269887972,-7.75963419345371));
#53699=CARTESIAN_POINT('Ctrl Pts',(-50.,5.35529468870783,-7.80893560674388));
#53700=CARTESIAN_POINT('Ctrl Pts',(-50.,5.45559153104423,-7.85628931405591));
#53701=CARTESIAN_POINT('Ctrl Pts',(-50.,5.5576484178972,-7.90164067817667));
#53702=CARTESIAN_POINT('Ctrl Pts',(-50.,5.66144582368073,-7.94495188520329));
#53703=CARTESIAN_POINT('Ctrl Pts',(-50.,5.75805784341865,-7.98274785508065));
#53704=CARTESIAN_POINT('Ctrl Pts',(-50.,5.83459703193086,-8.01098733792827));
#53705=CARTESIAN_POINT('Ctrl Pts',(-50.,5.89025885371265,-8.03066876757453));
#53706=CARTESIAN_POINT('Ctrl Pts',(-50.,5.92452703906404,-8.04247213408069));
#53707=CARTESIAN_POINT('Ctrl Pts',(-50.,5.93712762672279,-8.04677050399795));
#53708=CARTESIAN_POINT('',(-50.,2.45543694297674,-6.75507110762463));
#53709=CARTESIAN_POINT('Origin',(-50.,0.,0.));
#53710=CARTESIAN_POINT('',(-50.,2.55037217513312,-9.66931237308562));
#53711=CARTESIAN_POINT('Ctrl Pts',(-50.,2.55037217513312,-9.66931237308562));
#53712=CARTESIAN_POINT('Ctrl Pts',(-50.,2.55611128043686,-9.64665974290731));
#53713=CARTESIAN_POINT('Ctrl Pts',(-50.,2.57093577554682,-9.59816055611738));
#53714=CARTESIAN_POINT('Ctrl Pts',(-50.,2.60118245057803,-9.51956163099604));
#53715=CARTESIAN_POINT('Ctrl Pts',(-50.,2.6506378639391,-9.4077851093183));
#53716=CARTESIAN_POINT('Ctrl Pts',(-50.,2.71205611361093,-9.26593773005304));
#53717=CARTESIAN_POINT('Ctrl Pts',(-50.,2.76185693608665,-9.12774569066013));
#53718=CARTESIAN_POINT('Ctrl Pts',(-50.,2.79564609540172,-8.99695638729624));
#53719=CARTESIAN_POINT('Ctrl Pts',(-50.,2.81593951016314,-8.87218721998315));
#53720=CARTESIAN_POINT('Ctrl Pts',(-50.,2.8281804649272,-8.7503085875302));
#53721=CARTESIAN_POINT('Ctrl Pts',(-50.,2.838231660712,-8.62789111098118));
#53722=CARTESIAN_POINT('Ctrl Pts',(-50.,2.84893087833482,-8.50318672326558));
#53723=CARTESIAN_POINT('Ctrl Pts',(-50.,2.85932311928695,-8.37659160589212));
#53724=CARTESIAN_POINT('Ctrl Pts',(-50.,2.8666442371861,-8.24955186700095));
#53725=CARTESIAN_POINT('Ctrl Pts',(-50.,2.86748815125169,-8.12392974416385));
#53726=CARTESIAN_POINT('Ctrl Pts',(-50.,2.85947913898695,-8.00108902987832));
#53727=CARTESIAN_POINT('Ctrl Pts',(-50.,2.84216119689693,-7.88140953422486));
#53728=CARTESIAN_POINT('Ctrl Pts',(-50.,2.81629364412744,-7.76466852264525));
#53729=CARTESIAN_POINT('Ctrl Pts',(-50.,2.78345892001629,-7.65025207826714));
#53730=CARTESIAN_POINT('Ctrl Pts',(-50.,2.74553095355499,-7.53744508591865));
#53731=CARTESIAN_POINT('Ctrl Pts',(-50.,2.70427297026251,-7.42564364342468));
#53732=CARTESIAN_POINT('Ctrl Pts',(-50.,2.66128382072048,-7.31434056822034));
#53733=CARTESIAN_POINT('Ctrl Pts',(-50.,2.61790620462629,-7.20313763732345));
#53734=CARTESIAN_POINT('Ctrl Pts',(-50.,2.57514309471485,-7.09174914908801));
#53735=CARTESIAN_POINT('Ctrl Pts',(-50.,2.53358368474749,-6.98000697278327));
#53736=CARTESIAN_POINT('Ctrl Pts',(-50.,2.50153193679118,-6.89026394714059));
#53737=CARTESIAN_POINT('Ctrl Pts',(-50.,2.47820711493347,-6.82274841734025));
#53738=CARTESIAN_POINT('Ctrl Pts',(-50.,2.46297417772978,-6.77764561818537));
#53739=CARTESIAN_POINT('Ctrl Pts',(-50.,2.45543694297674,-6.75507110762463));
#53740=CARTESIAN_POINT('',(-50.,1.85780428234483,-9.82591284555798));
#53741=CARTESIAN_POINT('Origin',(-50.,0.,0.));
#53742=CARTESIAN_POINT('',(-50.,0.718643267461627,-7.15148293042304));
#53743=CARTESIAN_POINT('Ctrl Pts',(-50.,0.718643267461621,-7.15148293042304));
#53744=CARTESIAN_POINT('Ctrl Pts',(-50.,0.721388610069064,-7.17138797035723));
#53745=CARTESIAN_POINT('Ctrl Pts',(-50.,0.72671587532212,-7.21121317182152));
#53746=CARTESIAN_POINT('Ctrl Pts',(-50.,0.734216502709278,-7.2709963393441));
#53747=CARTESIAN_POINT('Ctrl Pts',(-50.,0.743235585416283,-7.35079807608913));
#53748=CARTESIAN_POINT('Ctrl Pts',(-50.,0.752929449590465,-7.45069670452966));
#53749=CARTESIAN_POINT('Ctrl Pts',(-50.,0.761227274615911,-7.55072560028829));
#53750=CARTESIAN_POINT('Ctrl Pts',(-50.,0.768504714146026,-7.65085154280962));
#53751=CARTESIAN_POINT('Ctrl Pts',(-50.,0.775405338877349,-7.75101782957587));
#53752=CARTESIAN_POINT('Ctrl Pts',(-50.,0.782886239966143,-7.85113936329068));
#53753=CARTESIAN_POINT('Ctrl Pts',(-50.,0.792066365329068,-7.95110843081948));
#53754=CARTESIAN_POINT('Ctrl Pts',(-50.,0.804093633570272,-8.05079907170372));
#53755=CARTESIAN_POINT('Ctrl Pts',(-50.,0.820012171364339,-8.15007218998677));
#53756=CARTESIAN_POINT('Ctrl Pts',(-50.,0.840611930230857,-8.24877960511329));
#53757=CARTESIAN_POINT('Ctrl Pts',(-50.,0.866338577132719,-8.34677071475058));
#53758=CARTESIAN_POINT('Ctrl Pts',(-50.,0.897367099160984,-8.4439050185459));
#53759=CARTESIAN_POINT('Ctrl Pts',(-50.,0.933642367528787,-8.5400643944807));
#53760=CARTESIAN_POINT('Ctrl Pts',(-50.,0.974931241694465,-8.63516410958082));
#53761=CARTESIAN_POINT('Ctrl Pts',(-50.,1.02086710880845,-8.72916840803945));
#53762=CARTESIAN_POINT('Ctrl Pts',(-50.,1.07099928020948,-8.82209124999857));
#53763=CARTESIAN_POINT('Ctrl Pts',(-50.,1.12484423754393,-8.91397482898789));
#53764=CARTESIAN_POINT('Ctrl Pts',(-50.,1.18193820283021,-9.00487302535333));
#53765=CARTESIAN_POINT('Ctrl Pts',(-50.,1.24188395306769,-9.09483443436949));
#53766=CARTESIAN_POINT('Ctrl Pts',(-50.,1.30441156144786,-9.18388242219763));
#53767=CARTESIAN_POINT('Ctrl Pts',(-50.,1.3693914299125,-9.27200835121914));
#53768=CARTESIAN_POINT('Ctrl Pts',(-50.,1.43678361338666,-9.35918315674388));
#53769=CARTESIAN_POINT('Ctrl Pts',(-50.,1.50660194229105,-9.44536454178638));
#53770=CARTESIAN_POINT('Ctrl Pts',(-50.,1.57887480066182,-9.53050553264656));
#53771=CARTESIAN_POINT('Ctrl Pts',(-50.,1.65360100339141,-9.61456358834088));
#53772=CARTESIAN_POINT('Ctrl Pts',(-50.,1.72424636870643,-9.69053496490009));
#53773=CARTESIAN_POINT('Ctrl Pts',(-50.,1.78095314232172,-9.7491869690921));
#53774=CARTESIAN_POINT('Ctrl Pts',(-50.,1.82256325859169,-9.79107008383992));
#53775=CARTESIAN_POINT('Ctrl Pts',(-50.,1.84831653795888,-9.81657295799139));
#53776=CARTESIAN_POINT('Ctrl Pts',(-50.,1.85780428234483,-9.82591284555798));
#53777=CARTESIAN_POINT('',(-50.,-0.718643267461624,-7.15148293042304));
#53778=CARTESIAN_POINT('Origin',(-50.,0.,0.));
#53779=CARTESIAN_POINT('',(-50.,-1.89755147577054,-9.81831443766195));
#53780=CARTESIAN_POINT('Ctrl Pts',(-50.,-1.89755147577054,-9.81831443766195));
#53781=CARTESIAN_POINT('Ctrl Pts',(-50.,-1.88255211267964,-9.80039522756355));
#53782=CARTESIAN_POINT('Ctrl Pts',(-50.,-1.84815269559462,-9.76313107751608));
#53783=CARTESIAN_POINT('Ctrl Pts',(-50.,-1.78679858751167,-9.70543943338958));
#53784=CARTESIAN_POINT('Ctrl Pts',(-50.,-1.69374278455301,-9.62619016686422));
#53785=CARTESIAN_POINT('Ctrl Pts',(-50.,-1.576861582378,-9.52503847397034));
#53786=CARTESIAN_POINT('Ctrl Pts',(-50.,-1.47203331296336,-9.42213951575228));
#53787=CARTESIAN_POINT('Ctrl Pts',(-50.,-1.38484298036779,-9.31896299195203));
#53788=CARTESIAN_POINT('Ctrl Pts',(-50.,-1.31242393260393,-9.21535483920498));
#53789=CARTESIAN_POINT('Ctrl Pts',(-50.,-1.24851405668088,-9.11085713692575));
#53790=CARTESIAN_POINT('Ctrl Pts',(-50.,-1.18634328973517,-9.00492385207762));
#53791=CARTESIAN_POINT('Ctrl Pts',(-50.,-1.12259642171968,-8.89721129760285));
#53792=CARTESIAN_POINT('Ctrl Pts',(-50.,-1.05830577327405,-8.78766206238304));
#53793=CARTESIAN_POINT('Ctrl Pts',(-50.,-0.996589197042053,-8.67637972666424));
#53794=CARTESIAN_POINT('Ctrl Pts',(-50.,-0.941323460369318,-8.56356426545847));
#53795=CARTESIAN_POINT('Ctrl Pts',(-50.,-0.895240742652424,-8.44941362598824));
#53796=CARTESIAN_POINT('Ctrl Pts',(-50.,-0.858916682261846,-8.33407215281038));
#53797=CARTESIAN_POINT('Ctrl Pts',(-50.,-0.831570515383447,-8.21766862525226));
#53798=CARTESIAN_POINT('Ctrl Pts',(-50.,-0.811510144890449,-8.10033651802127));
#53799=CARTESIAN_POINT('Ctrl Pts',(-50.,-0.796736942256156,-7.98224460192821));
#53800=CARTESIAN_POINT('Ctrl Pts',(-50.,-0.785400272847099,-7.86361381479518));
#53801=CARTESIAN_POINT('Ctrl Pts',(-50.,-0.775839563797133,-7.74468091618948));
#53802=CARTESIAN_POINT('Ctrl Pts',(-50.,-0.766672302003446,-7.62566969516693));
#53803=CARTESIAN_POINT('Ctrl Pts',(-50.,-0.756870878958097,-7.5067579169994));
#53804=CARTESIAN_POINT('Ctrl Pts',(-50.,-0.745831500234844,-7.38804974272502));
#53805=CARTESIAN_POINT('Ctrl Pts',(-50.,-0.735771087779772,-7.29328733826105));
#53806=CARTESIAN_POINT('Ctrl Pts',(-50.,-0.72749213560466,-7.22233768688913));
#53807=CARTESIAN_POINT('Ctrl Pts',(-50.,-0.721647166649912,-7.17509214524366));
#53808=CARTESIAN_POINT('Ctrl Pts',(-50.,-0.718643267461624,-7.15148293042304));
#53809=CARTESIAN_POINT('',(-50.,-2.58947998462545,-9.65891264114259));
#53810=CARTESIAN_POINT('Origin',(-50.,0.,0.));
#53811=CARTESIAN_POINT('',(-50.,-2.45543694297674,-6.75507110762463));
#53812=CARTESIAN_POINT('Ctrl Pts',(-50.,-2.45543694297675,-6.75507110762463));
#53813=CARTESIAN_POINT('Ctrl Pts',(-50.,-2.46159994790965,-6.77419608843536));
#53814=CARTESIAN_POINT('Ctrl Pts',(-50.,-2.47407975508802,-6.8123887688799));
#53815=CARTESIAN_POINT('Ctrl Pts',(-50.,-2.49326086758344,-6.8695059418988));
#53816=CARTESIAN_POINT('Ctrl Pts',(-50.,-2.5197596307744,-6.94531805563895));
#53817=CARTESIAN_POINT('Ctrl Pts',(-50.,-2.55437015138428,-7.03952961984441));
#53818=CARTESIAN_POINT('Ctrl Pts',(-50.,-2.59029498067661,-7.13325283216217));
#53819=CARTESIAN_POINT('Ctrl Pts',(-50.,-2.62718125254576,-7.22662075191781));
#53820=CARTESIAN_POINT('Ctrl Pts',(-50.,-2.66442452752942,-7.31986152676826));
#53821=CARTESIAN_POINT('Ctrl Pts',(-50.,-2.70112557395893,-7.41331375298832));
#53822=CARTESIAN_POINT('Ctrl Pts',(-50.,-2.73622951961898,-7.50736587770304));
#53823=CARTESIAN_POINT('Ctrl Pts',(-50.,-2.76864747338962,-7.60240247767684));
#53824=CARTESIAN_POINT('Ctrl Pts',(-50.,-2.79737835816915,-7.69875126136884));
#53825=CARTESIAN_POINT('Ctrl Pts',(-50.,-2.82164615909785,-7.79662146983088));
#53826=CARTESIAN_POINT('Ctrl Pts',(-50.,-2.84098400021346,-7.89607078269802));
#53827=CARTESIAN_POINT('Ctrl Pts',(-50.,-2.85517326277626,-7.9970485375799));
#53828=CARTESIAN_POINT('Ctrl Pts',(-50.,-2.86421236488387,-8.099424390731));
#53829=CARTESIAN_POINT('Ctrl Pts',(-50.,-2.8682745946465,-8.20302084448955));
#53830=CARTESIAN_POINT('Ctrl Pts',(-50.,-2.86767474496505,-8.30764661663281));
#53831=CARTESIAN_POINT('Ctrl Pts',(-50.,-2.86282492937103,-8.41311873833255));
#53832=CARTESIAN_POINT('Ctrl Pts',(-50.,-2.85417908993455,-8.51926543389428));
#53833=CARTESIAN_POINT('Ctrl Pts',(-50.,-2.84217845398458,-8.62593402210748));
#53834=CARTESIAN_POINT('Ctrl Pts',(-50.,-2.82720199177778,-8.73299593720093));
#53835=CARTESIAN_POINT('Ctrl Pts',(-50.,-2.80950303716262,-8.84035511450549));
#53836=CARTESIAN_POINT('Ctrl Pts',(-50.,-2.78919460623265,-8.94794754130566));
#53837=CARTESIAN_POINT('Ctrl Pts',(-50.,-2.76630007756038,-9.05572969970196));
#53838=CARTESIAN_POINT('Ctrl Pts',(-50.,-2.74078863839312,-9.16366948222194));
#53839=CARTESIAN_POINT('Ctrl Pts',(-50.,-2.71261433447333,-9.27173688239595));
#53840=CARTESIAN_POINT('Ctrl Pts',(-50.,-2.68175977570501,-9.37989305792331));
#53841=CARTESIAN_POINT('Ctrl Pts',(-50.,-2.65107324582197,-9.47899277830914));
#53842=CARTESIAN_POINT('Ctrl Pts',(-50.,-2.62543035908095,-9.55644055509579));
#53843=CARTESIAN_POINT('Ctrl Pts',(-50.,-2.60611334216455,-9.61222989040676));
#53844=CARTESIAN_POINT('Ctrl Pts',(-50.,-2.59397572160338,-9.64638111520572));
#53845=CARTESIAN_POINT('Ctrl Pts',(-50.,-2.58947998462532,-9.65891264114296));
#53846=CARTESIAN_POINT('',(-50.,-3.75038736519793,-6.13145585166881));
#53847=CARTESIAN_POINT('Origin',(-50.,0.,0.));
#53848=CARTESIAN_POINT('',(-50.,-5.96964178495622,-8.0226789141349));
#53849=CARTESIAN_POINT('Ctrl Pts',(-50.,-5.96964178495622,-8.0226789141349));
#53850=CARTESIAN_POINT('Ctrl Pts',(-50.,-5.94835297189343,-8.0130422434411));
#53851=CARTESIAN_POINT('Ctrl Pts',(-50.,-5.9011918592682,-7.9943937520678));
#53852=CARTESIAN_POINT('Ctrl Pts',(-50.,-5.8208822516981,-7.96903592659697));
#53853=CARTESIAN_POINT('Ctrl Pts',(-50.,-5.70265690217233,-7.93801020438781));
#53854=CARTESIAN_POINT('Ctrl Pts',(-50.,-5.55346250303877,-7.89758853118704));
#53855=CARTESIAN_POINT('Ctrl Pts',(-50.,-5.41436931107715,-7.85036305479183));
#53856=CARTESIAN_POINT('Ctrl Pts',(-50.,-5.29104691989087,-7.79523468647088));
#53857=CARTESIAN_POINT('Ctrl Pts',(-50.,-5.18084571969554,-7.73330841361203));
#53858=CARTESIAN_POINT('Ctrl Pts',(-50.,-5.07792505734327,-7.66688869302314));
#53859=CARTESIAN_POINT('Ctrl Pts',(-50.,-4.97594840210465,-7.59842098612654));
#53860=CARTESIAN_POINT('Ctrl Pts',(-50.,-4.87177973271099,-7.52903405731413));
#53861=CARTESIAN_POINT('Ctrl Pts',(-50.,-4.76632422816958,-7.45822827381644));
#53862=CARTESIAN_POINT('Ctrl Pts',(-50.,-4.66243591843162,-7.38474417264741));
#53863=CARTESIAN_POINT('Ctrl Pts',(-50.,-4.56369441608956,-7.30707985875561));
#53864=CARTESIAN_POINT('Ctrl Pts',(-50.,-4.4726472158023,-7.22422822821349));
#53865=CARTESIAN_POINT('Ctrl Pts',(-50.,-4.38987557857684,-7.13606957084443));
#53866=CARTESIAN_POINT('Ctrl Pts',(-50.,-4.31473193577955,-7.04305867353628));
#53867=CARTESIAN_POINT('Ctrl Pts',(-50.,-4.24574967308285,-6.94604996627335));
#53868=CARTESIAN_POINT('Ctrl Pts',(-50.,-4.18120131531612,-6.84606267872027));
#53869=CARTESIAN_POINT('Ctrl Pts',(-50.,-4.11951535961712,-6.74409882925098));
#53870=CARTESIAN_POINT('Ctrl Pts',(-50.,-4.0592984076569,-6.64109222642907));
#53871=CARTESIAN_POINT('Ctrl Pts',(-50.,-3.99940195660266,-6.53784434718121));
#53872=CARTESIAN_POINT('Ctrl Pts',(-50.,-3.93897729264122,-6.43496121510494));
#53873=CARTESIAN_POINT('Ctrl Pts',(-50.,-3.87752560957259,-6.33279865263617));
#53874=CARTESIAN_POINT('Ctrl Pts',(-50.,-3.82734562477572,-6.25178572573963));
#53875=CARTESIAN_POINT('Ctrl Pts',(-50.,-3.78910264658076,-6.19145440139071));
#53876=CARTESIAN_POINT('Ctrl Pts',(-50.,-3.7633374392529,-6.15142367620606));
#53877=CARTESIAN_POINT('Ctrl Pts',(-50.,-3.75038736519793,-6.13145585166881));
#53878=CARTESIAN_POINT('',(-50.,-6.52388598275276,-7.57884632935924));
#53879=CARTESIAN_POINT('Origin',(-50.,0.,0.));
#53880=CARTESIAN_POINT('',(-50.,-5.14318775290069,-5.02073460645077));
#53881=CARTESIAN_POINT('Ctrl Pts',(-50.,-5.14318775290069,-5.02073460645076));
#53882=CARTESIAN_POINT('Ctrl Pts',(-50.,-5.15703844666268,-5.03529159113598));
#53883=CARTESIAN_POINT('Ctrl Pts',(-50.,-5.18485354740602,-5.06428722179623));
#53884=CARTESIAN_POINT('Ctrl Pts',(-50.,-5.22691734521339,-5.10742564369891));
#53885=CARTESIAN_POINT('Ctrl Pts',(-50.,-5.28368554926634,-5.16423261553338));
#53886=CARTESIAN_POINT('Ctrl Pts',(-50.,-5.35574541658332,-5.23409735978387));
#53887=CARTESIAN_POINT('Ctrl Pts',(-50.,-5.42877754716296,-5.30295185702147));
#53888=CARTESIAN_POINT('Ctrl Pts',(-50.,-5.50252175190725,-5.37106909242141));
#53889=CARTESIAN_POINT('Ctrl Pts',(-50.,-5.57653243923659,-5.43891687637388));
#53890=CARTESIAN_POINT('Ctrl Pts',(-50.,-5.65014634083023,-5.50719043557996));
#53891=CARTESIAN_POINT('Ctrl Pts',(-50.,-5.72258159055366,-5.57669744070723));
#53892=CARTESIAN_POINT('Ctrl Pts',(-50.,-5.79302399301176,-5.64825683559838));
#53893=CARTESIAN_POINT('Ctrl Pts',(-50.,-5.86071379627312,-5.72259822644884));
#53894=CARTESIAN_POINT('Ctrl Pts',(-50.,-5.92504262139805,-5.80024683316115));
#53895=CARTESIAN_POINT('Ctrl Pts',(-50.,-5.98561485393513,-5.88145719317904));
#53896=CARTESIAN_POINT('Ctrl Pts',(-50.,-6.04221154361855,-5.96627851638222));
#53897=CARTESIAN_POINT('Ctrl Pts',(-50.,-6.09477471117184,-6.05459405347559));
#53898=CARTESIAN_POINT('Ctrl Pts',(-50.,-6.14338347043832,-6.14616869769857));
#53899=CARTESIAN_POINT('Ctrl Pts',(-50.,-6.18823844577549,-6.2406935262026));
#53900=CARTESIAN_POINT('Ctrl Pts',(-50.,-6.22963155144596,-6.33782488040964));
#53901=CARTESIAN_POINT('Ctrl Pts',(-50.,-6.2678972444421,-6.43721103768399));
#53902=CARTESIAN_POINT('Ctrl Pts',(-50.,-6.30336681095649,-6.53852299564495));
#53903=CARTESIAN_POINT('Ctrl Pts',(-50.,-6.33632590879467,-6.64148049150319));
#53904=CARTESIAN_POINT('Ctrl Pts',(-50.,-6.36696110296949,-6.74588705654512));
#53905=CARTESIAN_POINT('Ctrl Pts',(-50.,-6.39534644338642,-6.85163598146165));
#53906=CARTESIAN_POINT('Ctrl Pts',(-50.,-6.42148411170256,-6.9586779143977));
#53907=CARTESIAN_POINT('Ctrl Pts',(-50.,-6.44533241567678,-7.06699729667253));
#53908=CARTESIAN_POINT('Ctrl Pts',(-50.,-6.46683693263443,-7.17658703219621));
#53909=CARTESIAN_POINT('Ctrl Pts',(-50.,-6.48596514159778,-7.28741967054497));
#53910=CARTESIAN_POINT('Ctrl Pts',(-50.,-6.5013152907357,-7.39001981975656));
#53911=CARTESIAN_POINT('Ctrl Pts',(-50.,-6.51181517907742,-7.47092388711047));
#53912=CARTESIAN_POINT('Ctrl Pts',(-50.,-6.5186172336226,-7.52956968091483));
#53913=CARTESIAN_POINT('Ctrl Pts',(-50.,-6.52249927647778,-7.56560518745242));
#53914=CARTESIAN_POINT('Ctrl Pts',(-50.,-6.52388598275276,-7.57884632935924));
#53915=CARTESIAN_POINT('',(-50.,-6.03932124977421,-3.89701874412038));
#53916=CARTESIAN_POINT('Origin',(-50.,0.,0.));
#53917=CARTESIAN_POINT('',(-50.,-8.85937132577942,-4.63805343996351));
#53918=CARTESIAN_POINT('Ctrl Pts',(-50.,-8.85937132577942,-4.63805343996351));
#53919=CARTESIAN_POINT('Ctrl Pts',(-50.,-8.83600957326199,-4.63860796949123));
#53920=CARTESIAN_POINT('Ctrl Pts',(-50.,-8.78542760184506,-4.64226869921731));
#53921=CARTESIAN_POINT('Ctrl Pts',(-50.,-8.70206879749976,-4.65426712072998));
#53922=CARTESIAN_POINT('Ctrl Pts',(-50.,-8.58208988181923,-4.67760996762605));
#53923=CARTESIAN_POINT('Ctrl Pts',(-50.,-8.43013206622476,-4.7059243222351));
#53924=CARTESIAN_POINT('Ctrl Pts',(-50.,-8.2843230642502,-4.72372591244526));
#53925=CARTESIAN_POINT('Ctrl Pts',(-50.,-8.14929412649754,-4.72756454905465));
#53926=CARTESIAN_POINT('Ctrl Pts',(-50.,-8.02313747309844,-4.71958541389958));
#53927=CARTESIAN_POINT('Ctrl Pts',(-50.,-7.9015907237349,-4.70439891524807));
#53928=CARTESIAN_POINT('Ctrl Pts',(-50.,-7.78000590743498,-4.68695765535521));
#53929=CARTESIAN_POINT('Ctrl Pts',(-50.,-7.65604731918147,-4.66963928443128));
#53930=CARTESIAN_POINT('Ctrl Pts',(-50.,-7.53031371454558,-4.65160090645338));
#53931=CARTESIAN_POINT('Ctrl Pts',(-50.,-7.40483002515176,-4.63046946729401));
#53932=CARTESIAN_POINT('Ctrl Pts',(-50.,-7.28216972266428,-4.60333867057275));
#53933=CARTESIAN_POINT('Ctrl Pts',(-50.,-7.16419105444418,-4.56819583049617));
#53934=CARTESIAN_POINT('Ctrl Pts',(-50.,-7.05136577826386,-4.52468089222283));
#53935=CARTESIAN_POINT('Ctrl Pts',(-50.,-6.94330777957998,-4.47348457408032));
#53936=CARTESIAN_POINT('Ctrl Pts',(-50.,-6.83906640781858,-4.4160130309926));
#53937=CARTESIAN_POINT('Ctrl Pts',(-50.,-6.73752748880879,-4.35393408054299));
#53938=CARTESIAN_POINT('Ctrl Pts',(-50.,-6.63770990687462,-4.2888323596294));
#53939=CARTESIAN_POINT('Ctrl Pts',(-50.,-6.53876341785232,-4.22215377357323));
#53940=CARTESIAN_POINT('Ctrl Pts',(-50.,-6.44000100425059,-4.15511874483724));
#53941=CARTESIAN_POINT('Ctrl Pts',(-50.,-6.34092094513049,-4.08864152493875));
#53942=CARTESIAN_POINT('Ctrl Pts',(-50.,-6.24122821720367,-4.02325912271413));
#53943=CARTESIAN_POINT('Ctrl Pts',(-50.,-6.16086742147115,-3.97204127711522));
#53944=CARTESIAN_POINT('Ctrl Pts',(-50.,-6.10023490810719,-3.93427763849175));
#53945=CARTESIAN_POINT('Ctrl Pts',(-50.,-6.05965257770704,-3.90939030583537));
#53946=CARTESIAN_POINT('Ctrl Pts',(-50.,-6.03932124977421,-3.89701874412038));
#53947=CARTESIAN_POINT('',(-50.,-9.16615635178499,-3.9976965535958));
#53948=CARTESIAN_POINT('Origin',(-50.,0.,0.));
#53949=CARTESIAN_POINT('',(-50.,-6.8122671513043,-2.29198004120026));
#53950=CARTESIAN_POINT('Ctrl Pts',(-50.,-6.8122671513043,-2.29198004120026));
#53951=CARTESIAN_POINT('Ctrl Pts',(-50.,-6.8310622341282,-2.29908584041335));
#53952=CARTESIAN_POINT('Ctrl Pts',(-50.,-6.86870350660446,-2.31314148102898));
#53953=CARTESIAN_POINT('Ctrl Pts',(-50.,-6.92531873868941,-2.33375705829959));
#53954=CARTESIAN_POINT('Ctrl Pts',(-50.,-7.00111274457534,-2.36030757076476));
#53955=CARTESIAN_POINT('Ctrl Pts',(-50.,-7.09634961812101,-2.39198792562662));
#53956=CARTESIAN_POINT('Ctrl Pts',(-50.,-7.19202414084635,-2.42233623016115));
#53957=CARTESIAN_POINT('Ctrl Pts',(-50.,-7.28802033430286,-2.45171132733138));
#53958=CARTESIAN_POINT('Ctrl Pts',(-50.,-7.3841397096708,-2.4807280346756));
#53959=CARTESIAN_POINT('Ctrl Pts',(-50.,-7.4800863304027,-2.5103005111467));
#53960=CARTESIAN_POINT('Ctrl Pts',(-50.,-7.57550619462173,-2.54149568187359));
#53961=CARTESIAN_POINT('Ctrl Pts',(-50.,-7.67002106404108,-2.5754046559055));
#53962=CARTESIAN_POINT('Ctrl Pts',(-50.,-7.76326299008741,-2.61301442971916));
#53963=CARTESIAN_POINT('Ctrl Pts',(-50.,-7.85491172665132,-2.65506217582471));
#53964=CARTESIAN_POINT('Ctrl Pts',(-50.,-7.94472127708621,-2.70194887521209));
#53965=CARTESIAN_POINT('Ctrl Pts',(-50.,-8.03251572538561,-2.75381386341092));
#53966=CARTESIAN_POINT('Ctrl Pts',(-50.,-8.11819217840571,-2.81057710920625));
#53967=CARTESIAN_POINT('Ctrl Pts',(-50.,-8.201719906256,-2.87199246251599));
#53968=CARTESIAN_POINT('Ctrl Pts',(-50.,-8.28314562863609,-2.93769454582461));
#53969=CARTESIAN_POINT('Ctrl Pts',(-50.,-8.36258324333989,-3.00724707660037));
#53970=CARTESIAN_POINT('Ctrl Pts',(-50.,-8.44018147897284,-3.08018804824792));
#53971=CARTESIAN_POINT('Ctrl Pts',(-50.,-8.51609606529771,-3.15607730017284));
#53972=CARTESIAN_POINT('Ctrl Pts',(-50.,-8.59046276963722,-3.23453838205034));
#53973=CARTESIAN_POINT('Ctrl Pts',(-50.,-8.66336443667969,-3.31531333416059));
#53974=CARTESIAN_POINT('Ctrl Pts',(-50.,-8.7348214836506,-3.3982738856883));
#53975=CARTESIAN_POINT('Ctrl Pts',(-50.,-8.80481446318767,-3.48337462556297));
#53976=CARTESIAN_POINT('Ctrl Pts',(-50.,-8.87329906122102,-3.57061962548306));
#53977=CARTESIAN_POINT('Ctrl Pts',(-50.,-8.94022316573707,-3.66002610520606));
#53978=CARTESIAN_POINT('Ctrl Pts',(-50.,-9.0055455660548,-3.75158344307814));
#53979=CARTESIAN_POINT('Ctrl Pts',(-50.,-9.06389210891971,-3.83736280325601));
#53980=CARTESIAN_POINT('Ctrl Pts',(-50.,-9.10845514068543,-3.90569911841461));
#53981=CARTESIAN_POINT('Ctrl Pts',(-50.,-9.14002903636781,-3.95558585200608));
#53982=CARTESIAN_POINT('Ctrl Pts',(-50.,-9.15916185644175,-3.9863683662662));
#53983=CARTESIAN_POINT('Ctrl Pts',(-50.,-9.16615635178519,-3.99769655359614));
#53984=CARTESIAN_POINT('',(-50.,-7.13209349341826,-0.89072928050049));
#53985=CARTESIAN_POINT('Origin',(-50.,0.,0.));
#53986=CARTESIAN_POINT('',(-50.,-9.99439372247306,-0.334804600014791));
#53987=CARTESIAN_POINT('Ctrl Pts',(-50.,-9.99439372247306,-0.334804600014791));
#53988=CARTESIAN_POINT('Ctrl Pts',(-50.,-9.97358611210015,-0.345440498390201));
#53989=CARTESIAN_POINT('Ctrl Pts',(-50.,-9.92960166167783,-0.370685396797522));
#53990=CARTESIAN_POINT('Ctrl Pts',(-50.,-9.85970389408656,-0.417663630762108));
#53991=CARTESIAN_POINT('Ctrl Pts',(-50.,-9.76173470794663,-0.490751709654423));
#53992=CARTESIAN_POINT('Ctrl Pts',(-50.,-9.63711058491003,-0.582194086890198));
#53993=CARTESIAN_POINT('Ctrl Pts',(-50.,-9.51346503399365,-0.66149692044243));
#53994=CARTESIAN_POINT('Ctrl Pts',(-50.,-9.39347368681776,-0.723542272923874));
#53995=CARTESIAN_POINT('Ctrl Pts',(-50.,-9.27634845263042,-0.771090641047726));
#53996=CARTESIAN_POINT('Ctrl Pts',(-50.,-9.1602494406401,-0.810145236641717));
#53997=CARTESIAN_POINT('Ctrl Pts',(-50.,-9.04313782728701,-0.847184879177381));
#53998=CARTESIAN_POINT('Ctrl Pts',(-50.,-8.92394083882956,-0.885365181899303));
#53999=CARTESIAN_POINT('Ctrl Pts',(-50.,-8.80283221651881,-0.923666931425906));
#54000=CARTESIAN_POINT('Ctrl Pts',(-50.,-8.68060673111004,-0.959073494961789));
#54001=CARTESIAN_POINT('Ctrl Pts',(-50.,-8.55832200571467,-0.98784980243911));
#54002=CARTESIAN_POINT('Ctrl Pts',(-50.,-8.43677899171613,-1.00737622330388));
#54003=CARTESIAN_POINT('Ctrl Pts',(-50.,-8.31624650623966,-1.017123671327));
#54004=CARTESIAN_POINT('Ctrl Pts',(-50.,-8.19667636355292,-1.01788199103989));
#54005=CARTESIAN_POINT('Ctrl Pts',(-50.,-8.0778221648407,-1.01133055607812));
#54006=CARTESIAN_POINT('Ctrl Pts',(-50.,-7.95940371279084,-0.999455440216892));
#54007=CARTESIAN_POINT('Ctrl Pts',(-50.,-7.84122460090589,-0.984110042106142));
#54008=CARTESIAN_POINT('Ctrl Pts',(-50.,-7.72314614047142,-0.966965984543332));
#54009=CARTESIAN_POINT('Ctrl Pts',(-50.,-7.60507887157754,-0.949420915891056));
#54010=CARTESIAN_POINT('Ctrl Pts',(-50.,-7.4869674381447,-0.932516236860826));
#54011=CARTESIAN_POINT('Ctrl Pts',(-50.,-7.36877903277666,-0.916863781503486));
#54012=CARTESIAN_POINT('Ctrl Pts',(-50.,-7.27415386726379,-0.90558533966873));
#54013=CARTESIAN_POINT('Ctrl Pts',(-50.,-7.20314083161155,-0.89786893854071));
#54014=CARTESIAN_POINT('Ctrl Pts',(-50.,-7.15577920638447,-0.893054239868308));
#54015=CARTESIAN_POINT('Ctrl Pts',(-50.,-7.13209349341826,-0.89072928050049));
#54016=CARTESIAN_POINT('',(-50.,-9.99295703981581,0.375246053138014));
#54017=CARTESIAN_POINT('Origin',(-50.,0.,0.));
#54018=CARTESIAN_POINT('',(-50.,-7.13209349341826,0.890729280500487));
#54019=CARTESIAN_POINT('Ctrl Pts',(-50.,-7.13209349341826,0.890729280500492));
#54020=CARTESIAN_POINT('Ctrl Pts',(-50.,-7.15211036864424,0.892482057440589));
#54021=CARTESIAN_POINT('Ctrl Pts',(-50.,-7.19212249719958,0.89615029887462));
#54022=CARTESIAN_POINT('Ctrl Pts',(-50.,-7.25207582250743,0.902140734147994));
#54023=CARTESIAN_POINT('Ctrl Pts',(-50.,-7.33188369780814,0.911105335666499));
#54024=CARTESIAN_POINT('Ctrl Pts',(-50.,-7.43143474677318,0.923884053007731));
#54025=CARTESIAN_POINT('Ctrl Pts',(-50.,-7.53080214904746,0.938052795086852));
#54026=CARTESIAN_POINT('Ctrl Pts',(-50.,-7.63003710778607,0.953237934402831));
#54027=CARTESIAN_POINT('Ctrl Pts',(-50.,-7.7292275500742,0.968799418422935));
#54028=CARTESIAN_POINT('Ctrl Pts',(-50.,-7.82850348500033,0.983785216334555));
#54029=CARTESIAN_POINT('Ctrl Pts',(-50.,-7.92800888935854,0.997080466154163));
#54030=CARTESIAN_POINT('Ctrl Pts',(-50.,-8.02787639670185,1.00753800115478));
#54031=CARTESIAN_POINT('Ctrl Pts',(-50.,-8.12820273854249,1.01410892133532));
#54032=CARTESIAN_POINT('Ctrl Pts',(-50.,-8.2290192302709,1.01599010763451));
#54033=CARTESIAN_POINT('Ctrl Pts',(-50.,-8.33027821569813,1.01271355471894));
#54034=CARTESIAN_POINT('Ctrl Pts',(-50.,-8.43188165539955,1.00407739851957));
#54035=CARTESIAN_POINT('Ctrl Pts',(-50.,-8.53370212161309,0.990109101007577));
#54036=CARTESIAN_POINT('Ctrl Pts',(-50.,-8.63560512714608,0.971017102543951));
#54037=CARTESIAN_POINT('Ctrl Pts',(-50.,-8.73747423363077,0.947150867813171));
#54038=CARTESIAN_POINT('Ctrl Pts',(-50.,-8.83922276353739,0.918952892194649));
#54039=CARTESIAN_POINT('Ctrl Pts',(-50.,-8.94078425956014,0.886903960171005));
#54040=CARTESIAN_POINT('Ctrl Pts',(-50.,-9.04210805084257,0.851468211346448));
#54041=CARTESIAN_POINT('Ctrl Pts',(-50.,-9.14315312384119,0.813043722977555));
#54042=CARTESIAN_POINT('Ctrl Pts',(-50.,-9.24388219451328,0.771898853704203));
#54043=CARTESIAN_POINT('Ctrl Pts',(-50.,-9.34425800352241,0.728158030239756));
#54044=CARTESIAN_POINT('Ctrl Pts',(-50.,-9.44424332627553,0.68185372865074));
#54045=CARTESIAN_POINT('Ctrl Pts',(-50.,-9.54380000381903,0.632963053309265));
#54046=CARTESIAN_POINT('Ctrl Pts',(-50.,-9.64288855622378,0.581447879194613));
#54047=CARTESIAN_POINT('Ctrl Pts',(-50.,-9.74146724538631,0.527299895441832));
#54048=CARTESIAN_POINT('Ctrl Pts',(-50.,-9.83125393359035,0.475330978595834));
#54049=CARTESIAN_POINT('Ctrl Pts',(-50.,-9.90105385380907,0.433097260939727));
#54050=CARTESIAN_POINT('Ctrl Pts',(-50.,-9.95114599336025,0.401850266969692));
#54051=CARTESIAN_POINT('Ctrl Pts',(-50.,-9.98174010098861,0.382417599459157));
#54052=CARTESIAN_POINT('Ctrl Pts',(-50.,-9.99295703981581,0.375246053138014));
#54053=CARTESIAN_POINT('',(-50.,-6.8122671513043,2.29198004120026));
#54054=CARTESIAN_POINT('Origin',(-50.,0.,0.));
#54055=CARTESIAN_POINT('',(-50.,-9.14990386923577,4.03475639707581));
#54056=CARTESIAN_POINT('Ctrl Pts',(-50.,-9.14990386923577,4.03475639707581));
#54057=CARTESIAN_POINT('Ctrl Pts',(-50.,-9.13577160343033,4.01614569996669));
#54058=CARTESIAN_POINT('Ctrl Pts',(-50.,-9.10709633384263,3.97431669461607));
#54059=CARTESIAN_POINT('Ctrl Pts',(-50.,-9.06450371311672,3.90166326358647));
#54060=CARTESIAN_POINT('Ctrl Pts',(-50.,-9.00794825534563,3.79330594308901));
#54061=CARTESIAN_POINT('Ctrl Pts',(-50.,-8.93534116084886,3.65684682750522));
#54062=CARTESIAN_POINT('Ctrl Pts',(-50.,-8.85834857876282,3.53174964938136));
#54063=CARTESIAN_POINT('Ctrl Pts',(-50.,-8.77716058006919,3.42378642402312));
#54064=CARTESIAN_POINT('Ctrl Pts',(-50.,-8.69226485417113,3.33012809006974));
#54065=CARTESIAN_POINT('Ctrl Pts',(-50.,-8.60460841273967,3.24456764186082));
#54066=CARTESIAN_POINT('Ctrl Pts',(-50.,-8.51516539363766,3.16038325236223));
#54067=CARTESIAN_POINT('Ctrl Pts',(-50.,-8.4243384303954,3.07426635319921));
#54068=CARTESIAN_POINT('Ctrl Pts',(-50.,-8.33184183835821,2.98721060740198));
#54069=CARTESIAN_POINT('Ctrl Pts',(-50.,-8.2370828133169,2.90227874531213));
#54070=CARTESIAN_POINT('Ctrl Pts',(-50.,-8.13939365460193,2.82329483425037));
#54071=CARTESIAN_POINT('Ctrl Pts',(-50.,-8.03835937937461,2.75296659957235));
#54072=CARTESIAN_POINT('Ctrl Pts',(-50.,-7.93399262158453,2.69188736687836));
#54073=CARTESIAN_POINT('Ctrl Pts',(-50.,-7.82659266808561,2.63932460382938));
#54074=CARTESIAN_POINT('Ctrl Pts',(-50.,-7.71666617412861,2.59365833862295));
#54075=CARTESIAN_POINT('Ctrl Pts',(-50.,-7.60482241577417,2.55297760756074));
#54076=CARTESIAN_POINT('Ctrl Pts',(-50.,-7.49168859641893,2.51552733857386));
#54077=CARTESIAN_POINT('Ctrl Pts',(-50.,-7.37786505179862,2.47974127678492));
#54078=CARTESIAN_POINT('Ctrl Pts',(-50.,-7.26387759821705,2.44432136933076));
#54079=CARTESIAN_POINT('Ctrl Pts',(-50.,-7.15012820840451,2.4083053284885));
#54080=CARTESIAN_POINT('Ctrl Pts',(-50.,-7.03685278876406,2.37112767623027));
#54081=CARTESIAN_POINT('Ctrl Pts',(-50.,-6.94670492800217,2.34023288057449));
#54082=CARTESIAN_POINT('Ctrl Pts',(-50.,-6.8793763726903,2.31637371632821));
#54083=CARTESIAN_POINT('Ctrl Pts',(-50.,-6.83461600336474,2.30016217089616));
#54084=CARTESIAN_POINT('Ctrl Pts',(-50.,-6.8122671513043,2.29198004120026));
#54085=CARTESIAN_POINT('',(-50.,-8.84053003053573,4.67386657695701));
#54086=CARTESIAN_POINT('Origin',(-50.,0.,0.));
#54087=CARTESIAN_POINT('',(-50.,-6.03932124977422,3.89701874412038));
#54088=CARTESIAN_POINT('Ctrl Pts',(-50.,-6.03932124977421,3.89701874412039));
#54089=CARTESIAN_POINT('Ctrl Pts',(-50.,-6.0565953297729,3.90728293824429));
#54090=CARTESIAN_POINT('Ctrl Pts',(-50.,-6.09105342163039,3.92794852152394));
#54091=CARTESIAN_POINT('Ctrl Pts',(-50.,-6.14247034880463,3.95935849016754));
#54092=CARTESIAN_POINT('Ctrl Pts',(-50.,-6.21048516503746,4.00206265639536));
#54093=CARTESIAN_POINT('Ctrl Pts',(-50.,-6.29463308326085,4.05676946424956));
#54094=CARTESIAN_POINT('Ctrl Pts',(-50.,-6.37801243240243,4.11264895980536));
#54095=CARTESIAN_POINT('Ctrl Pts',(-50.,-6.46083145580807,4.1693867325325));
#54096=CARTESIAN_POINT('Ctrl Pts',(-50.,-6.54344708143028,4.22644426515767));
#54097=CARTESIAN_POINT('Ctrl Pts',(-50.,-6.62638951409907,4.28302021638686));
#54098=CARTESIAN_POINT('Ctrl Pts',(-50.,-6.71027219290964,4.33817259947066));
#54099=CARTESIAN_POINT('Ctrl Pts',(-50.,-6.79571235355295,4.39092540044367));
#54100=CARTESIAN_POINT('Ctrl Pts',(-50.,-6.88325224876452,4.44037556328962));
#54101=CARTESIAN_POINT('Ctrl Pts',(-50.,-6.9732685530375,4.48581308997575));
#54102=CARTESIAN_POINT('Ctrl Pts',(-50.,-7.06592138953324,4.5267956450212));
#54103=CARTESIAN_POINT('Ctrl Pts',(-50.,-7.16121001331941,4.56309881747208));
#54104=CARTESIAN_POINT('Ctrl Pts',(-50.,-7.25900770064673,4.59469206087561));
#54105=CARTESIAN_POINT('Ctrl Pts',(-50.,-7.35910284385827,4.62170482170181));
#54106=CARTESIAN_POINT('Ctrl Pts',(-50.,-7.46123890856565,4.64440143603747));
#54107=CARTESIAN_POINT('Ctrl Pts',(-50.,-7.56514580946327,4.66314297047291));
#54108=CARTESIAN_POINT('Ctrl Pts',(-50.,-7.67055506601851,4.67833376211481));
#54109=CARTESIAN_POINT('Ctrl Pts',(-50.,-7.77721964274024,4.69037000103626));
#54110=CARTESIAN_POINT('Ctrl Pts',(-50.,-7.8849298684541,4.69959254734285));
#54111=CARTESIAN_POINT('Ctrl Pts',(-50.,-7.99353571494822,4.70622700687469));
#54112=CARTESIAN_POINT('Ctrl Pts',(-50.,-8.1029496259928,4.71036931800664));
#54113=CARTESIAN_POINT('Ctrl Pts',(-50.,-8.21312397255121,4.71203258951797));
#54114=CARTESIAN_POINT('Ctrl Pts',(-50.,-8.32403430863484,4.71117963661127));
#54115=CARTESIAN_POINT('Ctrl Pts',(-50.,-8.4356616058832,4.70775898013052));
#54116=CARTESIAN_POINT('Ctrl Pts',(-50.,-8.5479718655136,4.70174502276072));
#54117=CARTESIAN_POINT('Ctrl Pts',(-50.,-8.65141534429661,4.69387963058481));
#54118=CARTESIAN_POINT('Ctrl Pts',(-50.,-8.73262742272929,4.68611341617548));
#54119=CARTESIAN_POINT('Ctrl Pts',(-50.,-8.79131644357152,4.6796950122018));
#54120=CARTESIAN_POINT('Ctrl Pts',(-50.,-8.8273123005265,4.67546106956725));
#54121=CARTESIAN_POINT('Ctrl Pts',(-50.,-8.84053003053612,4.67386657695697));
#54122=CARTESIAN_POINT('',(-50.,-5.14318775290069,5.02073460645076));
#54123=CARTESIAN_POINT('Origin',(-50.,0.,0.));
#54124=CARTESIAN_POINT('',(-50.,-6.49316333848958,7.60518440668567));
#54125=CARTESIAN_POINT('Ctrl Pts',(-50.,-6.49316333848958,7.60518440668567));
#54126=CARTESIAN_POINT('Ctrl Pts',(-50.,-6.48850548581524,7.58228498765052));
#54127=CARTESIAN_POINT('Ctrl Pts',(-50.,-6.48081888588311,7.53215662286537));
#54128=CARTESIAN_POINT('Ctrl Pts',(-50.,-6.47396740292153,7.44821789782204));
#54129=CARTESIAN_POINT('Ctrl Pts',(-50.,-6.47002717553801,7.32605283195927));
#54130=CARTESIAN_POINT('Ctrl Pts',(-50.,-6.46381783511374,7.17160437943005));
#54131=CARTESIAN_POINT('Ctrl Pts',(-50.,-6.44872754699223,7.02548988707821));
#54132=CARTESIAN_POINT('Ctrl Pts',(-50.,-6.42242317562759,6.89299222970744));
#54133=CARTESIAN_POINT('Ctrl Pts',(-50.,-6.38657159771068,6.77177411160809));
#54134=CARTESIAN_POINT('Ctrl Pts',(-50.,-6.34471916009928,6.65665410688205));
#54135=CARTESIAN_POINT('Ctrl Pts',(-50.,-6.30066002212815,6.5419987212145));
#54136=CARTESIAN_POINT('Ctrl Pts',(-50.,-6.25619247809081,6.42500173364409));
#54137=CARTESIAN_POINT('Ctrl Pts',(-50.,-6.2106280007764,6.30643444970003));
#54138=CARTESIAN_POINT('Ctrl Pts',(-50.,-6.16210362315516,6.18879908596403));
#54139=CARTESIAN_POINT('Ctrl Pts',(-50.,-6.108358567083,6.07525130357771));
#54140=CARTESIAN_POINT('Ctrl Pts',(-50.,-6.04784410793973,5.96805062448362));
#54141=CARTESIAN_POINT('Ctrl Pts',(-50.,-5.98031419419066,5.86773709824143));
#54142=CARTESIAN_POINT('Ctrl Pts',(-50.,-5.906356307844,5.77378059171821));
#54143=CARTESIAN_POINT('Ctrl Pts',(-50.,-5.82712980893039,5.68494139022769));
#54144=CARTESIAN_POINT('Ctrl Pts',(-50.,-5.74401277228714,5.59976212994534));
#54145=CARTESIAN_POINT('Ctrl Pts',(-50.,-5.65833178588016,5.51693367893109));
#54146=CARTESIAN_POINT('Ctrl Pts',(-50.,-5.57130730604024,5.43530536621495));
#54147=CARTESIAN_POINT('Ctrl Pts',(-50.,-5.48397628091718,5.35393582972231));
#54148=CARTESIAN_POINT('Ctrl Pts',(-50.,-5.39711839642203,5.27213248760413));
#54149=CARTESIAN_POINT('Ctrl Pts',(-50.,-5.31119154860082,5.18948821771405));
#54150=CARTESIAN_POINT('Ctrl Pts',(-50.,-5.24337588200476,5.12253927774717));
#54151=CARTESIAN_POINT('Ctrl Pts',(-50.,-5.19306705314332,5.071830148219));
#54152=CARTESIAN_POINT('Ctrl Pts',(-50.,-5.1597732798141,5.03780325407688));
#54153=CARTESIAN_POINT('Ctrl Pts',(-50.,-5.14318775290069,5.02073460645076));
#54154=CARTESIAN_POINT('',(-50.,-5.93712762672243,8.04677050399782));
#54155=CARTESIAN_POINT('Origin',(-50.,0.,0.));
#54156=CARTESIAN_POINT('',(-50.,-3.75038736519794,6.13145585166881));
#54157=CARTESIAN_POINT('Ctrl Pts',(-50.,-3.75038736519793,6.13145585166881));
#54158=CARTESIAN_POINT('Ctrl Pts',(-50.,-3.7614973065729,6.1481985134482));
#54159=CARTESIAN_POINT('Ctrl Pts',(-50.,-3.78357651403939,6.1817683663582));
#54160=CARTESIAN_POINT('Ctrl Pts',(-50.,-3.81627329006595,6.23237673886416));
#54161=CARTESIAN_POINT('Ctrl Pts',(-50.,-3.859023878729,6.30036238594766));
#54162=CARTESIAN_POINT('Ctrl Pts',(-50.,-3.91110213900011,6.38616193008433));
#54163=CARTESIAN_POINT('Ctrl Pts',(-50.,-3.96197913233089,6.47268455970493));
#54164=CARTESIAN_POINT('Ctrl Pts',(-50.,-4.01197889710939,6.55973735411151));
#54165=CARTESIAN_POINT('Ctrl Pts',(-50.,-4.06165666819706,6.64698999124062));
#54166=CARTESIAN_POINT('Ctrl Pts',(-50.,-4.11183783259628,6.73395053478792));
#54167=CARTESIAN_POINT('Ctrl Pts',(-50.,-4.16348379256721,6.82003644526658));
#54168=CARTESIAN_POINT('Ctrl Pts',(-50.,-4.21757413484033,6.90463617300865));
#54169=CARTESIAN_POINT('Ctrl Pts',(-50.,-4.27498923356982,6.98717136730191));
#54170=CARTESIAN_POINT('Ctrl Pts',(-50.,-4.33637651734857,7.06716577496009));
#54171=CARTESIAN_POINT('Ctrl Pts',(-50.,-4.40207217433237,7.14429034032177));
#54172=CARTESIAN_POINT('Ctrl Pts',(-50.,-4.47217290162416,7.21834255288981));
#54173=CARTESIAN_POINT('Ctrl Pts',(-50.,-4.54657777868016,7.28923990788708));
#54174=CARTESIAN_POINT('Ctrl Pts',(-50.,-4.62503998887083,7.35700721943171));
#54175=CARTESIAN_POINT('Ctrl Pts',(-50.,-4.70721371156899,7.42177134000892));
#54176=CARTESIAN_POINT('Ctrl Pts',(-50.,-4.79269894740031,7.48374039375355));
#54177=CARTESIAN_POINT('Ctrl Pts',(-50.,-4.88107836846757,7.54316218647348));
#54178=CARTESIAN_POINT('Ctrl Pts',(-50.,-4.9719575030537,7.60028648840776));
#54179=CARTESIAN_POINT('Ctrl Pts',(-50.,-5.06499955030094,7.65532943098672));
#54180=CARTESIAN_POINT('Ctrl Pts',(-50.,-5.15997145275563,7.70842918324715));
#54181=CARTESIAN_POINT('Ctrl Pts',(-50.,-5.25675269887972,7.75963419345371));
#54182=CARTESIAN_POINT('Ctrl Pts',(-50.,-5.35529468870783,7.80893560674388));
#54183=CARTESIAN_POINT('Ctrl Pts',(-50.,-5.45559153104423,7.85628931405591));
#54184=CARTESIAN_POINT('Ctrl Pts',(-50.,-5.5576484178972,7.90164067817667));
#54185=CARTESIAN_POINT('Ctrl Pts',(-50.,-5.66144582368073,7.94495188520329));
#54186=CARTESIAN_POINT('Ctrl Pts',(-50.,-5.75805784341858,7.98274785508062));
#54187=CARTESIAN_POINT('Ctrl Pts',(-50.,-5.83459703193072,8.01098733792821));
#54188=CARTESIAN_POINT('Ctrl Pts',(-50.,-5.89025885371243,8.03066876757445));
#54189=CARTESIAN_POINT('Ctrl Pts',(-50.,-5.92452703906375,8.04247213408059));
#54190=CARTESIAN_POINT('Ctrl Pts',(-50.,-5.93712762672243,8.04677050399782));
#54191=CARTESIAN_POINT('',(-50.,-2.45543694297674,6.75507110762463));
#54192=CARTESIAN_POINT('Origin',(-50.,0.,0.));
#54193=CARTESIAN_POINT('',(-50.,-2.55037217513312,9.66931237308562));
#54194=CARTESIAN_POINT('Ctrl Pts',(-50.,-2.55037217513312,9.66931237308562));
#54195=CARTESIAN_POINT('Ctrl Pts',(-50.,-2.55611128043686,9.64665974290731));
#54196=CARTESIAN_POINT('Ctrl Pts',(-50.,-2.57093577554682,9.59816055611737));
#54197=CARTESIAN_POINT('Ctrl Pts',(-50.,-2.60118245057803,9.51956163099604));
#54198=CARTESIAN_POINT('Ctrl Pts',(-50.,-2.6506378639391,9.4077851093183));
#54199=CARTESIAN_POINT('Ctrl Pts',(-50.,-2.71205611361093,9.26593773005304));
#54200=CARTESIAN_POINT('Ctrl Pts',(-50.,-2.76185693608665,9.12774569066013));
#54201=CARTESIAN_POINT('Ctrl Pts',(-50.,-2.79564609540172,8.99695638729624));
#54202=CARTESIAN_POINT('Ctrl Pts',(-50.,-2.81593951016314,8.87218721998315));
#54203=CARTESIAN_POINT('Ctrl Pts',(-50.,-2.8281804649272,8.7503085875302));
#54204=CARTESIAN_POINT('Ctrl Pts',(-50.,-2.838231660712,8.62789111098118));
#54205=CARTESIAN_POINT('Ctrl Pts',(-50.,-2.84893087833482,8.50318672326558));
#54206=CARTESIAN_POINT('Ctrl Pts',(-50.,-2.85932311928695,8.37659160589212));
#54207=CARTESIAN_POINT('Ctrl Pts',(-50.,-2.8666442371861,8.24955186700095));
#54208=CARTESIAN_POINT('Ctrl Pts',(-50.,-2.86748815125169,8.12392974416385));
#54209=CARTESIAN_POINT('Ctrl Pts',(-50.,-2.85947913898695,8.00108902987832));
#54210=CARTESIAN_POINT('Ctrl Pts',(-50.,-2.84216119689693,7.88140953422486));
#54211=CARTESIAN_POINT('Ctrl Pts',(-50.,-2.81629364412744,7.76466852264525));
#54212=CARTESIAN_POINT('Ctrl Pts',(-50.,-2.78345892001629,7.65025207826714));
#54213=CARTESIAN_POINT('Ctrl Pts',(-50.,-2.74553095355499,7.53744508591865));
#54214=CARTESIAN_POINT('Ctrl Pts',(-50.,-2.70427297026251,7.42564364342468));
#54215=CARTESIAN_POINT('Ctrl Pts',(-50.,-2.66128382072048,7.31434056822034));
#54216=CARTESIAN_POINT('Ctrl Pts',(-50.,-2.61790620462629,7.20313763732345));
#54217=CARTESIAN_POINT('Ctrl Pts',(-50.,-2.57514309471485,7.09174914908801));
#54218=CARTESIAN_POINT('Ctrl Pts',(-50.,-2.53358368474749,6.98000697278327));
#54219=CARTESIAN_POINT('Ctrl Pts',(-50.,-2.50153193679118,6.89026394714059));
#54220=CARTESIAN_POINT('Ctrl Pts',(-50.,-2.47820711493347,6.82274841734025));
#54221=CARTESIAN_POINT('Ctrl Pts',(-50.,-2.46297417772978,6.77764561818537));
#54222=CARTESIAN_POINT('Ctrl Pts',(-50.,-2.45543694297674,6.75507110762463));
#54223=CARTESIAN_POINT('',(-50.,-1.85780428234483,9.82591284555797));
#54224=CARTESIAN_POINT('Origin',(-50.,0.,0.));
#54225=CARTESIAN_POINT('',(-50.,-0.718643267461628,7.15148293042304));
#54226=CARTESIAN_POINT('Ctrl Pts',(-50.,-0.718643267461623,7.15148293042304));
#54227=CARTESIAN_POINT('Ctrl Pts',(-50.,-0.721388610069065,7.17138797035723));
#54228=CARTESIAN_POINT('Ctrl Pts',(-50.,-0.726715875322121,7.21121317182152));
#54229=CARTESIAN_POINT('Ctrl Pts',(-50.,-0.734216502709279,7.2709963393441));
#54230=CARTESIAN_POINT('Ctrl Pts',(-50.,-0.743235585416284,7.35079807608913));
#54231=CARTESIAN_POINT('Ctrl Pts',(-50.,-0.752929449590466,7.45069670452966));
#54232=CARTESIAN_POINT('Ctrl Pts',(-50.,-0.761227274615912,7.55072560028829));
#54233=CARTESIAN_POINT('Ctrl Pts',(-50.,-0.768504714146027,7.65085154280962));
#54234=CARTESIAN_POINT('Ctrl Pts',(-50.,-0.775405338877351,7.75101782957587));
#54235=CARTESIAN_POINT('Ctrl Pts',(-50.,-0.782886239966145,7.85113936329068));
#54236=CARTESIAN_POINT('Ctrl Pts',(-50.,-0.792066365329069,7.95110843081948));
#54237=CARTESIAN_POINT('Ctrl Pts',(-50.,-0.804093633570273,8.05079907170372));
#54238=CARTESIAN_POINT('Ctrl Pts',(-50.,-0.82001217136434,8.15007218998677));
#54239=CARTESIAN_POINT('Ctrl Pts',(-50.,-0.840611930230858,8.24877960511329));
#54240=CARTESIAN_POINT('Ctrl Pts',(-50.,-0.86633857713272,8.34677071475058));
#54241=CARTESIAN_POINT('Ctrl Pts',(-50.,-0.897367099160985,8.4439050185459));
#54242=CARTESIAN_POINT('Ctrl Pts',(-50.,-0.933642367528788,8.5400643944807));
#54243=CARTESIAN_POINT('Ctrl Pts',(-50.,-0.974931241694467,8.63516410958082));
#54244=CARTESIAN_POINT('Ctrl Pts',(-50.,-1.02086710880846,8.72916840803945));
#54245=CARTESIAN_POINT('Ctrl Pts',(-50.,-1.07099928020948,8.82209124999857));
#54246=CARTESIAN_POINT('Ctrl Pts',(-50.,-1.12484423754393,8.91397482898789));
#54247=CARTESIAN_POINT('Ctrl Pts',(-50.,-1.18193820283021,9.00487302535333));
#54248=CARTESIAN_POINT('Ctrl Pts',(-50.,-1.24188395306769,9.09483443436949));
#54249=CARTESIAN_POINT('Ctrl Pts',(-50.,-1.30441156144786,9.18388242219763));
#54250=CARTESIAN_POINT('Ctrl Pts',(-50.,-1.3693914299125,9.27200835121914));
#54251=CARTESIAN_POINT('Ctrl Pts',(-50.,-1.43678361338666,9.35918315674388));
#54252=CARTESIAN_POINT('Ctrl Pts',(-50.,-1.50660194229105,9.44536454178638));
#54253=CARTESIAN_POINT('Ctrl Pts',(-50.,-1.57887480066182,9.53050553264656));
#54254=CARTESIAN_POINT('Ctrl Pts',(-50.,-1.65360100339141,9.61456358834088));
#54255=CARTESIAN_POINT('Ctrl Pts',(-50.,-1.72424636870649,9.69053496490015));
#54256=CARTESIAN_POINT('Ctrl Pts',(-50.,-1.78095314232183,9.74918696909221));
#54257=CARTESIAN_POINT('Ctrl Pts',(-50.,-1.82256325859186,9.79107008384009));
#54258=CARTESIAN_POINT('Ctrl Pts',(-50.,-1.8483165379591,9.81657295799161));
#54259=CARTESIAN_POINT('Ctrl Pts',(-50.,-1.85780428234511,9.82591284555825));
#54260=CARTESIAN_POINT('',(-50.,0.718643267461623,7.15148293042304));
#54261=CARTESIAN_POINT('Origin',(-50.,0.,0.));
#54262=CARTESIAN_POINT('',(-50.,1.89755147577054,9.81831443766195));
#54263=CARTESIAN_POINT('Ctrl Pts',(-50.,1.89755147577054,9.81831443766194));
#54264=CARTESIAN_POINT('Ctrl Pts',(-50.,1.88255211267964,9.80039522756355));
#54265=CARTESIAN_POINT('Ctrl Pts',(-50.,1.84815269559462,9.76313107751608));
#54266=CARTESIAN_POINT('Ctrl Pts',(-50.,1.78679858751167,9.70543943338958));
#54267=CARTESIAN_POINT('Ctrl Pts',(-50.,1.69374278455301,9.62619016686422));
#54268=CARTESIAN_POINT('Ctrl Pts',(-50.,1.576861582378,9.52503847397034));
#54269=CARTESIAN_POINT('Ctrl Pts',(-50.,1.47203331296336,9.42213951575228));
#54270=CARTESIAN_POINT('Ctrl Pts',(-50.,1.38484298036779,9.31896299195203));
#54271=CARTESIAN_POINT('Ctrl Pts',(-50.,1.31242393260393,9.21535483920498));
#54272=CARTESIAN_POINT('Ctrl Pts',(-50.,1.24851405668088,9.11085713692575));
#54273=CARTESIAN_POINT('Ctrl Pts',(-50.,1.18634328973517,9.00492385207762));
#54274=CARTESIAN_POINT('Ctrl Pts',(-50.,1.12259642171968,8.89721129760285));
#54275=CARTESIAN_POINT('Ctrl Pts',(-50.,1.05830577327405,8.78766206238304));
#54276=CARTESIAN_POINT('Ctrl Pts',(-50.,0.996589197042052,8.67637972666424));
#54277=CARTESIAN_POINT('Ctrl Pts',(-50.,0.941323460369316,8.56356426545847));
#54278=CARTESIAN_POINT('Ctrl Pts',(-50.,0.895240742652423,8.44941362598824));
#54279=CARTESIAN_POINT('Ctrl Pts',(-50.,0.858916682261844,8.33407215281038));
#54280=CARTESIAN_POINT('Ctrl Pts',(-50.,0.831570515383446,8.21766862525226));
#54281=CARTESIAN_POINT('Ctrl Pts',(-50.,0.811510144890448,8.10033651802127));
#54282=CARTESIAN_POINT('Ctrl Pts',(-50.,0.796736942256154,7.98224460192821));
#54283=CARTESIAN_POINT('Ctrl Pts',(-50.,0.785400272847098,7.86361381479518));
#54284=CARTESIAN_POINT('Ctrl Pts',(-50.,0.775839563797132,7.74468091618948));
#54285=CARTESIAN_POINT('Ctrl Pts',(-50.,0.766672302003445,7.62566969516693));
#54286=CARTESIAN_POINT('Ctrl Pts',(-50.,0.756870878958096,7.5067579169994));
#54287=CARTESIAN_POINT('Ctrl Pts',(-50.,0.745831500234843,7.38804974272502));
#54288=CARTESIAN_POINT('Ctrl Pts',(-50.,0.735771087779772,7.29328733826105));
#54289=CARTESIAN_POINT('Ctrl Pts',(-50.,0.72749213560466,7.22233768688913));
#54290=CARTESIAN_POINT('Ctrl Pts',(-50.,0.721647166649911,7.17509214524366));
#54291=CARTESIAN_POINT('Ctrl Pts',(-50.,0.718643267461623,7.15148293042304));
#54292=CARTESIAN_POINT('',(-50.,2.58947998462545,9.65891264114259));
#54293=CARTESIAN_POINT('Origin',(-50.,0.,0.));
#54294=CARTESIAN_POINT('',(-50.,2.45543694297674,6.75507110762463));
#54295=CARTESIAN_POINT('Ctrl Pts',(-50.,2.45543694297675,6.75507110762463));
#54296=CARTESIAN_POINT('Ctrl Pts',(-50.,2.46159994790965,6.77419608843537));
#54297=CARTESIAN_POINT('Ctrl Pts',(-50.,2.47407975508802,6.8123887688799));
#54298=CARTESIAN_POINT('Ctrl Pts',(-50.,2.49326086758344,6.8695059418988));
#54299=CARTESIAN_POINT('Ctrl Pts',(-50.,2.5197596307744,6.94531805563895));
#54300=CARTESIAN_POINT('Ctrl Pts',(-50.,2.55437015138428,7.03952961984441));
#54301=CARTESIAN_POINT('Ctrl Pts',(-50.,2.59029498067661,7.13325283216217));
#54302=CARTESIAN_POINT('Ctrl Pts',(-50.,2.62718125254576,7.22662075191781));
#54303=CARTESIAN_POINT('Ctrl Pts',(-50.,2.66442452752942,7.31986152676826));
#54304=CARTESIAN_POINT('Ctrl Pts',(-50.,2.70112557395893,7.41331375298832));
#54305=CARTESIAN_POINT('Ctrl Pts',(-50.,2.73622951961898,7.50736587770304));
#54306=CARTESIAN_POINT('Ctrl Pts',(-50.,2.76864747338962,7.60240247767684));
#54307=CARTESIAN_POINT('Ctrl Pts',(-50.,2.79737835816915,7.69875126136884));
#54308=CARTESIAN_POINT('Ctrl Pts',(-50.,2.82164615909785,7.79662146983088));
#54309=CARTESIAN_POINT('Ctrl Pts',(-50.,2.84098400021345,7.89607078269802));
#54310=CARTESIAN_POINT('Ctrl Pts',(-50.,2.85517326277626,7.9970485375799));
#54311=CARTESIAN_POINT('Ctrl Pts',(-50.,2.86421236488386,8.099424390731));
#54312=CARTESIAN_POINT('Ctrl Pts',(-50.,2.8682745946465,8.20302084448955));
#54313=CARTESIAN_POINT('Ctrl Pts',(-50.,2.86767474496505,8.30764661663281));
#54314=CARTESIAN_POINT('Ctrl Pts',(-50.,2.86282492937103,8.41311873833255));
#54315=CARTESIAN_POINT('Ctrl Pts',(-50.,2.85417908993455,8.51926543389428));
#54316=CARTESIAN_POINT('Ctrl Pts',(-50.,2.84217845398458,8.62593402210748));
#54317=CARTESIAN_POINT('Ctrl Pts',(-50.,2.82720199177778,8.73299593720093));
#54318=CARTESIAN_POINT('Ctrl Pts',(-50.,2.80950303716262,8.84035511450549));
#54319=CARTESIAN_POINT('Ctrl Pts',(-50.,2.78919460623265,8.94794754130566));
#54320=CARTESIAN_POINT('Ctrl Pts',(-50.,2.76630007756038,9.05572969970197));
#54321=CARTESIAN_POINT('Ctrl Pts',(-50.,2.74078863839312,9.16366948222194));
#54322=CARTESIAN_POINT('Ctrl Pts',(-50.,2.71261433447332,9.27173688239595));
#54323=CARTESIAN_POINT('Ctrl Pts',(-50.,2.68175977570501,9.37989305792331));
#54324=CARTESIAN_POINT('Ctrl Pts',(-50.,2.65107324582199,9.47899277830907));
#54325=CARTESIAN_POINT('Ctrl Pts',(-50.,2.62543035908099,9.55644055509564));
#54326=CARTESIAN_POINT('Ctrl Pts',(-50.,2.60611334216463,9.61222989040654));
#54327=CARTESIAN_POINT('Ctrl Pts',(-50.,2.59397572160348,9.64638111520543));
#54328=CARTESIAN_POINT('Ctrl Pts',(-50.,2.58947998462545,9.65891264114259));
#54329=CARTESIAN_POINT('',(-50.,3.75038736519793,6.13145585166881));
#54330=CARTESIAN_POINT('Origin',(-50.,0.,0.));
#54331=CARTESIAN_POINT('',(-50.,5.96964178495622,8.0226789141349));
#54332=CARTESIAN_POINT('Ctrl Pts',(-50.,5.96964178495622,8.0226789141349));
#54333=CARTESIAN_POINT('Ctrl Pts',(-50.,5.94835297189343,8.0130422434411));
#54334=CARTESIAN_POINT('Ctrl Pts',(-50.,5.9011918592682,7.9943937520678));
#54335=CARTESIAN_POINT('Ctrl Pts',(-50.,5.82088225169809,7.96903592659697));
#54336=CARTESIAN_POINT('Ctrl Pts',(-50.,5.70265690217233,7.93801020438781));
#54337=CARTESIAN_POINT('Ctrl Pts',(-50.,5.55346250303877,7.89758853118705));
#54338=CARTESIAN_POINT('Ctrl Pts',(-50.,5.41436931107715,7.85036305479183));
#54339=CARTESIAN_POINT('Ctrl Pts',(-50.,5.29104691989087,7.79523468647088));
#54340=CARTESIAN_POINT('Ctrl Pts',(-50.,5.18084571969554,7.73330841361203));
#54341=CARTESIAN_POINT('Ctrl Pts',(-50.,5.07792505734327,7.66688869302314));
#54342=CARTESIAN_POINT('Ctrl Pts',(-50.,4.97594840210465,7.59842098612655));
#54343=CARTESIAN_POINT('Ctrl Pts',(-50.,4.87177973271099,7.52903405731413));
#54344=CARTESIAN_POINT('Ctrl Pts',(-50.,4.76632422816958,7.45822827381644));
#54345=CARTESIAN_POINT('Ctrl Pts',(-50.,4.66243591843161,7.38474417264741));
#54346=CARTESIAN_POINT('Ctrl Pts',(-50.,4.56369441608956,7.30707985875561));
#54347=CARTESIAN_POINT('Ctrl Pts',(-50.,4.4726472158023,7.22422822821349));
#54348=CARTESIAN_POINT('Ctrl Pts',(-50.,4.38987557857684,7.13606957084443));
#54349=CARTESIAN_POINT('Ctrl Pts',(-50.,4.31473193577955,7.04305867353628));
#54350=CARTESIAN_POINT('Ctrl Pts',(-50.,4.24574967308284,6.94604996627335));
#54351=CARTESIAN_POINT('Ctrl Pts',(-50.,4.18120131531612,6.84606267872027));
#54352=CARTESIAN_POINT('Ctrl Pts',(-50.,4.11951535961712,6.74409882925098));
#54353=CARTESIAN_POINT('Ctrl Pts',(-50.,4.05929840765689,6.64109222642907));
#54354=CARTESIAN_POINT('Ctrl Pts',(-50.,3.99940195660266,6.53784434718121));
#54355=CARTESIAN_POINT('Ctrl Pts',(-50.,3.93897729264122,6.43496121510494));
#54356=CARTESIAN_POINT('Ctrl Pts',(-50.,3.87752560957259,6.33279865263617));
#54357=CARTESIAN_POINT('Ctrl Pts',(-50.,3.82734562477572,6.25178572573963));
#54358=CARTESIAN_POINT('Ctrl Pts',(-50.,3.78910264658076,6.19145440139071));
#54359=CARTESIAN_POINT('Ctrl Pts',(-50.,3.7633374392529,6.15142367620606));
#54360=CARTESIAN_POINT('Ctrl Pts',(-50.,3.75038736519793,6.13145585166881));
#54361=CARTESIAN_POINT('',(-50.,6.52388598275276,7.57884632935924));
#54362=CARTESIAN_POINT('Origin',(-50.,0.,0.));
#54363=CARTESIAN_POINT('',(-50.,5.14318775290069,5.02073460645077));
#54364=CARTESIAN_POINT('Ctrl Pts',(-50.,5.14318775290069,5.02073460645076));
#54365=CARTESIAN_POINT('Ctrl Pts',(-50.,5.15703844666268,5.03529159113598));
#54366=CARTESIAN_POINT('Ctrl Pts',(-50.,5.18485354740602,5.06428722179623));
#54367=CARTESIAN_POINT('Ctrl Pts',(-50.,5.22691734521339,5.10742564369892));
#54368=CARTESIAN_POINT('Ctrl Pts',(-50.,5.28368554926634,5.16423261553338));
#54369=CARTESIAN_POINT('Ctrl Pts',(-50.,5.35574541658332,5.23409735978387));
#54370=CARTESIAN_POINT('Ctrl Pts',(-50.,5.42877754716296,5.30295185702147));
#54371=CARTESIAN_POINT('Ctrl Pts',(-50.,5.50252175190725,5.37106909242141));
#54372=CARTESIAN_POINT('Ctrl Pts',(-50.,5.57653243923659,5.43891687637388));
#54373=CARTESIAN_POINT('Ctrl Pts',(-50.,5.65014634083023,5.50719043557996));
#54374=CARTESIAN_POINT('Ctrl Pts',(-50.,5.72258159055366,5.57669744070723));
#54375=CARTESIAN_POINT('Ctrl Pts',(-50.,5.79302399301176,5.64825683559838));
#54376=CARTESIAN_POINT('Ctrl Pts',(-50.,5.86071379627312,5.72259822644884));
#54377=CARTESIAN_POINT('Ctrl Pts',(-50.,5.92504262139805,5.80024683316115));
#54378=CARTESIAN_POINT('Ctrl Pts',(-50.,5.98561485393513,5.88145719317904));
#54379=CARTESIAN_POINT('Ctrl Pts',(-50.,6.04221154361855,5.96627851638222));
#54380=CARTESIAN_POINT('Ctrl Pts',(-50.,6.09477471117184,6.05459405347559));
#54381=CARTESIAN_POINT('Ctrl Pts',(-50.,6.14338347043832,6.14616869769857));
#54382=CARTESIAN_POINT('Ctrl Pts',(-50.,6.18823844577549,6.2406935262026));
#54383=CARTESIAN_POINT('Ctrl Pts',(-50.,6.22963155144596,6.33782488040965));
#54384=CARTESIAN_POINT('Ctrl Pts',(-50.,6.2678972444421,6.43721103768399));
#54385=CARTESIAN_POINT('Ctrl Pts',(-50.,6.30336681095649,6.53852299564495));
#54386=CARTESIAN_POINT('Ctrl Pts',(-50.,6.33632590879467,6.64148049150319));
#54387=CARTESIAN_POINT('Ctrl Pts',(-50.,6.36696110296949,6.74588705654512));
#54388=CARTESIAN_POINT('Ctrl Pts',(-50.,6.39534644338642,6.85163598146165));
#54389=CARTESIAN_POINT('Ctrl Pts',(-50.,6.42148411170256,6.95867791439771));
#54390=CARTESIAN_POINT('Ctrl Pts',(-50.,6.44533241567678,7.06699729667253));
#54391=CARTESIAN_POINT('Ctrl Pts',(-50.,6.46683693263443,7.17658703219621));
#54392=CARTESIAN_POINT('Ctrl Pts',(-50.,6.48596514159778,7.28741967054497));
#54393=CARTESIAN_POINT('Ctrl Pts',(-50.,6.50131529073571,7.39001981975663));
#54394=CARTESIAN_POINT('Ctrl Pts',(-50.,6.51181517907743,7.47092388711063));
#54395=CARTESIAN_POINT('Ctrl Pts',(-50.,6.51861723362263,7.52956968091507));
#54396=CARTESIAN_POINT('Ctrl Pts',(-50.,6.52249927647781,7.56560518745274));
#54397=CARTESIAN_POINT('Ctrl Pts',(-50.,6.52388598275281,7.57884632935963));
#54398=CARTESIAN_POINT('',(-50.,6.03932124977421,3.89701874412038));
#54399=CARTESIAN_POINT('Origin',(-50.,0.,0.));
#54400=CARTESIAN_POINT('',(-50.,8.85937132577942,4.63805343996351));
#54401=CARTESIAN_POINT('Ctrl Pts',(-50.,8.85937132577942,4.63805343996351));
#54402=CARTESIAN_POINT('Ctrl Pts',(-50.,8.83600957326198,4.63860796949123));
#54403=CARTESIAN_POINT('Ctrl Pts',(-50.,8.78542760184506,4.64226869921732));
#54404=CARTESIAN_POINT('Ctrl Pts',(-50.,8.70206879749976,4.65426712072998));
#54405=CARTESIAN_POINT('Ctrl Pts',(-50.,8.58208988181924,4.67760996762605));
#54406=CARTESIAN_POINT('Ctrl Pts',(-50.,8.43013206622476,4.70592432223511));
#54407=CARTESIAN_POINT('Ctrl Pts',(-50.,8.2843230642502,4.72372591244527));
#54408=CARTESIAN_POINT('Ctrl Pts',(-50.,8.14929412649754,4.72756454905465));
#54409=CARTESIAN_POINT('Ctrl Pts',(-50.,8.02313747309844,4.71958541389958));
#54410=CARTESIAN_POINT('Ctrl Pts',(-50.,7.9015907237349,4.70439891524807));
#54411=CARTESIAN_POINT('Ctrl Pts',(-50.,7.78000590743498,4.68695765535521));
#54412=CARTESIAN_POINT('Ctrl Pts',(-50.,7.65604731918147,4.66963928443128));
#54413=CARTESIAN_POINT('Ctrl Pts',(-50.,7.53031371454558,4.65160090645339));
#54414=CARTESIAN_POINT('Ctrl Pts',(-50.,7.40483002515176,4.63046946729401));
#54415=CARTESIAN_POINT('Ctrl Pts',(-50.,7.28216972266428,4.60333867057275));
#54416=CARTESIAN_POINT('Ctrl Pts',(-50.,7.16419105444418,4.56819583049617));
#54417=CARTESIAN_POINT('Ctrl Pts',(-50.,7.05136577826386,4.52468089222283));
#54418=CARTESIAN_POINT('Ctrl Pts',(-50.,6.94330777957998,4.47348457408032));
#54419=CARTESIAN_POINT('Ctrl Pts',(-50.,6.83906640781858,4.4160130309926));
#54420=CARTESIAN_POINT('Ctrl Pts',(-50.,6.73752748880879,4.35393408054299));
#54421=CARTESIAN_POINT('Ctrl Pts',(-50.,6.63770990687462,4.2888323596294));
#54422=CARTESIAN_POINT('Ctrl Pts',(-50.,6.53876341785232,4.22215377357323));
#54423=CARTESIAN_POINT('Ctrl Pts',(-50.,6.44000100425059,4.15511874483725));
#54424=CARTESIAN_POINT('Ctrl Pts',(-50.,6.34092094513049,4.08864152493875));
#54425=CARTESIAN_POINT('Ctrl Pts',(-50.,6.24122821720367,4.02325912271413));
#54426=CARTESIAN_POINT('Ctrl Pts',(-50.,6.16086742147114,3.97204127711522));
#54427=CARTESIAN_POINT('Ctrl Pts',(-50.,6.10023490810719,3.93427763849175));
#54428=CARTESIAN_POINT('Ctrl Pts',(-50.,6.05965257770704,3.90939030583537));
#54429=CARTESIAN_POINT('Ctrl Pts',(-50.,6.03932124977421,3.89701874412038));
#54430=CARTESIAN_POINT('',(-50.,9.16615635178499,3.9976965535958));
#54431=CARTESIAN_POINT('Origin',(-50.,0.,0.));
#54432=CARTESIAN_POINT('',(-50.,6.8122671513043,2.29198004120026));
#54433=CARTESIAN_POINT('Ctrl Pts',(-50.,6.8122671513043,2.29198004120026));
#54434=CARTESIAN_POINT('Ctrl Pts',(-50.,6.8310622341282,2.29908584041335));
#54435=CARTESIAN_POINT('Ctrl Pts',(-50.,6.86870350660446,2.31314148102898));
#54436=CARTESIAN_POINT('Ctrl Pts',(-50.,6.92531873868941,2.33375705829959));
#54437=CARTESIAN_POINT('Ctrl Pts',(-50.,7.00111274457534,2.36030757076476));
#54438=CARTESIAN_POINT('Ctrl Pts',(-50.,7.09634961812101,2.39198792562662));
#54439=CARTESIAN_POINT('Ctrl Pts',(-50.,7.19202414084635,2.42233623016115));
#54440=CARTESIAN_POINT('Ctrl Pts',(-50.,7.28802033430286,2.45171132733138));
#54441=CARTESIAN_POINT('Ctrl Pts',(-50.,7.3841397096708,2.4807280346756));
#54442=CARTESIAN_POINT('Ctrl Pts',(-50.,7.4800863304027,2.5103005111467));
#54443=CARTESIAN_POINT('Ctrl Pts',(-50.,7.57550619462173,2.54149568187359));
#54444=CARTESIAN_POINT('Ctrl Pts',(-50.,7.67002106404108,2.5754046559055));
#54445=CARTESIAN_POINT('Ctrl Pts',(-50.,7.76326299008741,2.61301442971916));
#54446=CARTESIAN_POINT('Ctrl Pts',(-50.,7.85491172665132,2.65506217582471));
#54447=CARTESIAN_POINT('Ctrl Pts',(-50.,7.94472127708621,2.70194887521209));
#54448=CARTESIAN_POINT('Ctrl Pts',(-50.,8.03251572538561,2.75381386341092));
#54449=CARTESIAN_POINT('Ctrl Pts',(-50.,8.11819217840571,2.81057710920625));
#54450=CARTESIAN_POINT('Ctrl Pts',(-50.,8.201719906256,2.87199246251599));
#54451=CARTESIAN_POINT('Ctrl Pts',(-50.,8.28314562863609,2.93769454582461));
#54452=CARTESIAN_POINT('Ctrl Pts',(-50.,8.36258324333989,3.00724707660037));
#54453=CARTESIAN_POINT('Ctrl Pts',(-50.,8.44018147897284,3.08018804824792));
#54454=CARTESIAN_POINT('Ctrl Pts',(-50.,8.51609606529771,3.15607730017284));
#54455=CARTESIAN_POINT('Ctrl Pts',(-50.,8.59046276963722,3.23453838205034));
#54456=CARTESIAN_POINT('Ctrl Pts',(-50.,8.66336443667969,3.31531333416059));
#54457=CARTESIAN_POINT('Ctrl Pts',(-50.,8.7348214836506,3.3982738856883));
#54458=CARTESIAN_POINT('Ctrl Pts',(-50.,8.80481446318767,3.48337462556297));
#54459=CARTESIAN_POINT('Ctrl Pts',(-50.,8.87329906122102,3.57061962548306));
#54460=CARTESIAN_POINT('Ctrl Pts',(-50.,8.94022316573707,3.66002610520606));
#54461=CARTESIAN_POINT('Ctrl Pts',(-50.,9.0055455660548,3.75158344307814));
#54462=CARTESIAN_POINT('Ctrl Pts',(-50.,9.06389210891971,3.83736280325601));
#54463=CARTESIAN_POINT('Ctrl Pts',(-50.,9.10845514068543,3.90569911841461));
#54464=CARTESIAN_POINT('Ctrl Pts',(-50.,9.1400290363678,3.95558585200609));
#54465=CARTESIAN_POINT('Ctrl Pts',(-50.,9.15916185644175,3.9863683662662));
#54466=CARTESIAN_POINT('Ctrl Pts',(-50.,9.16615635178519,3.99769655359614));
#54467=CARTESIAN_POINT('',(-50.,7.13209349341826,0.890729280500491));
#54468=CARTESIAN_POINT('Origin',(-50.,0.,0.));
#54469=CARTESIAN_POINT('Ctrl Pts',(-50.,9.99439372247306,0.334804600014792));
#54470=CARTESIAN_POINT('Ctrl Pts',(-50.,9.97358611210015,0.345440498390202));
#54471=CARTESIAN_POINT('Ctrl Pts',(-50.,9.92960166167783,0.370685396797523));
#54472=CARTESIAN_POINT('Ctrl Pts',(-50.,9.85970389408656,0.417663630762109));
#54473=CARTESIAN_POINT('Ctrl Pts',(-50.,9.76173470794663,0.490751709654424));
#54474=CARTESIAN_POINT('Ctrl Pts',(-50.,9.63711058491003,0.582194086890199));
#54475=CARTESIAN_POINT('Ctrl Pts',(-50.,9.51346503399365,0.661496920442432));
#54476=CARTESIAN_POINT('Ctrl Pts',(-50.,9.39347368681776,0.723542272923875));
#54477=CARTESIAN_POINT('Ctrl Pts',(-50.,9.27634845263042,0.771090641047727));
#54478=CARTESIAN_POINT('Ctrl Pts',(-50.,9.1602494406401,0.810145236641718));
#54479=CARTESIAN_POINT('Ctrl Pts',(-50.,9.04313782728701,0.847184879177382));
#54480=CARTESIAN_POINT('Ctrl Pts',(-50.,8.92394083882956,0.885365181899305));
#54481=CARTESIAN_POINT('Ctrl Pts',(-50.,8.80283221651881,0.923666931425907));
#54482=CARTESIAN_POINT('Ctrl Pts',(-50.,8.68060673111004,0.95907349496179));
#54483=CARTESIAN_POINT('Ctrl Pts',(-50.,8.55832200571467,0.987849802439111));
#54484=CARTESIAN_POINT('Ctrl Pts',(-50.,8.43677899171613,1.00737622330388));
#54485=CARTESIAN_POINT('Ctrl Pts',(-50.,8.31624650623966,1.017123671327));
#54486=CARTESIAN_POINT('Ctrl Pts',(-50.,8.19667636355292,1.01788199103989));
#54487=CARTESIAN_POINT('Ctrl Pts',(-50.,8.0778221648407,1.01133055607812));
#54488=CARTESIAN_POINT('Ctrl Pts',(-50.,7.95940371279084,0.999455440216893));
#54489=CARTESIAN_POINT('Ctrl Pts',(-50.,7.84122460090589,0.984110042106143));
#54490=CARTESIAN_POINT('Ctrl Pts',(-50.,7.72314614047142,0.966965984543333));
#54491=CARTESIAN_POINT('Ctrl Pts',(-50.,7.60507887157754,0.949420915891057));
#54492=CARTESIAN_POINT('Ctrl Pts',(-50.,7.4869674381447,0.932516236860827));
#54493=CARTESIAN_POINT('Ctrl Pts',(-50.,7.36877903277666,0.916863781503487));
#54494=CARTESIAN_POINT('Ctrl Pts',(-50.,7.27415386726379,0.90558533966873));
#54495=CARTESIAN_POINT('Ctrl Pts',(-50.,7.20314083161155,0.897868938540711));
#54496=CARTESIAN_POINT('Ctrl Pts',(-50.,7.15577920638447,0.893054239868309));
#54497=CARTESIAN_POINT('Ctrl Pts',(-50.,7.13209349341826,0.890729280500491));
#54498=CARTESIAN_POINT('Origin',(-35.75,0.,0.));
#54499=CARTESIAN_POINT('',(-21.5,5.93712762672243,-8.04677050399782));
#54500=CARTESIAN_POINT('Origin',(-21.5,0.,0.));
#54501=CARTESIAN_POINT('Ctrl Pts',(-21.5,5.93712762672243,-8.04677050399782));
#54502=CARTESIAN_POINT('Ctrl Pts',(-26.3333333333333,5.93712762672243,-8.04677050399782));
#54503=CARTESIAN_POINT('Ctrl Pts',(-31.1666666666667,5.93712762672243,-8.04677050399782));
#54504=CARTESIAN_POINT('Ctrl Pts',(-40.6666666666667,5.93712762672243,-8.04677050399782));
#54505=CARTESIAN_POINT('Ctrl Pts',(-45.3333333333333,5.93712762672243,-8.04677050399782));
#54506=CARTESIAN_POINT('Ctrl Pts',(-50.,5.93712762672243,-8.04677050399782));
#54507=CARTESIAN_POINT('Origin',(-21.25,0.,0.));
#54508=CARTESIAN_POINT('Ctrl Pts',(-21.,5.38825861761966,-7.82410819644306));
#54509=CARTESIAN_POINT('Ctrl Pts',(-21.1171767610852,5.51032506808644,-7.88231976704313));
#54510=CARTESIAN_POINT('Ctrl Pts',(-21.2874825276342,5.69235044789971,-7.96327099664331));
#54511=CARTESIAN_POINT('Ctrl Pts',(-21.5,5.93712762672243,-8.04677050399782));
#54512=CARTESIAN_POINT('Ctrl Pts',(-50.,6.6617400018565,-8.24507247679879));
#54513=CARTESIAN_POINT('Ctrl Pts',(-21.,6.6617400018565,-8.24507247679879));
#54514=CARTESIAN_POINT('Ctrl Pts',(-50.,6.63837938775657,-8.24010262588658));
#54515=CARTESIAN_POINT('Ctrl Pts',(-21.,6.63837938775657,-8.24010262588658));
#54516=CARTESIAN_POINT('Ctrl Pts',(-50.,6.59177764993375,-8.2299772134607));
#54517=CARTESIAN_POINT('Ctrl Pts',(-21.,6.59177764993375,-8.2299772134607));
#54518=CARTESIAN_POINT('Ctrl Pts',(-50.,6.52223351516926,-8.21423196280605));
#54519=CARTESIAN_POINT('Ctrl Pts',(-21.,6.52223351516926,-8.21423196280605));
#54520=CARTESIAN_POINT('Ctrl Pts',(-50.,6.43022589217209,-8.1921225513));
#54521=CARTESIAN_POINT('Ctrl Pts',(-21.,6.43022589217209,-8.1921225513));
#54522=CARTESIAN_POINT('Ctrl Pts',(-50.,6.31642365942377,-8.16261538830187));
#54523=CARTESIAN_POINT('Ctrl Pts',(-21.,6.31642365942377,-8.16261538830187));
#54524=CARTESIAN_POINT('Ctrl Pts',(-50.,6.20385140809547,-8.1312203551374));
#54525=CARTESIAN_POINT('Ctrl Pts',(-21.,6.20385140809547,-8.1312203551374));
#54526=CARTESIAN_POINT('Ctrl Pts',(-50.,6.09254749437728,-8.0979137913074));
#54527=CARTESIAN_POINT('Ctrl Pts',(-21.,6.09254749437728,-8.0979137913074));
#54528=CARTESIAN_POINT('Ctrl Pts',(-50.,5.9825687506924,-8.06266677783295));
#54529=CARTESIAN_POINT('Ctrl Pts',(-21.,5.9825687506924,-8.06266677783295));
#54530=CARTESIAN_POINT('Ctrl Pts',(-50.,5.87399565540877,-8.02544535222689));
#54531=CARTESIAN_POINT('Ctrl Pts',(-21.,5.87399565540877,-8.02544535222689));
#54532=CARTESIAN_POINT('Ctrl Pts',(-50.,5.7669227832391,-7.98621594320599));
#54533=CARTESIAN_POINT('Ctrl Pts',(-21.,5.7669227832391,-7.98621594320599));
#54534=CARTESIAN_POINT('Ctrl Pts',(-50.,5.66144582368073,-7.94495188520329));
#54535=CARTESIAN_POINT('Ctrl Pts',(-21.,5.66144582368073,-7.94495188520329));
#54536=CARTESIAN_POINT('Ctrl Pts',(-50.,5.5576484178972,-7.90164067817667));
#54537=CARTESIAN_POINT('Ctrl Pts',(-21.,5.5576484178972,-7.90164067817667));
#54538=CARTESIAN_POINT('Ctrl Pts',(-50.,5.45559153104423,-7.85628931405591));
#54539=CARTESIAN_POINT('Ctrl Pts',(-21.,5.45559153104423,-7.85628931405591));
#54540=CARTESIAN_POINT('Ctrl Pts',(-50.,5.35529468870783,-7.80893560674388));
#54541=CARTESIAN_POINT('Ctrl Pts',(-21.,5.35529468870783,-7.80893560674388));
#54542=CARTESIAN_POINT('Ctrl Pts',(-50.,5.25675269887972,-7.75963419345371));
#54543=CARTESIAN_POINT('Ctrl Pts',(-21.,5.25675269887972,-7.75963419345371));
#54544=CARTESIAN_POINT('Ctrl Pts',(-50.,5.15997145275563,-7.70842918324715));
#54545=CARTESIAN_POINT('Ctrl Pts',(-21.,5.15997145275563,-7.70842918324715));
#54546=CARTESIAN_POINT('Ctrl Pts',(-50.,5.06499955030093,-7.65532943098672));
#54547=CARTESIAN_POINT('Ctrl Pts',(-21.,5.06499955030093,-7.65532943098672));
#54548=CARTESIAN_POINT('Ctrl Pts',(-50.,4.9719575030537,-7.60028648840776));
#54549=CARTESIAN_POINT('Ctrl Pts',(-21.,4.9719575030537,-7.60028648840776));
#54550=CARTESIAN_POINT('Ctrl Pts',(-50.,4.88107836846757,-7.54316218647348));
#54551=CARTESIAN_POINT('Ctrl Pts',(-21.,4.88107836846757,-7.54316218647348));
#54552=CARTESIAN_POINT('Ctrl Pts',(-50.,4.79269894740031,-7.48374039375355));
#54553=CARTESIAN_POINT('Ctrl Pts',(-21.,4.79269894740031,-7.48374039375355));
#54554=CARTESIAN_POINT('Ctrl Pts',(-50.,4.70721371156899,-7.42177134000892));
#54555=CARTESIAN_POINT('Ctrl Pts',(-21.,4.70721371156899,-7.42177134000892));
#54556=CARTESIAN_POINT('Ctrl Pts',(-50.,4.62503998887083,-7.35700721943171));
#54557=CARTESIAN_POINT('Ctrl Pts',(-21.,4.62503998887083,-7.35700721943171));
#54558=CARTESIAN_POINT('Ctrl Pts',(-50.,4.54657777868016,-7.28923990788708));
#54559=CARTESIAN_POINT('Ctrl Pts',(-21.,4.54657777868016,-7.28923990788708));
#54560=CARTESIAN_POINT('Ctrl Pts',(-50.,4.47217290162416,-7.21834255288981));
#54561=CARTESIAN_POINT('Ctrl Pts',(-21.,4.47217290162416,-7.21834255288981));
#54562=CARTESIAN_POINT('Ctrl Pts',(-50.,4.40207217433237,-7.14429034032177));
#54563=CARTESIAN_POINT('Ctrl Pts',(-21.,4.40207217433237,-7.14429034032177));
#54564=CARTESIAN_POINT('Ctrl Pts',(-50.,4.33637651734857,-7.06716577496009));
#54565=CARTESIAN_POINT('Ctrl Pts',(-21.,4.33637651734857,-7.06716577496009));
#54566=CARTESIAN_POINT('Ctrl Pts',(-50.,4.27498923356982,-6.98717136730191));
#54567=CARTESIAN_POINT('Ctrl Pts',(-21.,4.27498923356982,-6.98717136730191));
#54568=CARTESIAN_POINT('Ctrl Pts',(-50.,4.21757413484032,-6.90463617300865));
#54569=CARTESIAN_POINT('Ctrl Pts',(-21.,4.21757413484032,-6.90463617300865));
#54570=CARTESIAN_POINT('Ctrl Pts',(-50.,4.16348379256721,-6.82003644526658));
#54571=CARTESIAN_POINT('Ctrl Pts',(-21.,4.16348379256721,-6.82003644526658));
#54572=CARTESIAN_POINT('Ctrl Pts',(-50.,4.11183783259628,-6.73395053478792));
#54573=CARTESIAN_POINT('Ctrl Pts',(-21.,4.11183783259628,-6.73395053478792));
#54574=CARTESIAN_POINT('Ctrl Pts',(-50.,4.06165666819706,-6.64698999124062));
#54575=CARTESIAN_POINT('Ctrl Pts',(-21.,4.06165666819706,-6.64698999124062));
#54576=CARTESIAN_POINT('Ctrl Pts',(-50.,4.01197889710939,-6.55973735411151));
#54577=CARTESIAN_POINT('Ctrl Pts',(-21.,4.01197889710939,-6.55973735411151));
#54578=CARTESIAN_POINT('Ctrl Pts',(-50.,3.96197913233089,-6.47268455970493));
#54579=CARTESIAN_POINT('Ctrl Pts',(-21.,3.96197913233089,-6.47268455970493));
#54580=CARTESIAN_POINT('Ctrl Pts',(-50.,3.91110213900011,-6.38616193008433));
#54581=CARTESIAN_POINT('Ctrl Pts',(-21.,3.91110213900011,-6.38616193008433));
#54582=CARTESIAN_POINT('Ctrl Pts',(-50.,3.859023878729,-6.30036238594766));
#54583=CARTESIAN_POINT('Ctrl Pts',(-21.,3.859023878729,-6.30036238594766));
#54584=CARTESIAN_POINT('Ctrl Pts',(-50.,3.81627329006595,-6.23237673886416));
#54585=CARTESIAN_POINT('Ctrl Pts',(-21.,3.81627329006595,-6.23237673886416));
#54586=CARTESIAN_POINT('Ctrl Pts',(-50.,3.78357651403939,-6.1817683663582));
#54587=CARTESIAN_POINT('Ctrl Pts',(-21.,3.78357651403939,-6.1817683663582));
#54588=CARTESIAN_POINT('Ctrl Pts',(-50.,3.7614973065729,-6.1481985134482));
#54589=CARTESIAN_POINT('Ctrl Pts',(-21.,3.7614973065729,-6.1481985134482));
#54590=CARTESIAN_POINT('Ctrl Pts',(-50.,3.75038736519793,-6.13145585166881));
#54591=CARTESIAN_POINT('Ctrl Pts',(-21.,3.75038736519793,-6.13145585166881));
#54592=CARTESIAN_POINT('',(-50.,3.75038736519794,-6.13145585166881));
#54593=CARTESIAN_POINT('Origin',(-50.,0.,0.));
#54594=CARTESIAN_POINT('',(-50.,2.45543694297674,-6.75507110762463));
#54595=CARTESIAN_POINT('Ctrl Pts',(-50.,2.45543694297674,-6.75507110762463));
#54596=CARTESIAN_POINT('Ctrl Pts',(-21.,2.45543694297674,-6.75507110762463));
#54597=CARTESIAN_POINT('Ctrl Pts',(-50.,2.46297417772978,-6.77764561818537));
#54598=CARTESIAN_POINT('Ctrl Pts',(-21.,2.46297417772978,-6.77764561818537));
#54599=CARTESIAN_POINT('Ctrl Pts',(-50.,2.47820711493347,-6.82274841734025));
#54600=CARTESIAN_POINT('Ctrl Pts',(-21.,2.47820711493347,-6.82274841734025));
#54601=CARTESIAN_POINT('Ctrl Pts',(-50.,2.50153193679118,-6.89026394714059));
#54602=CARTESIAN_POINT('Ctrl Pts',(-21.,2.50153193679118,-6.89026394714059));
#54603=CARTESIAN_POINT('Ctrl Pts',(-50.,2.53358368474749,-6.98000697278327));
#54604=CARTESIAN_POINT('Ctrl Pts',(-21.,2.53358368474749,-6.98000697278327));
#54605=CARTESIAN_POINT('Ctrl Pts',(-50.,2.57514309471485,-7.09174914908801));
#54606=CARTESIAN_POINT('Ctrl Pts',(-21.,2.57514309471485,-7.09174914908801));
#54607=CARTESIAN_POINT('Ctrl Pts',(-50.,2.61790620462629,-7.20313763732345));
#54608=CARTESIAN_POINT('Ctrl Pts',(-21.,2.61790620462629,-7.20313763732345));
#54609=CARTESIAN_POINT('Ctrl Pts',(-50.,2.66128382072048,-7.31434056822034));
#54610=CARTESIAN_POINT('Ctrl Pts',(-21.,2.66128382072048,-7.31434056822034));
#54611=CARTESIAN_POINT('Ctrl Pts',(-50.,2.70427297026251,-7.42564364342468));
#54612=CARTESIAN_POINT('Ctrl Pts',(-21.,2.70427297026251,-7.42564364342468));
#54613=CARTESIAN_POINT('Ctrl Pts',(-50.,2.74553095355499,-7.53744508591865));
#54614=CARTESIAN_POINT('Ctrl Pts',(-21.,2.74553095355499,-7.53744508591865));
#54615=CARTESIAN_POINT('Ctrl Pts',(-50.,2.78345892001629,-7.65025207826714));
#54616=CARTESIAN_POINT('Ctrl Pts',(-21.,2.78345892001629,-7.65025207826714));
#54617=CARTESIAN_POINT('Ctrl Pts',(-50.,2.81629364412744,-7.76466852264525));
#54618=CARTESIAN_POINT('Ctrl Pts',(-21.,2.81629364412744,-7.76466852264525));
#54619=CARTESIAN_POINT('Ctrl Pts',(-50.,2.84216119689693,-7.88140953422486));
#54620=CARTESIAN_POINT('Ctrl Pts',(-21.,2.84216119689693,-7.88140953422486));
#54621=CARTESIAN_POINT('Ctrl Pts',(-50.,2.85947913898695,-8.00108902987832));
#54622=CARTESIAN_POINT('Ctrl Pts',(-21.,2.85947913898695,-8.00108902987832));
#54623=CARTESIAN_POINT('Ctrl Pts',(-50.,2.86748815125169,-8.12392974416385));
#54624=CARTESIAN_POINT('Ctrl Pts',(-21.,2.86748815125169,-8.12392974416385));
#54625=CARTESIAN_POINT('Ctrl Pts',(-50.,2.8666442371861,-8.24955186700095));
#54626=CARTESIAN_POINT('Ctrl Pts',(-21.,2.8666442371861,-8.24955186700095));
#54627=CARTESIAN_POINT('Ctrl Pts',(-50.,2.85932311928695,-8.37659160589212));
#54628=CARTESIAN_POINT('Ctrl Pts',(-21.,2.85932311928695,-8.37659160589212));
#54629=CARTESIAN_POINT('Ctrl Pts',(-50.,2.84893087833482,-8.50318672326558));
#54630=CARTESIAN_POINT('Ctrl Pts',(-21.,2.84893087833482,-8.50318672326558));
#54631=CARTESIAN_POINT('Ctrl Pts',(-50.,2.838231660712,-8.62789111098118));
#54632=CARTESIAN_POINT('Ctrl Pts',(-21.,2.838231660712,-8.62789111098118));
#54633=CARTESIAN_POINT('Ctrl Pts',(-50.,2.8281804649272,-8.7503085875302));
#54634=CARTESIAN_POINT('Ctrl Pts',(-21.,2.8281804649272,-8.7503085875302));
#54635=CARTESIAN_POINT('Ctrl Pts',(-50.,2.81593951016314,-8.87218721998315));
#54636=CARTESIAN_POINT('Ctrl Pts',(-21.,2.81593951016314,-8.87218721998315));
#54637=CARTESIAN_POINT('Ctrl Pts',(-50.,2.79564609540172,-8.99695638729624));
#54638=CARTESIAN_POINT('Ctrl Pts',(-21.,2.79564609540172,-8.99695638729624));
#54639=CARTESIAN_POINT('Ctrl Pts',(-50.,2.76185693608665,-9.12774569066013));
#54640=CARTESIAN_POINT('Ctrl Pts',(-21.,2.76185693608665,-9.12774569066013));
#54641=CARTESIAN_POINT('Ctrl Pts',(-50.,2.71205611361093,-9.26593773005304));
#54642=CARTESIAN_POINT('Ctrl Pts',(-21.,2.71205611361093,-9.26593773005304));
#54643=CARTESIAN_POINT('Ctrl Pts',(-50.,2.65001133311308,-9.40923210196585));
#54644=CARTESIAN_POINT('Ctrl Pts',(-21.,2.65001133311308,-9.40923210196585));
#54645=CARTESIAN_POINT('Ctrl Pts',(-50.,2.5873945538455,-9.5507160797281));
#54646=CARTESIAN_POINT('Ctrl Pts',(-21.,2.5873945538455,-9.5507160797281));
#54647=CARTESIAN_POINT('Ctrl Pts',(-50.,2.54042342638657,-9.68082891874335));
#54648=CARTESIAN_POINT('Ctrl Pts',(-21.,2.54042342638657,-9.68082891874335));
#54649=CARTESIAN_POINT('Ctrl Pts',(-50.,2.52733779392361,-9.78884102493588));
#54650=CARTESIAN_POINT('Ctrl Pts',(-21.,2.52733779392361,-9.78884102493588));
#54651=CARTESIAN_POINT('Ctrl Pts',(-50.,2.56562806487107,-9.86447715727042));
#54652=CARTESIAN_POINT('Ctrl Pts',(-21.,2.56562806487107,-9.86447715727042));
#54653=CARTESIAN_POINT('Ctrl Pts',(-50.,2.6691907234428,-9.89958344728561));
#54654=CARTESIAN_POINT('Ctrl Pts',(-21.,2.6691907234428,-9.89958344728561));
#54655=CARTESIAN_POINT('Ctrl Pts',(-50.,2.84860197903673,-9.88796382014256));
#54656=CARTESIAN_POINT('Ctrl Pts',(-21.,2.84860197903673,-9.88796382014256));
#54657=CARTESIAN_POINT('Ctrl Pts',(-50.,3.11165374758123,-9.82506278266417));
#54658=CARTESIAN_POINT('Ctrl Pts',(-21.,3.11165374758123,-9.82506278266417));
#54659=CARTESIAN_POINT('Ctrl Pts',(-50.,3.46376909107161,-9.70771911811945));
#54660=CARTESIAN_POINT('Ctrl Pts',(-21.,3.46376909107161,-9.70771911811945));
#54661=CARTESIAN_POINT('Ctrl Pts',(-50.,3.90844493048625,-9.5339037941241));
#54662=CARTESIAN_POINT('Ctrl Pts',(-21.,3.90844493048625,-9.5339037941241));
#54663=CARTESIAN_POINT('Ctrl Pts',(-50.,4.44766091491103,-9.30247791214345));
#54664=CARTESIAN_POINT('Ctrl Pts',(-21.,4.44766091491103,-9.30247791214345));
#54665=CARTESIAN_POINT('Ctrl Pts',(-50.,5.08228263794097,-9.01295415598311));
#54666=CARTESIAN_POINT('Ctrl Pts',(-21.,5.08228263794097,-9.01295415598311));
#54667=CARTESIAN_POINT('Ctrl Pts',(-50.,5.66641576644903,-8.73480497776003));
#54668=CARTESIAN_POINT('Ctrl Pts',(-21.,5.66641576644903,-8.73480497776003));
#54669=CARTESIAN_POINT('Ctrl Pts',(-50.,6.14741641494695,-8.50008023141016));
#54670=CARTESIAN_POINT('Ctrl Pts',(-21.,6.14741641494695,-8.50008023141016));
#54671=CARTESIAN_POINT('Ctrl Pts',(-50.,6.48712519233677,-8.33200677716551));
#54672=CARTESIAN_POINT('Ctrl Pts',(-21.,6.48712519233677,-8.33200677716551));
#54673=CARTESIAN_POINT('Ctrl Pts',(-50.,6.6617400018565,-8.24507247679879));
#54674=CARTESIAN_POINT('Ctrl Pts',(-21.,6.6617400018565,-8.24507247679879));
#54675=CARTESIAN_POINT('',(-21.5,2.55037217513312,-9.66931237308562));
#54676=CARTESIAN_POINT('Ctrl Pts',(-21.5,2.55037217513312,-9.66931237308562));
#54677=CARTESIAN_POINT('Ctrl Pts',(-21.4716714037525,2.55832628412868,-9.63791697607888));
#54678=CARTESIAN_POINT('Ctrl Pts',(-21.4424150110734,2.56959157653322,-9.60464841257241));
#54679=CARTESIAN_POINT('Ctrl Pts',(-21.2909879716435,2.63587850947584,-9.42991855559448));
#54680=CARTESIAN_POINT('Ctrl Pts',(-21.1630186724934,2.71837825362615,-9.27335939831189));
#54681=CARTESIAN_POINT('Ctrl Pts',(-21.,2.77045032493322,-9.08705700417233));
#54682=CARTESIAN_POINT('Ctrl Pts',(-50.,2.55037217513312,-9.66931237308562));
#54683=CARTESIAN_POINT('Ctrl Pts',(-45.1666666666667,2.55037217513312,-9.66931237308562));
#54684=CARTESIAN_POINT('Ctrl Pts',(-40.3333333333333,2.55037217513312,-9.66931237308562));
#54685=CARTESIAN_POINT('Ctrl Pts',(-30.8333333333333,2.55037217513312,-9.66931237308562));
#54686=CARTESIAN_POINT('Ctrl Pts',(-26.1666666666667,2.55037217513312,-9.66931237308562));
#54687=CARTESIAN_POINT('Ctrl Pts',(-21.5,2.55037217513312,-9.66931237308562));
#54688=CARTESIAN_POINT('Origin',(-21.25,0.,0.));
#54689=CARTESIAN_POINT('Origin',(-21.5,0.,0.));
#54690=CARTESIAN_POINT('Origin',(-35.75,0.,0.));
#54691=CARTESIAN_POINT('Ctrl Pts',(-50.,-0.718643267461624,-7.15148293042304));
#54692=CARTESIAN_POINT('Ctrl Pts',(-21.,-0.718643267461624,-7.15148293042304));
#54693=CARTESIAN_POINT('Ctrl Pts',(-50.,-0.721647166649912,-7.17509214524366));
#54694=CARTESIAN_POINT('Ctrl Pts',(-21.,-0.721647166649912,-7.17509214524366));
#54695=CARTESIAN_POINT('Ctrl Pts',(-50.,-0.72749213560466,-7.22233768688913));
#54696=CARTESIAN_POINT('Ctrl Pts',(-21.,-0.72749213560466,-7.22233768688913));
#54697=CARTESIAN_POINT('Ctrl Pts',(-50.,-0.735771087779772,-7.29328733826105));
#54698=CARTESIAN_POINT('Ctrl Pts',(-21.,-0.735771087779772,-7.29328733826105));
#54699=CARTESIAN_POINT('Ctrl Pts',(-50.,-0.745831500234844,-7.38804974272502));
#54700=CARTESIAN_POINT('Ctrl Pts',(-21.,-0.745831500234844,-7.38804974272502));
#54701=CARTESIAN_POINT('Ctrl Pts',(-50.,-0.756870878958097,-7.5067579169994));
#54702=CARTESIAN_POINT('Ctrl Pts',(-21.,-0.756870878958097,-7.5067579169994));
#54703=CARTESIAN_POINT('Ctrl Pts',(-50.,-0.766672302003446,-7.62566969516693));
#54704=CARTESIAN_POINT('Ctrl Pts',(-21.,-0.766672302003446,-7.62566969516693));
#54705=CARTESIAN_POINT('Ctrl Pts',(-50.,-0.775839563797133,-7.74468091618948));
#54706=CARTESIAN_POINT('Ctrl Pts',(-21.,-0.775839563797133,-7.74468091618948));
#54707=CARTESIAN_POINT('Ctrl Pts',(-50.,-0.785400272847099,-7.86361381479518));
#54708=CARTESIAN_POINT('Ctrl Pts',(-21.,-0.785400272847099,-7.86361381479518));
#54709=CARTESIAN_POINT('Ctrl Pts',(-50.,-0.796736942256156,-7.98224460192821));
#54710=CARTESIAN_POINT('Ctrl Pts',(-21.,-0.796736942256156,-7.98224460192821));
#54711=CARTESIAN_POINT('Ctrl Pts',(-50.,-0.811510144890449,-8.10033651802127));
#54712=CARTESIAN_POINT('Ctrl Pts',(-21.,-0.811510144890449,-8.10033651802127));
#54713=CARTESIAN_POINT('Ctrl Pts',(-50.,-0.831570515383447,-8.21766862525226));
#54714=CARTESIAN_POINT('Ctrl Pts',(-21.,-0.831570515383447,-8.21766862525226));
#54715=CARTESIAN_POINT('Ctrl Pts',(-50.,-0.858916682261846,-8.33407215281038));
#54716=CARTESIAN_POINT('Ctrl Pts',(-21.,-0.858916682261846,-8.33407215281038));
#54717=CARTESIAN_POINT('Ctrl Pts',(-50.,-0.895240742652424,-8.44941362598824));
#54718=CARTESIAN_POINT('Ctrl Pts',(-21.,-0.895240742652424,-8.44941362598824));
#54719=CARTESIAN_POINT('Ctrl Pts',(-50.,-0.941323460369318,-8.56356426545847));
#54720=CARTESIAN_POINT('Ctrl Pts',(-21.,-0.941323460369318,-8.56356426545847));
#54721=CARTESIAN_POINT('Ctrl Pts',(-50.,-0.996589197042053,-8.67637972666424));
#54722=CARTESIAN_POINT('Ctrl Pts',(-21.,-0.996589197042053,-8.67637972666424));
#54723=CARTESIAN_POINT('Ctrl Pts',(-50.,-1.05830577327405,-8.78766206238304));
#54724=CARTESIAN_POINT('Ctrl Pts',(-21.,-1.05830577327405,-8.78766206238304));
#54725=CARTESIAN_POINT('Ctrl Pts',(-50.,-1.12259642171968,-8.89721129760285));
#54726=CARTESIAN_POINT('Ctrl Pts',(-21.,-1.12259642171968,-8.89721129760285));
#54727=CARTESIAN_POINT('Ctrl Pts',(-50.,-1.18634328973517,-9.00492385207762));
#54728=CARTESIAN_POINT('Ctrl Pts',(-21.,-1.18634328973517,-9.00492385207762));
#54729=CARTESIAN_POINT('Ctrl Pts',(-50.,-1.24851405668088,-9.11085713692575));
#54730=CARTESIAN_POINT('Ctrl Pts',(-21.,-1.24851405668088,-9.11085713692575));
#54731=CARTESIAN_POINT('Ctrl Pts',(-50.,-1.31242393260393,-9.21535483920498));
#54732=CARTESIAN_POINT('Ctrl Pts',(-21.,-1.31242393260393,-9.21535483920498));
#54733=CARTESIAN_POINT('Ctrl Pts',(-50.,-1.38484298036779,-9.31896299195203));
#54734=CARTESIAN_POINT('Ctrl Pts',(-21.,-1.38484298036779,-9.31896299195203));
#54735=CARTESIAN_POINT('Ctrl Pts',(-50.,-1.47203331296336,-9.42213951575228));
#54736=CARTESIAN_POINT('Ctrl Pts',(-21.,-1.47203331296336,-9.42213951575228));
#54737=CARTESIAN_POINT('Ctrl Pts',(-50.,-1.576861582378,-9.52503847397034));
#54738=CARTESIAN_POINT('Ctrl Pts',(-21.,-1.576861582378,-9.52503847397034));
#54739=CARTESIAN_POINT('Ctrl Pts',(-50.,-1.69493509590243,-9.62722202065428));
#54740=CARTESIAN_POINT('Ctrl Pts',(-21.,-1.69493509590243,-9.62722202065428));
#54741=CARTESIAN_POINT('Ctrl Pts',(-50.,-1.81273846192755,-9.72752627760495));
#54742=CARTESIAN_POINT('Ctrl Pts',(-21.,-1.81273846192755,-9.72752627760495));
#54743=CARTESIAN_POINT('Ctrl Pts',(-50.,-1.91151183055746,-9.82437388645964));
#54744=CARTESIAN_POINT('Ctrl Pts',(-21.,-1.91151183055746,-9.82437388645964));
#54745=CARTESIAN_POINT('Ctrl Pts',(-50.,-1.97016627452818,-9.91601178835393));
#54746=CARTESIAN_POINT('Ctrl Pts',(-21.,-1.97016627452818,-9.91601178835393));
#54747=CARTESIAN_POINT('Ctrl Pts',(-50.,-1.96848522037067,-10.0007711148064));
#54748=CARTESIAN_POINT('Ctrl Pts',(-21.,-1.96848522037067,-10.0007711148064));
#54749=CARTESIAN_POINT('Ctrl Pts',(-50.,-1.89041053749867,-10.0773349427117));
#54750=CARTESIAN_POINT('Ctrl Pts',(-21.,-1.89041053749867,-10.0773349427117));
#54751=CARTESIAN_POINT('Ctrl Pts',(-50.,-1.72372501438528,-10.1447096468161));
#54752=CARTESIAN_POINT('Ctrl Pts',(-21.,-1.72372501438528,-10.1447096468161));
#54753=CARTESIAN_POINT('Ctrl Pts',(-50.,-1.45943182294451,-10.2021716552068));
#54754=CARTESIAN_POINT('Ctrl Pts',(-21.,-1.45943182294451,-10.2021716552068));
#54755=CARTESIAN_POINT('Ctrl Pts',(-50.,-1.09127335261449,-10.2492257884407));
#54756=CARTESIAN_POINT('Ctrl Pts',(-21.,-1.09127335261449,-10.2492257884407));
#54757=CARTESIAN_POINT('Ctrl Pts',(-50.,-0.615218622302492,-10.285561208657));
#54758=CARTESIAN_POINT('Ctrl Pts',(-21.,-0.615218622302492,-10.285561208657));
#54759=CARTESIAN_POINT('Ctrl Pts',(-50.,-0.0289898802580651,-10.3110107412798));
#54760=CARTESIAN_POINT('Ctrl Pts',(-21.,-0.0289898802580651,-10.3110107412798));
#54761=CARTESIAN_POINT('Ctrl Pts',(-50.,0.66840418497271,-10.3255108965746));
#54762=CARTESIAN_POINT('Ctrl Pts',(-21.,0.66840418497271,-10.3255108965746));
#54763=CARTESIAN_POINT('Ctrl Pts',(-50.,1.31537435394882,-10.3283530123025));
#54764=CARTESIAN_POINT('Ctrl Pts',(-21.,1.31537435394882,-10.3283530123025));
#54765=CARTESIAN_POINT('Ctrl Pts',(-50.,1.85058421429602,-10.3255716832032));
#54766=CARTESIAN_POINT('Ctrl Pts',(-21.,1.85058421429602,-10.3255716832032));
#54767=CARTESIAN_POINT('Ctrl Pts',(-50.,2.22957558565152,-10.3215368479529));
#54768=CARTESIAN_POINT('Ctrl Pts',(-21.,2.22957558565152,-10.3215368479529));
#54769=CARTESIAN_POINT('Ctrl Pts',(-50.,2.42461747220419,-10.3189742762293));
#54770=CARTESIAN_POINT('Ctrl Pts',(-21.,2.42461747220419,-10.3189742762293));
#54771=CARTESIAN_POINT('',(-21.5,-1.89755147577054,-9.81831443766195));
#54772=CARTESIAN_POINT('Ctrl Pts',(-50.,-1.89755147577054,-9.81831443766195));
#54773=CARTESIAN_POINT('Ctrl Pts',(-45.1666666666667,-1.89755147577054,
-9.81831443766195));
#54774=CARTESIAN_POINT('Ctrl Pts',(-40.3333333333333,-1.89755147577054,
-9.81831443766195));
#54775=CARTESIAN_POINT('Ctrl Pts',(-30.8333333333333,-1.89755147577054,
-9.81831443766195));
#54776=CARTESIAN_POINT('Ctrl Pts',(-26.1666666666667,-1.89755147577054,
-9.81831443766195));
#54777=CARTESIAN_POINT('Ctrl Pts',(-21.5,-1.89755147577054,-9.81831443766195));
#54778=CARTESIAN_POINT('',(-50.,-0.718643267461624,-7.15148293042304));
#54779=CARTESIAN_POINT('Ctrl Pts',(-21.5,-1.89755147577054,-9.81831443766195));
#54780=CARTESIAN_POINT('Ctrl Pts',(-21.4703246838902,-1.87577485631915,
-9.79229867840487));
#54781=CARTESIAN_POINT('Ctrl Pts',(-21.4396140182583,-1.84982079175854,
-9.7659920048413));
#54782=CARTESIAN_POINT('Ctrl Pts',(-21.2876118590989,-1.71298536185018,
-9.63694998390254));
#54783=CARTESIAN_POINT('Ctrl Pts',(-21.1610241576493,-1.57282267908268,
-9.53269100720236));
#54784=CARTESIAN_POINT('Ctrl Pts',(-21.,-1.44663677770971,-9.38920880763537));
#54785=CARTESIAN_POINT('Origin',(-50.,0.,0.));
#54786=CARTESIAN_POINT('',(-50.,0.718643267461627,-7.15148293042304));
#54787=CARTESIAN_POINT('Ctrl Pts',(-50.,2.42461747220419,-10.3189742762293));
#54788=CARTESIAN_POINT('Ctrl Pts',(-21.,2.42461747220419,-10.3189742762293));
#54789=CARTESIAN_POINT('Ctrl Pts',(-50.,2.40572662366171,-10.3043608046855));
#54790=CARTESIAN_POINT('Ctrl Pts',(-21.,2.40572662366171,-10.3043608046855));
#54791=CARTESIAN_POINT('Ctrl Pts',(-50.,2.36813316049665,-10.2750183870592));
#54792=CARTESIAN_POINT('Ctrl Pts',(-21.,2.36813316049665,-10.2750183870592));
#54793=CARTESIAN_POINT('Ctrl Pts',(-50.,2.31230766835601,-10.2306583371767));
#54794=CARTESIAN_POINT('Ctrl Pts',(-21.,2.31230766835601,-10.2306583371767));
#54795=CARTESIAN_POINT('Ctrl Pts',(-50.,2.2390045785598,-10.1708178342288));
#54796=CARTESIAN_POINT('Ctrl Pts',(-21.,2.2390045785598,-10.1708178342288));
#54797=CARTESIAN_POINT('Ctrl Pts',(-50.,2.14927498796815,-10.0948558607226));
#54798=CARTESIAN_POINT('Ctrl Pts',(-21.,2.14927498796815,-10.0948558607226));
#54799=CARTESIAN_POINT('Ctrl Pts',(-50.,2.06147268851079,-10.0177266439074));
#54800=CARTESIAN_POINT('Ctrl Pts',(-21.,2.06147268851079,-10.0177266439074));
#54801=CARTESIAN_POINT('Ctrl Pts',(-50.,1.97564250382672,-9.93942550853734));
#54802=CARTESIAN_POINT('Ctrl Pts',(-21.,1.97564250382672,-9.93942550853734));
#54803=CARTESIAN_POINT('Ctrl Pts',(-50.,1.89184818563464,-9.85995105817688));
#54804=CARTESIAN_POINT('Ctrl Pts',(-21.,1.89184818563464,-9.85995105817688));
#54805=CARTESIAN_POINT('Ctrl Pts',(-50.,1.81017697820953,-9.77930761193764));
#54806=CARTESIAN_POINT('Ctrl Pts',(-21.,1.81017697820953,-9.77930761193764));
#54807=CARTESIAN_POINT('Ctrl Pts',(-50.,1.73072865645713,-9.69750595756857));
#54808=CARTESIAN_POINT('Ctrl Pts',(-21.,1.73072865645713,-9.69750595756857));
#54809=CARTESIAN_POINT('Ctrl Pts',(-50.,1.65360100339141,-9.61456358834088));
#54810=CARTESIAN_POINT('Ctrl Pts',(-21.,1.65360100339141,-9.61456358834088));
#54811=CARTESIAN_POINT('Ctrl Pts',(-50.,1.57887480066182,-9.53050553264656));
#54812=CARTESIAN_POINT('Ctrl Pts',(-21.,1.57887480066182,-9.53050553264656));
#54813=CARTESIAN_POINT('Ctrl Pts',(-50.,1.50660194229105,-9.44536454178638));
#54814=CARTESIAN_POINT('Ctrl Pts',(-21.,1.50660194229105,-9.44536454178638));
#54815=CARTESIAN_POINT('Ctrl Pts',(-50.,1.43678361338666,-9.35918315674388));
#54816=CARTESIAN_POINT('Ctrl Pts',(-21.,1.43678361338666,-9.35918315674388));
#54817=CARTESIAN_POINT('Ctrl Pts',(-50.,1.3693914299125,-9.27200835121914));
#54818=CARTESIAN_POINT('Ctrl Pts',(-21.,1.3693914299125,-9.27200835121914));
#54819=CARTESIAN_POINT('Ctrl Pts',(-50.,1.30441156144786,-9.18388242219763));
#54820=CARTESIAN_POINT('Ctrl Pts',(-21.,1.30441156144786,-9.18388242219763));
#54821=CARTESIAN_POINT('Ctrl Pts',(-50.,1.24188395306769,-9.09483443436949));
#54822=CARTESIAN_POINT('Ctrl Pts',(-21.,1.24188395306769,-9.09483443436949));
#54823=CARTESIAN_POINT('Ctrl Pts',(-50.,1.18193820283021,-9.00487302535333));
#54824=CARTESIAN_POINT('Ctrl Pts',(-21.,1.18193820283021,-9.00487302535333));
#54825=CARTESIAN_POINT('Ctrl Pts',(-50.,1.12484423754393,-8.91397482898789));
#54826=CARTESIAN_POINT('Ctrl Pts',(-21.,1.12484423754393,-8.91397482898789));
#54827=CARTESIAN_POINT('Ctrl Pts',(-50.,1.07099928020948,-8.82209124999857));
#54828=CARTESIAN_POINT('Ctrl Pts',(-21.,1.07099928020948,-8.82209124999857));
#54829=CARTESIAN_POINT('Ctrl Pts',(-50.,1.02086710880845,-8.72916840803945));
#54830=CARTESIAN_POINT('Ctrl Pts',(-21.,1.02086710880845,-8.72916840803945));
#54831=CARTESIAN_POINT('Ctrl Pts',(-50.,0.974931241694465,-8.63516410958082));
#54832=CARTESIAN_POINT('Ctrl Pts',(-21.,0.974931241694465,-8.63516410958082));
#54833=CARTESIAN_POINT('Ctrl Pts',(-50.,0.933642367528787,-8.5400643944807));
#54834=CARTESIAN_POINT('Ctrl Pts',(-21.,0.933642367528787,-8.5400643944807));
#54835=CARTESIAN_POINT('Ctrl Pts',(-50.,0.897367099160984,-8.4439050185459));
#54836=CARTESIAN_POINT('Ctrl Pts',(-21.,0.897367099160984,-8.4439050185459));
#54837=CARTESIAN_POINT('Ctrl Pts',(-50.,0.866338577132719,-8.34677071475058));
#54838=CARTESIAN_POINT('Ctrl Pts',(-21.,0.866338577132719,-8.34677071475058));
#54839=CARTESIAN_POINT('Ctrl Pts',(-50.,0.840611930230857,-8.24877960511329));
#54840=CARTESIAN_POINT('Ctrl Pts',(-21.,0.840611930230857,-8.24877960511329));
#54841=CARTESIAN_POINT('Ctrl Pts',(-50.,0.820012171364339,-8.15007218998677));
#54842=CARTESIAN_POINT('Ctrl Pts',(-21.,0.820012171364339,-8.15007218998677));
#54843=CARTESIAN_POINT('Ctrl Pts',(-50.,0.804093633570272,-8.05079907170372));
#54844=CARTESIAN_POINT('Ctrl Pts',(-21.,0.804093633570272,-8.05079907170372));
#54845=CARTESIAN_POINT('Ctrl Pts',(-50.,0.792066365329068,-7.95110843081948));
#54846=CARTESIAN_POINT('Ctrl Pts',(-21.,0.792066365329068,-7.95110843081948));
#54847=CARTESIAN_POINT('Ctrl Pts',(-50.,0.782886239966143,-7.85113936329068));
#54848=CARTESIAN_POINT('Ctrl Pts',(-21.,0.782886239966143,-7.85113936329068));
#54849=CARTESIAN_POINT('Ctrl Pts',(-50.,0.775405338877349,-7.75101782957587));
#54850=CARTESIAN_POINT('Ctrl Pts',(-21.,0.775405338877349,-7.75101782957587));
#54851=CARTESIAN_POINT('Ctrl Pts',(-50.,0.768504714146026,-7.65085154280962));
#54852=CARTESIAN_POINT('Ctrl Pts',(-21.,0.768504714146026,-7.65085154280962));
#54853=CARTESIAN_POINT('Ctrl Pts',(-50.,0.761227274615911,-7.55072560028829));
#54854=CARTESIAN_POINT('Ctrl Pts',(-21.,0.761227274615911,-7.55072560028829));
#54855=CARTESIAN_POINT('Ctrl Pts',(-50.,0.752929449590465,-7.45069670452966));
#54856=CARTESIAN_POINT('Ctrl Pts',(-21.,0.752929449590465,-7.45069670452966));
#54857=CARTESIAN_POINT('Ctrl Pts',(-50.,0.743235585416283,-7.35079807608913));
#54858=CARTESIAN_POINT('Ctrl Pts',(-21.,0.743235585416283,-7.35079807608913));
#54859=CARTESIAN_POINT('Ctrl Pts',(-50.,0.734216502709278,-7.2709963393441));
#54860=CARTESIAN_POINT('Ctrl Pts',(-21.,0.734216502709278,-7.2709963393441));
#54861=CARTESIAN_POINT('Ctrl Pts',(-50.,0.72671587532212,-7.21121317182152));
#54862=CARTESIAN_POINT('Ctrl Pts',(-21.,0.72671587532212,-7.21121317182152));
#54863=CARTESIAN_POINT('Ctrl Pts',(-50.,0.721388610069064,-7.17138797035723));
#54864=CARTESIAN_POINT('Ctrl Pts',(-21.,0.721388610069064,-7.17138797035723));
#54865=CARTESIAN_POINT('Ctrl Pts',(-50.,0.718643267461621,-7.15148293042304));
#54866=CARTESIAN_POINT('Ctrl Pts',(-21.,0.718643267461621,-7.15148293042304));
#54867=CARTESIAN_POINT('',(-21.5,1.85780428234483,-9.82591284555797));
#54868=CARTESIAN_POINT('Ctrl Pts',(-21.5,1.85780428234483,-9.82591284555798));
#54869=CARTESIAN_POINT('Ctrl Pts',(-26.3333333333333,1.85780428234483,-9.82591284555798));
#54870=CARTESIAN_POINT('Ctrl Pts',(-31.1666666666667,1.85780428234483,-9.82591284555798));
#54871=CARTESIAN_POINT('Ctrl Pts',(-40.6666666666667,1.85780428234483,-9.82591284555798));
#54872=CARTESIAN_POINT('Ctrl Pts',(-45.3333333333333,1.85780428234483,-9.82591284555797));
#54873=CARTESIAN_POINT('Ctrl Pts',(-50.,1.85780428234483,-9.82591284555797));
#54874=CARTESIAN_POINT('Ctrl Pts',(-21.,1.45989994714919,-9.38715570044056));
#54875=CARTESIAN_POINT('Ctrl Pts',(-21.1708653764911,1.58343885080728,-9.54086217807748));
#54876=CARTESIAN_POINT('Ctrl Pts',(-21.337240031188,1.71664935045884,-9.68695766931646));
#54877=CARTESIAN_POINT('Ctrl Pts',(-21.5,1.85780428234483,-9.82591284555797));
#54878=CARTESIAN_POINT('Origin',(-35.75,0.,0.));
#54879=CARTESIAN_POINT('',(-21.5,-2.58947998462545,-9.65891264114259));
#54880=CARTESIAN_POINT('Origin',(-21.5,0.,0.));
#54881=CARTESIAN_POINT('Ctrl Pts',(-21.5,-2.58947998462545,-9.65891264114259));
#54882=CARTESIAN_POINT('Ctrl Pts',(-26.3333333333333,-2.58947998462545,
-9.65891264114259));
#54883=CARTESIAN_POINT('Ctrl Pts',(-31.1666666666667,-2.58947998462545,
-9.65891264114259));
#54884=CARTESIAN_POINT('Ctrl Pts',(-40.6666666666667,-2.58947998462545,
-9.65891264114259));
#54885=CARTESIAN_POINT('Ctrl Pts',(-45.3333333333333,-2.58947998462546,
-9.65891264114259));
#54886=CARTESIAN_POINT('Ctrl Pts',(-50.,-2.58947998462546,-9.65891264114259));
#54887=CARTESIAN_POINT('Origin',(-21.25,0.,0.));
#54888=CARTESIAN_POINT('Ctrl Pts',(-21.,-2.75760981235205,-9.09096189205628));
#54889=CARTESIAN_POINT('Ctrl Pts',(-21.0595504621632,-2.74206083288706,
-9.15790831820147));
#54890=CARTESIAN_POINT('Ctrl Pts',(-21.1201969196014,-2.72465875026456,
-9.22637318364334));
#54891=CARTESIAN_POINT('Ctrl Pts',(-21.1820623827142,-2.70512289983328,
-9.29649306846902));
#54892=CARTESIAN_POINT('Ctrl Pts',(-21.2426667634842,-2.68598527346419,
-9.36518361058578));
#54893=CARTESIAN_POINT('Ctrl Pts',(-21.304440959365,-2.66479906737499,-9.43546228599664));
#54894=CARTESIAN_POINT('Ctrl Pts',(-21.3675006106217,-2.64134946113942,
-9.50742323598161));
#54895=CARTESIAN_POINT('Ctrl Pts',(-21.4110415416836,-2.62515816181912,
-9.55711026564319));
#54896=CARTESIAN_POINT('Ctrl Pts',(-21.4551953158428,-2.60788916583244,
-9.60759844440427));
#54897=CARTESIAN_POINT('Ctrl Pts',(-21.5,-2.58947998461739,-9.65891264116508));
#54898=CARTESIAN_POINT('Ctrl Pts',(-50.,-2.29273028380004,-10.3490766663382));
#54899=CARTESIAN_POINT('Ctrl Pts',(-21.,-2.29273028380004,-10.3490766663382));
#54900=CARTESIAN_POINT('Ctrl Pts',(-50.,-2.30340980255016,-10.3277139514246));
#54901=CARTESIAN_POINT('Ctrl Pts',(-21.,-2.30340980255016,-10.3277139514246));
#54902=CARTESIAN_POINT('Ctrl Pts',(-50.,-2.32454914462407,-10.2849661542698));
#54903=CARTESIAN_POINT('Ctrl Pts',(-21.,-2.32454914462407,-10.2849661542698));
#54904=CARTESIAN_POINT('Ctrl Pts',(-50.,-2.35559907076766,-10.2207773570791));
#54905=CARTESIAN_POINT('Ctrl Pts',(-21.,-2.35559907076766,-10.2207773570791));
#54906=CARTESIAN_POINT('Ctrl Pts',(-50.,-2.39567905142538,-10.1350579081937));
#54907=CARTESIAN_POINT('Ctrl Pts',(-21.,-2.39567905142538,-10.1350579081937));
#54908=CARTESIAN_POINT('Ctrl Pts',(-50.,-2.44356395398247,-10.0276863246448));
#54909=CARTESIAN_POINT('Ctrl Pts',(-21.,-2.44356395398247,-10.0276863246448));
#54910=CARTESIAN_POINT('Ctrl Pts',(-50.,-2.48920597933682,-9.92009931149697));
#54911=CARTESIAN_POINT('Ctrl Pts',(-21.,-2.48920597933682,-9.92009931149697));
#54912=CARTESIAN_POINT('Ctrl Pts',(-50.,-2.53256271427195,-9.81231210474723));
#54913=CARTESIAN_POINT('Ctrl Pts',(-21.,-2.53256271427195,-9.81231210474723));
#54914=CARTESIAN_POINT('Ctrl Pts',(-50.,-2.57357611458342,-9.70435110708481));
#54915=CARTESIAN_POINT('Ctrl Pts',(-21.,-2.57357611458342,-9.70435110708481));
#54916=CARTESIAN_POINT('Ctrl Pts',(-50.,-2.61216944988784,-9.59625806376704));
#54917=CARTESIAN_POINT('Ctrl Pts',(-21.,-2.61216944988784,-9.59625806376704));
#54918=CARTESIAN_POINT('Ctrl Pts',(-50.,-2.6482575067302,-9.48808598492904));
#54919=CARTESIAN_POINT('Ctrl Pts',(-21.,-2.6482575067302,-9.48808598492904));
#54920=CARTESIAN_POINT('Ctrl Pts',(-50.,-2.68175977570501,-9.37989305792331));
#54921=CARTESIAN_POINT('Ctrl Pts',(-21.,-2.68175977570501,-9.37989305792331));
#54922=CARTESIAN_POINT('Ctrl Pts',(-50.,-2.71261433447333,-9.27173688239595));
#54923=CARTESIAN_POINT('Ctrl Pts',(-21.,-2.71261433447333,-9.27173688239595));
#54924=CARTESIAN_POINT('Ctrl Pts',(-50.,-2.74078863839312,-9.16366948222194));
#54925=CARTESIAN_POINT('Ctrl Pts',(-21.,-2.74078863839312,-9.16366948222194));
#54926=CARTESIAN_POINT('Ctrl Pts',(-50.,-2.76630007756038,-9.05572969970196));
#54927=CARTESIAN_POINT('Ctrl Pts',(-21.,-2.76630007756038,-9.05572969970196));
#54928=CARTESIAN_POINT('Ctrl Pts',(-50.,-2.78919460623265,-8.94794754130566));
#54929=CARTESIAN_POINT('Ctrl Pts',(-21.,-2.78919460623265,-8.94794754130566));
#54930=CARTESIAN_POINT('Ctrl Pts',(-50.,-2.80950303716262,-8.84035511450549));
#54931=CARTESIAN_POINT('Ctrl Pts',(-21.,-2.80950303716262,-8.84035511450549));
#54932=CARTESIAN_POINT('Ctrl Pts',(-50.,-2.82720199177778,-8.73299593720093));
#54933=CARTESIAN_POINT('Ctrl Pts',(-21.,-2.82720199177778,-8.73299593720093));
#54934=CARTESIAN_POINT('Ctrl Pts',(-50.,-2.84217845398458,-8.62593402210748));
#54935=CARTESIAN_POINT('Ctrl Pts',(-21.,-2.84217845398458,-8.62593402210748));
#54936=CARTESIAN_POINT('Ctrl Pts',(-50.,-2.85417908993455,-8.51926543389428));
#54937=CARTESIAN_POINT('Ctrl Pts',(-21.,-2.85417908993455,-8.51926543389428));
#54938=CARTESIAN_POINT('Ctrl Pts',(-50.,-2.86282492937103,-8.41311873833255));
#54939=CARTESIAN_POINT('Ctrl Pts',(-21.,-2.86282492937103,-8.41311873833255));
#54940=CARTESIAN_POINT('Ctrl Pts',(-50.,-2.86767474496505,-8.30764661663281));
#54941=CARTESIAN_POINT('Ctrl Pts',(-21.,-2.86767474496505,-8.30764661663281));
#54942=CARTESIAN_POINT('Ctrl Pts',(-50.,-2.8682745946465,-8.20302084448955));
#54943=CARTESIAN_POINT('Ctrl Pts',(-21.,-2.8682745946465,-8.20302084448955));
#54944=CARTESIAN_POINT('Ctrl Pts',(-50.,-2.86421236488387,-8.099424390731));
#54945=CARTESIAN_POINT('Ctrl Pts',(-21.,-2.86421236488387,-8.099424390731));
#54946=CARTESIAN_POINT('Ctrl Pts',(-50.,-2.85517326277626,-7.9970485375799));
#54947=CARTESIAN_POINT('Ctrl Pts',(-21.,-2.85517326277626,-7.9970485375799));
#54948=CARTESIAN_POINT('Ctrl Pts',(-50.,-2.84098400021346,-7.89607078269802));
#54949=CARTESIAN_POINT('Ctrl Pts',(-21.,-2.84098400021346,-7.89607078269802));
#54950=CARTESIAN_POINT('Ctrl Pts',(-50.,-2.82164615909785,-7.79662146983088));
#54951=CARTESIAN_POINT('Ctrl Pts',(-21.,-2.82164615909785,-7.79662146983088));
#54952=CARTESIAN_POINT('Ctrl Pts',(-50.,-2.79737835816915,-7.69875126136884));
#54953=CARTESIAN_POINT('Ctrl Pts',(-21.,-2.79737835816915,-7.69875126136884));
#54954=CARTESIAN_POINT('Ctrl Pts',(-50.,-2.76864747338962,-7.60240247767684));
#54955=CARTESIAN_POINT('Ctrl Pts',(-21.,-2.76864747338962,-7.60240247767684));
#54956=CARTESIAN_POINT('Ctrl Pts',(-50.,-2.73622951961898,-7.50736587770304));
#54957=CARTESIAN_POINT('Ctrl Pts',(-21.,-2.73622951961898,-7.50736587770304));
#54958=CARTESIAN_POINT('Ctrl Pts',(-50.,-2.70112557395893,-7.41331375298832));
#54959=CARTESIAN_POINT('Ctrl Pts',(-21.,-2.70112557395893,-7.41331375298832));
#54960=CARTESIAN_POINT('Ctrl Pts',(-50.,-2.66442452752942,-7.31986152676826));
#54961=CARTESIAN_POINT('Ctrl Pts',(-21.,-2.66442452752942,-7.31986152676826));
#54962=CARTESIAN_POINT('Ctrl Pts',(-50.,-2.62718125254576,-7.22662075191781));
#54963=CARTESIAN_POINT('Ctrl Pts',(-21.,-2.62718125254576,-7.22662075191781));
#54964=CARTESIAN_POINT('Ctrl Pts',(-50.,-2.59029498067661,-7.13325283216217));
#54965=CARTESIAN_POINT('Ctrl Pts',(-21.,-2.59029498067661,-7.13325283216217));
#54966=CARTESIAN_POINT('Ctrl Pts',(-50.,-2.55437015138428,-7.03952961984441));
#54967=CARTESIAN_POINT('Ctrl Pts',(-21.,-2.55437015138428,-7.03952961984441));
#54968=CARTESIAN_POINT('Ctrl Pts',(-50.,-2.5197596307744,-6.94531805563895));
#54969=CARTESIAN_POINT('Ctrl Pts',(-21.,-2.5197596307744,-6.94531805563895));
#54970=CARTESIAN_POINT('Ctrl Pts',(-50.,-2.49326086758344,-6.8695059418988));
#54971=CARTESIAN_POINT('Ctrl Pts',(-21.,-2.49326086758344,-6.8695059418988));
#54972=CARTESIAN_POINT('Ctrl Pts',(-50.,-2.47407975508802,-6.8123887688799));
#54973=CARTESIAN_POINT('Ctrl Pts',(-21.,-2.47407975508802,-6.8123887688799));
#54974=CARTESIAN_POINT('Ctrl Pts',(-50.,-2.46159994790965,-6.77419608843536));
#54975=CARTESIAN_POINT('Ctrl Pts',(-21.,-2.46159994790965,-6.77419608843536));
#54976=CARTESIAN_POINT('Ctrl Pts',(-50.,-2.45543694297675,-6.75507110762463));
#54977=CARTESIAN_POINT('Ctrl Pts',(-21.,-2.45543694297675,-6.75507110762463));
#54978=CARTESIAN_POINT('',(-50.,-2.45543694297674,-6.75507110762463));
#54979=CARTESIAN_POINT('Origin',(-50.,0.,0.));
#54980=CARTESIAN_POINT('',(-50.,-3.75038736519793,-6.13145585166881));
#54981=CARTESIAN_POINT('Ctrl Pts',(-50.,-3.75038736519793,-6.13145585166881));
#54982=CARTESIAN_POINT('Ctrl Pts',(-21.,-3.75038736519793,-6.13145585166881));
#54983=CARTESIAN_POINT('Ctrl Pts',(-50.,-3.7633374392529,-6.15142367620606));
#54984=CARTESIAN_POINT('Ctrl Pts',(-21.,-3.7633374392529,-6.15142367620606));
#54985=CARTESIAN_POINT('Ctrl Pts',(-50.,-3.78910264658076,-6.19145440139071));
#54986=CARTESIAN_POINT('Ctrl Pts',(-21.,-3.78910264658076,-6.19145440139071));
#54987=CARTESIAN_POINT('Ctrl Pts',(-50.,-3.82734562477572,-6.25178572573963));
#54988=CARTESIAN_POINT('Ctrl Pts',(-21.,-3.82734562477572,-6.25178572573963));
#54989=CARTESIAN_POINT('Ctrl Pts',(-50.,-3.87752560957259,-6.33279865263617));
#54990=CARTESIAN_POINT('Ctrl Pts',(-21.,-3.87752560957259,-6.33279865263617));
#54991=CARTESIAN_POINT('Ctrl Pts',(-50.,-3.93897729264122,-6.43496121510494));
#54992=CARTESIAN_POINT('Ctrl Pts',(-21.,-3.93897729264122,-6.43496121510494));
#54993=CARTESIAN_POINT('Ctrl Pts',(-50.,-3.99940195660266,-6.53784434718121));
#54994=CARTESIAN_POINT('Ctrl Pts',(-21.,-3.99940195660266,-6.53784434718121));
#54995=CARTESIAN_POINT('Ctrl Pts',(-50.,-4.0592984076569,-6.64109222642907));
#54996=CARTESIAN_POINT('Ctrl Pts',(-21.,-4.0592984076569,-6.64109222642907));
#54997=CARTESIAN_POINT('Ctrl Pts',(-50.,-4.11951535961712,-6.74409882925098));
#54998=CARTESIAN_POINT('Ctrl Pts',(-21.,-4.11951535961712,-6.74409882925098));
#54999=CARTESIAN_POINT('Ctrl Pts',(-50.,-4.18120131531612,-6.84606267872027));
#55000=CARTESIAN_POINT('Ctrl Pts',(-21.,-4.18120131531612,-6.84606267872027));
#55001=CARTESIAN_POINT('Ctrl Pts',(-50.,-4.24574967308285,-6.94604996627335));
#55002=CARTESIAN_POINT('Ctrl Pts',(-21.,-4.24574967308285,-6.94604996627335));
#55003=CARTESIAN_POINT('Ctrl Pts',(-50.,-4.31473193577955,-7.04305867353628));
#55004=CARTESIAN_POINT('Ctrl Pts',(-21.,-4.31473193577955,-7.04305867353628));
#55005=CARTESIAN_POINT('Ctrl Pts',(-50.,-4.38987557857684,-7.13606957084443));
#55006=CARTESIAN_POINT('Ctrl Pts',(-21.,-4.38987557857684,-7.13606957084443));
#55007=CARTESIAN_POINT('Ctrl Pts',(-50.,-4.4726472158023,-7.22422822821349));
#55008=CARTESIAN_POINT('Ctrl Pts',(-21.,-4.4726472158023,-7.22422822821349));
#55009=CARTESIAN_POINT('Ctrl Pts',(-50.,-4.56369441608956,-7.30707985875561));
#55010=CARTESIAN_POINT('Ctrl Pts',(-21.,-4.56369441608956,-7.30707985875561));
#55011=CARTESIAN_POINT('Ctrl Pts',(-50.,-4.66243591843162,-7.38474417264741));
#55012=CARTESIAN_POINT('Ctrl Pts',(-21.,-4.66243591843162,-7.38474417264741));
#55013=CARTESIAN_POINT('Ctrl Pts',(-50.,-4.76632422816958,-7.45822827381644));
#55014=CARTESIAN_POINT('Ctrl Pts',(-21.,-4.76632422816958,-7.45822827381644));
#55015=CARTESIAN_POINT('Ctrl Pts',(-50.,-4.87177973271099,-7.52903405731413));
#55016=CARTESIAN_POINT('Ctrl Pts',(-21.,-4.87177973271099,-7.52903405731413));
#55017=CARTESIAN_POINT('Ctrl Pts',(-50.,-4.97594840210465,-7.59842098612654));
#55018=CARTESIAN_POINT('Ctrl Pts',(-21.,-4.97594840210465,-7.59842098612654));
#55019=CARTESIAN_POINT('Ctrl Pts',(-50.,-5.07792505734327,-7.66688869302314));
#55020=CARTESIAN_POINT('Ctrl Pts',(-21.,-5.07792505734327,-7.66688869302314));
#55021=CARTESIAN_POINT('Ctrl Pts',(-50.,-5.18084571969554,-7.73330841361203));
#55022=CARTESIAN_POINT('Ctrl Pts',(-21.,-5.18084571969554,-7.73330841361203));
#55023=CARTESIAN_POINT('Ctrl Pts',(-50.,-5.29104691989087,-7.79523468647088));
#55024=CARTESIAN_POINT('Ctrl Pts',(-21.,-5.29104691989087,-7.79523468647088));
#55025=CARTESIAN_POINT('Ctrl Pts',(-50.,-5.41436931107715,-7.85036305479183));
#55026=CARTESIAN_POINT('Ctrl Pts',(-21.,-5.41436931107715,-7.85036305479183));
#55027=CARTESIAN_POINT('Ctrl Pts',(-50.,-5.55346250303877,-7.89758853118704));
#55028=CARTESIAN_POINT('Ctrl Pts',(-21.,-5.55346250303877,-7.89758853118704));
#55029=CARTESIAN_POINT('Ctrl Pts',(-50.,-5.70417884215966,-7.9384225480224));
#55030=CARTESIAN_POINT('Ctrl Pts',(-21.,-5.70417884215966,-7.9384225480224));
#55031=CARTESIAN_POINT('Ctrl Pts',(-50.,-5.85383639353758,-7.97768059592143));
#55032=CARTESIAN_POINT('Ctrl Pts',(-21.,-5.85383639353758,-7.97768059592143));
#55033=CARTESIAN_POINT('Ctrl Pts',(-50.,-5.98484872630544,-8.02208111792391));
#55034=CARTESIAN_POINT('Ctrl Pts',(-21.,-5.98484872630544,-8.02208111792391));
#55035=CARTESIAN_POINT('Ctrl Pts',(-50.,-6.07745474980597,-8.07919480518469));
#55036=CARTESIAN_POINT('Ctrl Pts',(-21.,-6.07745474980597,-8.07919480518469));
#55037=CARTESIAN_POINT('Ctrl Pts',(-50.,-6.11271586583108,-8.15628970164627));
#55038=CARTESIAN_POINT('Ctrl Pts',(-21.,-6.11271586583108,-8.15628970164627));
#55039=CARTESIAN_POINT('Ctrl Pts',(-50.,-6.07559280712476,-8.2591466623313));
#55040=CARTESIAN_POINT('Ctrl Pts',(-21.,-6.07559280712476,-8.2591466623313));
#55041=CARTESIAN_POINT('Ctrl Pts',(-50.,-5.9546471286083,-8.39217131123866));
#55042=CARTESIAN_POINT('Ctrl Pts',(-21.,-5.9546471286083,-8.39217131123866));
#55043=CARTESIAN_POINT('Ctrl Pts',(-50.,-5.74145902217939,-8.55861531001153));
#55044=CARTESIAN_POINT('Ctrl Pts',(-21.,-5.74145902217939,-8.55861531001153));
#55045=CARTESIAN_POINT('Ctrl Pts',(-50.,-5.43017572522592,-8.76074759285599));
#55046=CARTESIAN_POINT('Ctrl Pts',(-21.,-5.43017572522592,-8.76074759285599));
#55047=CARTESIAN_POINT('Ctrl Pts',(-50.,-5.01703058178298,-9.00003708168539));
#55048=CARTESIAN_POINT('Ctrl Pts',(-21.,-5.01703058178298,-9.00003708168539));
#55049=CARTESIAN_POINT('Ctrl Pts',(-50.,-4.49989887410451,-9.27732143685757));
#55050=CARTESIAN_POINT('Ctrl Pts',(-21.,-4.49989887410451,-9.27732143685757));
#55051=CARTESIAN_POINT('Ctrl Pts',(-50.,-3.87785991426877,-9.59297357001867));
#55052=CARTESIAN_POINT('Ctrl Pts',(-21.,-3.87785991426877,-9.59297357001867));
#55053=CARTESIAN_POINT('Ctrl Pts',(-50.,-3.29619308135874,-9.87624406382134));
#55054=CARTESIAN_POINT('Ctrl Pts',(-21.,-3.29619308135874,-9.87624406382134));
#55055=CARTESIAN_POINT('Ctrl Pts',(-50.,-2.8127788859222,-10.1059570283115));
#55056=CARTESIAN_POINT('Ctrl Pts',(-21.,-2.8127788859222,-10.1059570283115));
#55057=CARTESIAN_POINT('Ctrl Pts',(-50.,-2.46956880972213,-10.2667599606609));
#55058=CARTESIAN_POINT('Ctrl Pts',(-21.,-2.46956880972213,-10.2667599606609));
#55059=CARTESIAN_POINT('Ctrl Pts',(-50.,-2.29273028380004,-10.3490766663382));
#55060=CARTESIAN_POINT('Ctrl Pts',(-21.,-2.29273028380004,-10.3490766663382));
#55061=CARTESIAN_POINT('',(-21.5,-5.96964178495622,-8.0226789141349));
#55062=CARTESIAN_POINT('Ctrl Pts',(-21.5,-5.96964178495622,-8.0226789141349));
#55063=CARTESIAN_POINT('Ctrl Pts',(-21.4716400099246,-5.94010387156942,
-8.0093081760176));
#55064=CARTESIAN_POINT('Ctrl Pts',(-21.4423497933807,-5.90702876507278,
-7.99736128679948));
#55065=CARTESIAN_POINT('Ctrl Pts',(-21.2909092331881,-5.72905875837931,
-7.9402495905054));
#55066=CARTESIAN_POINT('Ctrl Pts',(-21.1629721875807,-5.55527241504855,
-7.90713720025227));
#55067=CARTESIAN_POINT('Ctrl Pts',(-21.,-5.37719972469147,-7.83171265565699));
#55068=CARTESIAN_POINT('Ctrl Pts',(-50.,-5.96964178495622,-8.0226789141349));
#55069=CARTESIAN_POINT('Ctrl Pts',(-45.1666666666667,-5.96964178495622,
-8.0226789141349));
#55070=CARTESIAN_POINT('Ctrl Pts',(-40.3333333333333,-5.96964178495622,
-8.0226789141349));
#55071=CARTESIAN_POINT('Ctrl Pts',(-30.8333333333333,-5.96964178495622,
-8.0226789141349));
#55072=CARTESIAN_POINT('Ctrl Pts',(-26.1666666666667,-5.96964178495622,
-8.0226789141349));
#55073=CARTESIAN_POINT('Ctrl Pts',(-21.5,-5.96964178495622,-8.0226789141349));
#55074=CARTESIAN_POINT('Origin',(-21.25,0.,0.));
#55075=CARTESIAN_POINT('Origin',(-21.5,0.,0.));
#55076=CARTESIAN_POINT('Origin',(-35.75,0.,0.));
#55077=CARTESIAN_POINT('Ctrl Pts',(-50.,-6.03932124977421,-3.89701874412038));
#55078=CARTESIAN_POINT('Ctrl Pts',(-21.,-6.03932124977421,-3.89701874412038));
#55079=CARTESIAN_POINT('Ctrl Pts',(-50.,-6.05965257770704,-3.90939030583537));
#55080=CARTESIAN_POINT('Ctrl Pts',(-21.,-6.05965257770704,-3.90939030583537));
#55081=CARTESIAN_POINT('Ctrl Pts',(-50.,-6.10023490810719,-3.93427763849175));
#55082=CARTESIAN_POINT('Ctrl Pts',(-21.,-6.10023490810719,-3.93427763849175));
#55083=CARTESIAN_POINT('Ctrl Pts',(-50.,-6.16086742147115,-3.97204127711522));
#55084=CARTESIAN_POINT('Ctrl Pts',(-21.,-6.16086742147115,-3.97204127711522));
#55085=CARTESIAN_POINT('Ctrl Pts',(-50.,-6.24122821720367,-4.02325912271413));
#55086=CARTESIAN_POINT('Ctrl Pts',(-21.,-6.24122821720367,-4.02325912271413));
#55087=CARTESIAN_POINT('Ctrl Pts',(-50.,-6.34092094513049,-4.08864152493875));
#55088=CARTESIAN_POINT('Ctrl Pts',(-21.,-6.34092094513049,-4.08864152493875));
#55089=CARTESIAN_POINT('Ctrl Pts',(-50.,-6.44000100425059,-4.15511874483724));
#55090=CARTESIAN_POINT('Ctrl Pts',(-21.,-6.44000100425059,-4.15511874483724));
#55091=CARTESIAN_POINT('Ctrl Pts',(-50.,-6.53876341785232,-4.22215377357323));
#55092=CARTESIAN_POINT('Ctrl Pts',(-21.,-6.53876341785232,-4.22215377357323));
#55093=CARTESIAN_POINT('Ctrl Pts',(-50.,-6.63770990687462,-4.2888323596294));
#55094=CARTESIAN_POINT('Ctrl Pts',(-21.,-6.63770990687462,-4.2888323596294));
#55095=CARTESIAN_POINT('Ctrl Pts',(-50.,-6.73752748880879,-4.35393408054299));
#55096=CARTESIAN_POINT('Ctrl Pts',(-21.,-6.73752748880879,-4.35393408054299));
#55097=CARTESIAN_POINT('Ctrl Pts',(-50.,-6.83906640781858,-4.4160130309926));
#55098=CARTESIAN_POINT('Ctrl Pts',(-21.,-6.83906640781858,-4.4160130309926));
#55099=CARTESIAN_POINT('Ctrl Pts',(-50.,-6.94330777957998,-4.47348457408032));
#55100=CARTESIAN_POINT('Ctrl Pts',(-21.,-6.94330777957998,-4.47348457408032));
#55101=CARTESIAN_POINT('Ctrl Pts',(-50.,-7.05136577826386,-4.52468089222283));
#55102=CARTESIAN_POINT('Ctrl Pts',(-21.,-7.05136577826386,-4.52468089222283));
#55103=CARTESIAN_POINT('Ctrl Pts',(-50.,-7.16419105444418,-4.56819583049617));
#55104=CARTESIAN_POINT('Ctrl Pts',(-21.,-7.16419105444418,-4.56819583049617));
#55105=CARTESIAN_POINT('Ctrl Pts',(-50.,-7.28216972266428,-4.60333867057275));
#55106=CARTESIAN_POINT('Ctrl Pts',(-21.,-7.28216972266428,-4.60333867057275));
#55107=CARTESIAN_POINT('Ctrl Pts',(-50.,-7.40483002515176,-4.63046946729401));
#55108=CARTESIAN_POINT('Ctrl Pts',(-21.,-7.40483002515176,-4.63046946729401));
#55109=CARTESIAN_POINT('Ctrl Pts',(-50.,-7.53031371454558,-4.65160090645338));
#55110=CARTESIAN_POINT('Ctrl Pts',(-21.,-7.53031371454558,-4.65160090645338));
#55111=CARTESIAN_POINT('Ctrl Pts',(-50.,-7.65604731918147,-4.66963928443128));
#55112=CARTESIAN_POINT('Ctrl Pts',(-21.,-7.65604731918147,-4.66963928443128));
#55113=CARTESIAN_POINT('Ctrl Pts',(-50.,-7.78000590743498,-4.68695765535521));
#55114=CARTESIAN_POINT('Ctrl Pts',(-21.,-7.78000590743498,-4.68695765535521));
#55115=CARTESIAN_POINT('Ctrl Pts',(-50.,-7.9015907237349,-4.70439891524807));
#55116=CARTESIAN_POINT('Ctrl Pts',(-21.,-7.9015907237349,-4.70439891524807));
#55117=CARTESIAN_POINT('Ctrl Pts',(-50.,-8.02313747309844,-4.71958541389958));
#55118=CARTESIAN_POINT('Ctrl Pts',(-21.,-8.02313747309844,-4.71958541389958));
#55119=CARTESIAN_POINT('Ctrl Pts',(-50.,-8.14929412649754,-4.72756454905465));
#55120=CARTESIAN_POINT('Ctrl Pts',(-21.,-8.14929412649754,-4.72756454905465));
#55121=CARTESIAN_POINT('Ctrl Pts',(-50.,-8.2843230642502,-4.72372591244526));
#55122=CARTESIAN_POINT('Ctrl Pts',(-21.,-8.2843230642502,-4.72372591244526));
#55123=CARTESIAN_POINT('Ctrl Pts',(-50.,-8.43013206622476,-4.7059243222351));
#55124=CARTESIAN_POINT('Ctrl Pts',(-21.,-8.43013206622476,-4.7059243222351));
#55125=CARTESIAN_POINT('Ctrl Pts',(-50.,-8.58364001156461,-4.67732113139128));
#55126=CARTESIAN_POINT('Ctrl Pts',(-21.,-8.58364001156461,-4.67732113139128));
#55127=CARTESIAN_POINT('Ctrl Pts',(-50.,-8.73551023481551,-4.6477574323839));
#55128=CARTESIAN_POINT('Ctrl Pts',(-21.,-8.73551023481551,-4.6477574323839));
#55129=CARTESIAN_POINT('Ctrl Pts',(-50.,-8.87281293245584,-4.63091679961492));
#55130=CARTESIAN_POINT('Ctrl Pts',(-21.,-8.87281293245584,-4.63091679961492));
#55131=CARTESIAN_POINT('Ctrl Pts',(-50.,-8.98102877679355,-4.64219420602678));
#55132=CARTESIAN_POINT('Ctrl Pts',(-21.,-8.98102877679355,-4.64219420602678));
#55133=CARTESIAN_POINT('Ctrl Pts',(-50.,-9.04624816652329,-4.69635508274639));
#55134=CARTESIAN_POINT('Ctrl Pts',(-21.,-9.04624816652329,-4.69635508274639));
#55135=CARTESIAN_POINT('Ctrl Pts',(-50.,-9.05742940904388,-4.80513309368965));
#55136=CARTESIAN_POINT('Ctrl Pts',(-21.,-9.05742940904388,-4.80513309368965));
#55137=CARTESIAN_POINT('Ctrl Pts',(-50.,-9.00617835005594,-4.97746052424366));
#55138=CARTESIAN_POINT('Ctrl Pts',(-21.,-9.00617835005594,-4.97746052424366));
#55139=CARTESIAN_POINT('Ctrl Pts',(-50.,-8.88631984769767,-5.21992023813997));
#55140=CARTESIAN_POINT('Ctrl Pts',(-21.,-8.88631984769767,-5.21992023813997));
#55141=CARTESIAN_POINT('Ctrl Pts',(-50.,-8.6935651987215,-5.53709589298789));
#55142=CARTESIAN_POINT('Ctrl Pts',(-21.,-8.6935651987215,-5.53709589298789));
#55143=CARTESIAN_POINT('Ctrl Pts',(-50.,-8.42515810469916,-5.93194523247474));
#55144=CARTESIAN_POINT('Ctrl Pts',(-21.,-8.42515810469916,-5.93194523247474));
#55145=CARTESIAN_POINT('Ctrl Pts',(-50.,-8.07954770829655,-6.40614484298506));
#55146=CARTESIAN_POINT('Ctrl Pts',(-21.,-8.07954770829655,-6.40614484298506));
#55147=CARTESIAN_POINT('Ctrl Pts',(-50.,-7.65606629865851,-6.96043017782053));
#55148=CARTESIAN_POINT('Ctrl Pts',(-21.,-7.65606629865851,-6.96043017782053));
#55149=CARTESIAN_POINT('Ctrl Pts',(-50.,-7.25490905174796,-7.46802385431575));
#55150=CARTESIAN_POINT('Ctrl Pts',(-21.,-7.25490905174796,-7.46802385431575));
#55151=CARTESIAN_POINT('Ctrl Pts',(-50.,-6.91903663131433,-7.8847336425335));
#55152=CARTESIAN_POINT('Ctrl Pts',(-21.,-6.91903663131433,-7.8847336425335));
#55153=CARTESIAN_POINT('Ctrl Pts',(-50.,-6.67958481505646,-8.17852534961221));
#55154=CARTESIAN_POINT('Ctrl Pts',(-21.,-6.67958481505646,-8.17852534961221));
#55155=CARTESIAN_POINT('Ctrl Pts',(-50.,-6.55597468860601,-8.32941749958287));
#55156=CARTESIAN_POINT('Ctrl Pts',(-21.,-6.55597468860601,-8.32941749958287));
#55157=CARTESIAN_POINT('',(-21.5,-8.85937132577942,-4.63805343996351));
#55158=CARTESIAN_POINT('Ctrl Pts',(-50.,-8.85937132577942,-4.63805343996351));
#55159=CARTESIAN_POINT('Ctrl Pts',(-45.1666666666667,-8.85937132577942,
-4.63805343996351));
#55160=CARTESIAN_POINT('Ctrl Pts',(-40.3333333333333,-8.85937132577942,
-4.63805343996351));
#55161=CARTESIAN_POINT('Ctrl Pts',(-30.8333333333333,-8.85937132577942,
-4.63805343996351));
#55162=CARTESIAN_POINT('Ctrl Pts',(-26.1666666666667,-8.85937132577942,
-4.63805343996351));
#55163=CARTESIAN_POINT('Ctrl Pts',(-21.5,-8.85937132577942,-4.63805343996351));
#55164=CARTESIAN_POINT('',(-50.,-6.03932124977421,-3.89701874412038));
#55165=CARTESIAN_POINT('Ctrl Pts',(-21.5,-8.85937132577942,-4.63805343996351));
#55166=CARTESIAN_POINT('Ctrl Pts',(-21.4716714037532,-8.82699312116188,
-4.63882198977592));
#55167=CARTESIAN_POINT('Ctrl Pts',(-21.442415011075,-8.79205190661509,-4.64240188595699));
#55168=CARTESIAN_POINT('Ctrl Pts',(-21.2909879716453,-8.60695266172876,
-4.66814581613047));
#55169=CARTESIAN_POINT('Ctrl Pts',(-21.1630186724949,-8.43596084926626,
-4.71373942955307));
#55170=CARTESIAN_POINT('Ctrl Pts',(-21.,-8.24274231917123,-4.72304976257329));
#55171=CARTESIAN_POINT('Origin',(-50.,0.,0.));
#55172=CARTESIAN_POINT('',(-50.,-5.14318775290069,-5.02073460645077));
#55173=CARTESIAN_POINT('Ctrl Pts',(-50.,-6.55597468860601,-8.32941749958287));
#55174=CARTESIAN_POINT('Ctrl Pts',(-21.,-6.55597468860601,-8.32941749958287));
#55175=CARTESIAN_POINT('Ctrl Pts',(-50.,-6.55632766789962,-8.30553668898452));
#55176=CARTESIAN_POINT('Ctrl Pts',(-21.,-6.55632766789962,-8.30553668898452));
#55177=CARTESIAN_POINT('Ctrl Pts',(-50.,-6.55682598292761,-8.25785023779518));
#55178=CARTESIAN_POINT('Ctrl Pts',(-21.,-6.55682598292761,-8.25785023779518));
#55179=CARTESIAN_POINT('Ctrl Pts',(-50.,-6.55695052439907,-8.18654607180369));
#55180=CARTESIAN_POINT('Ctrl Pts',(-21.,-6.55695052439907,-8.18654607180369));
#55181=CARTESIAN_POINT('Ctrl Pts',(-50.,-6.55586906420034,-8.0919254651127));
#55182=CARTESIAN_POINT('Ctrl Pts',(-21.,-6.55586906420034,-8.0919254651127));
#55183=CARTESIAN_POINT('Ctrl Pts',(-50.,-6.55242508650163,-7.97441053046901));
#55184=CARTESIAN_POINT('Ctrl Pts',(-21.,-6.55242508650163,-7.97441053046901));
#55185=CARTESIAN_POINT('Ctrl Pts',(-50.,-6.54686687486885,-7.85767464841055));
#55186=CARTESIAN_POINT('Ctrl Pts',(-21.,-6.54686687486885,-7.85767464841055));
#55187=CARTESIAN_POINT('Ctrl Pts',(-50.,-6.53916282696568,-7.74174994850129));
#55188=CARTESIAN_POINT('Ctrl Pts',(-21.,-6.53916282696568,-7.74174994850129));
#55189=CARTESIAN_POINT('Ctrl Pts',(-50.,-6.5292721024685,-7.6266854031787));
#55190=CARTESIAN_POINT('Ctrl Pts',(-21.,-6.5292721024685,-7.6266854031787));
#55191=CARTESIAN_POINT('Ctrl Pts',(-50.,-6.51714368227899,-7.51255191568566));
#55192=CARTESIAN_POINT('Ctrl Pts',(-21.,-6.51714368227899,-7.51255191568566));
#55193=CARTESIAN_POINT('Ctrl Pts',(-50.,-6.5027237919627,-7.39943421923609));
#55194=CARTESIAN_POINT('Ctrl Pts',(-21.,-6.5027237919627,-7.39943421923609));
#55195=CARTESIAN_POINT('Ctrl Pts',(-50.,-6.48596514159778,-7.28741967054497));
#55196=CARTESIAN_POINT('Ctrl Pts',(-21.,-6.48596514159778,-7.28741967054497));
#55197=CARTESIAN_POINT('Ctrl Pts',(-50.,-6.46683693263443,-7.17658703219621));
#55198=CARTESIAN_POINT('Ctrl Pts',(-21.,-6.46683693263443,-7.17658703219621));
#55199=CARTESIAN_POINT('Ctrl Pts',(-50.,-6.44533241567678,-7.06699729667253));
#55200=CARTESIAN_POINT('Ctrl Pts',(-21.,-6.44533241567678,-7.06699729667253));
#55201=CARTESIAN_POINT('Ctrl Pts',(-50.,-6.42148411170256,-6.9586779143977));
#55202=CARTESIAN_POINT('Ctrl Pts',(-21.,-6.42148411170256,-6.9586779143977));
#55203=CARTESIAN_POINT('Ctrl Pts',(-50.,-6.39534644338642,-6.85163598146165));
#55204=CARTESIAN_POINT('Ctrl Pts',(-21.,-6.39534644338642,-6.85163598146165));
#55205=CARTESIAN_POINT('Ctrl Pts',(-50.,-6.36696110296949,-6.74588705654512));
#55206=CARTESIAN_POINT('Ctrl Pts',(-21.,-6.36696110296949,-6.74588705654512));
#55207=CARTESIAN_POINT('Ctrl Pts',(-50.,-6.33632590879467,-6.64148049150319));
#55208=CARTESIAN_POINT('Ctrl Pts',(-21.,-6.33632590879467,-6.64148049150319));
#55209=CARTESIAN_POINT('Ctrl Pts',(-50.,-6.30336681095649,-6.53852299564495));
#55210=CARTESIAN_POINT('Ctrl Pts',(-21.,-6.30336681095649,-6.53852299564495));
#55211=CARTESIAN_POINT('Ctrl Pts',(-50.,-6.2678972444421,-6.43721103768399));
#55212=CARTESIAN_POINT('Ctrl Pts',(-21.,-6.2678972444421,-6.43721103768399));
#55213=CARTESIAN_POINT('Ctrl Pts',(-50.,-6.22963155144596,-6.33782488040964));
#55214=CARTESIAN_POINT('Ctrl Pts',(-21.,-6.22963155144596,-6.33782488040964));
#55215=CARTESIAN_POINT('Ctrl Pts',(-50.,-6.18823844577549,-6.2406935262026));
#55216=CARTESIAN_POINT('Ctrl Pts',(-21.,-6.18823844577549,-6.2406935262026));
#55217=CARTESIAN_POINT('Ctrl Pts',(-50.,-6.14338347043832,-6.14616869769857));
#55218=CARTESIAN_POINT('Ctrl Pts',(-21.,-6.14338347043832,-6.14616869769857));
#55219=CARTESIAN_POINT('Ctrl Pts',(-50.,-6.09477471117184,-6.05459405347559));
#55220=CARTESIAN_POINT('Ctrl Pts',(-21.,-6.09477471117184,-6.05459405347559));
#55221=CARTESIAN_POINT('Ctrl Pts',(-50.,-6.04221154361855,-5.96627851638222));
#55222=CARTESIAN_POINT('Ctrl Pts',(-21.,-6.04221154361855,-5.96627851638222));
#55223=CARTESIAN_POINT('Ctrl Pts',(-50.,-5.98561485393513,-5.88145719317904));
#55224=CARTESIAN_POINT('Ctrl Pts',(-21.,-5.98561485393513,-5.88145719317904));
#55225=CARTESIAN_POINT('Ctrl Pts',(-50.,-5.92504262139805,-5.80024683316115));
#55226=CARTESIAN_POINT('Ctrl Pts',(-21.,-5.92504262139805,-5.80024683316115));
#55227=CARTESIAN_POINT('Ctrl Pts',(-50.,-5.86071379627312,-5.72259822644884));
#55228=CARTESIAN_POINT('Ctrl Pts',(-21.,-5.86071379627312,-5.72259822644884));
#55229=CARTESIAN_POINT('Ctrl Pts',(-50.,-5.79302399301176,-5.64825683559838));
#55230=CARTESIAN_POINT('Ctrl Pts',(-21.,-5.79302399301176,-5.64825683559838));
#55231=CARTESIAN_POINT('Ctrl Pts',(-50.,-5.72258159055366,-5.57669744070723));
#55232=CARTESIAN_POINT('Ctrl Pts',(-21.,-5.72258159055366,-5.57669744070723));
#55233=CARTESIAN_POINT('Ctrl Pts',(-50.,-5.65014634083023,-5.50719043557996));
#55234=CARTESIAN_POINT('Ctrl Pts',(-21.,-5.65014634083023,-5.50719043557996));
#55235=CARTESIAN_POINT('Ctrl Pts',(-50.,-5.57653243923659,-5.43891687637388));
#55236=CARTESIAN_POINT('Ctrl Pts',(-21.,-5.57653243923659,-5.43891687637388));
#55237=CARTESIAN_POINT('Ctrl Pts',(-50.,-5.50252175190725,-5.37106909242141));
#55238=CARTESIAN_POINT('Ctrl Pts',(-21.,-5.50252175190725,-5.37106909242141));
#55239=CARTESIAN_POINT('Ctrl Pts',(-50.,-5.42877754716296,-5.30295185702147));
#55240=CARTESIAN_POINT('Ctrl Pts',(-21.,-5.42877754716296,-5.30295185702147));
#55241=CARTESIAN_POINT('Ctrl Pts',(-50.,-5.35574541658332,-5.23409735978387));
#55242=CARTESIAN_POINT('Ctrl Pts',(-21.,-5.35574541658332,-5.23409735978387));
#55243=CARTESIAN_POINT('Ctrl Pts',(-50.,-5.28368554926634,-5.16423261553338));
#55244=CARTESIAN_POINT('Ctrl Pts',(-21.,-5.28368554926634,-5.16423261553338));
#55245=CARTESIAN_POINT('Ctrl Pts',(-50.,-5.22691734521339,-5.10742564369891));
#55246=CARTESIAN_POINT('Ctrl Pts',(-21.,-5.22691734521339,-5.10742564369891));
#55247=CARTESIAN_POINT('Ctrl Pts',(-50.,-5.18485354740602,-5.06428722179623));
#55248=CARTESIAN_POINT('Ctrl Pts',(-21.,-5.18485354740602,-5.06428722179623));
#55249=CARTESIAN_POINT('Ctrl Pts',(-50.,-5.15703844666268,-5.03529159113598));
#55250=CARTESIAN_POINT('Ctrl Pts',(-21.,-5.15703844666268,-5.03529159113598));
#55251=CARTESIAN_POINT('Ctrl Pts',(-50.,-5.14318775290069,-5.02073460645076));
#55252=CARTESIAN_POINT('Ctrl Pts',(-21.,-5.14318775290069,-5.02073460645076));
#55253=CARTESIAN_POINT('',(-21.5,-6.52388598275277,-7.57884632935924));
#55254=CARTESIAN_POINT('Ctrl Pts',(-21.5,-6.52388598275277,-7.57884632935924));
#55255=CARTESIAN_POINT('Ctrl Pts',(-26.3333333333333,-6.52388598275277,
-7.57884632935924));
#55256=CARTESIAN_POINT('Ctrl Pts',(-31.1666666666667,-6.52388598275277,
-7.57884632935924));
#55257=CARTESIAN_POINT('Ctrl Pts',(-40.6666666666667,-6.52388598275277,
-7.57884632935924));
#55258=CARTESIAN_POINT('Ctrl Pts',(-45.3333333333333,-6.52388598275276,
-7.57884632935924));
#55259=CARTESIAN_POINT('Ctrl Pts',(-50.,-6.52388598275276,-7.57884632935924));
#55260=CARTESIAN_POINT('Ctrl Pts',(-21.,-6.42894112865204,-6.99419158761942));
#55261=CARTESIAN_POINT('Ctrl Pts',(-21.1171767610974,-6.45853087308246,
-7.12615087039119));
#55262=CARTESIAN_POINT('Ctrl Pts',(-21.2874825276444,-6.49694802882356,
-7.32162583711084));
#55263=CARTESIAN_POINT('Ctrl Pts',(-21.5,-6.52388598275277,-7.57884632935924));
#55264=CARTESIAN_POINT('Origin',(-35.75,0.,0.));
#55265=CARTESIAN_POINT('',(-21.5,-9.16615635178499,-3.9976965535958));
#55266=CARTESIAN_POINT('Origin',(-21.5,0.,0.));
#55267=CARTESIAN_POINT('Ctrl Pts',(-21.5,-9.16615635178499,-3.9976965535958));
#55268=CARTESIAN_POINT('Ctrl Pts',(-26.3333333333333,-9.16615635178499,
-3.9976965535958));
#55269=CARTESIAN_POINT('Ctrl Pts',(-31.1666666666667,-9.16615635178499,
-3.9976965535958));
#55270=CARTESIAN_POINT('Ctrl Pts',(-40.6666666666667,-9.16615635178499,
-3.9976965535958));
#55271=CARTESIAN_POINT('Ctrl Pts',(-45.3333333333333,-9.16615635178499,
-3.9976965535958));
#55272=CARTESIAN_POINT('Ctrl Pts',(-50.,-9.16615635178499,-3.9976965535958));
#55273=CARTESIAN_POINT('Origin',(-21.25,0.,0.));
#55274=CARTESIAN_POINT('Ctrl Pts',(-21.,-8.82694180863381,-3.51213586112389));
#55275=CARTESIAN_POINT('Ctrl Pts',(-21.1171767610952,-8.91085623419347,
-3.61818855777691));
#55276=CARTESIAN_POINT('Ctrl Pts',(-21.2874825276427,-9.03028230497426,
-3.77763683806661));
#55277=CARTESIAN_POINT('Ctrl Pts',(-21.5,-9.16615635178499,-3.9976965535958));
#55278=CARTESIAN_POINT('Ctrl Pts',(-50.,-9.52072790258051,-4.66001504343333));
#55279=CARTESIAN_POINT('Ctrl Pts',(-21.,-9.52072790258051,-4.66001504343333));
#55280=CARTESIAN_POINT('Ctrl Pts',(-50.,-9.5106844305395,-4.6383460245682));
#55281=CARTESIAN_POINT('Ctrl Pts',(-21.,-9.5106844305395,-4.6383460245682));
#55282=CARTESIAN_POINT('Ctrl Pts',(-50.,-9.49044302111884,-4.59516580583826));
#55283=CARTESIAN_POINT('Ctrl Pts',(-21.,-9.49044302111884,-4.59516580583826));
#55284=CARTESIAN_POINT('Ctrl Pts',(-50.,-9.45961751095234,-4.53086893560887));
#55285=CARTESIAN_POINT('Ctrl Pts',(-21.,-9.45961751095234,-4.53086893560887));
#55286=CARTESIAN_POINT('Ctrl Pts',(-50.,-9.41758880635275,-4.44608794271298));
#55287=CARTESIAN_POINT('Ctrl Pts',(-21.,-9.41758880635275,-4.44608794271298));
#55288=CARTESIAN_POINT('Ctrl Pts',(-50.,-9.36349807041911,-4.34170493100677));
#55289=CARTESIAN_POINT('Ctrl Pts',(-21.,-9.36349807041911,-4.34170493100677));
#55290=CARTESIAN_POINT('Ctrl Pts',(-50.,-9.30784049378005,-4.23894115315102));
#55291=CARTESIAN_POINT('Ctrl Pts',(-21.,-9.30784049378005,-4.23894115315102));
#55292=CARTESIAN_POINT('Ctrl Pts',(-50.,-9.25060154420976,-4.1378392686224));
#55293=CARTESIAN_POINT('Ctrl Pts',(-21.,-9.25060154420976,-4.1378392686224));
#55294=CARTESIAN_POINT('Ctrl Pts',(-50.,-9.19176567419237,-4.03846112001482));
#55295=CARTESIAN_POINT('Ctrl Pts',(-21.,-9.19176567419237,-4.03846112001482));
#55296=CARTESIAN_POINT('Ctrl Pts',(-50.,-9.13131768087278,-3.94089272529988));
#55297=CARTESIAN_POINT('Ctrl Pts',(-21.,-9.13131768087278,-3.94089272529988));
#55298=CARTESIAN_POINT('Ctrl Pts',(-50.,-9.06924587952332,-3.84523375831808));
#55299=CARTESIAN_POINT('Ctrl Pts',(-21.,-9.06924587952332,-3.84523375831808));
#55300=CARTESIAN_POINT('Ctrl Pts',(-50.,-9.0055455660548,-3.75158344307814));
#55301=CARTESIAN_POINT('Ctrl Pts',(-21.,-9.0055455660548,-3.75158344307814));
#55302=CARTESIAN_POINT('Ctrl Pts',(-50.,-8.94022316573707,-3.66002610520606));
#55303=CARTESIAN_POINT('Ctrl Pts',(-21.,-8.94022316573707,-3.66002610520606));
#55304=CARTESIAN_POINT('Ctrl Pts',(-50.,-8.87329906122102,-3.57061962548306));
#55305=CARTESIAN_POINT('Ctrl Pts',(-21.,-8.87329906122102,-3.57061962548306));
#55306=CARTESIAN_POINT('Ctrl Pts',(-50.,-8.80481446318767,-3.48337462556297));
#55307=CARTESIAN_POINT('Ctrl Pts',(-21.,-8.80481446318767,-3.48337462556297));
#55308=CARTESIAN_POINT('Ctrl Pts',(-50.,-8.7348214836506,-3.3982738856883));
#55309=CARTESIAN_POINT('Ctrl Pts',(-21.,-8.7348214836506,-3.3982738856883));
#55310=CARTESIAN_POINT('Ctrl Pts',(-50.,-8.66336443667969,-3.31531333416059));
#55311=CARTESIAN_POINT('Ctrl Pts',(-21.,-8.66336443667969,-3.31531333416059));
#55312=CARTESIAN_POINT('Ctrl Pts',(-50.,-8.59046276963722,-3.23453838205034));
#55313=CARTESIAN_POINT('Ctrl Pts',(-21.,-8.59046276963722,-3.23453838205034));
#55314=CARTESIAN_POINT('Ctrl Pts',(-50.,-8.51609606529771,-3.15607730017284));
#55315=CARTESIAN_POINT('Ctrl Pts',(-21.,-8.51609606529771,-3.15607730017284));
#55316=CARTESIAN_POINT('Ctrl Pts',(-50.,-8.44018147897284,-3.08018804824792));
#55317=CARTESIAN_POINT('Ctrl Pts',(-21.,-8.44018147897284,-3.08018804824792));
#55318=CARTESIAN_POINT('Ctrl Pts',(-50.,-8.36258324333989,-3.00724707660037));
#55319=CARTESIAN_POINT('Ctrl Pts',(-21.,-8.36258324333989,-3.00724707660037));
#55320=CARTESIAN_POINT('Ctrl Pts',(-50.,-8.28314562863609,-2.93769454582461));
#55321=CARTESIAN_POINT('Ctrl Pts',(-21.,-8.28314562863609,-2.93769454582461));
#55322=CARTESIAN_POINT('Ctrl Pts',(-50.,-8.201719906256,-2.87199246251599));
#55323=CARTESIAN_POINT('Ctrl Pts',(-21.,-8.201719906256,-2.87199246251599));
#55324=CARTESIAN_POINT('Ctrl Pts',(-50.,-8.11819217840571,-2.81057710920625));
#55325=CARTESIAN_POINT('Ctrl Pts',(-21.,-8.11819217840571,-2.81057710920625));
#55326=CARTESIAN_POINT('Ctrl Pts',(-50.,-8.03251572538561,-2.75381386341092));
#55327=CARTESIAN_POINT('Ctrl Pts',(-21.,-8.03251572538561,-2.75381386341092));
#55328=CARTESIAN_POINT('Ctrl Pts',(-50.,-7.94472127708621,-2.70194887521209));
#55329=CARTESIAN_POINT('Ctrl Pts',(-21.,-7.94472127708621,-2.70194887521209));
#55330=CARTESIAN_POINT('Ctrl Pts',(-50.,-7.85491172665132,-2.65506217582471));
#55331=CARTESIAN_POINT('Ctrl Pts',(-21.,-7.85491172665132,-2.65506217582471));
#55332=CARTESIAN_POINT('Ctrl Pts',(-50.,-7.76326299008741,-2.61301442971916));
#55333=CARTESIAN_POINT('Ctrl Pts',(-21.,-7.76326299008741,-2.61301442971916));
#55334=CARTESIAN_POINT('Ctrl Pts',(-50.,-7.67002106404108,-2.5754046559055));
#55335=CARTESIAN_POINT('Ctrl Pts',(-21.,-7.67002106404108,-2.5754046559055));
#55336=CARTESIAN_POINT('Ctrl Pts',(-50.,-7.57550619462173,-2.54149568187359));
#55337=CARTESIAN_POINT('Ctrl Pts',(-21.,-7.57550619462173,-2.54149568187359));
#55338=CARTESIAN_POINT('Ctrl Pts',(-50.,-7.4800863304027,-2.5103005111467));
#55339=CARTESIAN_POINT('Ctrl Pts',(-21.,-7.4800863304027,-2.5103005111467));
#55340=CARTESIAN_POINT('Ctrl Pts',(-50.,-7.3841397096708,-2.4807280346756));
#55341=CARTESIAN_POINT('Ctrl Pts',(-21.,-7.3841397096708,-2.4807280346756));
#55342=CARTESIAN_POINT('Ctrl Pts',(-50.,-7.28802033430286,-2.45171132733138));
#55343=CARTESIAN_POINT('Ctrl Pts',(-21.,-7.28802033430286,-2.45171132733138));
#55344=CARTESIAN_POINT('Ctrl Pts',(-50.,-7.19202414084635,-2.42233623016115));
#55345=CARTESIAN_POINT('Ctrl Pts',(-21.,-7.19202414084635,-2.42233623016115));
#55346=CARTESIAN_POINT('Ctrl Pts',(-50.,-7.09634961812101,-2.39198792562662));
#55347=CARTESIAN_POINT('Ctrl Pts',(-21.,-7.09634961812101,-2.39198792562662));
#55348=CARTESIAN_POINT('Ctrl Pts',(-50.,-7.00111274457534,-2.36030757076476));
#55349=CARTESIAN_POINT('Ctrl Pts',(-21.,-7.00111274457534,-2.36030757076476));
#55350=CARTESIAN_POINT('Ctrl Pts',(-50.,-6.92531873868941,-2.33375705829959));
#55351=CARTESIAN_POINT('Ctrl Pts',(-21.,-6.92531873868941,-2.33375705829959));
#55352=CARTESIAN_POINT('Ctrl Pts',(-50.,-6.86870350660446,-2.31314148102898));
#55353=CARTESIAN_POINT('Ctrl Pts',(-21.,-6.86870350660446,-2.31314148102898));
#55354=CARTESIAN_POINT('Ctrl Pts',(-50.,-6.8310622341282,-2.29908584041335));
#55355=CARTESIAN_POINT('Ctrl Pts',(-21.,-6.8310622341282,-2.29908584041335));
#55356=CARTESIAN_POINT('Ctrl Pts',(-50.,-6.8122671513043,-2.29198004120026));
#55357=CARTESIAN_POINT('Ctrl Pts',(-21.,-6.8122671513043,-2.29198004120026));
#55358=CARTESIAN_POINT('',(-50.,-6.8122671513043,-2.29198004120026));
#55359=CARTESIAN_POINT('Origin',(-50.,0.,0.));
#55360=CARTESIAN_POINT('',(-50.,-7.13209349341826,-0.89072928050049));
#55361=CARTESIAN_POINT('Ctrl Pts',(-50.,-7.13209349341826,-0.89072928050049));
#55362=CARTESIAN_POINT('Ctrl Pts',(-21.,-7.13209349341826,-0.89072928050049));
#55363=CARTESIAN_POINT('Ctrl Pts',(-50.,-7.15577920638447,-0.893054239868308));
#55364=CARTESIAN_POINT('Ctrl Pts',(-21.,-7.15577920638447,-0.893054239868308));
#55365=CARTESIAN_POINT('Ctrl Pts',(-50.,-7.20314083161155,-0.89786893854071));
#55366=CARTESIAN_POINT('Ctrl Pts',(-21.,-7.20314083161155,-0.89786893854071));
#55367=CARTESIAN_POINT('Ctrl Pts',(-50.,-7.27415386726379,-0.90558533966873));
#55368=CARTESIAN_POINT('Ctrl Pts',(-21.,-7.27415386726379,-0.90558533966873));
#55369=CARTESIAN_POINT('Ctrl Pts',(-50.,-7.36877903277666,-0.916863781503486));
#55370=CARTESIAN_POINT('Ctrl Pts',(-21.,-7.36877903277666,-0.916863781503486));
#55371=CARTESIAN_POINT('Ctrl Pts',(-50.,-7.4869674381447,-0.932516236860826));
#55372=CARTESIAN_POINT('Ctrl Pts',(-21.,-7.4869674381447,-0.932516236860826));
#55373=CARTESIAN_POINT('Ctrl Pts',(-50.,-7.60507887157754,-0.949420915891056));
#55374=CARTESIAN_POINT('Ctrl Pts',(-21.,-7.60507887157754,-0.949420915891056));
#55375=CARTESIAN_POINT('Ctrl Pts',(-50.,-7.72314614047142,-0.966965984543332));
#55376=CARTESIAN_POINT('Ctrl Pts',(-21.,-7.72314614047142,-0.966965984543332));
#55377=CARTESIAN_POINT('Ctrl Pts',(-50.,-7.84122460090589,-0.984110042106142));
#55378=CARTESIAN_POINT('Ctrl Pts',(-21.,-7.84122460090589,-0.984110042106142));
#55379=CARTESIAN_POINT('Ctrl Pts',(-50.,-7.95940371279084,-0.999455440216892));
#55380=CARTESIAN_POINT('Ctrl Pts',(-21.,-7.95940371279084,-0.999455440216892));
#55381=CARTESIAN_POINT('Ctrl Pts',(-50.,-8.0778221648407,-1.01133055607812));
#55382=CARTESIAN_POINT('Ctrl Pts',(-21.,-8.0778221648407,-1.01133055607812));
#55383=CARTESIAN_POINT('Ctrl Pts',(-50.,-8.19667636355292,-1.01788199103989));
#55384=CARTESIAN_POINT('Ctrl Pts',(-21.,-8.19667636355292,-1.01788199103989));
#55385=CARTESIAN_POINT('Ctrl Pts',(-50.,-8.31624650623966,-1.017123671327));
#55386=CARTESIAN_POINT('Ctrl Pts',(-21.,-8.31624650623966,-1.017123671327));
#55387=CARTESIAN_POINT('Ctrl Pts',(-50.,-8.43677899171613,-1.00737622330388));
#55388=CARTESIAN_POINT('Ctrl Pts',(-21.,-8.43677899171613,-1.00737622330388));
#55389=CARTESIAN_POINT('Ctrl Pts',(-50.,-8.55832200571467,-0.98784980243911));
#55390=CARTESIAN_POINT('Ctrl Pts',(-21.,-8.55832200571467,-0.98784980243911));
#55391=CARTESIAN_POINT('Ctrl Pts',(-50.,-8.68060673111004,-0.959073494961789));
#55392=CARTESIAN_POINT('Ctrl Pts',(-21.,-8.68060673111004,-0.959073494961789));
#55393=CARTESIAN_POINT('Ctrl Pts',(-50.,-8.80283221651881,-0.923666931425906));
#55394=CARTESIAN_POINT('Ctrl Pts',(-21.,-8.80283221651881,-0.923666931425906));
#55395=CARTESIAN_POINT('Ctrl Pts',(-50.,-8.92394083882956,-0.885365181899303));
#55396=CARTESIAN_POINT('Ctrl Pts',(-21.,-8.92394083882956,-0.885365181899303));
#55397=CARTESIAN_POINT('Ctrl Pts',(-50.,-9.04313782728701,-0.847184879177381));
#55398=CARTESIAN_POINT('Ctrl Pts',(-21.,-9.04313782728701,-0.847184879177381));
#55399=CARTESIAN_POINT('Ctrl Pts',(-50.,-9.1602494406401,-0.810145236641717));
#55400=CARTESIAN_POINT('Ctrl Pts',(-21.,-9.1602494406401,-0.810145236641717));
#55401=CARTESIAN_POINT('Ctrl Pts',(-50.,-9.27634845263042,-0.771090641047726));
#55402=CARTESIAN_POINT('Ctrl Pts',(-21.,-9.27634845263042,-0.771090641047726));
#55403=CARTESIAN_POINT('Ctrl Pts',(-50.,-9.39347368681776,-0.723542272923874));
#55404=CARTESIAN_POINT('Ctrl Pts',(-21.,-9.39347368681776,-0.723542272923874));
#55405=CARTESIAN_POINT('Ctrl Pts',(-50.,-9.51346503399365,-0.66149692044243));
#55406=CARTESIAN_POINT('Ctrl Pts',(-21.,-9.51346503399365,-0.66149692044243));
#55407=CARTESIAN_POINT('Ctrl Pts',(-50.,-9.63711058491003,-0.582194086890198));
#55408=CARTESIAN_POINT('Ctrl Pts',(-21.,-9.63711058491003,-0.582194086890198));
#55409=CARTESIAN_POINT('Ctrl Pts',(-50.,-9.76300600524289,-0.489818901108928));
#55410=CARTESIAN_POINT('Ctrl Pts',(-21.,-9.76300600524289,-0.489818901108928));
#55411=CARTESIAN_POINT('Ctrl Pts',(-50.,-9.88700914008587,-0.397288908358524));
#55412=CARTESIAN_POINT('Ctrl Pts',(-21.,-9.88700914008587,-0.397288908358524));
#55413=CARTESIAN_POINT('Ctrl Pts',(-50.,-10.0034077194239,-0.322542614674783));
#55414=CARTESIAN_POINT('Ctrl Pts',(-21.,-10.0034077194239,-0.322542614674783));
#55415=CARTESIAN_POINT('Ctrl Pts',(-50.,-10.1057999094475,-0.285750111589544));
#55416=CARTESIAN_POINT('Ctrl Pts',(-21.,-10.1057999094475,-0.285750111589544));
#55417=CARTESIAN_POINT('Ctrl Pts',(-50.,-10.1880600728826,-0.306249742693304));
#55418=CARTESIAN_POINT('Ctrl Pts',(-21.,-10.1880600728826,-0.306249742693304));
#55419=CARTESIAN_POINT('Ctrl Pts',(-50.,-10.2453310344199,-0.399403984752717));
#55420=CARTESIAN_POINT('Ctrl Pts',(-21.,-10.2453310344199,-0.399403984752717));
#55421=CARTESIAN_POINT('Ctrl Pts',(-50.,-10.2739254957461,-0.576902635874918));
#55422=CARTESIAN_POINT('Ctrl Pts',(-21.,-10.2739254957461,-0.576902635874918));
#55423=CARTESIAN_POINT('Ctrl Pts',(-50.,-10.2711360438186,-0.847355944984258));
#55424=CARTESIAN_POINT('Ctrl Pts',(-21.,-10.2711360438186,-0.847355944984258));
#55425=CARTESIAN_POINT('Ctrl Pts',(-50.,-10.23508746503,-1.21675444348887));
#55426=CARTESIAN_POINT('Ctrl Pts',(-21.,-10.23508746503,-1.21675444348887));
#55427=CARTESIAN_POINT('Ctrl Pts',(-50.,-10.1645797371964,-1.68895887943845));
#55428=CARTESIAN_POINT('Ctrl Pts',(-21.,-10.1645797371964,-1.68895887943845));
#55429=CARTESIAN_POINT('Ctrl Pts',(-50.,-10.0589430297105,-2.26615269674877));
#55430=CARTESIAN_POINT('Ctrl Pts',(-21.,-10.0589430297105,-2.26615269674877));
#55431=CARTESIAN_POINT('Ctrl Pts',(-50.,-9.91789485710769,-2.94928822483091));
#55432=CARTESIAN_POINT('Ctrl Pts',(-21.,-9.91789485710769,-2.94928822483091));
#55433=CARTESIAN_POINT('Ctrl Pts',(-50.,-9.77670130881801,-3.5806699311609));
#55434=CARTESIAN_POINT('Ctrl Pts',(-21.,-9.77670130881801,-3.5806699311609));
#55435=CARTESIAN_POINT('Ctrl Pts',(-50.,-9.65489431545908,-4.10184205893951));
#55436=CARTESIAN_POINT('Ctrl Pts',(-21.,-9.65489431545908,-4.10184205893951));
#55437=CARTESIAN_POINT('Ctrl Pts',(-50.,-9.56662712803709,-4.47043349004179));
#55438=CARTESIAN_POINT('Ctrl Pts',(-21.,-9.56662712803709,-4.47043349004179));
#55439=CARTESIAN_POINT('Ctrl Pts',(-50.,-9.52072790258051,-4.66001504343333));
#55440=CARTESIAN_POINT('Ctrl Pts',(-21.,-9.52072790258051,-4.66001504343333));
#55441=CARTESIAN_POINT('',(-21.5,-9.99439372247306,-0.334804600014791));
#55442=CARTESIAN_POINT('Ctrl Pts',(-21.5,-9.99439372247306,-0.334804600014791));
#55443=CARTESIAN_POINT('Ctrl Pts',(-21.4716714037528,-9.96555542937999,
-0.349545415954781));
#55444=CARTESIAN_POINT('Ctrl Pts',(-21.4424150110742,-9.9356277416069,-0.367931215781418));
#55445=CARTESIAN_POINT('Ctrl Pts',(-21.2909879716444,-9.78002895717525,
-0.471437247884559));
#55446=CARTESIAN_POINT('Ctrl Pts',(-21.1630186724943,-9.6457529849523,-0.586706241102769));
#55447=CARTESIAN_POINT('Ctrl Pts',(-21.,-9.47570870673866,-0.678928939607902));
#55448=CARTESIAN_POINT('Ctrl Pts',(-50.,-9.99439372247306,-0.334804600014792));
#55449=CARTESIAN_POINT('Ctrl Pts',(-45.1666666666667,-9.99439372247306,
-0.334804600014792));
#55450=CARTESIAN_POINT('Ctrl Pts',(-40.3333333333333,-9.99439372247306,
-0.334804600014792));
#55451=CARTESIAN_POINT('Ctrl Pts',(-30.8333333333333,-9.99439372247306,
-0.334804600014792));
#55452=CARTESIAN_POINT('Ctrl Pts',(-26.1666666666667,-9.99439372247306,
-0.334804600014791));
#55453=CARTESIAN_POINT('Ctrl Pts',(-21.5,-9.99439372247306,-0.334804600014791));
#55454=CARTESIAN_POINT('Origin',(-21.25,0.,0.));
#55455=CARTESIAN_POINT('Origin',(-21.5,0.,0.));
#55456=CARTESIAN_POINT('Origin',(-35.75,0.,0.));
#55457=CARTESIAN_POINT('Ctrl Pts',(-50.,-6.8122671513043,2.29198004120026));
#55458=CARTESIAN_POINT('Ctrl Pts',(-21.,-6.8122671513043,2.29198004120026));
#55459=CARTESIAN_POINT('Ctrl Pts',(-50.,-6.83461600336474,2.30016217089616));
#55460=CARTESIAN_POINT('Ctrl Pts',(-21.,-6.83461600336474,2.30016217089616));
#55461=CARTESIAN_POINT('Ctrl Pts',(-50.,-6.8793763726903,2.31637371632821));
#55462=CARTESIAN_POINT('Ctrl Pts',(-21.,-6.8793763726903,2.31637371632821));
#55463=CARTESIAN_POINT('Ctrl Pts',(-50.,-6.94670492800217,2.34023288057449));
#55464=CARTESIAN_POINT('Ctrl Pts',(-21.,-6.94670492800217,2.34023288057449));
#55465=CARTESIAN_POINT('Ctrl Pts',(-50.,-7.03685278876406,2.37112767623027));
#55466=CARTESIAN_POINT('Ctrl Pts',(-21.,-7.03685278876406,2.37112767623027));
#55467=CARTESIAN_POINT('Ctrl Pts',(-50.,-7.15012820840451,2.4083053284885));
#55468=CARTESIAN_POINT('Ctrl Pts',(-21.,-7.15012820840451,2.4083053284885));
#55469=CARTESIAN_POINT('Ctrl Pts',(-50.,-7.26387759821705,2.44432136933076));
#55470=CARTESIAN_POINT('Ctrl Pts',(-21.,-7.26387759821705,2.44432136933076));
#55471=CARTESIAN_POINT('Ctrl Pts',(-50.,-7.37786505179862,2.47974127678492));
#55472=CARTESIAN_POINT('Ctrl Pts',(-21.,-7.37786505179862,2.47974127678492));
#55473=CARTESIAN_POINT('Ctrl Pts',(-50.,-7.49168859641893,2.51552733857386));
#55474=CARTESIAN_POINT('Ctrl Pts',(-21.,-7.49168859641893,2.51552733857386));
#55475=CARTESIAN_POINT('Ctrl Pts',(-50.,-7.60482241577417,2.55297760756074));
#55476=CARTESIAN_POINT('Ctrl Pts',(-21.,-7.60482241577417,2.55297760756074));
#55477=CARTESIAN_POINT('Ctrl Pts',(-50.,-7.71666617412861,2.59365833862295));
#55478=CARTESIAN_POINT('Ctrl Pts',(-21.,-7.71666617412861,2.59365833862295));
#55479=CARTESIAN_POINT('Ctrl Pts',(-50.,-7.82659266808561,2.63932460382938));
#55480=CARTESIAN_POINT('Ctrl Pts',(-21.,-7.82659266808561,2.63932460382938));
#55481=CARTESIAN_POINT('Ctrl Pts',(-50.,-7.93399262158453,2.69188736687836));
#55482=CARTESIAN_POINT('Ctrl Pts',(-21.,-7.93399262158453,2.69188736687836));
#55483=CARTESIAN_POINT('Ctrl Pts',(-50.,-8.03835937937461,2.75296659957235));
#55484=CARTESIAN_POINT('Ctrl Pts',(-21.,-8.03835937937461,2.75296659957235));
#55485=CARTESIAN_POINT('Ctrl Pts',(-50.,-8.13939365460193,2.82329483425037));
#55486=CARTESIAN_POINT('Ctrl Pts',(-21.,-8.13939365460193,2.82329483425037));
#55487=CARTESIAN_POINT('Ctrl Pts',(-50.,-8.2370828133169,2.90227874531213));
#55488=CARTESIAN_POINT('Ctrl Pts',(-21.,-8.2370828133169,2.90227874531213));
#55489=CARTESIAN_POINT('Ctrl Pts',(-50.,-8.33184183835821,2.98721060740198));
#55490=CARTESIAN_POINT('Ctrl Pts',(-21.,-8.33184183835821,2.98721060740198));
#55491=CARTESIAN_POINT('Ctrl Pts',(-50.,-8.4243384303954,3.07426635319921));
#55492=CARTESIAN_POINT('Ctrl Pts',(-21.,-8.4243384303954,3.07426635319921));
#55493=CARTESIAN_POINT('Ctrl Pts',(-50.,-8.51516539363766,3.16038325236223));
#55494=CARTESIAN_POINT('Ctrl Pts',(-21.,-8.51516539363766,3.16038325236223));
#55495=CARTESIAN_POINT('Ctrl Pts',(-50.,-8.60460841273967,3.24456764186082));
#55496=CARTESIAN_POINT('Ctrl Pts',(-21.,-8.60460841273967,3.24456764186082));
#55497=CARTESIAN_POINT('Ctrl Pts',(-50.,-8.69226485417113,3.33012809006974));
#55498=CARTESIAN_POINT('Ctrl Pts',(-21.,-8.69226485417113,3.33012809006974));
#55499=CARTESIAN_POINT('Ctrl Pts',(-50.,-8.77716058006919,3.42378642402312));
#55500=CARTESIAN_POINT('Ctrl Pts',(-21.,-8.77716058006919,3.42378642402312));
#55501=CARTESIAN_POINT('Ctrl Pts',(-50.,-8.85834857876282,3.53174964938136));
#55502=CARTESIAN_POINT('Ctrl Pts',(-21.,-8.85834857876282,3.53174964938136));
#55503=CARTESIAN_POINT('Ctrl Pts',(-50.,-8.93534116084886,3.65684682750522));
#55504=CARTESIAN_POINT('Ctrl Pts',(-21.,-8.93534116084886,3.65684682750522));
#55505=CARTESIAN_POINT('Ctrl Pts',(-50.,-9.00868892417181,3.79469796977264));
#55506=CARTESIAN_POINT('Ctrl Pts',(-21.,-9.00868892417181,3.79469796977264));
#55507=CARTESIAN_POINT('Ctrl Pts',(-50.,-9.08026462895257,3.93186755639596));
#55508=CARTESIAN_POINT('Ctrl Pts',(-21.,-9.08026462895257,3.93186755639596));
#55509=CARTESIAN_POINT('Ctrl Pts',(-50.,-9.15270492381554,4.04971509082727));
#55510=CARTESIAN_POINT('Ctrl Pts',(-21.,-9.15270492381554,4.04971509082727));
#55511=CARTESIAN_POINT('Ctrl Pts',(-50.,-9.22899343053301,4.12729029694314));
#55512=CARTESIAN_POINT('Ctrl Pts',(-21.,-9.22899343053301,4.12729029694314));
#55513=CARTESIAN_POINT('Ctrl Pts',(-50.,-9.31200173345042,4.1445121148068));
#55514=CARTESIAN_POINT('Ctrl Pts',(-21.,-9.31200173345042,4.1445121148068));
#55515=CARTESIAN_POINT('Ctrl Pts',(-50.,-9.4040191976898,4.08543198173291));
#55516=CARTESIAN_POINT('Ctrl Pts',(-21.,-9.4040191976898,4.08543198173291));
#55517=CARTESIAN_POINT('Ctrl Pts',(-50.,-9.50679569557631,3.93791789477537));
#55518=CARTESIAN_POINT('Ctrl Pts',(-21.,-9.50679569557631,3.93791789477537));
#55519=CARTESIAN_POINT('Ctrl Pts',(-50.,-9.6216277792442,3.69303758521427));
#55520=CARTESIAN_POINT('Ctrl Pts',(-21.,-9.6216277792442,3.69303758521427));
#55521=CARTESIAN_POINT('Ctrl Pts',(-50.,-9.74942513377921,3.34458014605707));
#55522=CARTESIAN_POINT('Ctrl Pts',(-21.,-9.74942513377921,3.34458014605707));
#55523=CARTESIAN_POINT('Ctrl Pts',(-50.,-9.89078169235227,2.88854649339194));
#55524=CARTESIAN_POINT('Ctrl Pts',(-21.,-9.89078169235227,2.88854649339194));
#55525=CARTESIAN_POINT('Ctrl Pts',(-50.,-10.0460413192499,2.32267878361756));
#55526=CARTESIAN_POINT('Ctrl Pts',(-21.,-10.0460413192499,2.32267878361756));
#55527=CARTESIAN_POINT('Ctrl Pts',(-50.,-10.2153627041086,1.64599643173284));
#55528=CARTESIAN_POINT('Ctrl Pts',(-21.,-10.2153627041086,1.64599643173284));
#55529=CARTESIAN_POINT('Ctrl Pts',(-50.,-10.3620979683038,1.01587958589521));
#55530=CARTESIAN_POINT('Ctrl Pts',(-21.,-10.3620979683038,1.01587958589521));
#55531=CARTESIAN_POINT('Ctrl Pts',(-50.,-10.478481770919,0.493469650218983));
#55532=CARTESIAN_POINT('Ctrl Pts',(-21.,-10.478481770919,0.493469650218983));
#55533=CARTESIAN_POINT('Ctrl Pts',(-50.,-10.5588816113278,0.123082548500185));
#55534=CARTESIAN_POINT('Ctrl Pts',(-21.,-10.5588816113278,0.123082548500185));
#55535=CARTESIAN_POINT('Ctrl Pts',(-50.,-10.5997841913839,-0.0676394565978716));
#55536=CARTESIAN_POINT('Ctrl Pts',(-21.,-10.5997841913839,-0.0676394565978716));
#55537=CARTESIAN_POINT('',(-21.5,-9.14990386923578,4.03475639707581));
#55538=CARTESIAN_POINT('Ctrl Pts',(-50.,-9.14990386923578,4.03475639707581));
#55539=CARTESIAN_POINT('Ctrl Pts',(-45.1666666666667,-9.14990386923578,
4.03475639707581));
#55540=CARTESIAN_POINT('Ctrl Pts',(-40.3333333333333,-9.14990386923578,
4.03475639707581));
#55541=CARTESIAN_POINT('Ctrl Pts',(-30.8333333333333,-9.14990386923578,
4.03475639707581));
#55542=CARTESIAN_POINT('Ctrl Pts',(-26.1666666666667,-9.14990386923578,
4.03475639707581));
#55543=CARTESIAN_POINT('Ctrl Pts',(-21.5,-9.14990386923578,4.03475639707581));
#55544=CARTESIAN_POINT('',(-50.,-6.8122671513043,2.29198004120026));
#55545=CARTESIAN_POINT('Ctrl Pts',(-21.5,-9.14990386923578,4.03475639707581));
#55546=CARTESIAN_POINT('Ctrl Pts',(-21.4716714037525,-9.13031726529289,
4.00896291438906));
#55547=CARTESIAN_POINT('Ctrl Pts',(-21.4424150110734,-9.11133064989622,
3.97941274405917));
#55548=CARTESIAN_POINT('Ctrl Pts',(-21.2909879716434,-9.01605057346993,
3.81864524910234));
#55549=CARTESIAN_POINT('Ctrl Pts',(-21.1630186724937,-8.94508544457167,
3.65653131387716));
#55550=CARTESIAN_POINT('Ctrl Pts',(-21.,-8.83189477299562,3.49966208636385));
#55551=CARTESIAN_POINT('Origin',(-50.,0.,0.));
#55552=CARTESIAN_POINT('',(-50.,-7.13209349341826,0.890729280500487));
#55553=CARTESIAN_POINT('Ctrl Pts',(-50.,-10.5997841913839,-0.0676394565978716));
#55554=CARTESIAN_POINT('Ctrl Pts',(-21.,-10.5997841913839,-0.0676394565978716));
#55555=CARTESIAN_POINT('Ctrl Pts',(-50.,-10.5813335008211,-0.0524740444052785));
#55556=CARTESIAN_POINT('Ctrl Pts',(-21.,-10.5813335008211,-0.0524740444052785));
#55557=CARTESIAN_POINT('Ctrl Pts',(-50.,-10.5443614263321,-0.0223524300248229));
#55558=CARTESIAN_POINT('Ctrl Pts',(-21.,-10.5443614263321,-0.0223524300248229));
#55559=CARTESIAN_POINT('Ctrl Pts',(-50.,-10.4886912348662,0.0222023607441701));
#55560=CARTESIAN_POINT('Ctrl Pts',(-21.,-10.4886912348662,0.0222023607441701));
#55561=CARTESIAN_POINT('Ctrl Pts',(-50.,-10.4140395862599,0.0803518244312856));
#55562=CARTESIAN_POINT('Ctrl Pts',(-21.,-10.4140395862599,0.0803518244312856));
#55563=CARTESIAN_POINT('Ctrl Pts',(-50.,-10.3200154257224,0.150928577557961));
#55564=CARTESIAN_POINT('Ctrl Pts',(-21.,-10.3200154257224,0.150928577557961));
#55565=CARTESIAN_POINT('Ctrl Pts',(-50.,-10.2252821497258,0.219366624691659));
#55566=CARTESIAN_POINT('Ctrl Pts',(-21.,-10.2252821497258,0.219366624691659));
#55567=CARTESIAN_POINT('Ctrl Pts',(-50.,-10.1298451744404,0.285621225675486));
#55568=CARTESIAN_POINT('Ctrl Pts',(-21.,-10.1298451744404,0.285621225675486));
#55569=CARTESIAN_POINT('Ctrl Pts',(-50.,-10.0337173245343,0.349629916443316));
#55570=CARTESIAN_POINT('Ctrl Pts',(-21.,-10.0337173245343,0.349629916443316));
#55571=CARTESIAN_POINT('Ctrl Pts',(-50.,-9.93692222450759,0.411308601209035));
#55572=CARTESIAN_POINT('Ctrl Pts',(-21.,-9.93692222450759,0.411308601209035));
#55573=CARTESIAN_POINT('Ctrl Pts',(-50.,-9.83949259364292,0.470562407132083));
#55574=CARTESIAN_POINT('Ctrl Pts',(-21.,-9.83949259364292,0.470562407132083));
#55575=CARTESIAN_POINT('Ctrl Pts',(-50.,-9.74146724538631,0.527299895441832));
#55576=CARTESIAN_POINT('Ctrl Pts',(-21.,-9.74146724538631,0.527299895441832));
#55577=CARTESIAN_POINT('Ctrl Pts',(-50.,-9.64288855622378,0.581447879194613));
#55578=CARTESIAN_POINT('Ctrl Pts',(-21.,-9.64288855622378,0.581447879194613));
#55579=CARTESIAN_POINT('Ctrl Pts',(-50.,-9.54380000381903,0.632963053309265));
#55580=CARTESIAN_POINT('Ctrl Pts',(-21.,-9.54380000381903,0.632963053309265));
#55581=CARTESIAN_POINT('Ctrl Pts',(-50.,-9.44424332627553,0.68185372865074));
#55582=CARTESIAN_POINT('Ctrl Pts',(-21.,-9.44424332627553,0.68185372865074));
#55583=CARTESIAN_POINT('Ctrl Pts',(-50.,-9.34425800352241,0.728158030239756));
#55584=CARTESIAN_POINT('Ctrl Pts',(-21.,-9.34425800352241,0.728158030239756));
#55585=CARTESIAN_POINT('Ctrl Pts',(-50.,-9.24388219451328,0.771898853704203));
#55586=CARTESIAN_POINT('Ctrl Pts',(-21.,-9.24388219451328,0.771898853704203));
#55587=CARTESIAN_POINT('Ctrl Pts',(-50.,-9.14315312384119,0.813043722977555));
#55588=CARTESIAN_POINT('Ctrl Pts',(-21.,-9.14315312384119,0.813043722977555));
#55589=CARTESIAN_POINT('Ctrl Pts',(-50.,-9.04210805084257,0.851468211346448));
#55590=CARTESIAN_POINT('Ctrl Pts',(-21.,-9.04210805084257,0.851468211346448));
#55591=CARTESIAN_POINT('Ctrl Pts',(-50.,-8.94078425956014,0.886903960171005));
#55592=CARTESIAN_POINT('Ctrl Pts',(-21.,-8.94078425956014,0.886903960171005));
#55593=CARTESIAN_POINT('Ctrl Pts',(-50.,-8.83922276353739,0.918952892194649));
#55594=CARTESIAN_POINT('Ctrl Pts',(-21.,-8.83922276353739,0.918952892194649));
#55595=CARTESIAN_POINT('Ctrl Pts',(-50.,-8.73747423363077,0.947150867813171));
#55596=CARTESIAN_POINT('Ctrl Pts',(-21.,-8.73747423363077,0.947150867813171));
#55597=CARTESIAN_POINT('Ctrl Pts',(-50.,-8.63560512714608,0.971017102543951));
#55598=CARTESIAN_POINT('Ctrl Pts',(-21.,-8.63560512714608,0.971017102543951));
#55599=CARTESIAN_POINT('Ctrl Pts',(-50.,-8.53370212161309,0.990109101007577));
#55600=CARTESIAN_POINT('Ctrl Pts',(-21.,-8.53370212161309,0.990109101007577));
#55601=CARTESIAN_POINT('Ctrl Pts',(-50.,-8.43188165539955,1.00407739851957));
#55602=CARTESIAN_POINT('Ctrl Pts',(-21.,-8.43188165539955,1.00407739851957));
#55603=CARTESIAN_POINT('Ctrl Pts',(-50.,-8.33027821569813,1.01271355471894));
#55604=CARTESIAN_POINT('Ctrl Pts',(-21.,-8.33027821569813,1.01271355471894));
#55605=CARTESIAN_POINT('Ctrl Pts',(-50.,-8.2290192302709,1.01599010763451));
#55606=CARTESIAN_POINT('Ctrl Pts',(-21.,-8.2290192302709,1.01599010763451));
#55607=CARTESIAN_POINT('Ctrl Pts',(-50.,-8.12820273854249,1.01410892133532));
#55608=CARTESIAN_POINT('Ctrl Pts',(-21.,-8.12820273854249,1.01410892133532));
#55609=CARTESIAN_POINT('Ctrl Pts',(-50.,-8.02787639670185,1.00753800115478));
#55610=CARTESIAN_POINT('Ctrl Pts',(-21.,-8.02787639670185,1.00753800115478));
#55611=CARTESIAN_POINT('Ctrl Pts',(-50.,-7.92800888935854,0.997080466154163));
#55612=CARTESIAN_POINT('Ctrl Pts',(-21.,-7.92800888935854,0.997080466154163));
#55613=CARTESIAN_POINT('Ctrl Pts',(-50.,-7.82850348500033,0.983785216334555));
#55614=CARTESIAN_POINT('Ctrl Pts',(-21.,-7.82850348500033,0.983785216334555));
#55615=CARTESIAN_POINT('Ctrl Pts',(-50.,-7.7292275500742,0.968799418422935));
#55616=CARTESIAN_POINT('Ctrl Pts',(-21.,-7.7292275500742,0.968799418422935));
#55617=CARTESIAN_POINT('Ctrl Pts',(-50.,-7.63003710778607,0.953237934402831));
#55618=CARTESIAN_POINT('Ctrl Pts',(-21.,-7.63003710778607,0.953237934402831));
#55619=CARTESIAN_POINT('Ctrl Pts',(-50.,-7.53080214904746,0.938052795086852));
#55620=CARTESIAN_POINT('Ctrl Pts',(-21.,-7.53080214904746,0.938052795086852));
#55621=CARTESIAN_POINT('Ctrl Pts',(-50.,-7.43143474677318,0.923884053007731));
#55622=CARTESIAN_POINT('Ctrl Pts',(-21.,-7.43143474677318,0.923884053007731));
#55623=CARTESIAN_POINT('Ctrl Pts',(-50.,-7.33188369780814,0.911105335666499));
#55624=CARTESIAN_POINT('Ctrl Pts',(-21.,-7.33188369780814,0.911105335666499));
#55625=CARTESIAN_POINT('Ctrl Pts',(-50.,-7.25207582250743,0.902140734147994));
#55626=CARTESIAN_POINT('Ctrl Pts',(-21.,-7.25207582250743,0.902140734147994));
#55627=CARTESIAN_POINT('Ctrl Pts',(-50.,-7.19212249719958,0.89615029887462));
#55628=CARTESIAN_POINT('Ctrl Pts',(-21.,-7.19212249719958,0.89615029887462));
#55629=CARTESIAN_POINT('Ctrl Pts',(-50.,-7.15211036864424,0.892482057440589));
#55630=CARTESIAN_POINT('Ctrl Pts',(-21.,-7.15211036864424,0.892482057440589));
#55631=CARTESIAN_POINT('Ctrl Pts',(-50.,-7.13209349341826,0.890729280500492));
#55632=CARTESIAN_POINT('Ctrl Pts',(-21.,-7.13209349341826,0.890729280500492));
#55633=CARTESIAN_POINT('',(-21.5,-9.99295703981581,0.375246053138013));
#55634=CARTESIAN_POINT('Ctrl Pts',(-21.5,-9.99295703981581,0.375246053138014));
#55635=CARTESIAN_POINT('Ctrl Pts',(-26.3333333333333,-9.99295703981581,
0.375246053138014));
#55636=CARTESIAN_POINT('Ctrl Pts',(-31.1666666666667,-9.99295703981581,
0.375246053138014));
#55637=CARTESIAN_POINT('Ctrl Pts',(-40.6666666666667,-9.99295703981581,
0.375246053138014));
#55638=CARTESIAN_POINT('Ctrl Pts',(-45.3333333333333,-9.99295703981581,
0.375246053138014));
#55639=CARTESIAN_POINT('Ctrl Pts',(-50.,-9.99295703981581,0.375246053138014));
#55640=CARTESIAN_POINT('Ctrl Pts',(-21.,-9.47665840807863,0.665541446186863));
#55641=CARTESIAN_POINT('Ctrl Pts',(-21.0648600646508,-9.54397725880582,
0.632805485551036));
#55642=CARTESIAN_POINT('Ctrl Pts',(-21.1289204402943,-9.61037774907841,
0.598586462592499));
#55643=CARTESIAN_POINT('Ctrl Pts',(-21.1924157855611,-9.67606071176893,
0.562824879831496));
#55644=CARTESIAN_POINT('Ctrl Pts',(-21.2961101180201,-9.7833276451402,0.504422591655944));
#55645=CARTESIAN_POINT('Ctrl Pts',(-21.3982975031995,-9.88867999737076,
0.441915547520289));
#55646=CARTESIAN_POINT('Ctrl Pts',(-21.5,-9.99295703981581,0.375246053138013));
#55647=CARTESIAN_POINT('Origin',(-35.75,0.,0.));
#55648=CARTESIAN_POINT('',(-21.5,-8.84053003053573,4.67386657695701));
#55649=CARTESIAN_POINT('Origin',(-21.5,0.,0.));
#55650=CARTESIAN_POINT('Ctrl Pts',(-21.5,-8.84053003053573,4.67386657695702));
#55651=CARTESIAN_POINT('Ctrl Pts',(-26.3333333333333,-8.84053003053573,
4.67386657695702));
#55652=CARTESIAN_POINT('Ctrl Pts',(-31.1666666666667,-8.84053003053573,
4.67386657695702));
#55653=CARTESIAN_POINT('Ctrl Pts',(-40.6666666666667,-8.84053003053573,
4.67386657695702));
#55654=CARTESIAN_POINT('Ctrl Pts',(-45.3333333333333,-8.84053003053573,
4.67386657695702));
#55655=CARTESIAN_POINT('Ctrl Pts',(-50.,-8.84053003053573,4.67386657695702));
#55656=CARTESIAN_POINT('Origin',(-21.25,0.,0.));
#55657=CARTESIAN_POINT('Ctrl Pts',(-21.,-8.24940658621528,4.71140010775012));
#55658=CARTESIAN_POINT('Ctrl Pts',(-21.1171767610998,-8.38464171182995,
4.71088427266307));
#55659=CARTESIAN_POINT('Ctrl Pts',(-21.2874825276465,-8.58376433439286,
4.70484095794187));
#55660=CARTESIAN_POINT('Ctrl Pts',(-21.5,-8.84053003053573,4.67386657695702));
#55661=CARTESIAN_POINT('Ctrl Pts',(-50.,-9.57942322326164,4.53813295416029));
#55662=CARTESIAN_POINT('Ctrl Pts',(-21.,-9.57942322326164,4.53813295416029));
#55663=CARTESIAN_POINT('Ctrl Pts',(-50.,-9.55621969972587,4.54379106380403));
#55664=CARTESIAN_POINT('Ctrl Pts',(-21.,-9.55621969972587,4.54379106380403));
#55665=CARTESIAN_POINT('Ctrl Pts',(-50.,-9.50983973295391,4.55488811868959));
#55666=CARTESIAN_POINT('Ctrl Pts',(-21.,-9.50983973295391,4.55488811868959));
#55667=CARTESIAN_POINT('Ctrl Pts',(-50.,-9.44035102435851,4.57087620725774));
#55668=CARTESIAN_POINT('Ctrl Pts',(-21.,-9.44035102435851,4.57087620725774));
#55669=CARTESIAN_POINT('Ctrl Pts',(-50.,-9.34786210629442,4.59087692729648));
#55670=CARTESIAN_POINT('Ctrl Pts',(-21.,-9.34786210629442,4.59087692729648));
#55671=CARTESIAN_POINT('Ctrl Pts',(-50.,-9.23252715927803,4.61366883031981));
#55672=CARTESIAN_POINT('Ctrl Pts',(-21.,-9.23252715927803,4.61366883031981));
#55673=CARTESIAN_POINT('Ctrl Pts',(-50.,-9.11748127106242,4.63422615215906));
#55674=CARTESIAN_POINT('Ctrl Pts',(-21.,-9.11748127106242,4.63422615215906));
#55675=CARTESIAN_POINT('Ctrl Pts',(-50.,-9.00274873347492,4.65251093331389));
#55676=CARTESIAN_POINT('Ctrl Pts',(-21.,-9.00274873347492,4.65251093331389));
#55677=CARTESIAN_POINT('Ctrl Pts',(-50.,-8.8883682032848,4.66847246002033));
#55678=CARTESIAN_POINT('Ctrl Pts',(-21.,-8.8883682032848,4.66847246002033));
#55679=CARTESIAN_POINT('Ctrl Pts',(-50.,-8.7743974532252,4.68204521487955));
#55680=CARTESIAN_POINT('Ctrl Pts',(-21.,-8.7743974532252,4.68204521487955));
#55681=CARTESIAN_POINT('Ctrl Pts',(-50.,-8.66090712613407,4.69315791678054));
#55682=CARTESIAN_POINT('Ctrl Pts',(-21.,-8.66090712613407,4.69315791678054));
#55683=CARTESIAN_POINT('Ctrl Pts',(-50.,-8.5479718655136,4.70174502276072));
#55684=CARTESIAN_POINT('Ctrl Pts',(-21.,-8.5479718655136,4.70174502276072));
#55685=CARTESIAN_POINT('Ctrl Pts',(-50.,-8.4356616058832,4.70775898013052));
#55686=CARTESIAN_POINT('Ctrl Pts',(-21.,-8.4356616058832,4.70775898013052));
#55687=CARTESIAN_POINT('Ctrl Pts',(-50.,-8.32403430863484,4.71117963661127));
#55688=CARTESIAN_POINT('Ctrl Pts',(-21.,-8.32403430863484,4.71117963661127));
#55689=CARTESIAN_POINT('Ctrl Pts',(-50.,-8.21312397255121,4.71203258951797));
#55690=CARTESIAN_POINT('Ctrl Pts',(-21.,-8.21312397255121,4.71203258951797));
#55691=CARTESIAN_POINT('Ctrl Pts',(-50.,-8.1029496259928,4.71036931800664));
#55692=CARTESIAN_POINT('Ctrl Pts',(-21.,-8.1029496259928,4.71036931800664));
#55693=CARTESIAN_POINT('Ctrl Pts',(-50.,-7.99353571494822,4.70622700687469));
#55694=CARTESIAN_POINT('Ctrl Pts',(-21.,-7.99353571494822,4.70622700687469));
#55695=CARTESIAN_POINT('Ctrl Pts',(-50.,-7.8849298684541,4.69959254734285));
#55696=CARTESIAN_POINT('Ctrl Pts',(-21.,-7.8849298684541,4.69959254734285));
#55697=CARTESIAN_POINT('Ctrl Pts',(-50.,-7.77721964274024,4.69037000103626));
#55698=CARTESIAN_POINT('Ctrl Pts',(-21.,-7.77721964274024,4.69037000103626));
#55699=CARTESIAN_POINT('Ctrl Pts',(-50.,-7.67055506601851,4.67833376211481));
#55700=CARTESIAN_POINT('Ctrl Pts',(-21.,-7.67055506601851,4.67833376211481));
#55701=CARTESIAN_POINT('Ctrl Pts',(-50.,-7.56514580946327,4.66314297047291));
#55702=CARTESIAN_POINT('Ctrl Pts',(-21.,-7.56514580946327,4.66314297047291));
#55703=CARTESIAN_POINT('Ctrl Pts',(-50.,-7.46123890856565,4.64440143603747));
#55704=CARTESIAN_POINT('Ctrl Pts',(-21.,-7.46123890856565,4.64440143603747));
#55705=CARTESIAN_POINT('Ctrl Pts',(-50.,-7.35910284385827,4.62170482170181));
#55706=CARTESIAN_POINT('Ctrl Pts',(-21.,-7.35910284385827,4.62170482170181));
#55707=CARTESIAN_POINT('Ctrl Pts',(-50.,-7.25900770064673,4.59469206087561));
#55708=CARTESIAN_POINT('Ctrl Pts',(-21.,-7.25900770064673,4.59469206087561));
#55709=CARTESIAN_POINT('Ctrl Pts',(-50.,-7.16121001331941,4.56309881747208));
#55710=CARTESIAN_POINT('Ctrl Pts',(-21.,-7.16121001331941,4.56309881747208));
#55711=CARTESIAN_POINT('Ctrl Pts',(-50.,-7.06592138953324,4.5267956450212));
#55712=CARTESIAN_POINT('Ctrl Pts',(-21.,-7.06592138953324,4.5267956450212));
#55713=CARTESIAN_POINT('Ctrl Pts',(-50.,-6.9732685530375,4.48581308997575));
#55714=CARTESIAN_POINT('Ctrl Pts',(-21.,-6.9732685530375,4.48581308997575));
#55715=CARTESIAN_POINT('Ctrl Pts',(-50.,-6.88325224876452,4.44037556328962));
#55716=CARTESIAN_POINT('Ctrl Pts',(-21.,-6.88325224876452,4.44037556328962));
#55717=CARTESIAN_POINT('Ctrl Pts',(-50.,-6.79571235355295,4.39092540044367));
#55718=CARTESIAN_POINT('Ctrl Pts',(-21.,-6.79571235355295,4.39092540044367));
#55719=CARTESIAN_POINT('Ctrl Pts',(-50.,-6.71027219290964,4.33817259947066));
#55720=CARTESIAN_POINT('Ctrl Pts',(-21.,-6.71027219290964,4.33817259947066));
#55721=CARTESIAN_POINT('Ctrl Pts',(-50.,-6.62638951409907,4.28302021638686));
#55722=CARTESIAN_POINT('Ctrl Pts',(-21.,-6.62638951409907,4.28302021638686));
#55723=CARTESIAN_POINT('Ctrl Pts',(-50.,-6.54344708143028,4.22644426515767));
#55724=CARTESIAN_POINT('Ctrl Pts',(-21.,-6.54344708143028,4.22644426515767));
#55725=CARTESIAN_POINT('Ctrl Pts',(-50.,-6.46083145580807,4.1693867325325));
#55726=CARTESIAN_POINT('Ctrl Pts',(-21.,-6.46083145580807,4.1693867325325));
#55727=CARTESIAN_POINT('Ctrl Pts',(-50.,-6.37801243240243,4.11264895980536));
#55728=CARTESIAN_POINT('Ctrl Pts',(-21.,-6.37801243240243,4.11264895980536));
#55729=CARTESIAN_POINT('Ctrl Pts',(-50.,-6.29463308326085,4.05676946424956));
#55730=CARTESIAN_POINT('Ctrl Pts',(-21.,-6.29463308326085,4.05676946424956));
#55731=CARTESIAN_POINT('Ctrl Pts',(-50.,-6.21048516503746,4.00206265639536));
#55732=CARTESIAN_POINT('Ctrl Pts',(-21.,-6.21048516503746,4.00206265639536));
#55733=CARTESIAN_POINT('Ctrl Pts',(-50.,-6.14247034880463,3.95935849016754));
#55734=CARTESIAN_POINT('Ctrl Pts',(-21.,-6.14247034880463,3.95935849016754));
#55735=CARTESIAN_POINT('Ctrl Pts',(-50.,-6.09105342163039,3.92794852152394));
#55736=CARTESIAN_POINT('Ctrl Pts',(-21.,-6.09105342163039,3.92794852152394));
#55737=CARTESIAN_POINT('Ctrl Pts',(-50.,-6.0565953297729,3.90728293824429));
#55738=CARTESIAN_POINT('Ctrl Pts',(-21.,-6.0565953297729,3.90728293824429));
#55739=CARTESIAN_POINT('Ctrl Pts',(-50.,-6.03932124977421,3.89701874412039));
#55740=CARTESIAN_POINT('Ctrl Pts',(-21.,-6.03932124977421,3.89701874412039));
#55741=CARTESIAN_POINT('',(-50.,-6.03932124977422,3.89701874412038));
#55742=CARTESIAN_POINT('Origin',(-50.,0.,0.));
#55743=CARTESIAN_POINT('',(-50.,-5.14318775290069,5.02073460645076));
#55744=CARTESIAN_POINT('Ctrl Pts',(-50.,-5.14318775290069,5.02073460645076));
#55745=CARTESIAN_POINT('Ctrl Pts',(-21.,-5.14318775290069,5.02073460645076));
#55746=CARTESIAN_POINT('Ctrl Pts',(-50.,-5.1597732798141,5.03780325407688));
#55747=CARTESIAN_POINT('Ctrl Pts',(-21.,-5.1597732798141,5.03780325407688));
#55748=CARTESIAN_POINT('Ctrl Pts',(-50.,-5.19306705314332,5.071830148219));
#55749=CARTESIAN_POINT('Ctrl Pts',(-21.,-5.19306705314332,5.071830148219));
#55750=CARTESIAN_POINT('Ctrl Pts',(-50.,-5.24337588200476,5.12253927774717));
#55751=CARTESIAN_POINT('Ctrl Pts',(-21.,-5.24337588200476,5.12253927774717));
#55752=CARTESIAN_POINT('Ctrl Pts',(-50.,-5.31119154860082,5.18948821771405));
#55753=CARTESIAN_POINT('Ctrl Pts',(-21.,-5.31119154860082,5.18948821771405));
#55754=CARTESIAN_POINT('Ctrl Pts',(-50.,-5.39711839642203,5.27213248760413));
#55755=CARTESIAN_POINT('Ctrl Pts',(-21.,-5.39711839642203,5.27213248760413));
#55756=CARTESIAN_POINT('Ctrl Pts',(-50.,-5.48397628091718,5.35393582972231));
#55757=CARTESIAN_POINT('Ctrl Pts',(-21.,-5.48397628091718,5.35393582972231));
#55758=CARTESIAN_POINT('Ctrl Pts',(-50.,-5.57130730604024,5.43530536621495));
#55759=CARTESIAN_POINT('Ctrl Pts',(-21.,-5.57130730604024,5.43530536621495));
#55760=CARTESIAN_POINT('Ctrl Pts',(-50.,-5.65833178588016,5.51693367893109));
#55761=CARTESIAN_POINT('Ctrl Pts',(-21.,-5.65833178588016,5.51693367893109));
#55762=CARTESIAN_POINT('Ctrl Pts',(-50.,-5.74401277228714,5.59976212994534));
#55763=CARTESIAN_POINT('Ctrl Pts',(-21.,-5.74401277228714,5.59976212994534));
#55764=CARTESIAN_POINT('Ctrl Pts',(-50.,-5.82712980893039,5.68494139022769));
#55765=CARTESIAN_POINT('Ctrl Pts',(-21.,-5.82712980893039,5.68494139022769));
#55766=CARTESIAN_POINT('Ctrl Pts',(-50.,-5.906356307844,5.77378059171821));
#55767=CARTESIAN_POINT('Ctrl Pts',(-21.,-5.906356307844,5.77378059171821));
#55768=CARTESIAN_POINT('Ctrl Pts',(-50.,-5.98031419419066,5.86773709824143));
#55769=CARTESIAN_POINT('Ctrl Pts',(-21.,-5.98031419419066,5.86773709824143));
#55770=CARTESIAN_POINT('Ctrl Pts',(-50.,-6.04784410793973,5.96805062448362));
#55771=CARTESIAN_POINT('Ctrl Pts',(-21.,-6.04784410793973,5.96805062448362));
#55772=CARTESIAN_POINT('Ctrl Pts',(-50.,-6.108358567083,6.07525130357771));
#55773=CARTESIAN_POINT('Ctrl Pts',(-21.,-6.108358567083,6.07525130357771));
#55774=CARTESIAN_POINT('Ctrl Pts',(-50.,-6.16210362315516,6.18879908596403));
#55775=CARTESIAN_POINT('Ctrl Pts',(-21.,-6.16210362315516,6.18879908596403));
#55776=CARTESIAN_POINT('Ctrl Pts',(-50.,-6.2106280007764,6.30643444970003));
#55777=CARTESIAN_POINT('Ctrl Pts',(-21.,-6.2106280007764,6.30643444970003));
#55778=CARTESIAN_POINT('Ctrl Pts',(-50.,-6.25619247809081,6.42500173364409));
#55779=CARTESIAN_POINT('Ctrl Pts',(-21.,-6.25619247809081,6.42500173364409));
#55780=CARTESIAN_POINT('Ctrl Pts',(-50.,-6.30066002212815,6.5419987212145));
#55781=CARTESIAN_POINT('Ctrl Pts',(-21.,-6.30066002212815,6.5419987212145));
#55782=CARTESIAN_POINT('Ctrl Pts',(-50.,-6.34471916009928,6.65665410688205));
#55783=CARTESIAN_POINT('Ctrl Pts',(-21.,-6.34471916009928,6.65665410688205));
#55784=CARTESIAN_POINT('Ctrl Pts',(-50.,-6.38657159771068,6.77177411160809));
#55785=CARTESIAN_POINT('Ctrl Pts',(-21.,-6.38657159771068,6.77177411160809));
#55786=CARTESIAN_POINT('Ctrl Pts',(-50.,-6.42242317562759,6.89299222970744));
#55787=CARTESIAN_POINT('Ctrl Pts',(-21.,-6.42242317562759,6.89299222970744));
#55788=CARTESIAN_POINT('Ctrl Pts',(-50.,-6.44872754699223,7.02548988707821));
#55789=CARTESIAN_POINT('Ctrl Pts',(-21.,-6.44872754699223,7.02548988707821));
#55790=CARTESIAN_POINT('Ctrl Pts',(-50.,-6.46381783511374,7.17160437943005));
#55791=CARTESIAN_POINT('Ctrl Pts',(-21.,-6.46381783511374,7.17160437943005));
#55792=CARTESIAN_POINT('Ctrl Pts',(-50.,-6.47009051734937,7.32762836882426));
#55793=CARTESIAN_POINT('Ctrl Pts',(-21.,-6.47009051734937,7.32762836882426));
#55794=CARTESIAN_POINT('Ctrl Pts',(-50.,-6.47506234591768,7.48226943041517));
#55795=CARTESIAN_POINT('Ctrl Pts',(-21.,-6.47506234591768,7.48226943041517));
#55796=CARTESIAN_POINT('Ctrl Pts',(-50.,-6.48919666748604,7.61987705609476));
#55797=CARTESIAN_POINT('Ctrl Pts',(-21.,-6.48919666748604,7.61987705609476));
#55798=CARTESIAN_POINT('Ctrl Pts',(-50.,-6.52427161652488,7.72287024427254));
#55799=CARTESIAN_POINT('Ctrl Pts',(-21.,-6.52427161652488,7.72287024427254));
#55800=CARTESIAN_POINT('Ctrl Pts',(-50.,-6.59158724650179,7.774402518864));
#55801=CARTESIAN_POINT('Ctrl Pts',(-21.,-6.59158724650179,7.774402518864));
#55802=CARTESIAN_POINT('Ctrl Pts',(-50.,-6.70012602613047,7.76109803970118));
#55803=CARTESIAN_POINT('Ctrl Pts',(-21.,-6.70012602613047,7.76109803970118));
#55804=CARTESIAN_POINT('Ctrl Pts',(-50.,-6.8567284146999,7.67278549097179));
#55805=CARTESIAN_POINT('Ctrl Pts',(-21.,-6.8567284146999,7.67278549097179));
#55806=CARTESIAN_POINT('Ctrl Pts',(-50.,-7.06643813146967,7.50197972952742));
#55807=CARTESIAN_POINT('Ctrl Pts',(-21.,-7.06643813146967,7.50197972952742));
#55808=CARTESIAN_POINT('Ctrl Pts',(-50.,-7.33276958593085,7.24347961909277));
#55809=CARTESIAN_POINT('Ctrl Pts',(-21.,-7.33276958593085,7.24347961909277));
#55810=CARTESIAN_POINT('Ctrl Pts',(-50.,-7.65799303086079,6.89393980750813));
#55811=CARTESIAN_POINT('Ctrl Pts',(-21.,-7.65799303086079,6.89393980750813));
#55812=CARTESIAN_POINT('Ctrl Pts',(-50.,-8.04339791890053,6.45147524510253));
#55813=CARTESIAN_POINT('Ctrl Pts',(-21.,-8.04339791890053,6.45147524510253));
#55814=CARTESIAN_POINT('Ctrl Pts',(-50.,-8.48955268435888,5.91527130817043));
#55815=CARTESIAN_POINT('Ctrl Pts',(-21.,-8.48955268435888,5.91527130817043));
#55816=CARTESIAN_POINT('Ctrl Pts',(-50.,-8.89515404237518,5.41122169201928));
#55817=CARTESIAN_POINT('Ctrl Pts',(-21.,-8.89515404237518,5.41122169201928));
#55818=CARTESIAN_POINT('Ctrl Pts',(-50.,-9.22667740150299,4.99104364314351));
#55819=CARTESIAN_POINT('Ctrl Pts',(-21.,-9.22667740150299,4.99104364314351));
#55820=CARTESIAN_POINT('Ctrl Pts',(-50.,-9.45982009531033,4.6922205788033));
#55821=CARTESIAN_POINT('Ctrl Pts',(-21.,-9.45982009531033,4.6922205788033));
#55822=CARTESIAN_POINT('Ctrl Pts',(-50.,-9.57942322326164,4.53813295416029));
#55823=CARTESIAN_POINT('Ctrl Pts',(-21.,-9.57942322326164,4.53813295416029));
#55824=CARTESIAN_POINT('',(-21.5,-6.49316333848958,7.60518440668567));
#55825=CARTESIAN_POINT('Ctrl Pts',(-21.5,-6.49316333848958,7.60518440668567));
#55826=CARTESIAN_POINT('Ctrl Pts',(-21.471671403753,-6.48670779082223,7.57344697283542));
#55827=CARTESIAN_POINT('Ctrl Pts',(-21.4424150110746,-6.48242277983734,
7.5385852056463));
#55828=CARTESIAN_POINT('Ctrl Pts',(-21.290987971645,-6.46633279908609,7.35239822189698));
#55829=CARTESIAN_POINT('Ctrl Pts',(-21.1630186724948,-6.47273402762092,
7.17554799773173));
#55830=CARTESIAN_POINT('Ctrl Pts',(-21.,-6.43881576337966,6.98510211559241));
#55831=CARTESIAN_POINT('Ctrl Pts',(-50.,-6.49316333848958,7.60518440668567));
#55832=CARTESIAN_POINT('Ctrl Pts',(-45.1666666666667,-6.49316333848958,
7.60518440668567));
#55833=CARTESIAN_POINT('Ctrl Pts',(-40.3333333333333,-6.49316333848958,
7.60518440668567));
#55834=CARTESIAN_POINT('Ctrl Pts',(-30.8333333333333,-6.49316333848958,
7.60518440668567));
#55835=CARTESIAN_POINT('Ctrl Pts',(-26.1666666666667,-6.49316333848958,
7.60518440668567));
#55836=CARTESIAN_POINT('Ctrl Pts',(-21.5,-6.49316333848958,7.60518440668567));
#55837=CARTESIAN_POINT('Origin',(-21.25,0.,0.));
#55838=CARTESIAN_POINT('Origin',(-21.5,0.,0.));
#55839=CARTESIAN_POINT('Origin',(-35.75,0.,0.));
#55840=CARTESIAN_POINT('Ctrl Pts',(-50.,-2.45543694297674,6.75507110762463));
#55841=CARTESIAN_POINT('Ctrl Pts',(-21.,-2.45543694297674,6.75507110762463));
#55842=CARTESIAN_POINT('Ctrl Pts',(-50.,-2.46297417772978,6.77764561818537));
#55843=CARTESIAN_POINT('Ctrl Pts',(-21.,-2.46297417772978,6.77764561818537));
#55844=CARTESIAN_POINT('Ctrl Pts',(-50.,-2.47820711493347,6.82274841734025));
#55845=CARTESIAN_POINT('Ctrl Pts',(-21.,-2.47820711493347,6.82274841734025));
#55846=CARTESIAN_POINT('Ctrl Pts',(-50.,-2.50153193679118,6.89026394714059));
#55847=CARTESIAN_POINT('Ctrl Pts',(-21.,-2.50153193679118,6.89026394714059));
#55848=CARTESIAN_POINT('Ctrl Pts',(-50.,-2.53358368474749,6.98000697278327));
#55849=CARTESIAN_POINT('Ctrl Pts',(-21.,-2.53358368474749,6.98000697278327));
#55850=CARTESIAN_POINT('Ctrl Pts',(-50.,-2.57514309471485,7.09174914908801));
#55851=CARTESIAN_POINT('Ctrl Pts',(-21.,-2.57514309471485,7.09174914908801));
#55852=CARTESIAN_POINT('Ctrl Pts',(-50.,-2.61790620462629,7.20313763732345));
#55853=CARTESIAN_POINT('Ctrl Pts',(-21.,-2.61790620462629,7.20313763732345));
#55854=CARTESIAN_POINT('Ctrl Pts',(-50.,-2.66128382072048,7.31434056822034));
#55855=CARTESIAN_POINT('Ctrl Pts',(-21.,-2.66128382072048,7.31434056822034));
#55856=CARTESIAN_POINT('Ctrl Pts',(-50.,-2.70427297026251,7.42564364342468));
#55857=CARTESIAN_POINT('Ctrl Pts',(-21.,-2.70427297026251,7.42564364342468));
#55858=CARTESIAN_POINT('Ctrl Pts',(-50.,-2.74553095355499,7.53744508591865));
#55859=CARTESIAN_POINT('Ctrl Pts',(-21.,-2.74553095355499,7.53744508591865));
#55860=CARTESIAN_POINT('Ctrl Pts',(-50.,-2.78345892001629,7.65025207826714));
#55861=CARTESIAN_POINT('Ctrl Pts',(-21.,-2.78345892001629,7.65025207826714));
#55862=CARTESIAN_POINT('Ctrl Pts',(-50.,-2.81629364412744,7.76466852264525));
#55863=CARTESIAN_POINT('Ctrl Pts',(-21.,-2.81629364412744,7.76466852264525));
#55864=CARTESIAN_POINT('Ctrl Pts',(-50.,-2.84216119689693,7.88140953422486));
#55865=CARTESIAN_POINT('Ctrl Pts',(-21.,-2.84216119689693,7.88140953422486));
#55866=CARTESIAN_POINT('Ctrl Pts',(-50.,-2.85947913898695,8.00108902987832));
#55867=CARTESIAN_POINT('Ctrl Pts',(-21.,-2.85947913898695,8.00108902987832));
#55868=CARTESIAN_POINT('Ctrl Pts',(-50.,-2.86748815125169,8.12392974416385));
#55869=CARTESIAN_POINT('Ctrl Pts',(-21.,-2.86748815125169,8.12392974416385));
#55870=CARTESIAN_POINT('Ctrl Pts',(-50.,-2.8666442371861,8.24955186700095));
#55871=CARTESIAN_POINT('Ctrl Pts',(-21.,-2.8666442371861,8.24955186700095));
#55872=CARTESIAN_POINT('Ctrl Pts',(-50.,-2.85932311928695,8.37659160589212));
#55873=CARTESIAN_POINT('Ctrl Pts',(-21.,-2.85932311928695,8.37659160589212));
#55874=CARTESIAN_POINT('Ctrl Pts',(-50.,-2.84893087833482,8.50318672326558));
#55875=CARTESIAN_POINT('Ctrl Pts',(-21.,-2.84893087833482,8.50318672326558));
#55876=CARTESIAN_POINT('Ctrl Pts',(-50.,-2.838231660712,8.62789111098118));
#55877=CARTESIAN_POINT('Ctrl Pts',(-21.,-2.838231660712,8.62789111098118));
#55878=CARTESIAN_POINT('Ctrl Pts',(-50.,-2.8281804649272,8.7503085875302));
#55879=CARTESIAN_POINT('Ctrl Pts',(-21.,-2.8281804649272,8.7503085875302));
#55880=CARTESIAN_POINT('Ctrl Pts',(-50.,-2.81593951016314,8.87218721998315));
#55881=CARTESIAN_POINT('Ctrl Pts',(-21.,-2.81593951016314,8.87218721998315));
#55882=CARTESIAN_POINT('Ctrl Pts',(-50.,-2.79564609540172,8.99695638729624));
#55883=CARTESIAN_POINT('Ctrl Pts',(-21.,-2.79564609540172,8.99695638729624));
#55884=CARTESIAN_POINT('Ctrl Pts',(-50.,-2.76185693608665,9.12774569066013));
#55885=CARTESIAN_POINT('Ctrl Pts',(-21.,-2.76185693608665,9.12774569066013));
#55886=CARTESIAN_POINT('Ctrl Pts',(-50.,-2.71205611361093,9.26593773005304));
#55887=CARTESIAN_POINT('Ctrl Pts',(-21.,-2.71205611361093,9.26593773005304));
#55888=CARTESIAN_POINT('Ctrl Pts',(-50.,-2.65001133311308,9.40923210196585));
#55889=CARTESIAN_POINT('Ctrl Pts',(-21.,-2.65001133311308,9.40923210196585));
#55890=CARTESIAN_POINT('Ctrl Pts',(-50.,-2.5873945538455,9.5507160797281));
#55891=CARTESIAN_POINT('Ctrl Pts',(-21.,-2.5873945538455,9.5507160797281));
#55892=CARTESIAN_POINT('Ctrl Pts',(-50.,-2.54042342638657,9.68082891874335));
#55893=CARTESIAN_POINT('Ctrl Pts',(-21.,-2.54042342638657,9.68082891874335));
#55894=CARTESIAN_POINT('Ctrl Pts',(-50.,-2.52733779392361,9.78884102493588));
#55895=CARTESIAN_POINT('Ctrl Pts',(-21.,-2.52733779392361,9.78884102493588));
#55896=CARTESIAN_POINT('Ctrl Pts',(-50.,-2.56562806487107,9.86447715727042));
#55897=CARTESIAN_POINT('Ctrl Pts',(-21.,-2.56562806487107,9.86447715727042));
#55898=CARTESIAN_POINT('Ctrl Pts',(-50.,-2.6691907234428,9.89958344728561));
#55899=CARTESIAN_POINT('Ctrl Pts',(-21.,-2.6691907234428,9.89958344728561));
#55900=CARTESIAN_POINT('Ctrl Pts',(-50.,-2.84860197903673,9.88796382014256));
#55901=CARTESIAN_POINT('Ctrl Pts',(-21.,-2.84860197903673,9.88796382014256));
#55902=CARTESIAN_POINT('Ctrl Pts',(-50.,-3.11165374758123,9.82506278266417));
#55903=CARTESIAN_POINT('Ctrl Pts',(-21.,-3.11165374758123,9.82506278266417));
#55904=CARTESIAN_POINT('Ctrl Pts',(-50.,-3.46376909107161,9.70771911811945));
#55905=CARTESIAN_POINT('Ctrl Pts',(-21.,-3.46376909107161,9.70771911811945));
#55906=CARTESIAN_POINT('Ctrl Pts',(-50.,-3.90844493048625,9.5339037941241));
#55907=CARTESIAN_POINT('Ctrl Pts',(-21.,-3.90844493048625,9.5339037941241));
#55908=CARTESIAN_POINT('Ctrl Pts',(-50.,-4.44766091491103,9.30247791214345));
#55909=CARTESIAN_POINT('Ctrl Pts',(-21.,-4.44766091491103,9.30247791214345));
#55910=CARTESIAN_POINT('Ctrl Pts',(-50.,-5.08228263794097,9.01295415598311));
#55911=CARTESIAN_POINT('Ctrl Pts',(-21.,-5.08228263794097,9.01295415598311));
#55912=CARTESIAN_POINT('Ctrl Pts',(-50.,-5.66641576644903,8.73480497776003));
#55913=CARTESIAN_POINT('Ctrl Pts',(-21.,-5.66641576644903,8.73480497776003));
#55914=CARTESIAN_POINT('Ctrl Pts',(-50.,-6.14741641494695,8.50008023141016));
#55915=CARTESIAN_POINT('Ctrl Pts',(-21.,-6.14741641494695,8.50008023141016));
#55916=CARTESIAN_POINT('Ctrl Pts',(-50.,-6.48712519233678,8.33200677716551));
#55917=CARTESIAN_POINT('Ctrl Pts',(-21.,-6.48712519233678,8.33200677716551));
#55918=CARTESIAN_POINT('Ctrl Pts',(-50.,-6.6617400018565,8.24507247679879));
#55919=CARTESIAN_POINT('Ctrl Pts',(-21.,-6.6617400018565,8.24507247679879));
#55920=CARTESIAN_POINT('',(-21.5,-2.55037217513312,9.66931237308562));
#55921=CARTESIAN_POINT('Ctrl Pts',(-50.,-2.55037217513312,9.66931237308562));
#55922=CARTESIAN_POINT('Ctrl Pts',(-45.1666666666667,-2.55037217513312,
9.66931237308562));
#55923=CARTESIAN_POINT('Ctrl Pts',(-40.3333333333333,-2.55037217513312,
9.66931237308562));
#55924=CARTESIAN_POINT('Ctrl Pts',(-30.8333333333333,-2.55037217513312,
9.66931237308562));
#55925=CARTESIAN_POINT('Ctrl Pts',(-26.1666666666667,-2.55037217513312,
9.66931237308562));
#55926=CARTESIAN_POINT('Ctrl Pts',(-21.5,-2.55037217513312,9.66931237308562));
#55927=CARTESIAN_POINT('',(-50.,-2.45543694297674,6.75507110762463));
#55928=CARTESIAN_POINT('Ctrl Pts',(-21.5,-2.55037217513312,9.66931237308562));
#55929=CARTESIAN_POINT('Ctrl Pts',(-21.471671403753,-2.55832628412853,9.63791697607945));
#55930=CARTESIAN_POINT('Ctrl Pts',(-21.4424150110746,-2.56959157653279,
9.60464841257371));
#55931=CARTESIAN_POINT('Ctrl Pts',(-21.2909879716447,-2.63587850947504,
9.42991855559593));
#55932=CARTESIAN_POINT('Ctrl Pts',(-21.1630186724946,-2.71837825362579,
9.27335939831321));
#55933=CARTESIAN_POINT('Ctrl Pts',(-21.,-2.77045032493322,9.08705700417233));
#55934=CARTESIAN_POINT('Origin',(-50.,0.,0.));
#55935=CARTESIAN_POINT('',(-50.,-3.75038736519794,6.13145585166881));
#55936=CARTESIAN_POINT('Ctrl Pts',(-50.,-6.6617400018565,8.24507247679879));
#55937=CARTESIAN_POINT('Ctrl Pts',(-21.,-6.6617400018565,8.24507247679879));
#55938=CARTESIAN_POINT('Ctrl Pts',(-50.,-6.63837938775657,8.24010262588657));
#55939=CARTESIAN_POINT('Ctrl Pts',(-21.,-6.63837938775657,8.24010262588657));
#55940=CARTESIAN_POINT('Ctrl Pts',(-50.,-6.59177764993375,8.2299772134607));
#55941=CARTESIAN_POINT('Ctrl Pts',(-21.,-6.59177764993375,8.2299772134607));
#55942=CARTESIAN_POINT('Ctrl Pts',(-50.,-6.52223351516926,8.21423196280605));
#55943=CARTESIAN_POINT('Ctrl Pts',(-21.,-6.52223351516926,8.21423196280605));
#55944=CARTESIAN_POINT('Ctrl Pts',(-50.,-6.43022589217209,8.1921225513));
#55945=CARTESIAN_POINT('Ctrl Pts',(-21.,-6.43022589217209,8.1921225513));
#55946=CARTESIAN_POINT('Ctrl Pts',(-50.,-6.31642365942377,8.16261538830187));
#55947=CARTESIAN_POINT('Ctrl Pts',(-21.,-6.31642365942377,8.16261538830187));
#55948=CARTESIAN_POINT('Ctrl Pts',(-50.,-6.20385140809547,8.1312203551374));
#55949=CARTESIAN_POINT('Ctrl Pts',(-21.,-6.20385140809547,8.1312203551374));
#55950=CARTESIAN_POINT('Ctrl Pts',(-50.,-6.09254749437728,8.0979137913074));
#55951=CARTESIAN_POINT('Ctrl Pts',(-21.,-6.09254749437728,8.0979137913074));
#55952=CARTESIAN_POINT('Ctrl Pts',(-50.,-5.9825687506924,8.06266677783295));
#55953=CARTESIAN_POINT('Ctrl Pts',(-21.,-5.9825687506924,8.06266677783295));
#55954=CARTESIAN_POINT('Ctrl Pts',(-50.,-5.87399565540877,8.02544535222689));
#55955=CARTESIAN_POINT('Ctrl Pts',(-21.,-5.87399565540877,8.02544535222689));
#55956=CARTESIAN_POINT('Ctrl Pts',(-50.,-5.7669227832391,7.98621594320599));
#55957=CARTESIAN_POINT('Ctrl Pts',(-21.,-5.7669227832391,7.98621594320599));
#55958=CARTESIAN_POINT('Ctrl Pts',(-50.,-5.66144582368073,7.94495188520329));
#55959=CARTESIAN_POINT('Ctrl Pts',(-21.,-5.66144582368073,7.94495188520329));
#55960=CARTESIAN_POINT('Ctrl Pts',(-50.,-5.5576484178972,7.90164067817667));
#55961=CARTESIAN_POINT('Ctrl Pts',(-21.,-5.5576484178972,7.90164067817667));
#55962=CARTESIAN_POINT('Ctrl Pts',(-50.,-5.45559153104423,7.85628931405591));
#55963=CARTESIAN_POINT('Ctrl Pts',(-21.,-5.45559153104423,7.85628931405591));
#55964=CARTESIAN_POINT('Ctrl Pts',(-50.,-5.35529468870783,7.80893560674388));
#55965=CARTESIAN_POINT('Ctrl Pts',(-21.,-5.35529468870783,7.80893560674388));
#55966=CARTESIAN_POINT('Ctrl Pts',(-50.,-5.25675269887972,7.75963419345371));
#55967=CARTESIAN_POINT('Ctrl Pts',(-21.,-5.25675269887972,7.75963419345371));
#55968=CARTESIAN_POINT('Ctrl Pts',(-50.,-5.15997145275563,7.70842918324715));
#55969=CARTESIAN_POINT('Ctrl Pts',(-21.,-5.15997145275563,7.70842918324715));
#55970=CARTESIAN_POINT('Ctrl Pts',(-50.,-5.06499955030094,7.65532943098672));
#55971=CARTESIAN_POINT('Ctrl Pts',(-21.,-5.06499955030094,7.65532943098672));
#55972=CARTESIAN_POINT('Ctrl Pts',(-50.,-4.9719575030537,7.60028648840776));
#55973=CARTESIAN_POINT('Ctrl Pts',(-21.,-4.9719575030537,7.60028648840776));
#55974=CARTESIAN_POINT('Ctrl Pts',(-50.,-4.88107836846757,7.54316218647348));
#55975=CARTESIAN_POINT('Ctrl Pts',(-21.,-4.88107836846757,7.54316218647348));
#55976=CARTESIAN_POINT('Ctrl Pts',(-50.,-4.79269894740031,7.48374039375355));
#55977=CARTESIAN_POINT('Ctrl Pts',(-21.,-4.79269894740031,7.48374039375355));
#55978=CARTESIAN_POINT('Ctrl Pts',(-50.,-4.70721371156899,7.42177134000892));
#55979=CARTESIAN_POINT('Ctrl Pts',(-21.,-4.70721371156899,7.42177134000892));
#55980=CARTESIAN_POINT('Ctrl Pts',(-50.,-4.62503998887083,7.35700721943171));
#55981=CARTESIAN_POINT('Ctrl Pts',(-21.,-4.62503998887083,7.35700721943171));
#55982=CARTESIAN_POINT('Ctrl Pts',(-50.,-4.54657777868016,7.28923990788708));
#55983=CARTESIAN_POINT('Ctrl Pts',(-21.,-4.54657777868016,7.28923990788708));
#55984=CARTESIAN_POINT('Ctrl Pts',(-50.,-4.47217290162416,7.21834255288981));
#55985=CARTESIAN_POINT('Ctrl Pts',(-21.,-4.47217290162416,7.21834255288981));
#55986=CARTESIAN_POINT('Ctrl Pts',(-50.,-4.40207217433237,7.14429034032177));
#55987=CARTESIAN_POINT('Ctrl Pts',(-21.,-4.40207217433237,7.14429034032177));
#55988=CARTESIAN_POINT('Ctrl Pts',(-50.,-4.33637651734857,7.06716577496009));
#55989=CARTESIAN_POINT('Ctrl Pts',(-21.,-4.33637651734857,7.06716577496009));
#55990=CARTESIAN_POINT('Ctrl Pts',(-50.,-4.27498923356982,6.98717136730191));
#55991=CARTESIAN_POINT('Ctrl Pts',(-21.,-4.27498923356982,6.98717136730191));
#55992=CARTESIAN_POINT('Ctrl Pts',(-50.,-4.21757413484033,6.90463617300865));
#55993=CARTESIAN_POINT('Ctrl Pts',(-21.,-4.21757413484033,6.90463617300865));
#55994=CARTESIAN_POINT('Ctrl Pts',(-50.,-4.16348379256721,6.82003644526658));
#55995=CARTESIAN_POINT('Ctrl Pts',(-21.,-4.16348379256721,6.82003644526658));
#55996=CARTESIAN_POINT('Ctrl Pts',(-50.,-4.11183783259628,6.73395053478792));
#55997=CARTESIAN_POINT('Ctrl Pts',(-21.,-4.11183783259628,6.73395053478792));
#55998=CARTESIAN_POINT('Ctrl Pts',(-50.,-4.06165666819706,6.64698999124062));
#55999=CARTESIAN_POINT('Ctrl Pts',(-21.,-4.06165666819706,6.64698999124062));
#56000=CARTESIAN_POINT('Ctrl Pts',(-50.,-4.01197889710939,6.55973735411151));
#56001=CARTESIAN_POINT('Ctrl Pts',(-21.,-4.01197889710939,6.55973735411151));
#56002=CARTESIAN_POINT('Ctrl Pts',(-50.,-3.96197913233089,6.47268455970493));
#56003=CARTESIAN_POINT('Ctrl Pts',(-21.,-3.96197913233089,6.47268455970493));
#56004=CARTESIAN_POINT('Ctrl Pts',(-50.,-3.91110213900011,6.38616193008433));
#56005=CARTESIAN_POINT('Ctrl Pts',(-21.,-3.91110213900011,6.38616193008433));
#56006=CARTESIAN_POINT('Ctrl Pts',(-50.,-3.859023878729,6.30036238594766));
#56007=CARTESIAN_POINT('Ctrl Pts',(-21.,-3.859023878729,6.30036238594766));
#56008=CARTESIAN_POINT('Ctrl Pts',(-50.,-3.81627329006595,6.23237673886416));
#56009=CARTESIAN_POINT('Ctrl Pts',(-21.,-3.81627329006595,6.23237673886416));
#56010=CARTESIAN_POINT('Ctrl Pts',(-50.,-3.78357651403939,6.1817683663582));
#56011=CARTESIAN_POINT('Ctrl Pts',(-21.,-3.78357651403939,6.1817683663582));
#56012=CARTESIAN_POINT('Ctrl Pts',(-50.,-3.7614973065729,6.1481985134482));
#56013=CARTESIAN_POINT('Ctrl Pts',(-21.,-3.7614973065729,6.1481985134482));
#56014=CARTESIAN_POINT('Ctrl Pts',(-50.,-3.75038736519793,6.13145585166881));
#56015=CARTESIAN_POINT('Ctrl Pts',(-21.,-3.75038736519793,6.13145585166881));
#56016=CARTESIAN_POINT('',(-21.5,-5.93712762672243,8.04677050399782));
#56017=CARTESIAN_POINT('Ctrl Pts',(-21.5,-5.93712762672243,8.04677050399782));
#56018=CARTESIAN_POINT('Ctrl Pts',(-26.3333333333333,-5.93712762672243,
8.04677050399782));
#56019=CARTESIAN_POINT('Ctrl Pts',(-31.1666666666667,-5.93712762672243,
8.04677050399782));
#56020=CARTESIAN_POINT('Ctrl Pts',(-40.6666666666667,-5.93712762672243,
8.04677050399782));
#56021=CARTESIAN_POINT('Ctrl Pts',(-45.3333333333333,-5.93712762672243,
8.04677050399782));
#56022=CARTESIAN_POINT('Ctrl Pts',(-50.,-5.93712762672243,8.04677050399782));
#56023=CARTESIAN_POINT('Ctrl Pts',(-21.,-5.38825861761966,7.82410819644306));
#56024=CARTESIAN_POINT('Ctrl Pts',(-21.1171767610869,-5.5103250680882,7.88231976704395));
#56025=CARTESIAN_POINT('Ctrl Pts',(-21.2874825276357,-5.69235044790141,
7.96327099664389));
#56026=CARTESIAN_POINT('Ctrl Pts',(-21.5,-5.93712762672243,8.04677050399782));
#56027=CARTESIAN_POINT('Origin',(-35.75,0.,0.));
#56028=CARTESIAN_POINT('',(-21.5,-1.85780428234483,9.82591284555797));
#56029=CARTESIAN_POINT('Origin',(-21.5,0.,0.));
#56030=CARTESIAN_POINT('Ctrl Pts',(-21.5,-1.85780428234483,9.82591284555797));
#56031=CARTESIAN_POINT('Ctrl Pts',(-26.3333333333333,-1.85780428234483,
9.82591284555797));
#56032=CARTESIAN_POINT('Ctrl Pts',(-31.1666666666667,-1.85780428234483,
9.82591284555797));
#56033=CARTESIAN_POINT('Ctrl Pts',(-40.6666666666667,-1.85780428234483,
9.82591284555797));
#56034=CARTESIAN_POINT('Ctrl Pts',(-45.3333333333333,-1.85780428234483,
9.82591284555798));
#56035=CARTESIAN_POINT('Ctrl Pts',(-50.,-1.85780428234483,9.82591284555798));
#56036=CARTESIAN_POINT('Origin',(-21.25,0.,0.));
#56037=CARTESIAN_POINT('Ctrl Pts',(-21.,-1.45989994714919,9.38715570044056));
#56038=CARTESIAN_POINT('Ctrl Pts',(-21.1708653764906,-1.58343885080689,
9.54086217807701));
#56039=CARTESIAN_POINT('Ctrl Pts',(-21.3372400311872,-1.71664935045818,
9.68695766931578));
#56040=CARTESIAN_POINT('Ctrl Pts',(-21.5,-1.85780428234483,9.82591284555798));
#56041=CARTESIAN_POINT('Ctrl Pts',(-50.,-2.42461747220419,10.3189742762293));
#56042=CARTESIAN_POINT('Ctrl Pts',(-21.,-2.42461747220419,10.3189742762293));
#56043=CARTESIAN_POINT('Ctrl Pts',(-50.,-2.40572662366171,10.3043608046855));
#56044=CARTESIAN_POINT('Ctrl Pts',(-21.,-2.40572662366171,10.3043608046855));
#56045=CARTESIAN_POINT('Ctrl Pts',(-50.,-2.36813316049665,10.2750183870592));
#56046=CARTESIAN_POINT('Ctrl Pts',(-21.,-2.36813316049665,10.2750183870592));
#56047=CARTESIAN_POINT('Ctrl Pts',(-50.,-2.31230766835601,10.2306583371767));
#56048=CARTESIAN_POINT('Ctrl Pts',(-21.,-2.31230766835601,10.2306583371767));
#56049=CARTESIAN_POINT('Ctrl Pts',(-50.,-2.2390045785598,10.1708178342288));
#56050=CARTESIAN_POINT('Ctrl Pts',(-21.,-2.2390045785598,10.1708178342288));
#56051=CARTESIAN_POINT('Ctrl Pts',(-50.,-2.14927498796815,10.0948558607226));
#56052=CARTESIAN_POINT('Ctrl Pts',(-21.,-2.14927498796815,10.0948558607226));
#56053=CARTESIAN_POINT('Ctrl Pts',(-50.,-2.0614726885108,10.0177266439074));
#56054=CARTESIAN_POINT('Ctrl Pts',(-21.,-2.0614726885108,10.0177266439074));
#56055=CARTESIAN_POINT('Ctrl Pts',(-50.,-1.97564250382673,9.93942550853734));
#56056=CARTESIAN_POINT('Ctrl Pts',(-21.,-1.97564250382673,9.93942550853734));
#56057=CARTESIAN_POINT('Ctrl Pts',(-50.,-1.89184818563464,9.85995105817688));
#56058=CARTESIAN_POINT('Ctrl Pts',(-21.,-1.89184818563464,9.85995105817688));
#56059=CARTESIAN_POINT('Ctrl Pts',(-50.,-1.81017697820954,9.77930761193764));
#56060=CARTESIAN_POINT('Ctrl Pts',(-21.,-1.81017697820954,9.77930761193764));
#56061=CARTESIAN_POINT('Ctrl Pts',(-50.,-1.73072865645713,9.69750595756857));
#56062=CARTESIAN_POINT('Ctrl Pts',(-21.,-1.73072865645713,9.69750595756857));
#56063=CARTESIAN_POINT('Ctrl Pts',(-50.,-1.65360100339141,9.61456358834088));
#56064=CARTESIAN_POINT('Ctrl Pts',(-21.,-1.65360100339141,9.61456358834088));
#56065=CARTESIAN_POINT('Ctrl Pts',(-50.,-1.57887480066182,9.53050553264656));
#56066=CARTESIAN_POINT('Ctrl Pts',(-21.,-1.57887480066182,9.53050553264656));
#56067=CARTESIAN_POINT('Ctrl Pts',(-50.,-1.50660194229105,9.44536454178638));
#56068=CARTESIAN_POINT('Ctrl Pts',(-21.,-1.50660194229105,9.44536454178638));
#56069=CARTESIAN_POINT('Ctrl Pts',(-50.,-1.43678361338666,9.35918315674388));
#56070=CARTESIAN_POINT('Ctrl Pts',(-21.,-1.43678361338666,9.35918315674388));
#56071=CARTESIAN_POINT('Ctrl Pts',(-50.,-1.3693914299125,9.27200835121914));
#56072=CARTESIAN_POINT('Ctrl Pts',(-21.,-1.3693914299125,9.27200835121914));
#56073=CARTESIAN_POINT('Ctrl Pts',(-50.,-1.30441156144786,9.18388242219763));
#56074=CARTESIAN_POINT('Ctrl Pts',(-21.,-1.30441156144786,9.18388242219763));
#56075=CARTESIAN_POINT('Ctrl Pts',(-50.,-1.24188395306769,9.09483443436949));
#56076=CARTESIAN_POINT('Ctrl Pts',(-21.,-1.24188395306769,9.09483443436949));
#56077=CARTESIAN_POINT('Ctrl Pts',(-50.,-1.18193820283021,9.00487302535333));
#56078=CARTESIAN_POINT('Ctrl Pts',(-21.,-1.18193820283021,9.00487302535333));
#56079=CARTESIAN_POINT('Ctrl Pts',(-50.,-1.12484423754393,8.91397482898789));
#56080=CARTESIAN_POINT('Ctrl Pts',(-21.,-1.12484423754393,8.91397482898789));
#56081=CARTESIAN_POINT('Ctrl Pts',(-50.,-1.07099928020948,8.82209124999857));
#56082=CARTESIAN_POINT('Ctrl Pts',(-21.,-1.07099928020948,8.82209124999857));
#56083=CARTESIAN_POINT('Ctrl Pts',(-50.,-1.02086710880846,8.72916840803945));
#56084=CARTESIAN_POINT('Ctrl Pts',(-21.,-1.02086710880846,8.72916840803945));
#56085=CARTESIAN_POINT('Ctrl Pts',(-50.,-0.974931241694467,8.63516410958082));
#56086=CARTESIAN_POINT('Ctrl Pts',(-21.,-0.974931241694467,8.63516410958082));
#56087=CARTESIAN_POINT('Ctrl Pts',(-50.,-0.933642367528788,8.5400643944807));
#56088=CARTESIAN_POINT('Ctrl Pts',(-21.,-0.933642367528788,8.5400643944807));
#56089=CARTESIAN_POINT('Ctrl Pts',(-50.,-0.897367099160985,8.4439050185459));
#56090=CARTESIAN_POINT('Ctrl Pts',(-21.,-0.897367099160985,8.4439050185459));
#56091=CARTESIAN_POINT('Ctrl Pts',(-50.,-0.86633857713272,8.34677071475058));
#56092=CARTESIAN_POINT('Ctrl Pts',(-21.,-0.86633857713272,8.34677071475058));
#56093=CARTESIAN_POINT('Ctrl Pts',(-50.,-0.840611930230858,8.24877960511329));
#56094=CARTESIAN_POINT('Ctrl Pts',(-21.,-0.840611930230858,8.24877960511329));
#56095=CARTESIAN_POINT('Ctrl Pts',(-50.,-0.82001217136434,8.15007218998677));
#56096=CARTESIAN_POINT('Ctrl Pts',(-21.,-0.82001217136434,8.15007218998677));
#56097=CARTESIAN_POINT('Ctrl Pts',(-50.,-0.804093633570273,8.05079907170372));
#56098=CARTESIAN_POINT('Ctrl Pts',(-21.,-0.804093633570273,8.05079907170372));
#56099=CARTESIAN_POINT('Ctrl Pts',(-50.,-0.792066365329069,7.95110843081948));
#56100=CARTESIAN_POINT('Ctrl Pts',(-21.,-0.792066365329069,7.95110843081948));
#56101=CARTESIAN_POINT('Ctrl Pts',(-50.,-0.782886239966145,7.85113936329068));
#56102=CARTESIAN_POINT('Ctrl Pts',(-21.,-0.782886239966145,7.85113936329068));
#56103=CARTESIAN_POINT('Ctrl Pts',(-50.,-0.775405338877351,7.75101782957587));
#56104=CARTESIAN_POINT('Ctrl Pts',(-21.,-0.775405338877351,7.75101782957587));
#56105=CARTESIAN_POINT('Ctrl Pts',(-50.,-0.768504714146027,7.65085154280962));
#56106=CARTESIAN_POINT('Ctrl Pts',(-21.,-0.768504714146027,7.65085154280962));
#56107=CARTESIAN_POINT('Ctrl Pts',(-50.,-0.761227274615912,7.55072560028829));
#56108=CARTESIAN_POINT('Ctrl Pts',(-21.,-0.761227274615912,7.55072560028829));
#56109=CARTESIAN_POINT('Ctrl Pts',(-50.,-0.752929449590466,7.45069670452966));
#56110=CARTESIAN_POINT('Ctrl Pts',(-21.,-0.752929449590466,7.45069670452966));
#56111=CARTESIAN_POINT('Ctrl Pts',(-50.,-0.743235585416284,7.35079807608913));
#56112=CARTESIAN_POINT('Ctrl Pts',(-21.,-0.743235585416284,7.35079807608913));
#56113=CARTESIAN_POINT('Ctrl Pts',(-50.,-0.734216502709279,7.2709963393441));
#56114=CARTESIAN_POINT('Ctrl Pts',(-21.,-0.734216502709279,7.2709963393441));
#56115=CARTESIAN_POINT('Ctrl Pts',(-50.,-0.726715875322121,7.21121317182152));
#56116=CARTESIAN_POINT('Ctrl Pts',(-21.,-0.726715875322121,7.21121317182152));
#56117=CARTESIAN_POINT('Ctrl Pts',(-50.,-0.721388610069065,7.17138797035723));
#56118=CARTESIAN_POINT('Ctrl Pts',(-21.,-0.721388610069065,7.17138797035723));
#56119=CARTESIAN_POINT('Ctrl Pts',(-50.,-0.718643267461623,7.15148293042304));
#56120=CARTESIAN_POINT('Ctrl Pts',(-21.,-0.718643267461623,7.15148293042304));
#56121=CARTESIAN_POINT('',(-50.,-0.718643267461628,7.15148293042304));
#56122=CARTESIAN_POINT('Origin',(-50.,0.,0.));
#56123=CARTESIAN_POINT('',(-50.,0.718643267461623,7.15148293042304));
#56124=CARTESIAN_POINT('Ctrl Pts',(-50.,0.718643267461623,7.15148293042304));
#56125=CARTESIAN_POINT('Ctrl Pts',(-21.,0.718643267461623,7.15148293042304));
#56126=CARTESIAN_POINT('Ctrl Pts',(-50.,0.721647166649911,7.17509214524366));
#56127=CARTESIAN_POINT('Ctrl Pts',(-21.,0.721647166649911,7.17509214524366));
#56128=CARTESIAN_POINT('Ctrl Pts',(-50.,0.72749213560466,7.22233768688913));
#56129=CARTESIAN_POINT('Ctrl Pts',(-21.,0.72749213560466,7.22233768688913));
#56130=CARTESIAN_POINT('Ctrl Pts',(-50.,0.735771087779772,7.29328733826105));
#56131=CARTESIAN_POINT('Ctrl Pts',(-21.,0.735771087779772,7.29328733826105));
#56132=CARTESIAN_POINT('Ctrl Pts',(-50.,0.745831500234843,7.38804974272502));
#56133=CARTESIAN_POINT('Ctrl Pts',(-21.,0.745831500234843,7.38804974272502));
#56134=CARTESIAN_POINT('Ctrl Pts',(-50.,0.756870878958096,7.5067579169994));
#56135=CARTESIAN_POINT('Ctrl Pts',(-21.,0.756870878958096,7.5067579169994));
#56136=CARTESIAN_POINT('Ctrl Pts',(-50.,0.766672302003445,7.62566969516693));
#56137=CARTESIAN_POINT('Ctrl Pts',(-21.,0.766672302003445,7.62566969516693));
#56138=CARTESIAN_POINT('Ctrl Pts',(-50.,0.775839563797132,7.74468091618948));
#56139=CARTESIAN_POINT('Ctrl Pts',(-21.,0.775839563797132,7.74468091618948));
#56140=CARTESIAN_POINT('Ctrl Pts',(-50.,0.785400272847098,7.86361381479518));
#56141=CARTESIAN_POINT('Ctrl Pts',(-21.,0.785400272847098,7.86361381479518));
#56142=CARTESIAN_POINT('Ctrl Pts',(-50.,0.796736942256154,7.98224460192821));
#56143=CARTESIAN_POINT('Ctrl Pts',(-21.,0.796736942256154,7.98224460192821));
#56144=CARTESIAN_POINT('Ctrl Pts',(-50.,0.811510144890448,8.10033651802127));
#56145=CARTESIAN_POINT('Ctrl Pts',(-21.,0.811510144890448,8.10033651802127));
#56146=CARTESIAN_POINT('Ctrl Pts',(-50.,0.831570515383446,8.21766862525226));
#56147=CARTESIAN_POINT('Ctrl Pts',(-21.,0.831570515383446,8.21766862525226));
#56148=CARTESIAN_POINT('Ctrl Pts',(-50.,0.858916682261844,8.33407215281038));
#56149=CARTESIAN_POINT('Ctrl Pts',(-21.,0.858916682261844,8.33407215281038));
#56150=CARTESIAN_POINT('Ctrl Pts',(-50.,0.895240742652423,8.44941362598824));
#56151=CARTESIAN_POINT('Ctrl Pts',(-21.,0.895240742652423,8.44941362598824));
#56152=CARTESIAN_POINT('Ctrl Pts',(-50.,0.941323460369316,8.56356426545847));
#56153=CARTESIAN_POINT('Ctrl Pts',(-21.,0.941323460369316,8.56356426545847));
#56154=CARTESIAN_POINT('Ctrl Pts',(-50.,0.996589197042052,8.67637972666424));
#56155=CARTESIAN_POINT('Ctrl Pts',(-21.,0.996589197042052,8.67637972666424));
#56156=CARTESIAN_POINT('Ctrl Pts',(-50.,1.05830577327405,8.78766206238304));
#56157=CARTESIAN_POINT('Ctrl Pts',(-21.,1.05830577327405,8.78766206238304));
#56158=CARTESIAN_POINT('Ctrl Pts',(-50.,1.12259642171968,8.89721129760285));
#56159=CARTESIAN_POINT('Ctrl Pts',(-21.,1.12259642171968,8.89721129760285));
#56160=CARTESIAN_POINT('Ctrl Pts',(-50.,1.18634328973517,9.00492385207762));
#56161=CARTESIAN_POINT('Ctrl Pts',(-21.,1.18634328973517,9.00492385207762));
#56162=CARTESIAN_POINT('Ctrl Pts',(-50.,1.24851405668088,9.11085713692575));
#56163=CARTESIAN_POINT('Ctrl Pts',(-21.,1.24851405668088,9.11085713692575));
#56164=CARTESIAN_POINT('Ctrl Pts',(-50.,1.31242393260393,9.21535483920498));
#56165=CARTESIAN_POINT('Ctrl Pts',(-21.,1.31242393260393,9.21535483920498));
#56166=CARTESIAN_POINT('Ctrl Pts',(-50.,1.38484298036779,9.31896299195203));
#56167=CARTESIAN_POINT('Ctrl Pts',(-21.,1.38484298036779,9.31896299195203));
#56168=CARTESIAN_POINT('Ctrl Pts',(-50.,1.47203331296336,9.42213951575228));
#56169=CARTESIAN_POINT('Ctrl Pts',(-21.,1.47203331296336,9.42213951575228));
#56170=CARTESIAN_POINT('Ctrl Pts',(-50.,1.576861582378,9.52503847397034));
#56171=CARTESIAN_POINT('Ctrl Pts',(-21.,1.576861582378,9.52503847397034));
#56172=CARTESIAN_POINT('Ctrl Pts',(-50.,1.69493509590243,9.62722202065427));
#56173=CARTESIAN_POINT('Ctrl Pts',(-21.,1.69493509590243,9.62722202065427));
#56174=CARTESIAN_POINT('Ctrl Pts',(-50.,1.81273846192755,9.72752627760495));
#56175=CARTESIAN_POINT('Ctrl Pts',(-21.,1.81273846192755,9.72752627760495));
#56176=CARTESIAN_POINT('Ctrl Pts',(-50.,1.91151183055746,9.82437388645964));
#56177=CARTESIAN_POINT('Ctrl Pts',(-21.,1.91151183055746,9.82437388645964));
#56178=CARTESIAN_POINT('Ctrl Pts',(-50.,1.97016627452818,9.91601178835393));
#56179=CARTESIAN_POINT('Ctrl Pts',(-21.,1.97016627452818,9.91601178835393));
#56180=CARTESIAN_POINT('Ctrl Pts',(-50.,1.96848522037066,10.0007711148064));
#56181=CARTESIAN_POINT('Ctrl Pts',(-21.,1.96848522037066,10.0007711148064));
#56182=CARTESIAN_POINT('Ctrl Pts',(-50.,1.89041053749867,10.0773349427117));
#56183=CARTESIAN_POINT('Ctrl Pts',(-21.,1.89041053749867,10.0773349427117));
#56184=CARTESIAN_POINT('Ctrl Pts',(-50.,1.72372501438528,10.1447096468161));
#56185=CARTESIAN_POINT('Ctrl Pts',(-21.,1.72372501438528,10.1447096468161));
#56186=CARTESIAN_POINT('Ctrl Pts',(-50.,1.45943182294451,10.2021716552068));
#56187=CARTESIAN_POINT('Ctrl Pts',(-21.,1.45943182294451,10.2021716552068));
#56188=CARTESIAN_POINT('Ctrl Pts',(-50.,1.09127335261449,10.2492257884407));
#56189=CARTESIAN_POINT('Ctrl Pts',(-21.,1.09127335261449,10.2492257884407));
#56190=CARTESIAN_POINT('Ctrl Pts',(-50.,0.615218622302491,10.285561208657));
#56191=CARTESIAN_POINT('Ctrl Pts',(-21.,0.615218622302491,10.285561208657));
#56192=CARTESIAN_POINT('Ctrl Pts',(-50.,0.0289898802580638,10.3110107412798));
#56193=CARTESIAN_POINT('Ctrl Pts',(-21.,0.0289898802580638,10.3110107412798));
#56194=CARTESIAN_POINT('Ctrl Pts',(-50.,-0.668404184972711,10.3255108965746));
#56195=CARTESIAN_POINT('Ctrl Pts',(-21.,-0.668404184972711,10.3255108965746));
#56196=CARTESIAN_POINT('Ctrl Pts',(-50.,-1.31537435394882,10.3283530123025));
#56197=CARTESIAN_POINT('Ctrl Pts',(-21.,-1.31537435394882,10.3283530123025));
#56198=CARTESIAN_POINT('Ctrl Pts',(-50.,-1.85058421429603,10.3255716832032));
#56199=CARTESIAN_POINT('Ctrl Pts',(-21.,-1.85058421429603,10.3255716832032));
#56200=CARTESIAN_POINT('Ctrl Pts',(-50.,-2.22957558565152,10.3215368479529));
#56201=CARTESIAN_POINT('Ctrl Pts',(-21.,-2.22957558565152,10.3215368479529));
#56202=CARTESIAN_POINT('Ctrl Pts',(-50.,-2.42461747220419,10.3189742762293));
#56203=CARTESIAN_POINT('Ctrl Pts',(-21.,-2.42461747220419,10.3189742762293));
#56204=CARTESIAN_POINT('',(-21.5,1.89755147577054,9.81831443766195));
#56205=CARTESIAN_POINT('Ctrl Pts',(-21.5,1.89755147577054,9.81831443766194));
#56206=CARTESIAN_POINT('Ctrl Pts',(-21.47032468389,1.87577485631896,9.79229867840465));
#56207=CARTESIAN_POINT('Ctrl Pts',(-21.4396140182577,1.84982079175808,9.76599200484083));
#56208=CARTESIAN_POINT('Ctrl Pts',(-21.2876118590982,1.71298536184934,9.63694998390189));
#56209=CARTESIAN_POINT('Ctrl Pts',(-21.1610241576491,1.57282267908252,9.53269100720219));
#56210=CARTESIAN_POINT('Ctrl Pts',(-21.,1.44663677770971,9.38920880763537));
#56211=CARTESIAN_POINT('Ctrl Pts',(-50.,1.89755147577054,9.81831443766195));
#56212=CARTESIAN_POINT('Ctrl Pts',(-45.1666666666667,1.89755147577054,9.81831443766195));
#56213=CARTESIAN_POINT('Ctrl Pts',(-40.3333333333333,1.89755147577054,9.81831443766195));
#56214=CARTESIAN_POINT('Ctrl Pts',(-30.8333333333333,1.89755147577054,9.81831443766195));
#56215=CARTESIAN_POINT('Ctrl Pts',(-26.1666666666667,1.89755147577054,9.81831443766195));
#56216=CARTESIAN_POINT('Ctrl Pts',(-21.5,1.89755147577054,9.81831443766195));
#56217=CARTESIAN_POINT('Origin',(-21.25,0.,0.));
#56218=CARTESIAN_POINT('Origin',(-21.5,0.,0.));
#56219=CARTESIAN_POINT('Origin',(-35.75,0.,0.));
#56220=CARTESIAN_POINT('Ctrl Pts',(-50.,3.75038736519793,6.13145585166881));
#56221=CARTESIAN_POINT('Ctrl Pts',(-21.,3.75038736519793,6.13145585166881));
#56222=CARTESIAN_POINT('Ctrl Pts',(-50.,3.7633374392529,6.15142367620606));
#56223=CARTESIAN_POINT('Ctrl Pts',(-21.,3.7633374392529,6.15142367620606));
#56224=CARTESIAN_POINT('Ctrl Pts',(-50.,3.78910264658076,6.19145440139071));
#56225=CARTESIAN_POINT('Ctrl Pts',(-21.,3.78910264658076,6.19145440139071));
#56226=CARTESIAN_POINT('Ctrl Pts',(-50.,3.82734562477572,6.25178572573963));
#56227=CARTESIAN_POINT('Ctrl Pts',(-21.,3.82734562477572,6.25178572573963));
#56228=CARTESIAN_POINT('Ctrl Pts',(-50.,3.87752560957259,6.33279865263617));
#56229=CARTESIAN_POINT('Ctrl Pts',(-21.,3.87752560957259,6.33279865263617));
#56230=CARTESIAN_POINT('Ctrl Pts',(-50.,3.93897729264122,6.43496121510494));
#56231=CARTESIAN_POINT('Ctrl Pts',(-21.,3.93897729264122,6.43496121510494));
#56232=CARTESIAN_POINT('Ctrl Pts',(-50.,3.99940195660266,6.53784434718121));
#56233=CARTESIAN_POINT('Ctrl Pts',(-21.,3.99940195660266,6.53784434718121));
#56234=CARTESIAN_POINT('Ctrl Pts',(-50.,4.05929840765689,6.64109222642907));
#56235=CARTESIAN_POINT('Ctrl Pts',(-21.,4.05929840765689,6.64109222642907));
#56236=CARTESIAN_POINT('Ctrl Pts',(-50.,4.11951535961712,6.74409882925098));
#56237=CARTESIAN_POINT('Ctrl Pts',(-21.,4.11951535961712,6.74409882925098));
#56238=CARTESIAN_POINT('Ctrl Pts',(-50.,4.18120131531612,6.84606267872027));
#56239=CARTESIAN_POINT('Ctrl Pts',(-21.,4.18120131531612,6.84606267872027));
#56240=CARTESIAN_POINT('Ctrl Pts',(-50.,4.24574967308284,6.94604996627335));
#56241=CARTESIAN_POINT('Ctrl Pts',(-21.,4.24574967308284,6.94604996627335));
#56242=CARTESIAN_POINT('Ctrl Pts',(-50.,4.31473193577955,7.04305867353628));
#56243=CARTESIAN_POINT('Ctrl Pts',(-21.,4.31473193577955,7.04305867353628));
#56244=CARTESIAN_POINT('Ctrl Pts',(-50.,4.38987557857684,7.13606957084443));
#56245=CARTESIAN_POINT('Ctrl Pts',(-21.,4.38987557857684,7.13606957084443));
#56246=CARTESIAN_POINT('Ctrl Pts',(-50.,4.4726472158023,7.22422822821349));
#56247=CARTESIAN_POINT('Ctrl Pts',(-21.,4.4726472158023,7.22422822821349));
#56248=CARTESIAN_POINT('Ctrl Pts',(-50.,4.56369441608956,7.30707985875561));
#56249=CARTESIAN_POINT('Ctrl Pts',(-21.,4.56369441608956,7.30707985875561));
#56250=CARTESIAN_POINT('Ctrl Pts',(-50.,4.66243591843161,7.38474417264741));
#56251=CARTESIAN_POINT('Ctrl Pts',(-21.,4.66243591843161,7.38474417264741));
#56252=CARTESIAN_POINT('Ctrl Pts',(-50.,4.76632422816958,7.45822827381644));
#56253=CARTESIAN_POINT('Ctrl Pts',(-21.,4.76632422816958,7.45822827381644));
#56254=CARTESIAN_POINT('Ctrl Pts',(-50.,4.87177973271099,7.52903405731413));
#56255=CARTESIAN_POINT('Ctrl Pts',(-21.,4.87177973271099,7.52903405731413));
#56256=CARTESIAN_POINT('Ctrl Pts',(-50.,4.97594840210465,7.59842098612655));
#56257=CARTESIAN_POINT('Ctrl Pts',(-21.,4.97594840210465,7.59842098612655));
#56258=CARTESIAN_POINT('Ctrl Pts',(-50.,5.07792505734327,7.66688869302314));
#56259=CARTESIAN_POINT('Ctrl Pts',(-21.,5.07792505734327,7.66688869302314));
#56260=CARTESIAN_POINT('Ctrl Pts',(-50.,5.18084571969554,7.73330841361203));
#56261=CARTESIAN_POINT('Ctrl Pts',(-21.,5.18084571969554,7.73330841361203));
#56262=CARTESIAN_POINT('Ctrl Pts',(-50.,5.29104691989087,7.79523468647088));
#56263=CARTESIAN_POINT('Ctrl Pts',(-21.,5.29104691989087,7.79523468647088));
#56264=CARTESIAN_POINT('Ctrl Pts',(-50.,5.41436931107715,7.85036305479183));
#56265=CARTESIAN_POINT('Ctrl Pts',(-21.,5.41436931107715,7.85036305479183));
#56266=CARTESIAN_POINT('Ctrl Pts',(-50.,5.55346250303877,7.89758853118705));
#56267=CARTESIAN_POINT('Ctrl Pts',(-21.,5.55346250303877,7.89758853118705));
#56268=CARTESIAN_POINT('Ctrl Pts',(-50.,5.70417884215966,7.9384225480224));
#56269=CARTESIAN_POINT('Ctrl Pts',(-21.,5.70417884215966,7.9384225480224));
#56270=CARTESIAN_POINT('Ctrl Pts',(-50.,5.85383639353758,7.97768059592143));
#56271=CARTESIAN_POINT('Ctrl Pts',(-21.,5.85383639353758,7.97768059592143));
#56272=CARTESIAN_POINT('Ctrl Pts',(-50.,5.98484872630544,8.02208111792391));
#56273=CARTESIAN_POINT('Ctrl Pts',(-21.,5.98484872630544,8.02208111792391));
#56274=CARTESIAN_POINT('Ctrl Pts',(-50.,6.07745474980597,8.07919480518469));
#56275=CARTESIAN_POINT('Ctrl Pts',(-21.,6.07745474980597,8.07919480518469));
#56276=CARTESIAN_POINT('Ctrl Pts',(-50.,6.11271586583108,8.15628970164627));
#56277=CARTESIAN_POINT('Ctrl Pts',(-21.,6.11271586583108,8.15628970164627));
#56278=CARTESIAN_POINT('Ctrl Pts',(-50.,6.07559280712476,8.2591466623313));
#56279=CARTESIAN_POINT('Ctrl Pts',(-21.,6.07559280712476,8.2591466623313));
#56280=CARTESIAN_POINT('Ctrl Pts',(-50.,5.9546471286083,8.39217131123866));
#56281=CARTESIAN_POINT('Ctrl Pts',(-21.,5.9546471286083,8.39217131123866));
#56282=CARTESIAN_POINT('Ctrl Pts',(-50.,5.74145902217939,8.55861531001153));
#56283=CARTESIAN_POINT('Ctrl Pts',(-21.,5.74145902217939,8.55861531001153));
#56284=CARTESIAN_POINT('Ctrl Pts',(-50.,5.43017572522592,8.760747592856));
#56285=CARTESIAN_POINT('Ctrl Pts',(-21.,5.43017572522592,8.760747592856));
#56286=CARTESIAN_POINT('Ctrl Pts',(-50.,5.01703058178298,9.00003708168539));
#56287=CARTESIAN_POINT('Ctrl Pts',(-21.,5.01703058178298,9.00003708168539));
#56288=CARTESIAN_POINT('Ctrl Pts',(-50.,4.4998988741045,9.27732143685757));
#56289=CARTESIAN_POINT('Ctrl Pts',(-21.,4.4998988741045,9.27732143685757));
#56290=CARTESIAN_POINT('Ctrl Pts',(-50.,3.87785991426877,9.59297357001867));
#56291=CARTESIAN_POINT('Ctrl Pts',(-21.,3.87785991426877,9.59297357001867));
#56292=CARTESIAN_POINT('Ctrl Pts',(-50.,3.29619308135874,9.87624406382134));
#56293=CARTESIAN_POINT('Ctrl Pts',(-21.,3.29619308135874,9.87624406382134));
#56294=CARTESIAN_POINT('Ctrl Pts',(-50.,2.8127788859222,10.1059570283115));
#56295=CARTESIAN_POINT('Ctrl Pts',(-21.,2.8127788859222,10.1059570283115));
#56296=CARTESIAN_POINT('Ctrl Pts',(-50.,2.46956880972213,10.2667599606609));
#56297=CARTESIAN_POINT('Ctrl Pts',(-21.,2.46956880972213,10.2667599606609));
#56298=CARTESIAN_POINT('Ctrl Pts',(-50.,2.29273028380004,10.3490766663382));
#56299=CARTESIAN_POINT('Ctrl Pts',(-21.,2.29273028380004,10.3490766663382));
#56300=CARTESIAN_POINT('',(-21.5,5.96964178495622,8.0226789141349));
#56301=CARTESIAN_POINT('Ctrl Pts',(-50.,5.96964178495622,8.0226789141349));
#56302=CARTESIAN_POINT('Ctrl Pts',(-45.1666666666667,5.96964178495622,8.0226789141349));
#56303=CARTESIAN_POINT('Ctrl Pts',(-40.3333333333333,5.96964178495622,8.0226789141349));
#56304=CARTESIAN_POINT('Ctrl Pts',(-30.8333333333333,5.96964178495622,8.0226789141349));
#56305=CARTESIAN_POINT('Ctrl Pts',(-26.1666666666667,5.96964178495622,8.0226789141349));
#56306=CARTESIAN_POINT('Ctrl Pts',(-21.5,5.96964178495622,8.0226789141349));
#56307=CARTESIAN_POINT('',(-50.,3.75038736519793,6.13145585166881));
#56308=CARTESIAN_POINT('Ctrl Pts',(-21.5,5.96964178495622,8.0226789141349));
#56309=CARTESIAN_POINT('Ctrl Pts',(-21.471640009925,5.94010387156985,8.0093081760178));
#56310=CARTESIAN_POINT('Ctrl Pts',(-21.4423497933815,5.90702876507376,7.99736128679984));
#56311=CARTESIAN_POINT('Ctrl Pts',(-21.2909092331889,5.72905875838041,7.94024959050558));
#56312=CARTESIAN_POINT('Ctrl Pts',(-21.1629721875821,5.55527241504999,7.9071372002529));
#56313=CARTESIAN_POINT('Ctrl Pts',(-21.,5.37719972469147,7.83171265565699));
#56314=CARTESIAN_POINT('Origin',(-50.,0.,0.));
#56315=CARTESIAN_POINT('',(-50.,2.45543694297674,6.75507110762463));
#56316=CARTESIAN_POINT('Ctrl Pts',(-50.,2.29273028380004,10.3490766663382));
#56317=CARTESIAN_POINT('Ctrl Pts',(-21.,2.29273028380004,10.3490766663382));
#56318=CARTESIAN_POINT('Ctrl Pts',(-50.,2.30340980255016,10.3277139514246));
#56319=CARTESIAN_POINT('Ctrl Pts',(-21.,2.30340980255016,10.3277139514246));
#56320=CARTESIAN_POINT('Ctrl Pts',(-50.,2.32454914462406,10.2849661542698));
#56321=CARTESIAN_POINT('Ctrl Pts',(-21.,2.32454914462406,10.2849661542698));
#56322=CARTESIAN_POINT('Ctrl Pts',(-50.,2.35559907076766,10.2207773570791));
#56323=CARTESIAN_POINT('Ctrl Pts',(-21.,2.35559907076766,10.2207773570791));
#56324=CARTESIAN_POINT('Ctrl Pts',(-50.,2.39567905142538,10.1350579081937));
#56325=CARTESIAN_POINT('Ctrl Pts',(-21.,2.39567905142538,10.1350579081937));
#56326=CARTESIAN_POINT('Ctrl Pts',(-50.,2.44356395398246,10.0276863246448));
#56327=CARTESIAN_POINT('Ctrl Pts',(-21.,2.44356395398246,10.0276863246448));
#56328=CARTESIAN_POINT('Ctrl Pts',(-50.,2.48920597933682,9.92009931149698));
#56329=CARTESIAN_POINT('Ctrl Pts',(-21.,2.48920597933682,9.92009931149698));
#56330=CARTESIAN_POINT('Ctrl Pts',(-50.,2.53256271427195,9.81231210474723));
#56331=CARTESIAN_POINT('Ctrl Pts',(-21.,2.53256271427195,9.81231210474723));
#56332=CARTESIAN_POINT('Ctrl Pts',(-50.,2.57357611458342,9.70435110708481));
#56333=CARTESIAN_POINT('Ctrl Pts',(-21.,2.57357611458342,9.70435110708481));
#56334=CARTESIAN_POINT('Ctrl Pts',(-50.,2.61216944988784,9.59625806376705));
#56335=CARTESIAN_POINT('Ctrl Pts',(-21.,2.61216944988784,9.59625806376705));
#56336=CARTESIAN_POINT('Ctrl Pts',(-50.,2.64825750673019,9.48808598492904));
#56337=CARTESIAN_POINT('Ctrl Pts',(-21.,2.64825750673019,9.48808598492904));
#56338=CARTESIAN_POINT('Ctrl Pts',(-50.,2.68175977570501,9.37989305792331));
#56339=CARTESIAN_POINT('Ctrl Pts',(-21.,2.68175977570501,9.37989305792331));
#56340=CARTESIAN_POINT('Ctrl Pts',(-50.,2.71261433447332,9.27173688239595));
#56341=CARTESIAN_POINT('Ctrl Pts',(-21.,2.71261433447332,9.27173688239595));
#56342=CARTESIAN_POINT('Ctrl Pts',(-50.,2.74078863839312,9.16366948222194));
#56343=CARTESIAN_POINT('Ctrl Pts',(-21.,2.74078863839312,9.16366948222194));
#56344=CARTESIAN_POINT('Ctrl Pts',(-50.,2.76630007756038,9.05572969970197));
#56345=CARTESIAN_POINT('Ctrl Pts',(-21.,2.76630007756038,9.05572969970197));
#56346=CARTESIAN_POINT('Ctrl Pts',(-50.,2.78919460623265,8.94794754130566));
#56347=CARTESIAN_POINT('Ctrl Pts',(-21.,2.78919460623265,8.94794754130566));
#56348=CARTESIAN_POINT('Ctrl Pts',(-50.,2.80950303716262,8.84035511450549));
#56349=CARTESIAN_POINT('Ctrl Pts',(-21.,2.80950303716262,8.84035511450549));
#56350=CARTESIAN_POINT('Ctrl Pts',(-50.,2.82720199177778,8.73299593720093));
#56351=CARTESIAN_POINT('Ctrl Pts',(-21.,2.82720199177778,8.73299593720093));
#56352=CARTESIAN_POINT('Ctrl Pts',(-50.,2.84217845398458,8.62593402210748));
#56353=CARTESIAN_POINT('Ctrl Pts',(-21.,2.84217845398458,8.62593402210748));
#56354=CARTESIAN_POINT('Ctrl Pts',(-50.,2.85417908993455,8.51926543389428));
#56355=CARTESIAN_POINT('Ctrl Pts',(-21.,2.85417908993455,8.51926543389428));
#56356=CARTESIAN_POINT('Ctrl Pts',(-50.,2.86282492937103,8.41311873833255));
#56357=CARTESIAN_POINT('Ctrl Pts',(-21.,2.86282492937103,8.41311873833255));
#56358=CARTESIAN_POINT('Ctrl Pts',(-50.,2.86767474496505,8.30764661663281));
#56359=CARTESIAN_POINT('Ctrl Pts',(-21.,2.86767474496505,8.30764661663281));
#56360=CARTESIAN_POINT('Ctrl Pts',(-50.,2.8682745946465,8.20302084448955));
#56361=CARTESIAN_POINT('Ctrl Pts',(-21.,2.8682745946465,8.20302084448955));
#56362=CARTESIAN_POINT('Ctrl Pts',(-50.,2.86421236488386,8.099424390731));
#56363=CARTESIAN_POINT('Ctrl Pts',(-21.,2.86421236488386,8.099424390731));
#56364=CARTESIAN_POINT('Ctrl Pts',(-50.,2.85517326277626,7.9970485375799));
#56365=CARTESIAN_POINT('Ctrl Pts',(-21.,2.85517326277626,7.9970485375799));
#56366=CARTESIAN_POINT('Ctrl Pts',(-50.,2.84098400021345,7.89607078269802));
#56367=CARTESIAN_POINT('Ctrl Pts',(-21.,2.84098400021345,7.89607078269802));
#56368=CARTESIAN_POINT('Ctrl Pts',(-50.,2.82164615909785,7.79662146983088));
#56369=CARTESIAN_POINT('Ctrl Pts',(-21.,2.82164615909785,7.79662146983088));
#56370=CARTESIAN_POINT('Ctrl Pts',(-50.,2.79737835816915,7.69875126136884));
#56371=CARTESIAN_POINT('Ctrl Pts',(-21.,2.79737835816915,7.69875126136884));
#56372=CARTESIAN_POINT('Ctrl Pts',(-50.,2.76864747338962,7.60240247767684));
#56373=CARTESIAN_POINT('Ctrl Pts',(-21.,2.76864747338962,7.60240247767684));
#56374=CARTESIAN_POINT('Ctrl Pts',(-50.,2.73622951961898,7.50736587770304));
#56375=CARTESIAN_POINT('Ctrl Pts',(-21.,2.73622951961898,7.50736587770304));
#56376=CARTESIAN_POINT('Ctrl Pts',(-50.,2.70112557395893,7.41331375298832));
#56377=CARTESIAN_POINT('Ctrl Pts',(-21.,2.70112557395893,7.41331375298832));
#56378=CARTESIAN_POINT('Ctrl Pts',(-50.,2.66442452752942,7.31986152676826));
#56379=CARTESIAN_POINT('Ctrl Pts',(-21.,2.66442452752942,7.31986152676826));
#56380=CARTESIAN_POINT('Ctrl Pts',(-50.,2.62718125254576,7.22662075191781));
#56381=CARTESIAN_POINT('Ctrl Pts',(-21.,2.62718125254576,7.22662075191781));
#56382=CARTESIAN_POINT('Ctrl Pts',(-50.,2.59029498067661,7.13325283216217));
#56383=CARTESIAN_POINT('Ctrl Pts',(-21.,2.59029498067661,7.13325283216217));
#56384=CARTESIAN_POINT('Ctrl Pts',(-50.,2.55437015138428,7.03952961984441));
#56385=CARTESIAN_POINT('Ctrl Pts',(-21.,2.55437015138428,7.03952961984441));
#56386=CARTESIAN_POINT('Ctrl Pts',(-50.,2.5197596307744,6.94531805563895));
#56387=CARTESIAN_POINT('Ctrl Pts',(-21.,2.5197596307744,6.94531805563895));
#56388=CARTESIAN_POINT('Ctrl Pts',(-50.,2.49326086758344,6.8695059418988));
#56389=CARTESIAN_POINT('Ctrl Pts',(-21.,2.49326086758344,6.8695059418988));
#56390=CARTESIAN_POINT('Ctrl Pts',(-50.,2.47407975508802,6.8123887688799));
#56391=CARTESIAN_POINT('Ctrl Pts',(-21.,2.47407975508802,6.8123887688799));
#56392=CARTESIAN_POINT('Ctrl Pts',(-50.,2.46159994790965,6.77419608843537));
#56393=CARTESIAN_POINT('Ctrl Pts',(-21.,2.46159994790965,6.77419608843537));
#56394=CARTESIAN_POINT('Ctrl Pts',(-50.,2.45543694297675,6.75507110762463));
#56395=CARTESIAN_POINT('Ctrl Pts',(-21.,2.45543694297675,6.75507110762463));
#56396=CARTESIAN_POINT('',(-21.5,2.58947998462545,9.65891264114259));
#56397=CARTESIAN_POINT('Ctrl Pts',(-21.5,2.58947998462545,9.65891264114259));
#56398=CARTESIAN_POINT('Ctrl Pts',(-26.3333333333333,2.58947998462545,9.65891264114259));
#56399=CARTESIAN_POINT('Ctrl Pts',(-31.1666666666667,2.58947998462545,9.65891264114259));
#56400=CARTESIAN_POINT('Ctrl Pts',(-40.6666666666667,2.58947998462545,9.65891264114259));
#56401=CARTESIAN_POINT('Ctrl Pts',(-45.3333333333333,2.58947998462545,9.65891264114259));
#56402=CARTESIAN_POINT('Ctrl Pts',(-50.,2.58947998462545,9.65891264114259));
#56403=CARTESIAN_POINT('Ctrl Pts',(-21.,2.75760981235205,9.09096189205629));
#56404=CARTESIAN_POINT('Ctrl Pts',(-21.0595504621605,2.74206083288776,9.15790831819842));
#56405=CARTESIAN_POINT('Ctrl Pts',(-21.1201969195959,2.72465875026614,9.2263731836371));
#56406=CARTESIAN_POINT('Ctrl Pts',(-21.1820623827059,2.70512289983591,9.29649306845955));
#56407=CARTESIAN_POINT('Ctrl Pts',(-21.2426667634852,2.68598527346403,9.36518361058689));
#56408=CARTESIAN_POINT('Ctrl Pts',(-21.3044409593758,2.66479906737137,9.43546228600892));
#56409=CARTESIAN_POINT('Ctrl Pts',(-21.367500610643,2.64134946113152,9.50742323600585));
#56410=CARTESIAN_POINT('Ctrl Pts',(-21.4110415416979,2.62515816181354,9.5571102656595));
#56411=CARTESIAN_POINT('Ctrl Pts',(-21.45519531585,2.60788916582949,9.60759844441249));
#56412=CARTESIAN_POINT('Ctrl Pts',(-21.5,2.58947998461739,9.65891264116508));
#56413=CARTESIAN_POINT('Origin',(-35.75,0.,0.));
#56414=CARTESIAN_POINT('',(-21.5,6.52388598275276,7.57884632935924));
#56415=CARTESIAN_POINT('Origin',(-21.5,0.,0.));
#56416=CARTESIAN_POINT('Ctrl Pts',(-21.5,6.52388598275276,7.57884632935924));
#56417=CARTESIAN_POINT('Ctrl Pts',(-26.3333333333333,6.52388598275276,7.57884632935924));
#56418=CARTESIAN_POINT('Ctrl Pts',(-31.1666666666667,6.52388598275276,7.57884632935924));
#56419=CARTESIAN_POINT('Ctrl Pts',(-40.6666666666667,6.52388598275276,7.57884632935924));
#56420=CARTESIAN_POINT('Ctrl Pts',(-45.3333333333333,6.52388598275276,7.57884632935924));
#56421=CARTESIAN_POINT('Ctrl Pts',(-50.,6.52388598275276,7.57884632935924));
#56422=CARTESIAN_POINT('Origin',(-21.25,0.,0.));
#56423=CARTESIAN_POINT('Ctrl Pts',(-21.,6.42894112865204,6.99419158761941));
#56424=CARTESIAN_POINT('Ctrl Pts',(-21.1171767610994,6.45853087308296,7.12615087039341));
#56425=CARTESIAN_POINT('Ctrl Pts',(-21.2874825276462,6.49694802882376,7.32162583711294));
#56426=CARTESIAN_POINT('Ctrl Pts',(-21.5,6.52388598275277,7.57884632935924));
#56427=CARTESIAN_POINT('Ctrl Pts',(-50.,6.55597468860601,8.32941749958287));
#56428=CARTESIAN_POINT('Ctrl Pts',(-21.,6.55597468860601,8.32941749958287));
#56429=CARTESIAN_POINT('Ctrl Pts',(-50.,6.55632766789962,8.30553668898452));
#56430=CARTESIAN_POINT('Ctrl Pts',(-21.,6.55632766789962,8.30553668898452));
#56431=CARTESIAN_POINT('Ctrl Pts',(-50.,6.55682598292761,8.25785023779518));
#56432=CARTESIAN_POINT('Ctrl Pts',(-21.,6.55682598292761,8.25785023779518));
#56433=CARTESIAN_POINT('Ctrl Pts',(-50.,6.55695052439907,8.18654607180369));
#56434=CARTESIAN_POINT('Ctrl Pts',(-21.,6.55695052439907,8.18654607180369));
#56435=CARTESIAN_POINT('Ctrl Pts',(-50.,6.55586906420033,8.0919254651127));
#56436=CARTESIAN_POINT('Ctrl Pts',(-21.,6.55586906420033,8.0919254651127));
#56437=CARTESIAN_POINT('Ctrl Pts',(-50.,6.55242508650163,7.97441053046901));
#56438=CARTESIAN_POINT('Ctrl Pts',(-21.,6.55242508650163,7.97441053046901));
#56439=CARTESIAN_POINT('Ctrl Pts',(-50.,6.54686687486885,7.85767464841055));
#56440=CARTESIAN_POINT('Ctrl Pts',(-21.,6.54686687486885,7.85767464841055));
#56441=CARTESIAN_POINT('Ctrl Pts',(-50.,6.53916282696568,7.74174994850129));
#56442=CARTESIAN_POINT('Ctrl Pts',(-21.,6.53916282696568,7.74174994850129));
#56443=CARTESIAN_POINT('Ctrl Pts',(-50.,6.5292721024685,7.6266854031787));
#56444=CARTESIAN_POINT('Ctrl Pts',(-21.,6.5292721024685,7.6266854031787));
#56445=CARTESIAN_POINT('Ctrl Pts',(-50.,6.51714368227899,7.51255191568567));
#56446=CARTESIAN_POINT('Ctrl Pts',(-21.,6.51714368227899,7.51255191568567));
#56447=CARTESIAN_POINT('Ctrl Pts',(-50.,6.5027237919627,7.39943421923609));
#56448=CARTESIAN_POINT('Ctrl Pts',(-21.,6.5027237919627,7.39943421923609));
#56449=CARTESIAN_POINT('Ctrl Pts',(-50.,6.48596514159778,7.28741967054497));
#56450=CARTESIAN_POINT('Ctrl Pts',(-21.,6.48596514159778,7.28741967054497));
#56451=CARTESIAN_POINT('Ctrl Pts',(-50.,6.46683693263443,7.17658703219621));
#56452=CARTESIAN_POINT('Ctrl Pts',(-21.,6.46683693263443,7.17658703219621));
#56453=CARTESIAN_POINT('Ctrl Pts',(-50.,6.44533241567678,7.06699729667253));
#56454=CARTESIAN_POINT('Ctrl Pts',(-21.,6.44533241567678,7.06699729667253));
#56455=CARTESIAN_POINT('Ctrl Pts',(-50.,6.42148411170256,6.95867791439771));
#56456=CARTESIAN_POINT('Ctrl Pts',(-21.,6.42148411170256,6.95867791439771));
#56457=CARTESIAN_POINT('Ctrl Pts',(-50.,6.39534644338642,6.85163598146165));
#56458=CARTESIAN_POINT('Ctrl Pts',(-21.,6.39534644338642,6.85163598146165));
#56459=CARTESIAN_POINT('Ctrl Pts',(-50.,6.36696110296949,6.74588705654512));
#56460=CARTESIAN_POINT('Ctrl Pts',(-21.,6.36696110296949,6.74588705654512));
#56461=CARTESIAN_POINT('Ctrl Pts',(-50.,6.33632590879467,6.64148049150319));
#56462=CARTESIAN_POINT('Ctrl Pts',(-21.,6.33632590879467,6.64148049150319));
#56463=CARTESIAN_POINT('Ctrl Pts',(-50.,6.30336681095649,6.53852299564495));
#56464=CARTESIAN_POINT('Ctrl Pts',(-21.,6.30336681095649,6.53852299564495));
#56465=CARTESIAN_POINT('Ctrl Pts',(-50.,6.2678972444421,6.43721103768399));
#56466=CARTESIAN_POINT('Ctrl Pts',(-21.,6.2678972444421,6.43721103768399));
#56467=CARTESIAN_POINT('Ctrl Pts',(-50.,6.22963155144596,6.33782488040965));
#56468=CARTESIAN_POINT('Ctrl Pts',(-21.,6.22963155144596,6.33782488040965));
#56469=CARTESIAN_POINT('Ctrl Pts',(-50.,6.18823844577549,6.2406935262026));
#56470=CARTESIAN_POINT('Ctrl Pts',(-21.,6.18823844577549,6.2406935262026));
#56471=CARTESIAN_POINT('Ctrl Pts',(-50.,6.14338347043832,6.14616869769857));
#56472=CARTESIAN_POINT('Ctrl Pts',(-21.,6.14338347043832,6.14616869769857));
#56473=CARTESIAN_POINT('Ctrl Pts',(-50.,6.09477471117184,6.05459405347559));
#56474=CARTESIAN_POINT('Ctrl Pts',(-21.,6.09477471117184,6.05459405347559));
#56475=CARTESIAN_POINT('Ctrl Pts',(-50.,6.04221154361855,5.96627851638222));
#56476=CARTESIAN_POINT('Ctrl Pts',(-21.,6.04221154361855,5.96627851638222));
#56477=CARTESIAN_POINT('Ctrl Pts',(-50.,5.98561485393513,5.88145719317904));
#56478=CARTESIAN_POINT('Ctrl Pts',(-21.,5.98561485393513,5.88145719317904));
#56479=CARTESIAN_POINT('Ctrl Pts',(-50.,5.92504262139805,5.80024683316115));
#56480=CARTESIAN_POINT('Ctrl Pts',(-21.,5.92504262139805,5.80024683316115));
#56481=CARTESIAN_POINT('Ctrl Pts',(-50.,5.86071379627312,5.72259822644884));
#56482=CARTESIAN_POINT('Ctrl Pts',(-21.,5.86071379627312,5.72259822644884));
#56483=CARTESIAN_POINT('Ctrl Pts',(-50.,5.79302399301176,5.64825683559838));
#56484=CARTESIAN_POINT('Ctrl Pts',(-21.,5.79302399301176,5.64825683559838));
#56485=CARTESIAN_POINT('Ctrl Pts',(-50.,5.72258159055366,5.57669744070723));
#56486=CARTESIAN_POINT('Ctrl Pts',(-21.,5.72258159055366,5.57669744070723));
#56487=CARTESIAN_POINT('Ctrl Pts',(-50.,5.65014634083023,5.50719043557996));
#56488=CARTESIAN_POINT('Ctrl Pts',(-21.,5.65014634083023,5.50719043557996));
#56489=CARTESIAN_POINT('Ctrl Pts',(-50.,5.57653243923659,5.43891687637388));
#56490=CARTESIAN_POINT('Ctrl Pts',(-21.,5.57653243923659,5.43891687637388));
#56491=CARTESIAN_POINT('Ctrl Pts',(-50.,5.50252175190725,5.37106909242141));
#56492=CARTESIAN_POINT('Ctrl Pts',(-21.,5.50252175190725,5.37106909242141));
#56493=CARTESIAN_POINT('Ctrl Pts',(-50.,5.42877754716296,5.30295185702147));
#56494=CARTESIAN_POINT('Ctrl Pts',(-21.,5.42877754716296,5.30295185702147));
#56495=CARTESIAN_POINT('Ctrl Pts',(-50.,5.35574541658332,5.23409735978387));
#56496=CARTESIAN_POINT('Ctrl Pts',(-21.,5.35574541658332,5.23409735978387));
#56497=CARTESIAN_POINT('Ctrl Pts',(-50.,5.28368554926634,5.16423261553338));
#56498=CARTESIAN_POINT('Ctrl Pts',(-21.,5.28368554926634,5.16423261553338));
#56499=CARTESIAN_POINT('Ctrl Pts',(-50.,5.22691734521339,5.10742564369892));
#56500=CARTESIAN_POINT('Ctrl Pts',(-21.,5.22691734521339,5.10742564369892));
#56501=CARTESIAN_POINT('Ctrl Pts',(-50.,5.18485354740602,5.06428722179623));
#56502=CARTESIAN_POINT('Ctrl Pts',(-21.,5.18485354740602,5.06428722179623));
#56503=CARTESIAN_POINT('Ctrl Pts',(-50.,5.15703844666268,5.03529159113598));
#56504=CARTESIAN_POINT('Ctrl Pts',(-21.,5.15703844666268,5.03529159113598));
#56505=CARTESIAN_POINT('Ctrl Pts',(-50.,5.14318775290069,5.02073460645076));
#56506=CARTESIAN_POINT('Ctrl Pts',(-21.,5.14318775290069,5.02073460645076));
#56507=CARTESIAN_POINT('',(-50.,5.14318775290069,5.02073460645077));
#56508=CARTESIAN_POINT('Origin',(-50.,0.,0.));
#56509=CARTESIAN_POINT('',(-50.,6.03932124977421,3.89701874412038));
#56510=CARTESIAN_POINT('Ctrl Pts',(-50.,6.03932124977421,3.89701874412038));
#56511=CARTESIAN_POINT('Ctrl Pts',(-21.,6.03932124977421,3.89701874412038));
#56512=CARTESIAN_POINT('Ctrl Pts',(-50.,6.05965257770704,3.90939030583537));
#56513=CARTESIAN_POINT('Ctrl Pts',(-21.,6.05965257770704,3.90939030583537));
#56514=CARTESIAN_POINT('Ctrl Pts',(-50.,6.10023490810719,3.93427763849175));
#56515=CARTESIAN_POINT('Ctrl Pts',(-21.,6.10023490810719,3.93427763849175));
#56516=CARTESIAN_POINT('Ctrl Pts',(-50.,6.16086742147114,3.97204127711522));
#56517=CARTESIAN_POINT('Ctrl Pts',(-21.,6.16086742147114,3.97204127711522));
#56518=CARTESIAN_POINT('Ctrl Pts',(-50.,6.24122821720367,4.02325912271413));
#56519=CARTESIAN_POINT('Ctrl Pts',(-21.,6.24122821720367,4.02325912271413));
#56520=CARTESIAN_POINT('Ctrl Pts',(-50.,6.34092094513049,4.08864152493875));
#56521=CARTESIAN_POINT('Ctrl Pts',(-21.,6.34092094513049,4.08864152493875));
#56522=CARTESIAN_POINT('Ctrl Pts',(-50.,6.44000100425059,4.15511874483725));
#56523=CARTESIAN_POINT('Ctrl Pts',(-21.,6.44000100425059,4.15511874483725));
#56524=CARTESIAN_POINT('Ctrl Pts',(-50.,6.53876341785232,4.22215377357323));
#56525=CARTESIAN_POINT('Ctrl Pts',(-21.,6.53876341785232,4.22215377357323));
#56526=CARTESIAN_POINT('Ctrl Pts',(-50.,6.63770990687462,4.2888323596294));
#56527=CARTESIAN_POINT('Ctrl Pts',(-21.,6.63770990687462,4.2888323596294));
#56528=CARTESIAN_POINT('Ctrl Pts',(-50.,6.73752748880879,4.35393408054299));
#56529=CARTESIAN_POINT('Ctrl Pts',(-21.,6.73752748880879,4.35393408054299));
#56530=CARTESIAN_POINT('Ctrl Pts',(-50.,6.83906640781858,4.4160130309926));
#56531=CARTESIAN_POINT('Ctrl Pts',(-21.,6.83906640781858,4.4160130309926));
#56532=CARTESIAN_POINT('Ctrl Pts',(-50.,6.94330777957998,4.47348457408032));
#56533=CARTESIAN_POINT('Ctrl Pts',(-21.,6.94330777957998,4.47348457408032));
#56534=CARTESIAN_POINT('Ctrl Pts',(-50.,7.05136577826386,4.52468089222283));
#56535=CARTESIAN_POINT('Ctrl Pts',(-21.,7.05136577826386,4.52468089222283));
#56536=CARTESIAN_POINT('Ctrl Pts',(-50.,7.16419105444418,4.56819583049617));
#56537=CARTESIAN_POINT('Ctrl Pts',(-21.,7.16419105444418,4.56819583049617));
#56538=CARTESIAN_POINT('Ctrl Pts',(-50.,7.28216972266428,4.60333867057275));
#56539=CARTESIAN_POINT('Ctrl Pts',(-21.,7.28216972266428,4.60333867057275));
#56540=CARTESIAN_POINT('Ctrl Pts',(-50.,7.40483002515176,4.63046946729401));
#56541=CARTESIAN_POINT('Ctrl Pts',(-21.,7.40483002515176,4.63046946729401));
#56542=CARTESIAN_POINT('Ctrl Pts',(-50.,7.53031371454558,4.65160090645339));
#56543=CARTESIAN_POINT('Ctrl Pts',(-21.,7.53031371454558,4.65160090645339));
#56544=CARTESIAN_POINT('Ctrl Pts',(-50.,7.65604731918147,4.66963928443128));
#56545=CARTESIAN_POINT('Ctrl Pts',(-21.,7.65604731918147,4.66963928443128));
#56546=CARTESIAN_POINT('Ctrl Pts',(-50.,7.78000590743498,4.68695765535521));
#56547=CARTESIAN_POINT('Ctrl Pts',(-21.,7.78000590743498,4.68695765535521));
#56548=CARTESIAN_POINT('Ctrl Pts',(-50.,7.9015907237349,4.70439891524807));
#56549=CARTESIAN_POINT('Ctrl Pts',(-21.,7.9015907237349,4.70439891524807));
#56550=CARTESIAN_POINT('Ctrl Pts',(-50.,8.02313747309844,4.71958541389958));
#56551=CARTESIAN_POINT('Ctrl Pts',(-21.,8.02313747309844,4.71958541389958));
#56552=CARTESIAN_POINT('Ctrl Pts',(-50.,8.14929412649754,4.72756454905465));
#56553=CARTESIAN_POINT('Ctrl Pts',(-21.,8.14929412649754,4.72756454905465));
#56554=CARTESIAN_POINT('Ctrl Pts',(-50.,8.2843230642502,4.72372591244527));
#56555=CARTESIAN_POINT('Ctrl Pts',(-21.,8.2843230642502,4.72372591244527));
#56556=CARTESIAN_POINT('Ctrl Pts',(-50.,8.43013206622476,4.70592432223511));
#56557=CARTESIAN_POINT('Ctrl Pts',(-21.,8.43013206622476,4.70592432223511));
#56558=CARTESIAN_POINT('Ctrl Pts',(-50.,8.58364001156461,4.67732113139128));
#56559=CARTESIAN_POINT('Ctrl Pts',(-21.,8.58364001156461,4.67732113139128));
#56560=CARTESIAN_POINT('Ctrl Pts',(-50.,8.73551023481551,4.6477574323839));
#56561=CARTESIAN_POINT('Ctrl Pts',(-21.,8.73551023481551,4.6477574323839));
#56562=CARTESIAN_POINT('Ctrl Pts',(-50.,8.87281293245584,4.63091679961492));
#56563=CARTESIAN_POINT('Ctrl Pts',(-21.,8.87281293245584,4.63091679961492));
#56564=CARTESIAN_POINT('Ctrl Pts',(-50.,8.98102877679355,4.64219420602678));
#56565=CARTESIAN_POINT('Ctrl Pts',(-21.,8.98102877679355,4.64219420602678));
#56566=CARTESIAN_POINT('Ctrl Pts',(-50.,9.04624816652329,4.69635508274639));
#56567=CARTESIAN_POINT('Ctrl Pts',(-21.,9.04624816652329,4.69635508274639));
#56568=CARTESIAN_POINT('Ctrl Pts',(-50.,9.05742940904388,4.80513309368965));
#56569=CARTESIAN_POINT('Ctrl Pts',(-21.,9.05742940904388,4.80513309368965));
#56570=CARTESIAN_POINT('Ctrl Pts',(-50.,9.00617835005594,4.97746052424366));
#56571=CARTESIAN_POINT('Ctrl Pts',(-21.,9.00617835005594,4.97746052424366));
#56572=CARTESIAN_POINT('Ctrl Pts',(-50.,8.88631984769767,5.21992023813997));
#56573=CARTESIAN_POINT('Ctrl Pts',(-21.,8.88631984769767,5.21992023813997));
#56574=CARTESIAN_POINT('Ctrl Pts',(-50.,8.6935651987215,5.53709589298789));
#56575=CARTESIAN_POINT('Ctrl Pts',(-21.,8.6935651987215,5.53709589298789));
#56576=CARTESIAN_POINT('Ctrl Pts',(-50.,8.42515810469916,5.93194523247474));
#56577=CARTESIAN_POINT('Ctrl Pts',(-21.,8.42515810469916,5.93194523247474));
#56578=CARTESIAN_POINT('Ctrl Pts',(-50.,8.07954770829655,6.40614484298506));
#56579=CARTESIAN_POINT('Ctrl Pts',(-21.,8.07954770829655,6.40614484298506));
#56580=CARTESIAN_POINT('Ctrl Pts',(-50.,7.65606629865851,6.96043017782053));
#56581=CARTESIAN_POINT('Ctrl Pts',(-21.,7.65606629865851,6.96043017782053));
#56582=CARTESIAN_POINT('Ctrl Pts',(-50.,7.25490905174796,7.46802385431575));
#56583=CARTESIAN_POINT('Ctrl Pts',(-21.,7.25490905174796,7.46802385431575));
#56584=CARTESIAN_POINT('Ctrl Pts',(-50.,6.91903663131433,7.8847336425335));
#56585=CARTESIAN_POINT('Ctrl Pts',(-21.,6.91903663131433,7.8847336425335));
#56586=CARTESIAN_POINT('Ctrl Pts',(-50.,6.67958481505646,8.17852534961222));
#56587=CARTESIAN_POINT('Ctrl Pts',(-21.,6.67958481505646,8.17852534961222));
#56588=CARTESIAN_POINT('Ctrl Pts',(-50.,6.55597468860601,8.32941749958287));
#56589=CARTESIAN_POINT('Ctrl Pts',(-21.,6.55597468860601,8.32941749958287));
#56590=CARTESIAN_POINT('',(-21.5,8.85937132577942,4.63805343996351));
#56591=CARTESIAN_POINT('Ctrl Pts',(-21.5,8.85937132577942,4.63805343996351));
#56592=CARTESIAN_POINT('Ctrl Pts',(-21.4716714037526,8.82699312116116,4.63882198977594));
#56593=CARTESIAN_POINT('Ctrl Pts',(-21.4424150110737,8.79205190661356,4.64240188595715));
#56594=CARTESIAN_POINT('Ctrl Pts',(-21.2909879716439,8.6069526617269,4.66814581613095));
#56595=CARTESIAN_POINT('Ctrl Pts',(-21.1630186724939,8.43596084926503,4.71373942955312));
#56596=CARTESIAN_POINT('Ctrl Pts',(-21.,8.24274231917123,4.72304976257329));
#56597=CARTESIAN_POINT('Ctrl Pts',(-50.,8.85937132577942,4.63805343996351));
#56598=CARTESIAN_POINT('Ctrl Pts',(-45.1666666666667,8.85937132577942,4.63805343996351));
#56599=CARTESIAN_POINT('Ctrl Pts',(-40.3333333333333,8.85937132577942,4.63805343996351));
#56600=CARTESIAN_POINT('Ctrl Pts',(-30.8333333333333,8.85937132577942,4.63805343996351));
#56601=CARTESIAN_POINT('Ctrl Pts',(-26.1666666666667,8.85937132577942,4.63805343996351));
#56602=CARTESIAN_POINT('Ctrl Pts',(-21.5,8.85937132577942,4.63805343996351));
#56603=CARTESIAN_POINT('Origin',(-21.25,0.,0.));
#56604=CARTESIAN_POINT('Origin',(-21.5,0.,0.));
#56605=CARTESIAN_POINT('Origin',(-35.75,0.,0.));
#56606=CARTESIAN_POINT('Ctrl Pts',(-50.,9.52072790258051,4.66001504343333));
#56607=CARTESIAN_POINT('Ctrl Pts',(-21.,9.52072790258051,4.66001504343333));
#56608=CARTESIAN_POINT('Ctrl Pts',(-50.,9.5106844305395,4.6383460245682));
#56609=CARTESIAN_POINT('Ctrl Pts',(-21.,9.5106844305395,4.6383460245682));
#56610=CARTESIAN_POINT('Ctrl Pts',(-50.,9.49044302111884,4.59516580583826));
#56611=CARTESIAN_POINT('Ctrl Pts',(-21.,9.49044302111884,4.59516580583826));
#56612=CARTESIAN_POINT('Ctrl Pts',(-50.,9.45961751095234,4.53086893560887));
#56613=CARTESIAN_POINT('Ctrl Pts',(-21.,9.45961751095234,4.53086893560887));
#56614=CARTESIAN_POINT('Ctrl Pts',(-50.,9.41758880635275,4.44608794271298));
#56615=CARTESIAN_POINT('Ctrl Pts',(-21.,9.41758880635275,4.44608794271298));
#56616=CARTESIAN_POINT('Ctrl Pts',(-50.,9.36349807041911,4.34170493100677));
#56617=CARTESIAN_POINT('Ctrl Pts',(-21.,9.36349807041911,4.34170493100677));
#56618=CARTESIAN_POINT('Ctrl Pts',(-50.,9.30784049378005,4.23894115315102));
#56619=CARTESIAN_POINT('Ctrl Pts',(-21.,9.30784049378005,4.23894115315102));
#56620=CARTESIAN_POINT('Ctrl Pts',(-50.,9.25060154420976,4.1378392686224));
#56621=CARTESIAN_POINT('Ctrl Pts',(-21.,9.25060154420976,4.1378392686224));
#56622=CARTESIAN_POINT('Ctrl Pts',(-50.,9.19176567419237,4.03846112001482));
#56623=CARTESIAN_POINT('Ctrl Pts',(-21.,9.19176567419237,4.03846112001482));
#56624=CARTESIAN_POINT('Ctrl Pts',(-50.,9.13131768087278,3.94089272529988));
#56625=CARTESIAN_POINT('Ctrl Pts',(-21.,9.13131768087278,3.94089272529988));
#56626=CARTESIAN_POINT('Ctrl Pts',(-50.,9.06924587952332,3.84523375831808));
#56627=CARTESIAN_POINT('Ctrl Pts',(-21.,9.06924587952332,3.84523375831808));
#56628=CARTESIAN_POINT('Ctrl Pts',(-50.,9.0055455660548,3.75158344307814));
#56629=CARTESIAN_POINT('Ctrl Pts',(-21.,9.0055455660548,3.75158344307814));
#56630=CARTESIAN_POINT('Ctrl Pts',(-50.,8.94022316573707,3.66002610520606));
#56631=CARTESIAN_POINT('Ctrl Pts',(-21.,8.94022316573707,3.66002610520606));
#56632=CARTESIAN_POINT('Ctrl Pts',(-50.,8.87329906122102,3.57061962548306));
#56633=CARTESIAN_POINT('Ctrl Pts',(-21.,8.87329906122102,3.57061962548306));
#56634=CARTESIAN_POINT('Ctrl Pts',(-50.,8.80481446318767,3.48337462556297));
#56635=CARTESIAN_POINT('Ctrl Pts',(-21.,8.80481446318767,3.48337462556297));
#56636=CARTESIAN_POINT('Ctrl Pts',(-50.,8.7348214836506,3.3982738856883));
#56637=CARTESIAN_POINT('Ctrl Pts',(-21.,8.7348214836506,3.3982738856883));
#56638=CARTESIAN_POINT('Ctrl Pts',(-50.,8.66336443667969,3.31531333416059));
#56639=CARTESIAN_POINT('Ctrl Pts',(-21.,8.66336443667969,3.31531333416059));
#56640=CARTESIAN_POINT('Ctrl Pts',(-50.,8.59046276963722,3.23453838205034));
#56641=CARTESIAN_POINT('Ctrl Pts',(-21.,8.59046276963722,3.23453838205034));
#56642=CARTESIAN_POINT('Ctrl Pts',(-50.,8.51609606529771,3.15607730017284));
#56643=CARTESIAN_POINT('Ctrl Pts',(-21.,8.51609606529771,3.15607730017284));
#56644=CARTESIAN_POINT('Ctrl Pts',(-50.,8.44018147897284,3.08018804824792));
#56645=CARTESIAN_POINT('Ctrl Pts',(-21.,8.44018147897284,3.08018804824792));
#56646=CARTESIAN_POINT('Ctrl Pts',(-50.,8.36258324333989,3.00724707660037));
#56647=CARTESIAN_POINT('Ctrl Pts',(-21.,8.36258324333989,3.00724707660037));
#56648=CARTESIAN_POINT('Ctrl Pts',(-50.,8.28314562863609,2.93769454582461));
#56649=CARTESIAN_POINT('Ctrl Pts',(-21.,8.28314562863609,2.93769454582461));
#56650=CARTESIAN_POINT('Ctrl Pts',(-50.,8.201719906256,2.87199246251599));
#56651=CARTESIAN_POINT('Ctrl Pts',(-21.,8.201719906256,2.87199246251599));
#56652=CARTESIAN_POINT('Ctrl Pts',(-50.,8.11819217840571,2.81057710920625));
#56653=CARTESIAN_POINT('Ctrl Pts',(-21.,8.11819217840571,2.81057710920625));
#56654=CARTESIAN_POINT('Ctrl Pts',(-50.,8.03251572538561,2.75381386341092));
#56655=CARTESIAN_POINT('Ctrl Pts',(-21.,8.03251572538561,2.75381386341092));
#56656=CARTESIAN_POINT('Ctrl Pts',(-50.,7.94472127708621,2.70194887521209));
#56657=CARTESIAN_POINT('Ctrl Pts',(-21.,7.94472127708621,2.70194887521209));
#56658=CARTESIAN_POINT('Ctrl Pts',(-50.,7.85491172665132,2.65506217582471));
#56659=CARTESIAN_POINT('Ctrl Pts',(-21.,7.85491172665132,2.65506217582471));
#56660=CARTESIAN_POINT('Ctrl Pts',(-50.,7.76326299008741,2.61301442971916));
#56661=CARTESIAN_POINT('Ctrl Pts',(-21.,7.76326299008741,2.61301442971916));
#56662=CARTESIAN_POINT('Ctrl Pts',(-50.,7.67002106404108,2.5754046559055));
#56663=CARTESIAN_POINT('Ctrl Pts',(-21.,7.67002106404108,2.5754046559055));
#56664=CARTESIAN_POINT('Ctrl Pts',(-50.,7.57550619462173,2.54149568187359));
#56665=CARTESIAN_POINT('Ctrl Pts',(-21.,7.57550619462173,2.54149568187359));
#56666=CARTESIAN_POINT('Ctrl Pts',(-50.,7.4800863304027,2.5103005111467));
#56667=CARTESIAN_POINT('Ctrl Pts',(-21.,7.4800863304027,2.5103005111467));
#56668=CARTESIAN_POINT('Ctrl Pts',(-50.,7.3841397096708,2.4807280346756));
#56669=CARTESIAN_POINT('Ctrl Pts',(-21.,7.3841397096708,2.4807280346756));
#56670=CARTESIAN_POINT('Ctrl Pts',(-50.,7.28802033430286,2.45171132733138));
#56671=CARTESIAN_POINT('Ctrl Pts',(-21.,7.28802033430286,2.45171132733138));
#56672=CARTESIAN_POINT('Ctrl Pts',(-50.,7.19202414084635,2.42233623016115));
#56673=CARTESIAN_POINT('Ctrl Pts',(-21.,7.19202414084635,2.42233623016115));
#56674=CARTESIAN_POINT('Ctrl Pts',(-50.,7.09634961812101,2.39198792562662));
#56675=CARTESIAN_POINT('Ctrl Pts',(-21.,7.09634961812101,2.39198792562662));
#56676=CARTESIAN_POINT('Ctrl Pts',(-50.,7.00111274457534,2.36030757076476));
#56677=CARTESIAN_POINT('Ctrl Pts',(-21.,7.00111274457534,2.36030757076476));
#56678=CARTESIAN_POINT('Ctrl Pts',(-50.,6.92531873868941,2.33375705829959));
#56679=CARTESIAN_POINT('Ctrl Pts',(-21.,6.92531873868941,2.33375705829959));
#56680=CARTESIAN_POINT('Ctrl Pts',(-50.,6.86870350660446,2.31314148102898));
#56681=CARTESIAN_POINT('Ctrl Pts',(-21.,6.86870350660446,2.31314148102898));
#56682=CARTESIAN_POINT('Ctrl Pts',(-50.,6.8310622341282,2.29908584041335));
#56683=CARTESIAN_POINT('Ctrl Pts',(-21.,6.8310622341282,2.29908584041335));
#56684=CARTESIAN_POINT('Ctrl Pts',(-50.,6.8122671513043,2.29198004120026));
#56685=CARTESIAN_POINT('Ctrl Pts',(-21.,6.8122671513043,2.29198004120026));
#56686=CARTESIAN_POINT('',(-21.5,9.16615635178499,3.9976965535958));
#56687=CARTESIAN_POINT('Ctrl Pts',(-21.,8.82694180863381,3.51213586112389));
#56688=CARTESIAN_POINT('Ctrl Pts',(-21.1171767610705,8.91085623417581,3.61818855775461));
#56689=CARTESIAN_POINT('Ctrl Pts',(-21.2874825276219,9.03028230496099,3.77763683804508));
#56690=CARTESIAN_POINT('Ctrl Pts',(-21.5,9.16615635178498,3.9976965535958));
#56691=CARTESIAN_POINT('',(-50.,6.8122671513043,2.29198004120026));
#56692=CARTESIAN_POINT('Ctrl Pts',(-21.5,9.16615635178499,3.9976965535958));
#56693=CARTESIAN_POINT('Ctrl Pts',(-26.3333333333333,9.16615635178499,3.9976965535958));
#56694=CARTESIAN_POINT('Ctrl Pts',(-31.1666666666667,9.16615635178499,3.9976965535958));
#56695=CARTESIAN_POINT('Ctrl Pts',(-40.6666666666667,9.16615635178499,3.9976965535958));
#56696=CARTESIAN_POINT('Ctrl Pts',(-45.3333333333333,9.16615635178499,3.9976965535958));
#56697=CARTESIAN_POINT('Ctrl Pts',(-50.,9.16615635178499,3.9976965535958));
#56698=CARTESIAN_POINT('Origin',(-50.,0.,0.));
#56699=CARTESIAN_POINT('',(-50.,7.13209349341826,0.890729280500491));
#56700=CARTESIAN_POINT('Ctrl Pts',(-50.,7.13209349341826,0.890729280500491));
#56701=CARTESIAN_POINT('Ctrl Pts',(-21.,7.13209349341826,0.890729280500491));
#56702=CARTESIAN_POINT('Ctrl Pts',(-50.,7.15577920638447,0.893054239868309));
#56703=CARTESIAN_POINT('Ctrl Pts',(-21.,7.15577920638447,0.893054239868309));
#56704=CARTESIAN_POINT('Ctrl Pts',(-50.,7.20314083161155,0.897868938540711));
#56705=CARTESIAN_POINT('Ctrl Pts',(-21.,7.20314083161155,0.897868938540711));
#56706=CARTESIAN_POINT('Ctrl Pts',(-50.,7.27415386726379,0.90558533966873));
#56707=CARTESIAN_POINT('Ctrl Pts',(-21.,7.27415386726379,0.90558533966873));
#56708=CARTESIAN_POINT('Ctrl Pts',(-50.,7.36877903277666,0.916863781503487));
#56709=CARTESIAN_POINT('Ctrl Pts',(-21.,7.36877903277666,0.916863781503487));
#56710=CARTESIAN_POINT('Ctrl Pts',(-50.,7.4869674381447,0.932516236860827));
#56711=CARTESIAN_POINT('Ctrl Pts',(-21.,7.4869674381447,0.932516236860827));
#56712=CARTESIAN_POINT('Ctrl Pts',(-50.,7.60507887157754,0.949420915891057));
#56713=CARTESIAN_POINT('Ctrl Pts',(-21.,7.60507887157754,0.949420915891057));
#56714=CARTESIAN_POINT('Ctrl Pts',(-50.,7.72314614047142,0.966965984543333));
#56715=CARTESIAN_POINT('Ctrl Pts',(-21.,7.72314614047142,0.966965984543333));
#56716=CARTESIAN_POINT('Ctrl Pts',(-50.,7.84122460090589,0.984110042106143));
#56717=CARTESIAN_POINT('Ctrl Pts',(-21.,7.84122460090589,0.984110042106143));
#56718=CARTESIAN_POINT('Ctrl Pts',(-50.,7.95940371279084,0.999455440216893));
#56719=CARTESIAN_POINT('Ctrl Pts',(-21.,7.95940371279084,0.999455440216893));
#56720=CARTESIAN_POINT('Ctrl Pts',(-50.,8.0778221648407,1.01133055607812));
#56721=CARTESIAN_POINT('Ctrl Pts',(-21.,8.0778221648407,1.01133055607812));
#56722=CARTESIAN_POINT('Ctrl Pts',(-50.,8.19667636355292,1.01788199103989));
#56723=CARTESIAN_POINT('Ctrl Pts',(-21.,8.19667636355292,1.01788199103989));
#56724=CARTESIAN_POINT('Ctrl Pts',(-50.,8.31624650623966,1.017123671327));
#56725=CARTESIAN_POINT('Ctrl Pts',(-21.,8.31624650623966,1.017123671327));
#56726=CARTESIAN_POINT('Ctrl Pts',(-50.,8.43677899171613,1.00737622330388));
#56727=CARTESIAN_POINT('Ctrl Pts',(-21.,8.43677899171613,1.00737622330388));
#56728=CARTESIAN_POINT('Ctrl Pts',(-50.,8.55832200571467,0.987849802439111));
#56729=CARTESIAN_POINT('Ctrl Pts',(-21.,8.55832200571467,0.987849802439111));
#56730=CARTESIAN_POINT('Ctrl Pts',(-50.,8.68060673111004,0.95907349496179));
#56731=CARTESIAN_POINT('Ctrl Pts',(-21.,8.68060673111004,0.95907349496179));
#56732=CARTESIAN_POINT('Ctrl Pts',(-50.,8.80283221651881,0.923666931425907));
#56733=CARTESIAN_POINT('Ctrl Pts',(-21.,8.80283221651881,0.923666931425907));
#56734=CARTESIAN_POINT('Ctrl Pts',(-50.,8.92394083882956,0.885365181899305));
#56735=CARTESIAN_POINT('Ctrl Pts',(-21.,8.92394083882956,0.885365181899305));
#56736=CARTESIAN_POINT('Ctrl Pts',(-50.,9.04313782728701,0.847184879177382));
#56737=CARTESIAN_POINT('Ctrl Pts',(-21.,9.04313782728701,0.847184879177382));
#56738=CARTESIAN_POINT('Ctrl Pts',(-50.,9.1602494406401,0.810145236641718));
#56739=CARTESIAN_POINT('Ctrl Pts',(-21.,9.1602494406401,0.810145236641718));
#56740=CARTESIAN_POINT('Ctrl Pts',(-50.,9.27634845263042,0.771090641047727));
#56741=CARTESIAN_POINT('Ctrl Pts',(-21.,9.27634845263042,0.771090641047727));
#56742=CARTESIAN_POINT('Ctrl Pts',(-50.,9.39347368681776,0.723542272923875));
#56743=CARTESIAN_POINT('Ctrl Pts',(-21.,9.39347368681776,0.723542272923875));
#56744=CARTESIAN_POINT('Ctrl Pts',(-50.,9.51346503399365,0.661496920442432));
#56745=CARTESIAN_POINT('Ctrl Pts',(-21.,9.51346503399365,0.661496920442432));
#56746=CARTESIAN_POINT('Ctrl Pts',(-50.,9.63711058491003,0.582194086890199));
#56747=CARTESIAN_POINT('Ctrl Pts',(-21.,9.63711058491003,0.582194086890199));
#56748=CARTESIAN_POINT('Ctrl Pts',(-50.,9.76300600524289,0.489818901108929));
#56749=CARTESIAN_POINT('Ctrl Pts',(-21.,9.76300600524289,0.489818901108929));
#56750=CARTESIAN_POINT('Ctrl Pts',(-50.,9.88700914008587,0.397288908358525));
#56751=CARTESIAN_POINT('Ctrl Pts',(-21.,9.88700914008587,0.397288908358525));
#56752=CARTESIAN_POINT('Ctrl Pts',(-50.,10.0034077194239,0.322542614674784));
#56753=CARTESIAN_POINT('Ctrl Pts',(-21.,10.0034077194239,0.322542614674784));
#56754=CARTESIAN_POINT('Ctrl Pts',(-50.,10.1057999094475,0.285750111589545));
#56755=CARTESIAN_POINT('Ctrl Pts',(-21.,10.1057999094475,0.285750111589545));
#56756=CARTESIAN_POINT('Ctrl Pts',(-50.,10.1880600728826,0.306249742693306));
#56757=CARTESIAN_POINT('Ctrl Pts',(-21.,10.1880600728826,0.306249742693306));
#56758=CARTESIAN_POINT('Ctrl Pts',(-50.,10.2453310344199,0.399403984752718));
#56759=CARTESIAN_POINT('Ctrl Pts',(-21.,10.2453310344199,0.399403984752718));
#56760=CARTESIAN_POINT('Ctrl Pts',(-50.,10.2739254957461,0.576902635874919));
#56761=CARTESIAN_POINT('Ctrl Pts',(-21.,10.2739254957461,0.576902635874919));
#56762=CARTESIAN_POINT('Ctrl Pts',(-50.,10.2711360438186,0.847355944984259));
#56763=CARTESIAN_POINT('Ctrl Pts',(-21.,10.2711360438186,0.847355944984259));
#56764=CARTESIAN_POINT('Ctrl Pts',(-50.,10.23508746503,1.21675444348887));
#56765=CARTESIAN_POINT('Ctrl Pts',(-21.,10.23508746503,1.21675444348887));
#56766=CARTESIAN_POINT('Ctrl Pts',(-50.,10.1645797371964,1.68895887943845));
#56767=CARTESIAN_POINT('Ctrl Pts',(-21.,10.1645797371964,1.68895887943845));
#56768=CARTESIAN_POINT('Ctrl Pts',(-50.,10.0589430297105,2.26615269674877));
#56769=CARTESIAN_POINT('Ctrl Pts',(-21.,10.0589430297105,2.26615269674877));
#56770=CARTESIAN_POINT('Ctrl Pts',(-50.,9.91789485710769,2.94928822483092));
#56771=CARTESIAN_POINT('Ctrl Pts',(-21.,9.91789485710769,2.94928822483092));
#56772=CARTESIAN_POINT('Ctrl Pts',(-50.,9.77670130881801,3.5806699311609));
#56773=CARTESIAN_POINT('Ctrl Pts',(-21.,9.77670130881801,3.5806699311609));
#56774=CARTESIAN_POINT('Ctrl Pts',(-50.,9.65489431545908,4.10184205893951));
#56775=CARTESIAN_POINT('Ctrl Pts',(-21.,9.65489431545908,4.10184205893951));
#56776=CARTESIAN_POINT('Ctrl Pts',(-50.,9.56662712803709,4.47043349004179));
#56777=CARTESIAN_POINT('Ctrl Pts',(-21.,9.56662712803709,4.47043349004179));
#56778=CARTESIAN_POINT('Ctrl Pts',(-50.,9.52072790258051,4.66001504343333));
#56779=CARTESIAN_POINT('Ctrl Pts',(-21.,9.52072790258051,4.66001504343333));
#56780=CARTESIAN_POINT('Ctrl Pts',(-66.,13.847248627403,-2.45104298226008));
#56781=CARTESIAN_POINT('Ctrl Pts',(-50.,13.847248627403,-2.45104298226008));
#56782=CARTESIAN_POINT('Ctrl Pts',(-66.,13.8704109184829,-2.45416751351779));
#56783=CARTESIAN_POINT('Ctrl Pts',(-50.,13.8704109184829,-2.45416751351779));
#56784=CARTESIAN_POINT('Ctrl Pts',(-66.,13.9167144589915,-2.46064068498796));
#56785=CARTESIAN_POINT('Ctrl Pts',(-50.,13.9167144589915,-2.46064068498796));
#56786=CARTESIAN_POINT('Ctrl Pts',(-66.,13.9861066530346,-2.47102275853729));
#56787=CARTESIAN_POINT('Ctrl Pts',(-50.,13.9861066530346,-2.47102275853729));
#56788=CARTESIAN_POINT('Ctrl Pts',(-66.,14.0785031060049,-2.48621203480011));
#56789=CARTESIAN_POINT('Ctrl Pts',(-50.,14.0785031060049,-2.48621203480011));
#56790=CARTESIAN_POINT('Ctrl Pts',(-66.,14.1937640331043,-2.50749463728168));
#56791=CARTESIAN_POINT('Ctrl Pts',(-50.,14.1937640331043,-2.50749463728168));
#56792=CARTESIAN_POINT('Ctrl Pts',(-66.,14.3087190397278,-2.53121250086624));
#56793=CARTESIAN_POINT('Ctrl Pts',(-50.,14.3087190397278,-2.53121250086624));
#56794=CARTESIAN_POINT('Ctrl Pts',(-66.,14.423228955274,-2.55762788131115));
#56795=CARTESIAN_POINT('Ctrl Pts',(-50.,14.423228955274,-2.55762788131115));
#56796=CARTESIAN_POINT('Ctrl Pts',(-66.,14.537056384215,-2.58717382256056));
#56797=CARTESIAN_POINT('Ctrl Pts',(-50.,14.537056384215,-2.58717382256056));
#56798=CARTESIAN_POINT('Ctrl Pts',(-66.,14.6499173448672,-2.62041096375855));
#56799=CARTESIAN_POINT('Ctrl Pts',(-50.,14.6499173448672,-2.62041096375855));
#56800=CARTESIAN_POINT('Ctrl Pts',(-66.,14.7615516365331,-2.65797355871958));
#56801=CARTESIAN_POINT('Ctrl Pts',(-50.,14.7615516365331,-2.65797355871958));
#56802=CARTESIAN_POINT('Ctrl Pts',(-66.,14.8717795409674,-2.70050907188802));
#56803=CARTESIAN_POINT('Ctrl Pts',(-50.,14.8717795409674,-2.70050907188802));
#56804=CARTESIAN_POINT('Ctrl Pts',(-66.,14.9805825983482,-2.74864579544975));
#56805=CARTESIAN_POINT('Ctrl Pts',(-50.,14.9805825983482,-2.74864579544975));
#56806=CARTESIAN_POINT('Ctrl Pts',(-66.,15.0880810351184,-2.80279667637514));
#56807=CARTESIAN_POINT('Ctrl Pts',(-50.,15.0880810351184,-2.80279667637514));
#56808=CARTESIAN_POINT('Ctrl Pts',(-66.,15.1944599098748,-2.86283428974206));
#56809=CARTESIAN_POINT('Ctrl Pts',(-50.,15.1944599098748,-2.86283428974206));
#56810=CARTESIAN_POINT('Ctrl Pts',(-66.,15.299916309402,-2.9278833773088));
#56811=CARTESIAN_POINT('Ctrl Pts',(-50.,15.299916309402,-2.9278833773088));
#56812=CARTESIAN_POINT('Ctrl Pts',(-66.,15.4045879562307,-2.99587287520288));
#56813=CARTESIAN_POINT('Ctrl Pts',(-50.,15.4045879562307,-2.99587287520288));
#56814=CARTESIAN_POINT('Ctrl Pts',(-66.,15.5085273245779,-3.06389197726713));
#56815=CARTESIAN_POINT('Ctrl Pts',(-50.,15.5085273245779,-3.06389197726713));
#56816=CARTESIAN_POINT('Ctrl Pts',(-66.,15.6117260024113,-3.1296030647124));
#56817=CARTESIAN_POINT('Ctrl Pts',(-50.,15.6117260024113,-3.1296030647124));
#56818=CARTESIAN_POINT('Ctrl Pts',(-66.,15.7141266693079,-3.19226978910788));
#56819=CARTESIAN_POINT('Ctrl Pts',(-50.,15.7141266693079,-3.19226978910788));
#56820=CARTESIAN_POINT('Ctrl Pts',(-66.,15.8156387361042,-3.25420659877988));
#56821=CARTESIAN_POINT('Ctrl Pts',(-50.,15.8156387361042,-3.25420659877988));
#56822=CARTESIAN_POINT('Ctrl Pts',(-66.,15.9161557197846,-3.32129162127238));
#56823=CARTESIAN_POINT('Ctrl Pts',(-50.,15.9161557197846,-3.32129162127238));
#56824=CARTESIAN_POINT('Ctrl Pts',(-66.,16.0155897253002,-3.39971935742472));
#56825=CARTESIAN_POINT('Ctrl Pts',(-50.,16.0155897253002,-3.39971935742472));
#56826=CARTESIAN_POINT('Ctrl Pts',(-66.,16.1139042055915,-3.49322345403937));
#56827=CARTESIAN_POINT('Ctrl Pts',(-50.,16.1139042055915,-3.49322345403937));
#56828=CARTESIAN_POINT('Ctrl Pts',(-66.,16.211146002486,-3.60024269640763));
#56829=CARTESIAN_POINT('Ctrl Pts',(-50.,16.211146002486,-3.60024269640763));
#56830=CARTESIAN_POINT('Ctrl Pts',(-66.,16.3074829231181,-3.71072189651349));
#56831=CARTESIAN_POINT('Ctrl Pts',(-50.,16.3074829231181,-3.71072189651349));
#56832=CARTESIAN_POINT('Ctrl Pts',(-66.,16.4031678857067,-3.80856758682422));
#56833=CARTESIAN_POINT('Ctrl Pts',(-50.,16.4031678857067,-3.80856758682422));
#56834=CARTESIAN_POINT('Ctrl Pts',(-66.,16.4984944917342,-3.87477327683275));
#56835=CARTESIAN_POINT('Ctrl Pts',(-50.,16.4984944917342,-3.87477327683275));
#56836=CARTESIAN_POINT('Ctrl Pts',(-66.,16.5937589714353,-3.89007667331238));
#56837=CARTESIAN_POINT('Ctrl Pts',(-50.,16.5937589714353,-3.89007667331238));
#56838=CARTESIAN_POINT('Ctrl Pts',(-66.,16.68921248971,-3.83831350468403));
#56839=CARTESIAN_POINT('Ctrl Pts',(-50.,16.68921248971,-3.83831350468403));
#56840=CARTESIAN_POINT('Ctrl Pts',(-66.,16.7850480556278,-3.70731931187133));
#56841=CARTESIAN_POINT('Ctrl Pts',(-50.,16.7850480556278,-3.70731931187133));
#56842=CARTESIAN_POINT('Ctrl Pts',(-66.,16.8814129124086,-3.48803104347221));
#56843=CARTESIAN_POINT('Ctrl Pts',(-50.,16.8814129124086,-3.48803104347221));
#56844=CARTESIAN_POINT('Ctrl Pts',(-66.,16.9784132750883,-3.17413405024117));
#56845=CARTESIAN_POINT('Ctrl Pts',(-50.,16.9784132750883,-3.17413405024117));
#56846=CARTESIAN_POINT('Ctrl Pts',(-66.,17.0761219213447,-2.76151077690173));
#56847=CARTESIAN_POINT('Ctrl Pts',(-50.,17.0761219213447,-2.76151077690173));
#56848=CARTESIAN_POINT('Ctrl Pts',(-66.,17.1745842847512,-2.24779890242269));
#56849=CARTESIAN_POINT('Ctrl Pts',(-50.,17.1745842847512,-2.24779890242269));
#56850=CARTESIAN_POINT('Ctrl Pts',(-66.,17.2738249451951,-1.6319247049175));
#56851=CARTESIAN_POINT('Ctrl Pts',(-50.,17.2738249451951,-1.6319247049175));
#56852=CARTESIAN_POINT('Ctrl Pts',(-66.,17.3538479729472,-1.05731872182051));
#56853=CARTESIAN_POINT('Ctrl Pts',(-50.,17.3538479729472,-1.05731872182051));
#56854=CARTESIAN_POINT('Ctrl Pts',(-66.,17.4142204208888,-0.580381911529879));
#56855=CARTESIAN_POINT('Ctrl Pts',(-50.,17.4142204208888,-0.580381911529879));
#56856=CARTESIAN_POINT('Ctrl Pts',(-66.,17.4546263659151,-0.242014631789217));
#56857=CARTESIAN_POINT('Ctrl Pts',(-50.,17.4546263659151,-0.242014631789217));
#56858=CARTESIAN_POINT('Ctrl Pts',(-66.,17.4748687500531,-0.0677286381032094));
#56859=CARTESIAN_POINT('Ctrl Pts',(-50.,17.4748687500531,-0.0677286381032094));
#56860=CARTESIAN_POINT('',(-65.5,16.4355406675768,-3.82604599612027));
#56861=CARTESIAN_POINT('Ctrl Pts',(-66.,16.017075735697,-3.40498309495743));
#56862=CARTESIAN_POINT('Ctrl Pts',(-65.7933280154027,16.1952885331162,-3.5605803063597));
#56863=CARTESIAN_POINT('Ctrl Pts',(-65.6370761749495,16.3149639463236,-3.73942475662406));
#56864=CARTESIAN_POINT('Ctrl Pts',(-65.5,16.4355406675768,-3.82604599612027));
#56865=CARTESIAN_POINT('',(-66.,13.847248627403,-2.45104298226008));
#56866=CARTESIAN_POINT('',(-50.5,16.4355406675768,-3.82604599612027));
#56867=CARTESIAN_POINT('Ctrl Pts',(-50.5,16.4355406675768,-3.82604599612027));
#56868=CARTESIAN_POINT('Ctrl Pts',(-50.4948519989264,16.4310123161643,-3.82279286891502));
#56869=CARTESIAN_POINT('Ctrl Pts',(-50.4896830984798,16.4264908162217,-3.81941633340717));
#56870=CARTESIAN_POINT('Ctrl Pts',(-50.3487582866786,16.3038396642987,-3.72461708742528));
#56871=CARTESIAN_POINT('Ctrl Pts',(-50.1996600197157,16.1892421312326,-3.55530120583648));
#56872=CARTESIAN_POINT('Ctrl Pts',(-50.,16.017075735697,-3.40498309495743));
#56873=CARTESIAN_POINT('Ctrl Pts',(-65.5,16.4355406675768,-3.82604599612027));
#56874=CARTESIAN_POINT('Ctrl Pts',(-60.5,16.4355406675768,-3.82604599612027));
#56875=CARTESIAN_POINT('Ctrl Pts',(-55.5,16.4355406675768,-3.82604599612027));
#56876=CARTESIAN_POINT('Ctrl Pts',(-50.5,16.4355406675768,-3.82604599612027));
#56877=CARTESIAN_POINT('Origin',(-66.,0.,0.));
#56878=CARTESIAN_POINT('',(-66.,14.0217614511585,-1.06963173887292));
#56879=CARTESIAN_POINT('Ctrl Pts',(-66.,17.4748687500531,-0.0677286381032094));
#56880=CARTESIAN_POINT('Ctrl Pts',(-50.,17.4748687500531,-0.0677286381032094));
#56881=CARTESIAN_POINT('Ctrl Pts',(-66.,17.4559219893477,-0.0798814582063345));
#56882=CARTESIAN_POINT('Ctrl Pts',(-50.,17.4559219893477,-0.0798814582063345));
#56883=CARTESIAN_POINT('Ctrl Pts',(-66.,17.4179952684683,-0.104043012351033));
#56884=CARTESIAN_POINT('Ctrl Pts',(-50.,17.4179952684683,-0.104043012351033));
#56885=CARTESIAN_POINT('Ctrl Pts',(-66.,17.3610055888369,-0.139853086053525));
#56886=CARTESIAN_POINT('Ctrl Pts',(-50.,17.3610055888369,-0.139853086053525));
#56887=CARTESIAN_POINT('Ctrl Pts',(-66.,17.2848198869808,-0.186734180470151));
#56888=CARTESIAN_POINT('Ctrl Pts',(-50.,17.2848198869808,-0.186734180470151));
#56889=CARTESIAN_POINT('Ctrl Pts',(-66.,17.1892542640251,-0.24388678747065));
#56890=CARTESIAN_POINT('Ctrl Pts',(-50.,17.1892542640251,-0.24388678747065));
#56891=CARTESIAN_POINT('Ctrl Pts',(-66.,17.0933546347573,-0.299584219228362));
#56892=CARTESIAN_POINT('Ctrl Pts',(-50.,17.0933546347573,-0.299584219228362));
#56893=CARTESIAN_POINT('Ctrl Pts',(-66.,16.9971220426505,-0.353822666243593));
#56894=CARTESIAN_POINT('Ctrl Pts',(-50.,16.9971220426505,-0.353822666243593));
#56895=CARTESIAN_POINT('Ctrl Pts',(-66.,16.9005600486991,-0.406603490394105));
#56896=CARTESIAN_POINT('Ctrl Pts',(-50.,16.9005600486991,-0.406603490394105));
#56897=CARTESIAN_POINT('Ctrl Pts',(-66.,16.8036759306869,-0.457937485755119));
#56898=CARTESIAN_POINT('Ctrl Pts',(-50.,16.8036759306869,-0.457937485755119));
#56899=CARTESIAN_POINT('Ctrl Pts',(-66.,16.7064800689097,-0.507835335884597));
#56900=CARTESIAN_POINT('Ctrl Pts',(-50.,16.7064800689097,-0.507835335884597));
#56901=CARTESIAN_POINT('Ctrl Pts',(-66.,16.608985095069,-0.556296581714668));
#56902=CARTESIAN_POINT('Ctrl Pts',(-50.,16.608985095069,-0.556296581714668));
#56903=CARTESIAN_POINT('Ctrl Pts',(-66.,16.5112051709817,-0.603298348866388));
#56904=CARTESIAN_POINT('Ctrl Pts',(-50.,16.5112051709817,-0.603298348866388));
#56905=CARTESIAN_POINT('Ctrl Pts',(-66.,16.4131552634766,-0.648786238597103));
#56906=CARTESIAN_POINT('Ctrl Pts',(-50.,16.4131552634766,-0.648786238597103));
#56907=CARTESIAN_POINT('Ctrl Pts',(-66.,16.3148504473396,-0.692659157159194));
#56908=CARTESIAN_POINT('Ctrl Pts',(-50.,16.3148504473396,-0.692659157159194));
#56909=CARTESIAN_POINT('Ctrl Pts',(-66.,16.2163053509993,-0.734791658433232));
#56910=CARTESIAN_POINT('Ctrl Pts',(-50.,16.2163053509993,-0.734791658433232));
#56911=CARTESIAN_POINT('Ctrl Pts',(-66.,16.1175336986507,-0.775065535573949));
#56912=CARTESIAN_POINT('Ctrl Pts',(-50.,16.1175336986507,-0.775065535573949));
#56913=CARTESIAN_POINT('Ctrl Pts',(-66.,16.018547775909,-0.813401076758624));
#56914=CARTESIAN_POINT('Ctrl Pts',(-50.,16.018547775909,-0.813401076758624));
#56915=CARTESIAN_POINT('Ctrl Pts',(-66.,15.9193580975472,-0.849783012021725));
#56916=CARTESIAN_POINT('Ctrl Pts',(-50.,15.9193580975472,-0.849783012021725));
#56917=CARTESIAN_POINT('Ctrl Pts',(-66.,15.8199726227578,-0.884304144422378));
#56918=CARTESIAN_POINT('Ctrl Pts',(-50.,15.8199726227578,-0.884304144422378));
#56919=CARTESIAN_POINT('Ctrl Pts',(-66.,15.7203984586304,-0.917113393337539));
#56920=CARTESIAN_POINT('Ctrl Pts',(-50.,15.7203984586304,-0.917113393337539));
#56921=CARTESIAN_POINT('Ctrl Pts',(-66.,15.6206443917204,-0.948332278883351));
#56922=CARTESIAN_POINT('Ctrl Pts',(-50.,15.6206443917204,-0.948332278883351));
#56923=CARTESIAN_POINT('Ctrl Pts',(-66.,15.5207233107191,-0.977976807855906));
#56924=CARTESIAN_POINT('Ctrl Pts',(-50.,15.5207233107191,-0.977976807855906));
#56925=CARTESIAN_POINT('Ctrl Pts',(-66.,15.42065441025,-1.00588830882699));
#56926=CARTESIAN_POINT('Ctrl Pts',(-50.,15.42065441025,-1.00588830882699));
#56927=CARTESIAN_POINT('Ctrl Pts',(-66.,15.3204663197849,-1.03163045186508));
#56928=CARTESIAN_POINT('Ctrl Pts',(-50.,15.3204663197849,-1.03163045186508));
#56929=CARTESIAN_POINT('Ctrl Pts',(-66.,15.2201951366894,-1.05457808085916));
#56930=CARTESIAN_POINT('Ctrl Pts',(-50.,15.2201951366894,-1.05457808085916));
#56931=CARTESIAN_POINT('Ctrl Pts',(-66.,15.1198807137451,-1.07407094658941));
#56932=CARTESIAN_POINT('Ctrl Pts',(-50.,15.1198807137451,-1.07407094658941));
#56933=CARTESIAN_POINT('Ctrl Pts',(-66.,15.0195634762927,-1.08955145679141));
#56934=CARTESIAN_POINT('Ctrl Pts',(-50.,15.0195634762927,-1.08955145679141));
#56935=CARTESIAN_POINT('Ctrl Pts',(-66.,14.9192812134642,-1.100697501046));
#56936=CARTESIAN_POINT('Ctrl Pts',(-50.,14.9192812134642,-1.100697501046));
#56937=CARTESIAN_POINT('Ctrl Pts',(-66.,14.8190654065121,-1.10759084369408));
#56938=CARTESIAN_POINT('Ctrl Pts',(-50.,14.8190654065121,-1.10759084369408));
#56939=CARTESIAN_POINT('Ctrl Pts',(-66.,14.7189411465911,-1.11063958426619));
#56940=CARTESIAN_POINT('Ctrl Pts',(-50.,14.7189411465911,-1.11063958426619));
#56941=CARTESIAN_POINT('Ctrl Pts',(-66.,14.6189280002071,-1.11043751754959));
#56942=CARTESIAN_POINT('Ctrl Pts',(-50.,14.6189280002071,-1.11043751754959));
#56943=CARTESIAN_POINT('Ctrl Pts',(-66.,14.5190405063557,-1.10764458318629));
#56944=CARTESIAN_POINT('Ctrl Pts',(-50.,14.5190405063557,-1.10764458318629));
#56945=CARTESIAN_POINT('Ctrl Pts',(-66.,14.4192887981899,-1.10286394535002));
#56946=CARTESIAN_POINT('Ctrl Pts',(-50.,14.4192887981899,-1.10286394535002));
#56947=CARTESIAN_POINT('Ctrl Pts',(-66.,14.3196790995356,-1.09650878711472));
#56948=CARTESIAN_POINT('Ctrl Pts',(-50.,14.3196790995356,-1.09650878711472));
#56949=CARTESIAN_POINT('Ctrl Pts',(-66.,14.2202146396052,-1.08882773106131));
#56950=CARTESIAN_POINT('Ctrl Pts',(-50.,14.2202146396052,-1.08882773106131));
#56951=CARTESIAN_POINT('Ctrl Pts',(-66.,14.1407601934611,-1.08172501415579));
#56952=CARTESIAN_POINT('Ctrl Pts',(-50.,14.1407601934611,-1.08172501415579));
#56953=CARTESIAN_POINT('Ctrl Pts',(-66.,14.0812352370361,-1.07587965991017));
#56954=CARTESIAN_POINT('Ctrl Pts',(-50.,14.0812352370361,-1.07587965991017));
#56955=CARTESIAN_POINT('Ctrl Pts',(-66.,14.0415811730659,-1.0717527195609));
#56956=CARTESIAN_POINT('Ctrl Pts',(-50.,14.0415811730659,-1.0717527195609));
#56957=CARTESIAN_POINT('Ctrl Pts',(-66.,14.0217614511585,-1.06963173887291));
#56958=CARTESIAN_POINT('Ctrl Pts',(-50.,14.0217614511585,-1.06963173887291));
#56959=CARTESIAN_POINT('',(-65.5,16.8697044894034,-0.422723834437671));
#56960=CARTESIAN_POINT('Ctrl Pts',(-65.5,16.8697044894034,-0.422723834437665));
#56961=CARTESIAN_POINT('Ctrl Pts',(-65.5824813699687,16.7860826756777,-0.46728689022706));
#56962=CARTESIAN_POINT('Ctrl Pts',(-65.6660554230592,16.7012035668841,-0.510709500683481));
#56963=CARTESIAN_POINT('Ctrl Pts',(-65.7497221071122,16.6161031834905,-0.552412690850408));
#56964=CARTESIAN_POINT('Ctrl Pts',(-65.8185920154888,16.5460531310298,-0.586740511037283));
#56965=CARTESIAN_POINT('Ctrl Pts',(-65.8875246877872,16.47585467524,-0.61990802303423));
#56966=CARTESIAN_POINT('Ctrl Pts',(-65.9559623561336,16.406105057495,-0.651556799133145));
#56967=CARTESIAN_POINT('Ctrl Pts',(-65.9706662645635,16.3911192752916,-0.65835657353987));
#56968=CARTESIAN_POINT('Ctrl Pts',(-65.985347323118,16.376154254472,-0.66508604655682));
#56969=CARTESIAN_POINT('Ctrl Pts',(-66.,16.3612159786808,-0.671741541784794));
#56970=CARTESIAN_POINT('',(-50.5,16.8697044894034,-0.422723834437671));
#56971=CARTESIAN_POINT('Ctrl Pts',(-50.5,16.8697044894034,-0.42272383443767));
#56972=CARTESIAN_POINT('Ctrl Pts',(-55.5,16.8697044894034,-0.42272383443767));
#56973=CARTESIAN_POINT('Ctrl Pts',(-60.5,16.8697044894034,-0.42272383443767));
#56974=CARTESIAN_POINT('Ctrl Pts',(-65.5,16.8697044894034,-0.42272383443767));
#56975=CARTESIAN_POINT('Ctrl Pts',(-50.,16.3612159786808,-0.671741541784793));
#56976=CARTESIAN_POINT('Ctrl Pts',(-50.0723811193609,16.4350078961438,-0.638864805446282));
#56977=CARTESIAN_POINT('Ctrl Pts',(-50.1454547942982,16.50945142814,-0.604185038169576));
#56978=CARTESIAN_POINT('Ctrl Pts',(-50.2185542315269,16.5838300931957,-0.568140357464802));
#56979=CARTESIAN_POINT('Ctrl Pts',(-50.3042498183568,16.6710253383469,-0.525884627705495));
#56980=CARTESIAN_POINT('Ctrl Pts',(-50.389980810899,16.7581291023942,-0.481748382293282));
#56981=CARTESIAN_POINT('Ctrl Pts',(-50.4746729118433,16.8440226549228,-0.436353334136896));
#56982=CARTESIAN_POINT('Ctrl Pts',(-50.4831259799697,16.8525956392158,-0.431822481431791));
#56983=CARTESIAN_POINT('Ctrl Pts',(-50.491568698744,16.8611566112176,-0.427279100049654));
#56984=CARTESIAN_POINT('Ctrl Pts',(-50.5,16.8697044894034,-0.422723834437666));
#56985=CARTESIAN_POINT('Origin',(-65.75,0.,0.));
#56986=CARTESIAN_POINT('',(-65.5,16.234584558964,-4.60476809381824));
#56987=CARTESIAN_POINT('Origin',(-65.5,0.,0.));
#56988=CARTESIAN_POINT('Ctrl Pts',(-65.5,16.234584558964,-4.60476809381825));
#56989=CARTESIAN_POINT('Ctrl Pts',(-65.693336649146,16.0187500351764,-4.6571980681224));
#56990=CARTESIAN_POINT('Ctrl Pts',(-65.8613255387785,15.8327432857568,-4.69365622380825));
#56991=CARTESIAN_POINT('Ctrl Pts',(-66.,15.6801429643085,-4.71950650162129));
#56992=CARTESIAN_POINT('Origin',(-58.,0.,0.));
#56993=CARTESIAN_POINT('',(-50.5,16.234584558964,-4.60476809381824));
#56994=CARTESIAN_POINT('Origin',(-50.5,0.,0.));
#56995=CARTESIAN_POINT('Ctrl Pts',(-50.5,16.234584558964,-4.60476809381824));
#56996=CARTESIAN_POINT('Ctrl Pts',(-55.5,16.234584558964,-4.60476809381824));
#56997=CARTESIAN_POINT('Ctrl Pts',(-60.5,16.234584558964,-4.60476809381825));
#56998=CARTESIAN_POINT('Ctrl Pts',(-65.5,16.234584558964,-4.60476809381825));
#56999=CARTESIAN_POINT('Origin',(-50.25,0.,0.));
#57000=CARTESIAN_POINT('Ctrl Pts',(-50.,15.6801429643085,-4.71950650162129));
#57001=CARTESIAN_POINT('Ctrl Pts',(-50.1386744612147,15.8327432857494,-4.69365622380952));
#57002=CARTESIAN_POINT('Ctrl Pts',(-50.3066633508514,16.0187500351735,-4.65719806812311));
#57003=CARTESIAN_POINT('Ctrl Pts',(-50.5,16.234584558964,-4.60476809381824));
#57004=CARTESIAN_POINT('Ctrl Pts',(-66.,12.8026622457696,-5.81770965851216));
#57005=CARTESIAN_POINT('Ctrl Pts',(-50.,12.8026622457696,-5.81770965851216));
#57006=CARTESIAN_POINT('Ctrl Pts',(-66.,12.8243198115569,-5.82649625442995));
#57007=CARTESIAN_POINT('Ctrl Pts',(-50.,12.8243198115569,-5.82649625442995));
#57008=CARTESIAN_POINT('Ctrl Pts',(-66.,12.8675588289116,-5.84428128157946));
#57009=CARTESIAN_POINT('Ctrl Pts',(-50.,12.8675588289116,-5.84428128157946));
#57010=CARTESIAN_POINT('Ctrl Pts',(-66.,12.932189022876,-5.87159432010365));
#57011=CARTESIAN_POINT('Ctrl Pts',(-50.,12.932189022876,-5.87159432010365));
#57012=CARTESIAN_POINT('Ctrl Pts',(-66.,13.0179052519711,-5.90928446078516));
#57013=CARTESIAN_POINT('Ctrl Pts',(-50.,13.0179052519711,-5.90928446078516));
#57014=CARTESIAN_POINT('Ctrl Pts',(-66.,13.124252277086,-5.95856265812867));
#57015=CARTESIAN_POINT('Ctrl Pts',(-50.,13.124252277086,-5.95856265812867));
#57016=CARTESIAN_POINT('Ctrl Pts',(-66.,13.2296973679703,-6.01012352904084));
#57017=CARTESIAN_POINT('Ctrl Pts',(-50.,13.2296973679703,-6.01012352904084));
#57018=CARTESIAN_POINT('Ctrl Pts',(-66.,13.3340405059683,-6.06418647971103));
#57019=CARTESIAN_POINT('Ctrl Pts',(-50.,13.3340405059683,-6.06418647971103));
#57020=CARTESIAN_POINT('Ctrl Pts',(-66.,13.4369440601197,-6.12111191134452));
#57021=CARTESIAN_POINT('Ctrl Pts',(-50.,13.4369440601197,-6.12111191134452));
#57022=CARTESIAN_POINT('Ctrl Pts',(-66.,13.537993545262,-6.18137222620287));
#57023=CARTESIAN_POINT('Ctrl Pts',(-50.,13.537993545262,-6.18137222620287));
#57024=CARTESIAN_POINT('Ctrl Pts',(-66.,13.6367792028716,-6.24551704256852));
#57025=CARTESIAN_POINT('Ctrl Pts',(-50.,13.6367792028716,-6.24551704256852));
#57026=CARTESIAN_POINT('Ctrl Pts',(-66.,13.7329659430228,-6.31412878948963));
#57027=CARTESIAN_POINT('Ctrl Pts',(-50.,13.7329659430228,-6.31412878948963));
#57028=CARTESIAN_POINT('Ctrl Pts',(-66.,13.8263796359301,-6.38781142942664));
#57029=CARTESIAN_POINT('Ctrl Pts',(-50.,13.8263796359301,-6.38781142942664));
#57030=CARTESIAN_POINT('Ctrl Pts',(-66.,13.9170340351662,-6.46699483496205));
#57031=CARTESIAN_POINT('Ctrl Pts',(-50.,13.9170340351662,-6.46699483496205));
#57032=CARTESIAN_POINT('Ctrl Pts',(-66.,14.0051400746611,-6.55160160666348));
#57033=CARTESIAN_POINT('Ctrl Pts',(-50.,14.0051400746611,-6.55160160666348));
#57034=CARTESIAN_POINT('Ctrl Pts',(-66.,14.0911063172293,-6.64083299762664));
#57035=CARTESIAN_POINT('Ctrl Pts',(-50.,14.0911063172293,-6.64083299762664));
#57036=CARTESIAN_POINT('Ctrl Pts',(-66.,14.1755812112355,-6.73271726045961));
#57037=CARTESIAN_POINT('Ctrl Pts',(-50.,14.1755812112355,-6.73271726045961));
#57038=CARTESIAN_POINT('Ctrl Pts',(-66.,14.2593394703776,-6.8244480871404));
#57039=CARTESIAN_POINT('Ctrl Pts',(-50.,14.2593394703776,-6.8244480871404));
#57040=CARTESIAN_POINT('Ctrl Pts',(-66.,14.3429542890555,-6.9137592074853));
#57041=CARTESIAN_POINT('Ctrl Pts',(-50.,14.3429542890555,-6.9137592074853));
#57042=CARTESIAN_POINT('Ctrl Pts',(-66.,14.426553270081,-6.99992315179396));
#57043=CARTESIAN_POINT('Ctrl Pts',(-50.,14.426553270081,-6.99992315179396));
#57044=CARTESIAN_POINT('Ctrl Pts',(-66.,14.5094730904225,-7.08515912713373));
#57045=CARTESIAN_POINT('Ctrl Pts',(-50.,14.5094730904225,-7.08515912713373));
#57046=CARTESIAN_POINT('Ctrl Pts',(-66.,14.5901487815487,-7.17513410761352));
#57047=CARTESIAN_POINT('Ctrl Pts',(-50.,14.5901487815487,-7.17513410761352));
#57048=CARTESIAN_POINT('Ctrl Pts',(-66.,14.6669547000804,-7.27582612382816));
#57049=CARTESIAN_POINT('Ctrl Pts',(-50.,14.6669547000804,-7.27582612382816));
#57050=CARTESIAN_POINT('Ctrl Pts',(-66.,14.7389269269491,-7.39084243431597));
#57051=CARTESIAN_POINT('Ctrl Pts',(-50.,14.7389269269491,-7.39084243431597));
#57052=CARTESIAN_POINT('Ctrl Pts',(-66.,14.80649909067,-7.51868252188801));
#57053=CARTESIAN_POINT('Ctrl Pts',(-50.,14.80649909067,-7.51868252188801));
#57054=CARTESIAN_POINT('Ctrl Pts',(-66.,14.8723343499808,-7.64964883268732));
#57055=CARTESIAN_POINT('Ctrl Pts',(-50.,14.8723343499808,-7.64964883268732));
#57056=CARTESIAN_POINT('Ctrl Pts',(-66.,14.9406799598344,-7.76821640326081));
#57057=CARTESIAN_POINT('Ctrl Pts',(-50.,14.9406799598344,-7.76821640326081));
#57058=CARTESIAN_POINT('Ctrl Pts',(-66.,15.0165470196623,-7.85604888267077));
#57059=CARTESIAN_POINT('Ctrl Pts',(-50.,15.0165470196623,-7.85604888267077));
#57060=CARTESIAN_POINT('Ctrl Pts',(-66.,15.1050127906107,-7.8945628075167));
#57061=CARTESIAN_POINT('Ctrl Pts',(-50.,15.1050127906107,-7.8945628075167));
#57062=CARTESIAN_POINT('Ctrl Pts',(-66.,15.2103404376476,-7.86816419870585));
#57063=CARTESIAN_POINT('Ctrl Pts',(-50.,15.2103404376476,-7.86816419870585));
#57064=CARTESIAN_POINT('Ctrl Pts',(-66.,15.3357420840626,-7.76511876541631));
#57065=CARTESIAN_POINT('Ctrl Pts',(-50.,15.3357420840626,-7.76511876541631));
#57066=CARTESIAN_POINT('Ctrl Pts',(-66.,15.4836142363898,-7.57668480657135));
#57067=CARTESIAN_POINT('Ctrl Pts',(-50.,15.4836142363898,-7.57668480657135));
#57068=CARTESIAN_POINT('Ctrl Pts',(-66.,15.6556301621328,-7.29677247384862));
#57069=CARTESIAN_POINT('Ctrl Pts',(-50.,15.6556301621328,-7.29677247384862));
#57070=CARTESIAN_POINT('Ctrl Pts',(-66.,15.8528843468817,-6.92141167161478));
#57071=CARTESIAN_POINT('Ctrl Pts',(-50.,15.8528843468817,-6.92141167161478));
#57072=CARTESIAN_POINT('Ctrl Pts',(-66.,16.0760082821817,-6.44832559436811));
#57073=CARTESIAN_POINT('Ctrl Pts',(-50.,16.0760082821817,-6.44832559436811));
#57074=CARTESIAN_POINT('Ctrl Pts',(-66.,16.3252927994722,-5.87648036593892));
#57075=CARTESIAN_POINT('Ctrl Pts',(-50.,16.3252927994722,-5.87648036593892));
#57076=CARTESIAN_POINT('Ctrl Pts',(-66.,16.545700453756,-5.33982760416968));
#57077=CARTESIAN_POINT('Ctrl Pts',(-50.,16.545700453756,-5.33982760416968));
#57078=CARTESIAN_POINT('Ctrl Pts',(-66.,16.7227855517644,-4.89288865806624));
#57079=CARTESIAN_POINT('Ctrl Pts',(-50.,16.7227855517644,-4.89288865806624));
#57080=CARTESIAN_POINT('Ctrl Pts',(-66.,16.8460705903453,-4.57520035854192));
#57081=CARTESIAN_POINT('Ctrl Pts',(-50.,16.8460705903453,-4.57520035854192));
#57082=CARTESIAN_POINT('Ctrl Pts',(-66.,16.9090201868666,-4.41142395606429));
#57083=CARTESIAN_POINT('Ctrl Pts',(-50.,16.9090201868666,-4.41142395606429));
#57084=CARTESIAN_POINT('',(-65.5,14.967688987597,-7.79319647965878));
#57085=CARTESIAN_POINT('Ctrl Pts',(-66.,14.6670849864349,-7.28129404712485));
#57086=CARTESIAN_POINT('Ctrl Pts',(-65.793328015403,14.8010034481658,-7.47632260648893));
#57087=CARTESIAN_POINT('Ctrl Pts',(-65.6370761749494,14.8724422320436,-7.67931039448365));
#57088=CARTESIAN_POINT('Ctrl Pts',(-65.5,14.9676889875971,-7.79319647965879));
#57089=CARTESIAN_POINT('',(-66.,12.8026622457696,-5.81770965851216));
#57090=CARTESIAN_POINT('',(-50.5,14.9676889875971,-7.79319647965878));
#57091=CARTESIAN_POINT('Ctrl Pts',(-50.5,14.967688987597,-7.79319647965878));
#57092=CARTESIAN_POINT('Ctrl Pts',(-50.4506066448269,14.933368239824,-7.75215932745924));
#57093=CARTESIAN_POINT('Ctrl Pts',(-50.3985811798094,14.9019662355384,-7.699722088817));
#57094=CARTESIAN_POINT('Ctrl Pts',(-50.2410584360541,14.8108032651412,-7.53250027576706));
#57095=CARTESIAN_POINT('Ctrl Pts',(-50.1348334000372,14.7544537778951,-7.40853124289031));
#57096=CARTESIAN_POINT('Ctrl Pts',(-50.,14.6670849864349,-7.28129404712485));
#57097=CARTESIAN_POINT('Ctrl Pts',(-65.5,14.967688987597,-7.79319647965878));
#57098=CARTESIAN_POINT('Ctrl Pts',(-60.5,14.967688987597,-7.79319647965878));
#57099=CARTESIAN_POINT('Ctrl Pts',(-55.5,14.967688987597,-7.79319647965878));
#57100=CARTESIAN_POINT('Ctrl Pts',(-50.5,14.967688987597,-7.79319647965878));
#57101=CARTESIAN_POINT('Origin',(-66.,0.,0.));
#57102=CARTESIAN_POINT('',(-66.,13.3152354345065,-4.52309756402218));
#57103=CARTESIAN_POINT('Ctrl Pts',(-66.,16.9090201868666,-4.41142395606429));
#57104=CARTESIAN_POINT('Ctrl Pts',(-50.,16.9090201868666,-4.41142395606429));
#57105=CARTESIAN_POINT('Ctrl Pts',(-66.,16.8876463900293,-4.41848310519446));
#57106=CARTESIAN_POINT('Ctrl Pts',(-50.,16.8876463900293,-4.41848310519446));
#57107=CARTESIAN_POINT('Ctrl Pts',(-66.,16.8449024726547,-4.43245358774968));
#57108=CARTESIAN_POINT('Ctrl Pts',(-50.,16.8449024726547,-4.43245358774968));
#57109=CARTESIAN_POINT('Ctrl Pts',(-66.,16.7807976254172,-4.4529658651396));
#57110=CARTESIAN_POINT('Ctrl Pts',(-50.,16.7807976254172,-4.4529658651396));
#57111=CARTESIAN_POINT('Ctrl Pts',(-66.,16.6953465834,-4.47942749016865));
#57112=CARTESIAN_POINT('Ctrl Pts',(-50.,16.6953465834,-4.47942749016865));
#57113=CARTESIAN_POINT('Ctrl Pts',(-66.,16.5885700548362,-4.51101833893424));
#57114=CARTESIAN_POINT('Ctrl Pts',(-50.,16.5885700548362,-4.51101833893424));
#57115=CARTESIAN_POINT('Ctrl Pts',(-66.,16.4818319007497,-4.54111666547111));
#57116=CARTESIAN_POINT('Ctrl Pts',(-50.,16.4818319007497,-4.54111666547111));
#57117=CARTESIAN_POINT('Ctrl Pts',(-66.,16.3751340792151,-4.56971903946321));
#57118=CARTESIAN_POINT('Ctrl Pts',(-50.,16.3751340792151,-4.56971903946321));
#57119=CARTESIAN_POINT('Ctrl Pts',(-66.,16.2684797006663,-4.5968276655857));
#57120=CARTESIAN_POINT('Ctrl Pts',(-50.,16.2684797006663,-4.5968276655857));
#57121=CARTESIAN_POINT('Ctrl Pts',(-66.,16.1618731298649,-4.62245480870932));
#57122=CARTESIAN_POINT('Ctrl Pts',(-50.,16.1618731298649,-4.62245480870932));
#57123=CARTESIAN_POINT('Ctrl Pts',(-66.,16.0553217640976,-4.64661339822299));
#57124=CARTESIAN_POINT('Ctrl Pts',(-50.,16.0553217640976,-4.64661339822299));
#57125=CARTESIAN_POINT('Ctrl Pts',(-66.,15.9488379523835,-4.66930613085772));
#57126=CARTESIAN_POINT('Ctrl Pts',(-50.,15.9488379523835,-4.66930613085772));
#57127=CARTESIAN_POINT('Ctrl Pts',(-66.,15.8424411002465,-4.6905143727759));
#57128=CARTESIAN_POINT('Ctrl Pts',(-50.,15.8424411002465,-4.6905143727759));
#57129=CARTESIAN_POINT('Ctrl Pts',(-66.,15.7361592327224,-4.71018915637038));
#57130=CARTESIAN_POINT('Ctrl Pts',(-50.,15.7361592327224,-4.71018915637038));
#57131=CARTESIAN_POINT('Ctrl Pts',(-66.,15.6300320919874,-4.72823631288632));
#57132=CARTESIAN_POINT('Ctrl Pts',(-50.,15.6300320919874,-4.72823631288632));
#57133=CARTESIAN_POINT('Ctrl Pts',(-66.,15.5241050440726,-4.74453797526706));
#57134=CARTESIAN_POINT('Ctrl Pts',(-50.,15.5241050440726,-4.74453797526706));
#57135=CARTESIAN_POINT('Ctrl Pts',(-66.,15.418420778849,-4.75898306342126));
#57136=CARTESIAN_POINT('Ctrl Pts',(-50.,15.418420778849,-4.75898306342126));
#57137=CARTESIAN_POINT('Ctrl Pts',(-66.,15.3130110194811,-4.77149742512795));
#57138=CARTESIAN_POINT('Ctrl Pts',(-50.,15.3130110194811,-4.77149742512795));
#57139=CARTESIAN_POINT('Ctrl Pts',(-66.,15.2078897478867,-4.78206888507335));
#57140=CARTESIAN_POINT('Ctrl Pts',(-50.,15.2078897478867,-4.78206888507335));
#57141=CARTESIAN_POINT('Ctrl Pts',(-66.,15.1030415940234,-4.79078931010852));
#57142=CARTESIAN_POINT('Ctrl Pts',(-50.,15.1030415940234,-4.79078931010852));
#57143=CARTESIAN_POINT('Ctrl Pts',(-66.,14.9984364069554,-4.79780470849564));
#57144=CARTESIAN_POINT('Ctrl Pts',(-50.,14.9984364069554,-4.79780470849564));
#57145=CARTESIAN_POINT('Ctrl Pts',(-66.,14.8940524763685,-4.80323496770043));
#57146=CARTESIAN_POINT('Ctrl Pts',(-50.,14.8940524763685,-4.80323496770043));
#57147=CARTESIAN_POINT('Ctrl Pts',(-66.,14.7898983053036,-4.80709879692323));
#57148=CARTESIAN_POINT('Ctrl Pts',(-50.,14.7898983053036,-4.80709879692323));
#57149=CARTESIAN_POINT('Ctrl Pts',(-66.,14.6860319453295,-4.80924728319928));
#57150=CARTESIAN_POINT('Ctrl Pts',(-50.,14.6860319453295,-4.80924728319928));
#57151=CARTESIAN_POINT('Ctrl Pts',(-66.,14.5825896373118,-4.80926492456431));
#57152=CARTESIAN_POINT('Ctrl Pts',(-50.,14.5825896373118,-4.80926492456431));
#57153=CARTESIAN_POINT('Ctrl Pts',(-66.,14.4797618145538,-4.80655518238588));
#57154=CARTESIAN_POINT('Ctrl Pts',(-50.,14.4797618145538,-4.80655518238588));
#57155=CARTESIAN_POINT('Ctrl Pts',(-66.,14.3777512750926,-4.80048846137132));
#57156=CARTESIAN_POINT('Ctrl Pts',(-50.,14.3777512750926,-4.80048846137132));
#57157=CARTESIAN_POINT('Ctrl Pts',(-66.,14.27673584179,-4.79053474041595));
#57158=CARTESIAN_POINT('Ctrl Pts',(-50.,14.27673584179,-4.79053474041595));
#57159=CARTESIAN_POINT('Ctrl Pts',(-66.,14.1768322221664,-4.77639142656668));
#57160=CARTESIAN_POINT('Ctrl Pts',(-50.,14.1768322221664,-4.77639142656668));
#57161=CARTESIAN_POINT('Ctrl Pts',(-66.,14.0780505744683,-4.75814554445644));
#57162=CARTESIAN_POINT('Ctrl Pts',(-50.,14.0780505744683,-4.75814554445644));
#57163=CARTESIAN_POINT('Ctrl Pts',(-66.,13.9803137113395,-4.73619861233502));
#57164=CARTESIAN_POINT('Ctrl Pts',(-50.,13.9803137113395,-4.73619861233502));
#57165=CARTESIAN_POINT('Ctrl Pts',(-66.,13.8834929138094,-4.71113063582666));
#57166=CARTESIAN_POINT('Ctrl Pts',(-50.,13.8834929138094,-4.71113063582666));
#57167=CARTESIAN_POINT('Ctrl Pts',(-66.,13.7874381437893,-4.68358443705714));
#57168=CARTESIAN_POINT('Ctrl Pts',(-50.,13.7874381437893,-4.68358443705714));
#57169=CARTESIAN_POINT('Ctrl Pts',(-66.,13.6920092152502,-4.65414675070122));
#57170=CARTESIAN_POINT('Ctrl Pts',(-50.,13.6920092152502,-4.65414675070122));
#57171=CARTESIAN_POINT('Ctrl Pts',(-66.,13.5971094020329,-4.62321932672933));
#57172=CARTESIAN_POINT('Ctrl Pts',(-50.,13.5971094020329,-4.62321932672933));
#57173=CARTESIAN_POINT('Ctrl Pts',(-66.,13.5026800019769,-4.59104377985933));
#57174=CARTESIAN_POINT('Ctrl Pts',(-50.,13.5026800019769,-4.59104377985933));
#57175=CARTESIAN_POINT('Ctrl Pts',(-66.,13.4274881372306,-4.56440469062003));
#57176=CARTESIAN_POINT('Ctrl Pts',(-50.,13.4274881372306,-4.56440469062003));
#57177=CARTESIAN_POINT('Ctrl Pts',(-66.,13.3712869472582,-4.54393972423008));
#57178=CARTESIAN_POINT('Ctrl Pts',(-50.,13.3712869472582,-4.54393972423008));
#57179=CARTESIAN_POINT('Ctrl Pts',(-66.,13.3339050169562,-4.53008087460641));
#57180=CARTESIAN_POINT('Ctrl Pts',(-50.,13.3339050169562,-4.53008087460641));
#57181=CARTESIAN_POINT('Ctrl Pts',(-66.,13.3152354345065,-4.52309756402217));
#57182=CARTESIAN_POINT('Ctrl Pts',(-50.,13.3152354345065,-4.52309756402217));
#57183=CARTESIAN_POINT('Origin',(-65.75,0.,0.));
#57184=CARTESIAN_POINT('',(-65.5,14.5793859740595,-8.49747783871179));
#57185=CARTESIAN_POINT('Origin',(-65.5,0.,0.));
#57186=CARTESIAN_POINT('Ctrl Pts',(-65.5,14.5793859740595,-8.49747783871179));
#57187=CARTESIAN_POINT('Ctrl Pts',(-65.6931595476758,14.3574969269134,-8.49458741572547));
#57188=CARTESIAN_POINT('Ctrl Pts',(-65.8611256967112,14.1682859702542,-8.48365813109589));
#57189=CARTESIAN_POINT('Ctrl Pts',(-66.,14.0138288999568,-8.47072751083015));
#57190=CARTESIAN_POINT('Origin',(-58.,0.,0.));
#57191=CARTESIAN_POINT('',(-50.5,14.5793859740595,-8.49747783871179));
#57192=CARTESIAN_POINT('Origin',(-50.5,0.,0.));
#57193=CARTESIAN_POINT('Ctrl Pts',(-50.5,14.5793859740595,-8.49747783871179));
#57194=CARTESIAN_POINT('Ctrl Pts',(-55.5,14.5793859740595,-8.49747783871179));
#57195=CARTESIAN_POINT('Ctrl Pts',(-60.5,14.5793859740595,-8.49747783871179));
#57196=CARTESIAN_POINT('Ctrl Pts',(-65.5,14.5793859740595,-8.49747783871179));
#57197=CARTESIAN_POINT('Origin',(-50.25,0.,0.));
#57198=CARTESIAN_POINT('Ctrl Pts',(-50.,14.0138288999568,-8.47072751083015));
#57199=CARTESIAN_POINT('Ctrl Pts',(-50.1388743032911,14.1682859702568,-8.48365813109611));
#57200=CARTESIAN_POINT('Ctrl Pts',(-50.3068404523263,14.3574969269158,-8.49458741572551));
#57201=CARTESIAN_POINT('Ctrl Pts',(-50.5,14.5793859740595,-8.49747783871179));
#57202=CARTESIAN_POINT('Ctrl Pts',(-66.,10.9536375103364,-8.81882824088046));
#57203=CARTESIAN_POINT('Ctrl Pts',(-50.,10.9536375103364,-8.81882824088046));
#57204=CARTESIAN_POINT('Ctrl Pts',(-66.,10.9724295263217,-8.83272480732197));
#57205=CARTESIAN_POINT('Ctrl Pts',(-50.,10.9724295263217,-8.83272480732197));
#57206=CARTESIAN_POINT('Ctrl Pts',(-66.,11.0098871540402,-8.86070419148627));
#57207=CARTESIAN_POINT('Ctrl Pts',(-50.,11.0098871540402,-8.86070419148627));
#57208=CARTESIAN_POINT('Ctrl Pts',(-66.,11.0656943951459,-8.90323201632451));
#57209=CARTESIAN_POINT('Ctrl Pts',(-50.,11.0656943951459,-8.90323201632451));
#57210=CARTESIAN_POINT('Ctrl Pts',(-66.,11.1393445344495,-8.96105481127105));
#57211=CARTESIAN_POINT('Ctrl Pts',(-50.,11.1393445344495,-8.96105481127105));
#57212=CARTESIAN_POINT('Ctrl Pts',(-66.,11.2300954828748,-9.03523227310488));
#57213=CARTESIAN_POINT('Ctrl Pts',(-50.,11.2300954828748,-9.03523227310488));
#57214=CARTESIAN_POINT('Ctrl Pts',(-66.,11.3194051551598,-9.11139639219764));
#57215=CARTESIAN_POINT('Ctrl Pts',(-50.,11.3194051551598,-9.11139639219764));
#57216=CARTESIAN_POINT('Ctrl Pts',(-66.,11.407025252502,-9.18970993907287));
#57217=CARTESIAN_POINT('Ctrl Pts',(-50.,11.407025252502,-9.18970993907287));
#57218=CARTESIAN_POINT('Ctrl Pts',(-66.,11.4925391231036,-9.27043802686381));
#57219=CARTESIAN_POINT('Ctrl Pts',(-50.,11.4925391231036,-9.27043802686381));
#57220=CARTESIAN_POINT('Ctrl Pts',(-66.,11.5754278219505,-9.35393513817802));
#57221=CARTESIAN_POINT('Ctrl Pts',(-50.,11.5754278219505,-9.35393513817802));
#57222=CARTESIAN_POINT('Ctrl Pts',(-66.,11.655157779328,-9.44063172122792));
#57223=CARTESIAN_POINT('Ctrl Pts',(-50.,11.655157779328,-9.44063172122792));
#57224=CARTESIAN_POINT('Ctrl Pts',(-66.,11.7312595885623,-9.53100857350628));
#57225=CARTESIAN_POINT('Ctrl Pts',(-50.,11.7312595885623,-9.53100857350628));
#57226=CARTESIAN_POINT('Ctrl Pts',(-66.,11.8034143911192,-9.62560737856555));
#57227=CARTESIAN_POINT('Ctrl Pts',(-50.,11.8034143911192,-9.62560737856555));
#57228=CARTESIAN_POINT('Ctrl Pts',(-66.,11.8715286035136,-9.724847924125));
#57229=CARTESIAN_POINT('Ctrl Pts',(-50.,11.8715286035136,-9.724847924125));
#57230=CARTESIAN_POINT('Ctrl Pts',(-66.,11.9358257812543,-9.82870769953299));
#57231=CARTESIAN_POINT('Ctrl Pts',(-50.,11.9358257812543,-9.82870769953299));
#57232=CARTESIAN_POINT('Ctrl Pts',(-66.,11.9969002916812,-9.93651465742827));
#57233=CARTESIAN_POINT('Ctrl Pts',(-50.,11.9969002916812,-9.93651465742827));
#57234=CARTESIAN_POINT('Ctrl Pts',(-66.,12.0558705645975,-10.0465202590396));
#57235=CARTESIAN_POINT('Ctrl Pts',(-50.,12.0558705645975,-10.0465202590396));
#57236=CARTESIAN_POINT('Ctrl Pts',(-66.,12.1141848750712,-10.1561990251342));
#57237=CARTESIAN_POINT('Ctrl Pts',(-50.,12.1141848750712,-10.1561990251342));
#57238=CARTESIAN_POINT('Ctrl Pts',(-66.,12.1729620080223,-10.2634984322242));
#57239=CARTESIAN_POINT('Ctrl Pts',(-50.,12.1729620080223,-10.2634984322242));
#57240=CARTESIAN_POINT('Ctrl Pts',(-66.,12.2325064717433,-10.3677455989363));
#57241=CARTESIAN_POINT('Ctrl Pts',(-50.,12.2325064717433,-10.3677455989363));
#57242=CARTESIAN_POINT('Ctrl Pts',(-66.,12.2916238883603,-10.4709250501372));
#57243=CARTESIAN_POINT('Ctrl Pts',(-50.,12.2916238883603,-10.4709250501372));
#57244=CARTESIAN_POINT('Ctrl Pts',(-66.,12.3473891365543,-10.5781365296759));
#57245=CARTESIAN_POINT('Ctrl Pts',(-50.,12.3473891365543,-10.5781365296759));
#57246=CARTESIAN_POINT('Ctrl Pts',(-66.,12.3967409697684,-10.6947659762548));
#57247=CARTESIAN_POINT('Ctrl Pts',(-50.,12.3967409697684,-10.6947659762548));
#57248=CARTESIAN_POINT('Ctrl Pts',(-66.,12.437848663505,-10.8240676028274));
#57249=CARTESIAN_POINT('Ctrl Pts',(-50.,12.437848663505,-10.8240676028274));
#57250=CARTESIAN_POINT('Ctrl Pts',(-66.,12.4715053864926,-10.9646958727381));
#57251=CARTESIAN_POINT('Ctrl Pts',(-50.,12.4715053864926,-10.9646958727381));
#57252=CARTESIAN_POINT('Ctrl Pts',(-66.,12.5027023130146,-11.107920199263));
#57253=CARTESIAN_POINT('Ctrl Pts',(-50.,12.5027023130146,-11.107920199263));
#57254=CARTESIAN_POINT('Ctrl Pts',(-66.,12.5394141641085,-11.239759613579));
#57255=CARTESIAN_POINT('Ctrl Pts',(-50.,12.5394141641085,-11.239759613579));
#57256=CARTESIAN_POINT('Ctrl Pts',(-66.,12.5910546713482,-11.3437000446838));
#57257=CARTESIAN_POINT('Ctrl Pts',(-50.,12.5910546713482,-11.3437000446838));
#57258=CARTESIAN_POINT('Ctrl Pts',(-66.,12.6671631038009,-11.4030045263537));
#57259=CARTESIAN_POINT('Ctrl Pts',(-50.,12.6671631038009,-11.4030045263537));
#57260=CARTESIAN_POINT('Ctrl Pts',(-66.,12.7757467561686,-11.4036291990392));
#57261=CARTESIAN_POINT('Ctrl Pts',(-50.,12.7757467561686,-11.4036291990392));
#57262=CARTESIAN_POINT('Ctrl Pts',(-66.,12.9228350364417,-11.335007248821));
#57263=CARTESIAN_POINT('Ctrl Pts',(-50.,12.9228350364417,-11.335007248821));
#57264=CARTESIAN_POINT('Ctrl Pts',(-66.,13.1129231331489,-11.1892675981761));
#57265=CARTESIAN_POINT('Ctrl Pts',(-50.,13.1129231331489,-11.1892675981761));
#57266=CARTESIAN_POINT('Ctrl Pts',(-66.,13.3491462287103,-10.9609278472722));
#57267=CARTESIAN_POINT('Ctrl Pts',(-50.,13.3491462287103,-10.9609278472722));
#57268=CARTESIAN_POINT('Ctrl Pts',(-66.,13.6335517460739,-10.6464148158287));
#57269=CARTESIAN_POINT('Ctrl Pts',(-50.,13.6335517460739,-10.6464148158287));
#57270=CARTESIAN_POINT('Ctrl Pts',(-66.,13.9673175558199,-10.2436802739367));
#57271=CARTESIAN_POINT('Ctrl Pts',(-50.,13.9673175558199,-10.2436802739367));
#57272=CARTESIAN_POINT('Ctrl Pts',(-66.,14.3509824669314,-9.75179515338539));
#57273=CARTESIAN_POINT('Ctrl Pts',(-50.,14.3509824669314,-9.75179515338539));
#57274=CARTESIAN_POINT('Ctrl Pts',(-66.,14.6979257242257,-9.28681547963666));
#57275=CARTESIAN_POINT('Ctrl Pts',(-50.,14.6979257242257,-9.28681547963666));
#57276=CARTESIAN_POINT('Ctrl Pts',(-66.,14.9805965643194,-8.89795721543056));
#57277=CARTESIAN_POINT('Ctrl Pts',(-50.,14.9805965643194,-8.89795721543056));
#57278=CARTESIAN_POINT('Ctrl Pts',(-66.,15.1790142440703,-8.62090942035752));
#57279=CARTESIAN_POINT('Ctrl Pts',(-50.,15.1790142440703,-8.62090942035752));
#57280=CARTESIAN_POINT('Ctrl Pts',(-66.,15.2807156983131,-8.47793328278342));
#57281=CARTESIAN_POINT('Ctrl Pts',(-50.,15.2807156983131,-8.47793328278342));
#57282=CARTESIAN_POINT('',(-65.5,12.5593623612171,-11.2706717670086));
#57283=CARTESIAN_POINT('Ctrl Pts',(-66.,12.3955073457098,-10.7000945155851));
#57284=CARTESIAN_POINT('Ctrl Pts',(-65.7933280154029,12.4767168822844,-10.9223000612616));
#57285=CARTESIAN_POINT('Ctrl Pts',(-65.6370761749496,12.4954302753076,-11.1366767177294));
#57286=CARTESIAN_POINT('Ctrl Pts',(-65.5,12.5593623612171,-11.2706717670086));
#57287=CARTESIAN_POINT('',(-66.,10.9536375103364,-8.81882824088046));
#57288=CARTESIAN_POINT('',(-50.5,12.5593623612171,-11.2706717670086));
#57289=CARTESIAN_POINT('Ctrl Pts',(-50.5,12.5593623612171,-11.2706717670086));
#57290=CARTESIAN_POINT('Ctrl Pts',(-50.4518618349124,12.5369108060359,-11.2236156261038));
#57291=CARTESIAN_POINT('Ctrl Pts',(-50.4012423593889,12.5198465875944,-11.1667793509398));
#57292=CARTESIAN_POINT('Ctrl Pts',(-50.2441129793807,12.4729367680423,-10.982980939431));
#57293=CARTESIAN_POINT('Ctrl Pts',(-50.1366827452944,12.449215362424,-10.847050398657));
#57294=CARTESIAN_POINT('Ctrl Pts',(-50.,12.3955073457098,-10.7000945155851));
#57295=CARTESIAN_POINT('Ctrl Pts',(-65.5,12.5593623612171,-11.2706717670086));
#57296=CARTESIAN_POINT('Ctrl Pts',(-60.5,12.5593623612171,-11.2706717670086));
#57297=CARTESIAN_POINT('Ctrl Pts',(-55.5,12.5593623612171,-11.2706717670086));
#57298=CARTESIAN_POINT('Ctrl Pts',(-50.5,12.5593623612171,-11.2706717670086));
#57299=CARTESIAN_POINT('Origin',(-66.,0.,0.));
#57300=CARTESIAN_POINT('',(-66.,11.7720642054939,-7.6923605344347));
#57301=CARTESIAN_POINT('Ctrl Pts',(-66.,15.2807156983131,-8.47793328278342));
#57302=CARTESIAN_POINT('Ctrl Pts',(-50.,15.2807156983131,-8.47793328278342));
#57303=CARTESIAN_POINT('Ctrl Pts',(-66.,15.2582578596065,-8.47945520863905));
#57304=CARTESIAN_POINT('Ctrl Pts',(-50.,15.2582578596065,-8.47945520863905));
#57305=CARTESIAN_POINT('Ctrl Pts',(-66.,15.2133825032665,-8.482356802806));
#57306=CARTESIAN_POINT('Ctrl Pts',(-50.,15.2133825032665,-8.482356802806));
#57307=CARTESIAN_POINT('Ctrl Pts',(-66.,15.1461904317359,-8.48628242205606));
#57308=CARTESIAN_POINT('Ctrl Pts',(-50.,15.1461904317359,-8.48628242205606));
#57309=CARTESIAN_POINT('Ctrl Pts',(-66.,15.0568432527945,-8.49066189647792));
#57310=CARTESIAN_POINT('Ctrl Pts',(-50.,15.0568432527945,-8.49066189647792));
#57311=CARTESIAN_POINT('Ctrl Pts',(-66.,14.9455649806088,-8.49470601779764));
#57312=CARTESIAN_POINT('Ctrl Pts',(-50.,14.9455649806088,-8.49470601779764));
#57313=CARTESIAN_POINT('Ctrl Pts',(-66.,14.8346950524804,-8.49731405056346));
#57314=CARTESIAN_POINT('Ctrl Pts',(-50.,14.8346950524804,-8.49731405056346));
#57315=CARTESIAN_POINT('Ctrl Pts',(-66.,14.7242362180521,-8.49848315918232));
#57316=CARTESIAN_POINT('Ctrl Pts',(-50.,14.7242362180521,-8.49848315918232));
#57317=CARTESIAN_POINT('Ctrl Pts',(-66.,14.6141909417575,-8.49821625259896));
#57318=CARTESIAN_POINT('Ctrl Pts',(-50.,14.6141909417575,-8.49821625259896));
#57319=CARTESIAN_POINT('Ctrl Pts',(-66.,14.5045604010818,-8.49652629583269));
#57320=CARTESIAN_POINT('Ctrl Pts',(-50.,14.5045604010818,-8.49652629583269));
#57321=CARTESIAN_POINT('Ctrl Pts',(-66.,14.3953485455042,-8.49342765170233));
#57322=CARTESIAN_POINT('Ctrl Pts',(-50.,14.3953485455042,-8.49342765170233));
#57323=CARTESIAN_POINT('Ctrl Pts',(-66.,14.2865666654267,-8.48892600329226));
#57324=CARTESIAN_POINT('Ctrl Pts',(-50.,14.2865666654267,-8.48892600329226));
#57325=CARTESIAN_POINT('Ctrl Pts',(-66.,14.1782381907602,-8.48300812813872));
#57326=CARTESIAN_POINT('Ctrl Pts',(-50.,14.1782381907602,-8.48300812813872));
#57327=CARTESIAN_POINT('Ctrl Pts',(-66.,14.0704024438309,-8.47563356658493));
#57328=CARTESIAN_POINT('Ctrl Pts',(-50.,14.0704024438309,-8.47563356658493));
#57329=CARTESIAN_POINT('Ctrl Pts',(-66.,13.9631213370587,-8.46672099183801));
#57330=CARTESIAN_POINT('Ctrl Pts',(-50.,13.9631213370587,-8.46672099183801));
#57331=CARTESIAN_POINT('Ctrl Pts',(-66.,13.8564681235622,-8.45616752192477));
#57332=CARTESIAN_POINT('Ctrl Pts',(-50.,13.8564681235622,-8.45616752192477));
#57333=CARTESIAN_POINT('Ctrl Pts',(-66.,13.7505117765273,-8.44387618307839));
#57334=CARTESIAN_POINT('Ctrl Pts',(-50.,13.7505117765273,-8.44387618307839));
#57335=CARTESIAN_POINT('Ctrl Pts',(-66.,13.6453014633841,-8.42978304193647));
#57336=CARTESIAN_POINT('Ctrl Pts',(-50.,13.6453014633841,-8.42978304193647));
#57337=CARTESIAN_POINT('Ctrl Pts',(-66.,13.5408537546603,-8.41387978285669));
#57338=CARTESIAN_POINT('Ctrl Pts',(-50.,13.5408537546603,-8.41387978285669));
#57339=CARTESIAN_POINT('Ctrl Pts',(-66.,13.4371309168349,-8.39625156414993));
#57340=CARTESIAN_POINT('Ctrl Pts',(-50.,13.4371309168349,-8.39625156414993));
#57341=CARTESIAN_POINT('Ctrl Pts',(-66.,13.3340674354409,-8.37703230872753));
#57342=CARTESIAN_POINT('Ctrl Pts',(-50.,13.3340674354409,-8.37703230872753));
#57343=CARTESIAN_POINT('Ctrl Pts',(-66.,13.231612467433,-8.35633273843435));
#57344=CARTESIAN_POINT('Ctrl Pts',(-50.,13.231612467433,-8.35633273843435));
#57345=CARTESIAN_POINT('Ctrl Pts',(-66.,13.1297695959248,-8.33417308930716));
#57346=CARTESIAN_POINT('Ctrl Pts',(-50.,13.1297695959248,-8.33417308930716));
#57347=CARTESIAN_POINT('Ctrl Pts',(-66.,13.0286320818366,-8.31042356359388));
#57348=CARTESIAN_POINT('Ctrl Pts',(-50.,13.0286320818366,-8.31042356359388));
#57349=CARTESIAN_POINT('Ctrl Pts',(-66.,12.9284352169133,-8.284715594814));
#57350=CARTESIAN_POINT('Ctrl Pts',(-50.,12.9284352169133,-8.284715594814));
#57351=CARTESIAN_POINT('Ctrl Pts',(-66.,12.829511804771,-8.25651874452987));
#57352=CARTESIAN_POINT('Ctrl Pts',(-50.,12.829511804771,-8.25651874452987));
#57353=CARTESIAN_POINT('Ctrl Pts',(-66.,12.7322148461558,-8.22527363116368));
#57354=CARTESIAN_POINT('Ctrl Pts',(-50.,12.7322148461558,-8.22527363116368));
#57355=CARTESIAN_POINT('Ctrl Pts',(-66.,12.636848388186,-8.19051110794578));
#57356=CARTESIAN_POINT('Ctrl Pts',(-50.,12.636848388186,-8.19051110794578));
#57357=CARTESIAN_POINT('Ctrl Pts',(-66.,12.5436007236081,-8.15196711241727));
#57358=CARTESIAN_POINT('Ctrl Pts',(-50.,12.5436007236081,-8.15196711241727));
#57359=CARTESIAN_POINT('Ctrl Pts',(-66.,12.4524600493824,-8.10972846142537));
#57360=CARTESIAN_POINT('Ctrl Pts',(-50.,12.4524600493824,-8.10972846142537));
#57361=CARTESIAN_POINT('Ctrl Pts',(-66.,12.3632517496072,-8.06416486307078));
#57362=CARTESIAN_POINT('Ctrl Pts',(-50.,12.3632517496072,-8.06416486307078));
#57363=CARTESIAN_POINT('Ctrl Pts',(-66.,12.2757069077219,-8.01580608992824));
#57364=CARTESIAN_POINT('Ctrl Pts',(-50.,12.2757069077219,-8.01580608992824));
#57365=CARTESIAN_POINT('Ctrl Pts',(-66.,12.1895203359981,-7.96523745572904));
#57366=CARTESIAN_POINT('Ctrl Pts',(-50.,12.1895203359981,-7.96523745572904));
#57367=CARTESIAN_POINT('Ctrl Pts',(-66.,12.1044103376288,-7.91299239895144));
#57368=CARTESIAN_POINT('Ctrl Pts',(-50.,12.1044103376288,-7.91299239895144));
#57369=CARTESIAN_POINT('Ctrl Pts',(-66.,12.0201833141302,-7.85943599303422));
#57370=CARTESIAN_POINT('Ctrl Pts',(-50.,12.0201833141302,-7.85943599303422));
#57371=CARTESIAN_POINT('Ctrl Pts',(-66.,11.936722320441,-7.80478766329085));
#57372=CARTESIAN_POINT('Ctrl Pts',(-50.,11.936722320441,-7.80478766329085));
#57373=CARTESIAN_POINT('Ctrl Pts',(-66.,11.870517618491,-7.7602860336664));
#57374=CARTESIAN_POINT('Ctrl Pts',(-50.,11.870517618491,-7.7602860336664));
#57375=CARTESIAN_POINT('Ctrl Pts',(-66.,11.8211715224307,-7.72648734423527));
#57376=CARTESIAN_POINT('Ctrl Pts',(-50.,11.8211715224307,-7.72648734423527));
#57377=CARTESIAN_POINT('Ctrl Pts',(-66.,11.7884105699588,-7.70376738782835));
#57378=CARTESIAN_POINT('Ctrl Pts',(-50.,11.7884105699588,-7.70376738782835));
#57379=CARTESIAN_POINT('Ctrl Pts',(-66.,11.7720642054939,-7.69236053443469));
#57380=CARTESIAN_POINT('Ctrl Pts',(-50.,11.7720642054939,-7.69236053443469));
#57381=CARTESIAN_POINT('Origin',(-65.75,0.,0.));
#57382=CARTESIAN_POINT('',(-65.5,12.0081109491739,-11.8562597994617));
#57383=CARTESIAN_POINT('Origin',(-65.5,0.,0.));
#57384=CARTESIAN_POINT('Ctrl Pts',(-65.5,12.0081109491739,-11.8562597994617));
#57385=CARTESIAN_POINT('Ctrl Pts',(-65.6931595476832,11.7939117734275,-11.7982786223285));
#57386=CARTESIAN_POINT('Ctrl Pts',(-65.8611256967229,11.6133632294635,-11.7406378498091));
#57387=CARTESIAN_POINT('Ctrl Pts',(-66.,11.4669744265634,-11.689701557377));
#57388=CARTESIAN_POINT('Origin',(-58.,0.,0.));
#57389=CARTESIAN_POINT('',(-50.5,12.0081109491739,-11.8562597994617));
#57390=CARTESIAN_POINT('Origin',(-50.5,0.,0.));
#57391=CARTESIAN_POINT('Ctrl Pts',(-50.5,12.0081109491739,-11.8562597994617));
#57392=CARTESIAN_POINT('Ctrl Pts',(-55.5,12.0081109491739,-11.8562597994617));
#57393=CARTESIAN_POINT('Ctrl Pts',(-60.5,12.0081109491739,-11.8562597994617));
#57394=CARTESIAN_POINT('Ctrl Pts',(-65.5,12.0081109491739,-11.8562597994617));
#57395=CARTESIAN_POINT('Origin',(-50.25,0.,0.));
#57396=CARTESIAN_POINT('Ctrl Pts',(-50.,11.4669744265634,-11.689701557377));
#57397=CARTESIAN_POINT('Ctrl Pts',(-50.1388743032958,11.6133632294832,-11.740637849816));
#57398=CARTESIAN_POINT('Ctrl Pts',(-50.3068404523301,11.7939117734422,-11.7982786223325));
#57399=CARTESIAN_POINT('Ctrl Pts',(-50.5,12.0081109491739,-11.8562597994617));
#57400=CARTESIAN_POINT('Ctrl Pts',(-66.,8.41635544546801,-11.2658274114927));
#57401=CARTESIAN_POINT('Ctrl Pts',(-50.,8.41635544546801,-11.2658274114927));
#57402=CARTESIAN_POINT('Ctrl Pts',(-66.,8.43110114017464,-11.2839607760805));
#57403=CARTESIAN_POINT('Ctrl Pts',(-50.,8.43110114017464,-11.2839607760805));
#57404=CARTESIAN_POINT('Ctrl Pts',(-66.,8.46042377774785,-11.3203764696515));
#57405=CARTESIAN_POINT('Ctrl Pts',(-50.,8.46042377774785,-11.3203764696515));
#57406=CARTESIAN_POINT('Ctrl Pts',(-66.,8.50390149179148,-11.3754469011628));
#57407=CARTESIAN_POINT('Ctrl Pts',(-50.,8.50390149179148,-11.3754469011628));
#57408=CARTESIAN_POINT('Ctrl Pts',(-66.,8.56085783218497,-11.4497691315105));
#57409=CARTESIAN_POINT('Ctrl Pts',(-50.,8.56085783218497,-11.4497691315105));
#57410=CARTESIAN_POINT('Ctrl Pts',(-66.,8.63031048807256,-11.544185015102));
#57411=CARTESIAN_POINT('Ctrl Pts',(-50.,8.63031048807256,-11.544185015102));
#57412=CARTESIAN_POINT('Ctrl Pts',(-66.,8.69787308659046,-11.6401667106607));
#57413=CARTESIAN_POINT('Ctrl Pts',(-50.,8.69787308659046,-11.6401667106607));
#57414=CARTESIAN_POINT('Ctrl Pts',(-66.,8.76326465031677,-11.7378101255738));
#57415=CARTESIAN_POINT('Ctrl Pts',(-50.,8.76326465031677,-11.7378101255738));
#57416=CARTESIAN_POINT('Ctrl Pts',(-66.,8.8260156863806,-11.8372684268691));
#57417=CARTESIAN_POINT('Ctrl Pts',(-50.,8.8260156863806,-11.8372684268691));
#57418=CARTESIAN_POINT('Ctrl Pts',(-66.,8.88553539714026,-11.9387559040544));
#57419=CARTESIAN_POINT('Ctrl Pts',(-50.,8.88553539714026,-11.9387559040544));
#57420=CARTESIAN_POINT('Ctrl Pts',(-66.,8.94119992783734,-12.0425567886278));
#57421=CARTESIAN_POINT('Ctrl Pts',(-50.,8.94119992783734,-12.0425567886278));
#57422=CARTESIAN_POINT('Ctrl Pts',(-66.,8.99243504959771,-12.149020036252));
#57423=CARTESIAN_POINT('Ctrl Pts',(-50.,8.99243504959771,-12.149020036252));
#57424=CARTESIAN_POINT('Ctrl Pts',(-66.,9.03879721019277,-12.2585910156016));
#57425=CARTESIAN_POINT('Ctrl Pts',(-50.,9.03879721019277,-12.2585910156016));
#57426=CARTESIAN_POINT('Ctrl Pts',(-66.,9.08009136927418,-12.3716530527263));
#57427=CARTESIAN_POINT('Ctrl Pts',(-50.,9.08009136927418,-12.3716530527263));
#57428=CARTESIAN_POINT('Ctrl Pts',(-66.,9.11653965711474,-12.4882399401825));
#57429=CARTESIAN_POINT('Ctrl Pts',(-50.,9.11653965711474,-12.4882399401825));
#57430=CARTESIAN_POINT('Ctrl Pts',(-66.,9.14888489929381,-12.6078485573591));
#57431=CARTESIAN_POINT('Ctrl Pts',(-50.,9.14888489929381,-12.6078485573591));
#57432=CARTESIAN_POINT('Ctrl Pts',(-66.,9.17864523199547,-12.7290634412273));
#57433=CARTESIAN_POINT('Ctrl Pts',(-50.,9.17864523199547,-12.7290634412273));
#57434=CARTESIAN_POINT('Ctrl Pts',(-66.,9.20785149120868,-12.8497986264917));
#57435=CARTESIAN_POINT('Ctrl Pts',(-50.,9.20785149120868,-12.8497986264917));
#57436=CARTESIAN_POINT('Ctrl Pts',(-66.,9.23809775500251,-12.9683443039596));
#57437=CARTESIAN_POINT('Ctrl Pts',(-50.,9.23809775500251,-12.9683443039596));
#57438=CARTESIAN_POINT('Ctrl Pts',(-66.,9.26984630377419,-13.0841244601964));
#57439=CARTESIAN_POINT('Ctrl Pts',(-50.,9.26984630377419,-13.0841244601964));
#57440=CARTESIAN_POINT('Ctrl Pts',(-66.,9.30144675196197,-13.1987642428721));
#57441=CARTESIAN_POINT('Ctrl Pts',(-50.,9.30144675196197,-13.1987642428721));
#57442=CARTESIAN_POINT('Ctrl Pts',(-66.,9.32879762158958,-13.316475729914));
#57443=CARTESIAN_POINT('Ctrl Pts',(-50.,9.32879762158958,-13.316475729914));
#57444=CARTESIAN_POINT('Ctrl Pts',(-66.,9.34759441230173,-13.4417143497954));
#57445=CARTESIAN_POINT('Ctrl Pts',(-50.,9.34759441230173,-13.4417143497954));
#57446=CARTESIAN_POINT('Ctrl Pts',(-66.,9.35525462532529,-13.5771767957172));
#57447=CARTESIAN_POINT('Ctrl Pts',(-50.,9.35525462532529,-13.5771767957172));
#57448=CARTESIAN_POINT('Ctrl Pts',(-66.,9.35288113189361,-13.7217570565735));
#57449=CARTESIAN_POINT('Ctrl Pts',(-50.,9.35288113189361,-13.7217570565735));
#57450=CARTESIAN_POINT('Ctrl Pts',(-66.,9.34747950799902,-13.8682400876461));
#57451=CARTESIAN_POINT('Ctrl Pts',(-50.,9.34747950799902,-13.8682400876461));
#57452=CARTESIAN_POINT('Ctrl Pts',(-66.,9.35025085971223,-14.0050673904318));
#57453=CARTESIAN_POINT('Ctrl Pts',(-50.,9.35025085971223,-14.0050673904318));
#57454=CARTESIAN_POINT('Ctrl Pts',(-66.,9.37442005137349,-14.118584813679));
#57455=CARTESIAN_POINT('Ctrl Pts',(-50.,9.37442005137349,-14.118584813679));
#57456=CARTESIAN_POINT('Ctrl Pts',(-66.,9.43338897261223,-14.1949535334828));
#57457=CARTESIAN_POINT('Ctrl Pts',(-50.,9.43338897261223,-14.1949535334828));
#57458=CARTESIAN_POINT('Ctrl Pts',(-66.,9.53840592008975,-14.2225622371825));
#57459=CARTESIAN_POINT('Ctrl Pts',(-50.,9.53840592008975,-14.2225622371825));
#57460=CARTESIAN_POINT('Ctrl Pts',(-66.,9.69793873661838,-14.1926755395417));
#57461=CARTESIAN_POINT('Ctrl Pts',(-50.,9.69793873661838,-14.1926755395417));
#57462=CARTESIAN_POINT('Ctrl Pts',(-66.,9.9182988434943,-14.0987875553398));
#57463=CARTESIAN_POINT('Ctrl Pts',(-50.,9.9182988434943,-14.0987875553398));
#57464=CARTESIAN_POINT('Ctrl Pts',(-66.,10.2038863430123,-13.9363678125788));
#57465=CARTESIAN_POINT('Ctrl Pts',(-50.,10.2038863430123,-13.9363678125788));
#57466=CARTESIAN_POINT('Ctrl Pts',(-66.,10.5575729483643,-13.7024645623894));
#57467=CARTESIAN_POINT('Ctrl Pts',(-50.,10.5575729483643,-13.7024645623894));
#57468=CARTESIAN_POINT('Ctrl Pts',(-66.,10.9810088992253,-13.3953868482732));
#57469=CARTESIAN_POINT('Ctrl Pts',(-50.,10.9810088992253,-13.3953868482732));
#57470=CARTESIAN_POINT('Ctrl Pts',(-66.,11.4749471267718,-13.0143687867509));
#57471=CARTESIAN_POINT('Ctrl Pts',(-50.,11.4749471267718,-13.0143687867509));
#57472=CARTESIAN_POINT('Ctrl Pts',(-66.,11.9266262662527,-12.6502785839999));
#57473=CARTESIAN_POINT('Ctrl Pts',(-50.,11.9266262662527,-12.6502785839999));
#57474=CARTESIAN_POINT('Ctrl Pts',(-66.,12.2971215999581,-12.3439343965519));
#57475=CARTESIAN_POINT('Ctrl Pts',(-50.,12.2971215999581,-12.3439343965519));
#57476=CARTESIAN_POINT('Ctrl Pts',(-66.,12.558204608331,-12.1249350378051));
#57477=CARTESIAN_POINT('Ctrl Pts',(-50.,12.558204608331,-12.1249350378051));
#57478=CARTESIAN_POINT('Ctrl Pts',(-66.,12.6922676438934,-12.0117428816877));
#57479=CARTESIAN_POINT('Ctrl Pts',(-50.,12.6922676438934,-12.0117428816877));
#57480=CARTESIAN_POINT('',(-65.5,9.3618848075781,-14.039969296606));
#57481=CARTESIAN_POINT('Ctrl Pts',(-66.,9.34507439096662,-13.4465686934362));
#57482=CARTESIAN_POINT('Ctrl Pts',(-65.7933280154029,9.36847230853418,-13.6819892337753));
#57483=CARTESIAN_POINT('Ctrl Pts',(-65.6370761749495,9.33328447939624,-13.8942846849687));
#57484=CARTESIAN_POINT('Ctrl Pts',(-65.5,9.3618848075781,-14.039969296606));
#57485=CARTESIAN_POINT('',(-66.,8.41635544546801,-11.2658274114927));
#57486=CARTESIAN_POINT('',(-50.5,9.3618848075781,-14.039969296606));
#57487=CARTESIAN_POINT('Ctrl Pts',(-50.5,9.3618848075781,-14.039969296606));
#57488=CARTESIAN_POINT('Ctrl Pts',(-50.4518618349121,9.35184099566044,-13.9888080361729));
#57489=CARTESIAN_POINT('Ctrl Pts',(-50.4012423593883,9.34944748787756,-13.9295136785486));
#57490=CARTESIAN_POINT('Ctrl Pts',(-50.2441129793799,9.34972023278718,-13.7398236343874));
#57491=CARTESIAN_POINT('Ctrl Pts',(-50.1366827452941,9.36054862959424,-13.6022643278246));
#57492=CARTESIAN_POINT('Ctrl Pts',(-50.,9.34507439096662,-13.4465686934362));
#57493=CARTESIAN_POINT('Ctrl Pts',(-65.5,9.3618848075781,-14.039969296606));
#57494=CARTESIAN_POINT('Ctrl Pts',(-60.5,9.3618848075781,-14.039969296606));
#57495=CARTESIAN_POINT('Ctrl Pts',(-55.5,9.3618848075781,-14.039969296606));
#57496=CARTESIAN_POINT('Ctrl Pts',(-50.5,9.3618848075781,-14.039969296606));
#57497=CARTESIAN_POINT('Origin',(-66.,0.,0.));
#57498=CARTESIAN_POINT('',(-66.,9.48921088782657,-10.3782842019456));
#57499=CARTESIAN_POINT('Ctrl Pts',(-66.,12.6922676438934,-12.0117428816877));
#57500=CARTESIAN_POINT('Ctrl Pts',(-50.,12.6922676438934,-12.0117428816877));
#57501=CARTESIAN_POINT('Ctrl Pts',(-66.,12.6701368719175,-12.00763195607));
#57502=CARTESIAN_POINT('Ctrl Pts',(-50.,12.6701368719175,-12.00763195607));
#57503=CARTESIAN_POINT('Ctrl Pts',(-66.,12.625949760291,-11.9992823440159));
#57504=CARTESIAN_POINT('Ctrl Pts',(-50.,12.625949760291,-11.9992823440159));
#57505=CARTESIAN_POINT('Ctrl Pts',(-66.,12.5598923894368,-11.9863746440312));
#57506=CARTESIAN_POINT('Ctrl Pts',(-50.,12.5598923894368,-11.9863746440312));
#57507=CARTESIAN_POINT('Ctrl Pts',(-66.,12.4722630854199,-11.9683967893614));
#57508=CARTESIAN_POINT('Ctrl Pts',(-50.,12.4722630854199,-11.9683967893614));
#57509=CARTESIAN_POINT('Ctrl Pts',(-66.,12.3634750927067,-11.9446400762195));
#57510=CARTESIAN_POINT('Ctrl Pts',(-50.,12.3634750927067,-11.9446400762195));
#57511=CARTESIAN_POINT('Ctrl Pts',(-66.,12.2554397558718,-11.9195939429239));
#57512=CARTESIAN_POINT('Ctrl Pts',(-50.,12.2554397558718,-11.9195939429239));
#57513=CARTESIAN_POINT('Ctrl Pts',(-66.,12.1481604433561,-11.8932563267753));
#57514=CARTESIAN_POINT('Ctrl Pts',(-50.,12.1481604433561,-11.8932563267753));
#57515=CARTESIAN_POINT('Ctrl Pts',(-66.,12.0416388187435,-11.8656306582083));
#57516=CARTESIAN_POINT('Ctrl Pts',(-50.,12.0416388187435,-11.8656306582083));
#57517=CARTESIAN_POINT('Ctrl Pts',(-66.,11.9358727982571,-11.836729787751));
#57518=CARTESIAN_POINT('Ctrl Pts',(-50.,11.9358727982571,-11.836729787751));
#57519=CARTESIAN_POINT('Ctrl Pts',(-66.,11.8308626354082,-11.8065686091834));
#57520=CARTESIAN_POINT('Ctrl Pts',(-50.,11.8308626354082,-11.8065686091834));
#57521=CARTESIAN_POINT('Ctrl Pts',(-66.,11.7266178525644,-11.775155434854));
#57522=CARTESIAN_POINT('Ctrl Pts',(-50.,11.7266178525644,-11.775155434854));
#57523=CARTESIAN_POINT('Ctrl Pts',(-66.,11.6231644318358,-11.7424832844891));
#57524=CARTESIAN_POINT('Ctrl Pts',(-50.,11.6231644318358,-11.7424832844891));
#57525=CARTESIAN_POINT('Ctrl Pts',(-66.,11.520550522073,-11.7085227486112));
#57526=CARTESIAN_POINT('Ctrl Pts',(-50.,11.520550522073,-11.7085227486112));
#57527=CARTESIAN_POINT('Ctrl Pts',(-66.,11.4188563157544,-11.6732104524509));
#57528=CARTESIAN_POINT('Ctrl Pts',(-50.,11.4188563157544,-11.6732104524509));
#57529=CARTESIAN_POINT('Ctrl Pts',(-66.,11.3181783503234,-11.6364649635713));
#57530=CARTESIAN_POINT('Ctrl Pts',(-50.,11.3181783503234,-11.6364649635713));
#57531=CARTESIAN_POINT('Ctrl Pts',(-66.,11.2186075484415,-11.5982095077484));
#57532=CARTESIAN_POINT('Ctrl Pts',(-50.,11.2186075484415,-11.5982095077484));
#57533=CARTESIAN_POINT('Ctrl Pts',(-66.,11.1202074324343,-11.5583943876468));
#57534=CARTESIAN_POINT('Ctrl Pts',(-50.,11.1202074324343,-11.5583943876468));
#57535=CARTESIAN_POINT('Ctrl Pts',(-66.,11.0229961202521,-11.5170156697979));
#57536=CARTESIAN_POINT('Ctrl Pts',(-50.,11.0229961202521,-11.5170156697979));
#57537=CARTESIAN_POINT('Ctrl Pts',(-66.,10.926915885831,-11.4741464531626));
#57538=CARTESIAN_POINT('Ctrl Pts',(-50.,10.926915885831,-11.4741464531626));
#57539=CARTESIAN_POINT('Ctrl Pts',(-66.,10.8318699676878,-11.4299001604323));
#57540=CARTESIAN_POINT('Ctrl Pts',(-50.,10.8318699676878,-11.4299001604323));
#57541=CARTESIAN_POINT('Ctrl Pts',(-66.,10.737781584702,-11.3843713907704));
#57542=CARTESIAN_POINT('Ctrl Pts',(-50.,10.737781584702,-11.3843713907704));
#57543=CARTESIAN_POINT('Ctrl Pts',(-66.,10.6446491749193,-11.3375806355454));
#57544=CARTESIAN_POINT('Ctrl Pts',(-50.,10.6446491749193,-11.3375806355454));
#57545=CARTESIAN_POINT('Ctrl Pts',(-66.,10.5525953486849,-11.289425367888));
#57546=CARTESIAN_POINT('Ctrl Pts',(-50.,10.5525953486849,-11.289425367888));
#57547=CARTESIAN_POINT('Ctrl Pts',(-66.,10.4619396643774,-11.2396071151889));
#57548=CARTESIAN_POINT('Ctrl Pts',(-50.,10.4619396643774,-11.2396071151889));
#57549=CARTESIAN_POINT('Ctrl Pts',(-66.,10.3731363846505,-11.1876948686032));
#57550=CARTESIAN_POINT('Ctrl Pts',(-50.,10.3731363846505,-11.1876948686032));
#57551=CARTESIAN_POINT('Ctrl Pts',(-66.,10.2866665326243,-11.1332346082697));
#57552=CARTESIAN_POINT('Ctrl Pts',(-50.,10.2866665326243,-11.1332346082697));
#57553=CARTESIAN_POINT('Ctrl Pts',(-66.,10.2029412752749,-11.0758475399707));
#57554=CARTESIAN_POINT('Ctrl Pts',(-50.,10.2029412752749,-11.0758475399707));
#57555=CARTESIAN_POINT('Ctrl Pts',(-66.,10.1222086594491,-11.0153247237569));
#57556=CARTESIAN_POINT('Ctrl Pts',(-50.,10.1222086594491,-11.0153247237569));
#57557=CARTESIAN_POINT('Ctrl Pts',(-66.,10.0444356624493,-10.951747313668));
#57558=CARTESIAN_POINT('Ctrl Pts',(-50.,10.0444356624493,-10.951747313668));
#57559=CARTESIAN_POINT('Ctrl Pts',(-66.,9.9693612115878,-10.885429977536));
#57560=CARTESIAN_POINT('Ctrl Pts',(-50.,9.9693612115878,-10.885429977536));
#57561=CARTESIAN_POINT('Ctrl Pts',(-66.,9.89659308973021,-10.816818967327));
#57562=CARTESIAN_POINT('Ctrl Pts',(-50.,9.89659308973021,-10.816818967327));
#57563=CARTESIAN_POINT('Ctrl Pts',(-66.,9.82569013557624,-10.7464053109633));
#57564=CARTESIAN_POINT('Ctrl Pts',(-50.,9.82569013557624,-10.7464053109633));
#57565=CARTESIAN_POINT('Ctrl Pts',(-66.,9.75624684158698,-10.6746356328252));
#57566=CARTESIAN_POINT('Ctrl Pts',(-50.,9.75624684158698,-10.6746356328252));
#57567=CARTESIAN_POINT('Ctrl Pts',(-66.,9.68798490145875,-10.6018153909131));
#57568=CARTESIAN_POINT('Ctrl Pts',(-50.,9.68798490145875,-10.6018153909131));
#57569=CARTESIAN_POINT('Ctrl Pts',(-66.,9.62073647531797,-10.5281280338367));
#57570=CARTESIAN_POINT('Ctrl Pts',(-50.,9.62073647531797,-10.5281280338367));
#57571=CARTESIAN_POINT('Ctrl Pts',(-66.,9.56767882107163,-10.4685600648819));
#57572=CARTESIAN_POINT('Ctrl Pts',(-50.,9.56767882107163,-10.4685600648819));
#57573=CARTESIAN_POINT('Ctrl Pts',(-66.,9.52828841562115,-10.4235513483695));
#57574=CARTESIAN_POINT('Ctrl Pts',(-50.,9.52828841562115,-10.4235513483695));
#57575=CARTESIAN_POINT('Ctrl Pts',(-66.,9.50220693210954,-10.3933978635985));
#57576=CARTESIAN_POINT('Ctrl Pts',(-50.,9.50220693210954,-10.3933978635985));
#57577=CARTESIAN_POINT('Ctrl Pts',(-66.,9.48921088782658,-10.3782842019456));
#57578=CARTESIAN_POINT('Ctrl Pts',(-50.,9.48921088782658,-10.3782842019456));
#57579=CARTESIAN_POINT('Origin',(-65.75,0.,0.));
#57580=CARTESIAN_POINT('',(-65.5,8.6823221506088,-14.470069352738));
#57581=CARTESIAN_POINT('Origin',(-65.5,0.,0.));
#57582=CARTESIAN_POINT('Ctrl Pts',(-65.5,8.68232215060881,-14.470069352738));
#57583=CARTESIAN_POINT('Ctrl Pts',(-65.6931595476828,8.4892717682525,-14.3606405920574));
#57584=CARTESIAN_POINT('Ctrl Pts',(-65.8611256967192,8.32873016601974,-14.2599101133766));
#57585=CARTESIAN_POINT('Ctrl Pts',(-66.,8.19960777736701,-14.1741686633588));
#57586=CARTESIAN_POINT('Origin',(-58.,0.,0.));
#57587=CARTESIAN_POINT('',(-50.5,8.68232215060881,-14.470069352738));
#57588=CARTESIAN_POINT('Origin',(-50.5,0.,0.));
#57589=CARTESIAN_POINT('Ctrl Pts',(-50.5,8.6823221506088,-14.470069352738));
#57590=CARTESIAN_POINT('Ctrl Pts',(-55.5,8.6823221506088,-14.470069352738));
#57591=CARTESIAN_POINT('Ctrl Pts',(-60.5,8.68232215060881,-14.470069352738));
#57592=CARTESIAN_POINT('Ctrl Pts',(-65.5,8.68232215060881,-14.470069352738));
#57593=CARTESIAN_POINT('Origin',(-50.25,0.,0.));
#57594=CARTESIAN_POINT('Ctrl Pts',(-50.,8.199607777367,-14.1741686633588));
#57595=CARTESIAN_POINT('Ctrl Pts',(-50.1388743032879,8.32873016602638,-14.259910113381));
#57596=CARTESIAN_POINT('Ctrl Pts',(-50.3068404523237,8.48927176825896,-14.3606405920611));
#57597=CARTESIAN_POINT('Ctrl Pts',(-50.5,8.6823221506088,-14.470069352738));
#57598=CARTESIAN_POINT('Ctrl Pts',(-66.,5.35024281477071,-13.004953213026));
#57599=CARTESIAN_POINT('Ctrl Pts',(-50.,5.35024281477071,-13.004953213026));
#57600=CARTESIAN_POINT('Ctrl Pts',(-66.,5.36001566196946,-13.026183989773));
#57601=CARTESIAN_POINT('Ctrl Pts',(-50.,5.36001566196946,-13.026183989773));
#57602=CARTESIAN_POINT('Ctrl Pts',(-66.,5.37936086023753,-13.0687478607962));
#57603=CARTESIAN_POINT('Ctrl Pts',(-50.,5.37936086023753,-13.0687478607962));
#57604=CARTESIAN_POINT('Ctrl Pts',(-66.,5.40777718254589,-13.1329006212338));
#57605=CARTESIAN_POINT('Ctrl Pts',(-50.,5.40777718254589,-13.1329006212338));
#57606=CARTESIAN_POINT('Ctrl Pts',(-66.,5.44446094769152,-13.2190523479119));
#57607=CARTESIAN_POINT('Ctrl Pts',(-50.,5.44446094769152,-13.2190523479119));
#57608=CARTESIAN_POINT('Ctrl Pts',(-66.,5.48825134524296,-13.3277741560577));
#57609=CARTESIAN_POINT('Ctrl Pts',(-50.,5.48825134524296,-13.3277741560577));
#57610=CARTESIAN_POINT('Ctrl Pts',(-66.,5.52982166345111,-13.4375425451545));
#57611=CARTESIAN_POINT('Ctrl Pts',(-50.,5.52982166345111,-13.4375425451545));
#57612=CARTESIAN_POINT('Ctrl Pts',(-66.,5.56887590111916,-13.548380533239));
#57613=CARTESIAN_POINT('Ctrl Pts',(-50.,5.56887590111916,-13.548380533239));
#57614=CARTESIAN_POINT('Ctrl Pts',(-66.,5.60492122426722,-13.6603197171863));
#57615=CARTESIAN_POINT('Ctrl Pts',(-50.,5.60492122426722,-13.6603197171863));
#57616=CARTESIAN_POINT('Ctrl Pts',(-66.,5.63733210461441,-13.7734207288063));
#57617=CARTESIAN_POINT('Ctrl Pts',(-50.,5.63733210461441,-13.7734207288063));
#57618=CARTESIAN_POINT('Ctrl Pts',(-66.,5.66543360144756,-13.8878037235725));
#57619=CARTESIAN_POINT('Ctrl Pts',(-50.,5.66543360144756,-13.8878037235725));
#57620=CARTESIAN_POINT('Ctrl Pts',(-66.,5.68858274460417,-14.0036638891498));
#57621=CARTESIAN_POINT('Ctrl Pts',(-50.,5.68858274460417,-14.0036638891498));
#57622=CARTESIAN_POINT('Ctrl Pts',(-66.,5.7062391581791,-14.1213222951832));
#57623=CARTESIAN_POINT('Ctrl Pts',(-50.,5.7062391581791,-14.1213222951832));
#57624=CARTESIAN_POINT('Ctrl Pts',(-66.,5.71811860006313,-14.2411017202677));
#57625=CARTESIAN_POINT('Ctrl Pts',(-50.,5.71811860006313,-14.2411017202677));
#57626=CARTESIAN_POINT('Ctrl Pts',(-66.,5.7244278180311,-14.3630901368566));
#57627=CARTESIAN_POINT('Ctrl Pts',(-50.,5.7244278180311,-14.3630901368566));
#57628=CARTESIAN_POINT('Ctrl Pts',(-66.,5.72601142143879,-14.4869849640075));
#57629=CARTESIAN_POINT('Ctrl Pts',(-50.,5.72601142143879,-14.4869849640075));
#57630=CARTESIAN_POINT('Ctrl Pts',(-66.,5.72469186277131,-14.611792753182));
#57631=CARTESIAN_POINT('Ctrl Pts',(-50.,5.72469186277131,-14.611792753182));
#57632=CARTESIAN_POINT('Ctrl Pts',(-66.,5.72295493404455,-14.7359981218931));
#57633=CARTESIAN_POINT('Ctrl Pts',(-50.,5.72295493404455,-14.7359981218931));
#57634=CARTESIAN_POINT('Ctrl Pts',(-66.,5.72276984468895,-14.8583414088431));
#57635=CARTESIAN_POINT('Ctrl Pts',(-50.,5.72276984468895,-14.8583414088431));
#57636=CARTESIAN_POINT('Ctrl Pts',(-66.,5.72472760042901,-14.9783796615786));
#57637=CARTESIAN_POINT('Ctrl Pts',(-50.,5.72472760042901,-14.9783796615786));
#57638=CARTESIAN_POINT('Ctrl Pts',(-66.,5.72682550780959,-15.0972765365679));
#57639=CARTESIAN_POINT('Ctrl Pts',(-50.,5.72682550780959,-15.0972765365679));
#57640=CARTESIAN_POINT('Ctrl Pts',(-66.,5.72404344314264,-15.2180917854697));
#57641=CARTESIAN_POINT('Ctrl Pts',(-50.,5.72404344314264,-15.2180917854697));
#57642=CARTESIAN_POINT('Ctrl Pts',(-66.,5.7111041198627,-15.3440703755711));
#57643=CARTESIAN_POINT('Ctrl Pts',(-50.,5.7111041198627,-15.3440703755711));
#57644=CARTESIAN_POINT('Ctrl Pts',(-66.,5.68483553281663,-15.4771820371687));
#57645=CARTESIAN_POINT('Ctrl Pts',(-50.,5.68483553281663,-15.4771820371687));
#57646=CARTESIAN_POINT('Ctrl Pts',(-66.,5.64658095828703,-15.616629779452));
#57647=CARTESIAN_POINT('Ctrl Pts',(-50.,5.64658095828703,-15.616629779452));
#57648=CARTESIAN_POINT('Ctrl Pts',(-66.,5.60492018787097,-15.7571674475031));
#57649=CARTESIAN_POINT('Ctrl Pts',(-50.,5.60492018787097,-15.7571674475031));
#57650=CARTESIAN_POINT('Ctrl Pts',(-66.,5.57357690598309,-15.8903852761089));
#57651=CARTESIAN_POINT('Ctrl Pts',(-50.,5.57357690598309,-15.8903852761089));
#57652=CARTESIAN_POINT('Ctrl Pts',(-66.,5.5687561428657,-16.0063469743079));
#57653=CARTESIAN_POINT('Ctrl Pts',(-50.,5.5687561428657,-16.0063469743079));
#57654=CARTESIAN_POINT('Ctrl Pts',(-66.,5.60688031869652,-16.0949814047159));
#57655=CARTESIAN_POINT('Ctrl Pts',(-50.,5.60688031869652,-16.0949814047159));
#57656=CARTESIAN_POINT('Ctrl Pts',(-66.,5.70173196024853,-16.1478393830386));
#57657=CARTESIAN_POINT('Ctrl Pts',(-50.,5.70173196024853,-16.1478393830386));
#57658=CARTESIAN_POINT('Ctrl Pts',(-66.,5.8636852794496,-16.1585658291036));
#57659=CARTESIAN_POINT('Ctrl Pts',(-50.,5.8636852794496,-16.1585658291036));
#57660=CARTESIAN_POINT('Ctrl Pts',(-66.,6.10047136055145,-16.1224288386879));
#57661=CARTESIAN_POINT('Ctrl Pts',(-50.,6.10047136055145,-16.1224288386879));
#57662=CARTESIAN_POINT('Ctrl Pts',(-66.,6.41747875111399,-16.0361345338456));
#57663=CARTESIAN_POINT('Ctrl Pts',(-50.,6.41747875111399,-16.0361345338456));
#57664=CARTESIAN_POINT('Ctrl Pts',(-66.,6.8182230142718,-15.8975380663557));
#57665=CARTESIAN_POINT('Ctrl Pts',(-50.,6.8182230142718,-15.8975380663557));
#57666=CARTESIAN_POINT('Ctrl Pts',(-66.,7.30472306816663,-15.705412002146));
#57667=CARTESIAN_POINT('Ctrl Pts',(-50.,7.30472306816663,-15.705412002146));
#57668=CARTESIAN_POINT('Ctrl Pts',(-66.,7.87789865673363,-15.4592017657445));
#57669=CARTESIAN_POINT('Ctrl Pts',(-50.,7.87789865673363,-15.4592017657445));
#57670=CARTESIAN_POINT('Ctrl Pts',(-66.,8.40593301690788,-15.2188781604602));
#57671=CARTESIAN_POINT('Ctrl Pts',(-50.,8.40593301690788,-15.2188781604602));
#57672=CARTESIAN_POINT('Ctrl Pts',(-66.,8.84097325982172,-15.0142967817227));
#57673=CARTESIAN_POINT('Ctrl Pts',(-50.,8.84097325982172,-15.0142967817227));
#57674=CARTESIAN_POINT('Ctrl Pts',(-66.,9.14831679120446,-14.8671063944355));
#57675=CARTESIAN_POINT('Ctrl Pts',(-50.,9.14831679120446,-14.8671063944355));
#57676=CARTESIAN_POINT('Ctrl Pts',(-66.,9.30631773451278,-14.7908104992354));
#57677=CARTESIAN_POINT('Ctrl Pts',(-50.,9.30631773451278,-14.7908104992354));
#57678=CARTESIAN_POINT('',(-65.5,5.57616560087513,-15.9270839199025));
#57679=CARTESIAN_POINT('Ctrl Pts',(-66.,5.70745604345954,-15.3481455072584));
#57680=CARTESIAN_POINT('Ctrl Pts',(-65.7933280154029,5.67157216480773,-15.5819887038945));
#57681=CARTESIAN_POINT('Ctrl Pts',(-65.6370761749494,5.58469409422519,-15.7788636458467));
#57682=CARTESIAN_POINT('Ctrl Pts',(-65.5,5.57616560087513,-15.9270839199025));
#57683=CARTESIAN_POINT('',(-66.,5.35024281477071,-13.004953213026));
#57684=CARTESIAN_POINT('',(-50.5,5.57616560087513,-15.9270839199025));
#57685=CARTESIAN_POINT('Ctrl Pts',(-50.5,5.57616560087513,-15.9270839199025));
#57686=CARTESIAN_POINT('Ctrl Pts',(-50.4518618349118,5.57916062186248,-15.8750321900921));
#57687=CARTESIAN_POINT('Ctrl Pts',(-50.4012423593877,5.59158821763518,-15.8170054325664));
#57688=CARTESIAN_POINT('Ctrl Pts',(-50.2441129793791,5.63902638944085,-15.6333426788586));
#57689=CARTESIAN_POINT('Ctrl Pts',(-50.1366827452935,5.68372420067752,-15.5027979636459));
#57690=CARTESIAN_POINT('Ctrl Pts',(-50.,5.70745604345953,-15.3481455072584));
#57691=CARTESIAN_POINT('Ctrl Pts',(-65.5,5.57616560087513,-15.9270839199025));
#57692=CARTESIAN_POINT('Ctrl Pts',(-60.5,5.57616560087513,-15.9270839199025));
#57693=CARTESIAN_POINT('Ctrl Pts',(-55.5,5.57616560087513,-15.9270839199025));
#57694=CARTESIAN_POINT('Ctrl Pts',(-50.5,5.57616560087513,-15.9270839199025));
#57695=CARTESIAN_POINT('Origin',(-66.,0.,0.));
#57696=CARTESIAN_POINT('',(-66.,6.61011555120063,-12.4121021043889));
#57697=CARTESIAN_POINT('Ctrl Pts',(-66.,9.30631773451278,-14.7908104992354));
#57698=CARTESIAN_POINT('Ctrl Pts',(-50.,9.30631773451278,-14.7908104992354));
#57699=CARTESIAN_POINT('Ctrl Pts',(-66.,9.28590458706215,-14.7813250267199));
#57700=CARTESIAN_POINT('Ctrl Pts',(-50.,9.28590458706215,-14.7813250267199));
#57701=CARTESIAN_POINT('Ctrl Pts',(-66.,9.24518215888137,-14.7622488452778));
#57702=CARTESIAN_POINT('Ctrl Pts',(-50.,9.24518215888137,-14.7622488452778));
#57703=CARTESIAN_POINT('Ctrl Pts',(-66.,9.18441011625632,-14.7333188643196));
#57704=CARTESIAN_POINT('Ctrl Pts',(-50.,9.18441011625632,-14.7333188643196));
#57705=CARTESIAN_POINT('Ctrl Pts',(-66.,9.10400475861348,-14.6941132952849));
#57706=CARTESIAN_POINT('Ctrl Pts',(-50.,9.10400475861348,-14.6941132952849));
#57707=CARTESIAN_POINT('Ctrl Pts',(-66.,9.00454259504917,-14.6440484693391));
#57708=CARTESIAN_POINT('Ctrl Pts',(-50.,9.00454259504917,-14.6440484693391));
#57709=CARTESIAN_POINT('Ctrl Pts',(-66.,8.90613010704717,-14.5929219106503));
#57710=CARTESIAN_POINT('Ctrl Pts',(-50.,8.90613010704717,-14.5929219106503));
#57711=CARTESIAN_POINT('Ctrl Pts',(-66.,8.80877107019522,-14.5407324590199));
#57712=CARTESIAN_POINT('Ctrl Pts',(-50.,8.80877107019522,-14.5407324590199));
#57713=CARTESIAN_POINT('Ctrl Pts',(-66.,8.71246624269817,-14.4874838508255));
#57714=CARTESIAN_POINT('Ctrl Pts',(-50.,8.71246624269817,-14.4874838508255));
#57715=CARTESIAN_POINT('Ctrl Pts',(-66.,8.61721041044846,-14.433188014658));
#57716=CARTESIAN_POINT('Ctrl Pts',(-50.,8.61721041044846,-14.433188014658));
#57717=CARTESIAN_POINT('Ctrl Pts',(-66.,8.52300011506032,-14.3778594394275));
#57718=CARTESIAN_POINT('Ctrl Pts',(-50.,8.52300011506032,-14.3778594394275));
#57719=CARTESIAN_POINT('Ctrl Pts',(-66.,8.42984251254175,-14.3215085444515));
#57720=CARTESIAN_POINT('Ctrl Pts',(-50.,8.42984251254175,-14.3215085444515));
#57721=CARTESIAN_POINT('Ctrl Pts',(-66.,8.33776450465061,-14.2641350302423));
#57722=CARTESIAN_POINT('Ctrl Pts',(-50.,8.33776450465061,-14.2641350302423));
#57723=CARTESIAN_POINT('Ctrl Pts',(-66.,8.24682004139236,-14.2057223854076));
#57724=CARTESIAN_POINT('Ctrl Pts',(-50.,8.24682004139236,-14.2057223854076));
#57725=CARTESIAN_POINT('Ctrl Pts',(-66.,8.15710255651542,-14.1462291692713));
#57726=CARTESIAN_POINT('Ctrl Pts',(-50.,8.15710255651542,-14.1462291692713));
#57727=CARTESIAN_POINT('Ctrl Pts',(-66.,8.06872580598559,-14.0856005156321));
#57728=CARTESIAN_POINT('Ctrl Pts',(-50.,8.06872580598559,-14.0856005156321));
#57729=CARTESIAN_POINT('Ctrl Pts',(-66.,7.98179694893469,-14.0237846738158));
#57730=CARTESIAN_POINT('Ctrl Pts',(-50.,7.98179694893469,-14.0237846738158));
#57731=CARTESIAN_POINT('Ctrl Pts',(-66.,7.89638987124254,-13.9607493051802));
#57732=CARTESIAN_POINT('Ctrl Pts',(-50.,7.89638987124254,-13.9607493051802));
#57733=CARTESIAN_POINT('Ctrl Pts',(-66.,7.81252309986449,-13.8964951055849));
#57734=CARTESIAN_POINT('Ctrl Pts',(-50.,7.81252309986449,-13.8964951055849));
#57735=CARTESIAN_POINT('Ctrl Pts',(-66.,7.7301225433348,-13.8310785215643));
#57736=CARTESIAN_POINT('Ctrl Pts',(-50.,7.7301225433348,-13.8310785215643));
#57737=CARTESIAN_POINT('Ctrl Pts',(-66.,7.6490662730339,-13.7645853488249));
#57738=CARTESIAN_POINT('Ctrl Pts',(-50.,7.6490662730339,-13.7645853488249));
#57739=CARTESIAN_POINT('Ctrl Pts',(-66.,7.56925639420599,-13.6970881198352));
#57740=CARTESIAN_POINT('Ctrl Pts',(-50.,7.56925639420599,-13.6970881198352));
#57741=CARTESIAN_POINT('Ctrl Pts',(-66.,7.49068629797234,-13.6286062937474));
#57742=CARTESIAN_POINT('Ctrl Pts',(-50.,7.49068629797234,-13.6286062937474));
#57743=CARTESIAN_POINT('Ctrl Pts',(-66.,7.41350024004436,-13.5590710567155));
#57744=CARTESIAN_POINT('Ctrl Pts',(-50.,7.41350024004436,-13.5590710567155));
#57745=CARTESIAN_POINT('Ctrl Pts',(-66.,7.33808196640605,-13.4882727841331));
#57746=CARTESIAN_POINT('Ctrl Pts',(-50.,7.33808196640605,-13.4882727841331));
#57747=CARTESIAN_POINT('Ctrl Pts',(-66.,7.26497865575545,-13.4159069786186));
#57748=CARTESIAN_POINT('Ctrl Pts',(-50.,7.26497865575545,-13.4159069786186));
#57749=CARTESIAN_POINT('Ctrl Pts',(-66.,7.19476912913493,-13.3416535097654));
#57750=CARTESIAN_POINT('Ctrl Pts',(-50.,7.19476912913493,-13.3416535097654));
#57751=CARTESIAN_POINT('Ctrl Pts',(-66.,7.12794583824513,-13.2652477369413));
#57752=CARTESIAN_POINT('Ctrl Pts',(-50.,7.12794583824513,-13.2652477369413));
#57753=CARTESIAN_POINT('Ctrl Pts',(-66.,7.06480099833745,-13.1865489711723));
#57754=CARTESIAN_POINT('Ctrl Pts',(-50.,7.06480099833745,-13.1865489711723));
#57755=CARTESIAN_POINT('Ctrl Pts',(-66.,7.00528244199424,-13.1056276044837));
#57756=CARTESIAN_POINT('Ctrl Pts',(-50.,7.00528244199424,-13.1056276044837));
#57757=CARTESIAN_POINT('Ctrl Pts',(-66.,6.94905904389849,-13.0227234927017));
#57758=CARTESIAN_POINT('Ctrl Pts',(-50.,6.94905904389849,-13.0227234927017));
#57759=CARTESIAN_POINT('Ctrl Pts',(-66.,6.89563993078743,-12.9381713275312));
#57760=CARTESIAN_POINT('Ctrl Pts',(-50.,6.89563993078743,-12.9381713275312));
#57761=CARTESIAN_POINT('Ctrl Pts',(-66.,6.84447568757558,-12.8523369979956));
#57762=CARTESIAN_POINT('Ctrl Pts',(-50.,6.84447568757558,-12.8523369979956));
#57763=CARTESIAN_POINT('Ctrl Pts',(-66.,6.79506247552229,-12.7655522513249));
#57764=CARTESIAN_POINT('Ctrl Pts',(-50.,6.79506247552229,-12.7655522513249));
#57765=CARTESIAN_POINT('Ctrl Pts',(-66.,6.74705476751256,-12.6780437370314));
#57766=CARTESIAN_POINT('Ctrl Pts',(-50.,6.74705476751256,-12.6780437370314));
#57767=CARTESIAN_POINT('Ctrl Pts',(-66.,6.70024437485702,-12.5899474002701));
#57768=CARTESIAN_POINT('Ctrl Pts',(-50.,6.70024437485702,-12.5899474002701));
#57769=CARTESIAN_POINT('Ctrl Pts',(-66.,6.66366757586302,-12.5190559665502));
#57770=CARTESIAN_POINT('Ctrl Pts',(-50.,6.66366757586302,-12.5190559665502));
#57771=CARTESIAN_POINT('Ctrl Pts',(-66.,6.63670790506457,-12.4656652861453));
#57772=CARTESIAN_POINT('Ctrl Pts',(-50.,6.63670790506457,-12.4656652861453));
#57773=CARTESIAN_POINT('Ctrl Pts',(-66.,6.6189446860433,-12.4299729273552));
#57774=CARTESIAN_POINT('Ctrl Pts',(-50.,6.6189446860433,-12.4299729273552));
#57775=CARTESIAN_POINT('Ctrl Pts',(-66.,6.61011555120064,-12.4121021043889));
#57776=CARTESIAN_POINT('Ctrl Pts',(-50.,6.61011555120064,-12.4121021043889));
#57777=CARTESIAN_POINT('Origin',(-65.75,0.,0.));
#57778=CARTESIAN_POINT('',(-65.5,4.81099111997379,-16.1746712313893));
#57779=CARTESIAN_POINT('Origin',(-65.5,0.,0.));
#57780=CARTESIAN_POINT('Ctrl Pts',(-65.5,4.81099111997379,-16.1746712313893));
#57781=CARTESIAN_POINT('Ctrl Pts',(-65.6931595476677,4.65121959653276,-16.0206706986577));
#57782=CARTESIAN_POINT('Ctrl Pts',(-65.8611256967025,4.52077235532675,-15.8831797802523));
#57783=CARTESIAN_POINT('Ctrl Pts',(-66.,4.41702961547072,-15.7680206232759));
#57784=CARTESIAN_POINT('Origin',(-58.,0.,0.));
#57785=CARTESIAN_POINT('',(-50.5,4.81099111997379,-16.1746712313893));
#57786=CARTESIAN_POINT('Origin',(-50.5,0.,0.));
#57787=CARTESIAN_POINT('Ctrl Pts',(-50.5,4.81099111997379,-16.1746712313893));
#57788=CARTESIAN_POINT('Ctrl Pts',(-55.5,4.81099111997379,-16.1746712313893));
#57789=CARTESIAN_POINT('Ctrl Pts',(-60.5,4.81099111997379,-16.1746712313893));
#57790=CARTESIAN_POINT('Ctrl Pts',(-65.5,4.81099111997379,-16.1746712313893));
#57791=CARTESIAN_POINT('Origin',(-50.25,0.,0.));
#57792=CARTESIAN_POINT('Ctrl Pts',(-50.,4.41702961547073,-15.7680206232759));
#57793=CARTESIAN_POINT('Ctrl Pts',(-50.1388743032811,4.52077235531448,-15.8831797802387));
#57794=CARTESIAN_POINT('Ctrl Pts',(-50.3068404523174,4.65121959652049,-16.0206706986458));
#57795=CARTESIAN_POINT('Ctrl Pts',(-50.5,4.81099111997378,-16.1746712313893));
#57796=CARTESIAN_POINT('Ctrl Pts',(-66.,1.94795475120472,-13.9269299753125));
#57797=CARTESIAN_POINT('Ctrl Pts',(-50.,1.94795475120472,-13.9269299753125));
#57798=CARTESIAN_POINT('Ctrl Pts',(-66.,1.95214068696407,-13.9499241564345));
#57799=CARTESIAN_POINT('Ctrl Pts',(-50.,1.95214068696407,-13.9499241564345));
#57800=CARTESIAN_POINT('Ctrl Pts',(-66.,1.96029291597316,-13.9959617603545));
#57801=CARTESIAN_POINT('Ctrl Pts',(-50.,1.96029291597316,-13.9959617603545));
#57802=CARTESIAN_POINT('Ctrl Pts',(-66.,1.9718623445077,-14.0651658958429));
#57803=CARTESIAN_POINT('Ctrl Pts',(-50.,1.9718623445077,-14.0651658958429));
#57804=CARTESIAN_POINT('Ctrl Pts',(-66.,1.98596855852791,-14.1577338890203));
#57805=CARTESIAN_POINT('Ctrl Pts',(-50.,1.98596855852791,-14.1577338890203));
#57806=CARTESIAN_POINT('Ctrl Pts',(-66.,2.00134518601523,-14.2739302306637));
#57807=CARTESIAN_POINT('Ctrl Pts',(-50.,2.00134518601523,-14.2739302306637));
#57808=CARTESIAN_POINT('Ctrl Pts',(-66.,2.01431120793567,-14.3905881617116));
#57809=CARTESIAN_POINT('Ctrl Pts',(-50.,2.01431120793567,-14.3905881617116));
#57810=CARTESIAN_POINT('Ctrl Pts',(-66.,2.02457419816135,-14.5076563645426));
#57811=CARTESIAN_POINT('Ctrl Pts',(-50.,2.02457419816135,-14.5076563645426));
#57812=CARTESIAN_POINT('Ctrl Pts',(-66.,2.03164894817481,-14.625042880531));
#57813=CARTESIAN_POINT('Ctrl Pts',(-50.,2.03164894817481,-14.625042880531));
#57814=CARTESIAN_POINT('Ctrl Pts',(-66.,2.03491450329845,-14.7426508740692));
#57815=CARTESIAN_POINT('Ctrl Pts',(-50.,2.03491450329845,-14.7426508740692));
#57816=CARTESIAN_POINT('Ctrl Pts',(-66.,2.03368724587156,-14.8604288747958));
#57817=CARTESIAN_POINT('Ctrl Pts',(-50.,2.03368724587156,-14.8604288747958));
#57818=CARTESIAN_POINT('Ctrl Pts',(-66.,2.02729586462329,-14.9784060380191));
#57819=CARTESIAN_POINT('Ctrl Pts',(-50.,2.02729586462329,-14.9784060380191));
#57820=CARTESIAN_POINT('Ctrl Pts',(-66.,2.01513711377743,-15.096758960368));
#57821=CARTESIAN_POINT('Ctrl Pts',(-50.,2.01513711377743,-15.096758960368));
#57822=CARTESIAN_POINT('Ctrl Pts',(-66.,1.99685540944097,-15.2157295916163));
#57823=CARTESIAN_POINT('Ctrl Pts',(-50.,1.99685540944097,-15.2157295916163));
#57824=CARTESIAN_POINT('Ctrl Pts',(-66.,1.97262912616775,-15.3354545564815));
#57825=CARTESIAN_POINT('Ctrl Pts',(-50.,1.97262912616775,-15.3354545564815));
#57826=CARTESIAN_POINT('Ctrl Pts',(-66.,1.94335158717786,-15.4558508259636));
#57827=CARTESIAN_POINT('Ctrl Pts',(-50.,1.94335158717786,-15.4558508259636));
#57828=CARTESIAN_POINT('Ctrl Pts',(-66.,1.91103504986532,-15.5764093880396));
#57829=CARTESIAN_POINT('Ctrl Pts',(-50.,1.91103504986532,-15.5764093880396));
#57830=CARTESIAN_POINT('Ctrl Pts',(-66.,1.87846407081847,-15.6962806600859));
#57831=CARTESIAN_POINT('Ctrl Pts',(-50.,1.87846407081847,-15.6962806600859));
#57832=CARTESIAN_POINT('Ctrl Pts',(-66.,1.84785925815835,-15.8147342778518));
#57833=CARTESIAN_POINT('Ctrl Pts',(-50.,1.84785925815835,-15.8147342778518));
#57834=CARTESIAN_POINT('Ctrl Pts',(-66.,1.81990320787353,-15.9314881821968));
#57835=CARTESIAN_POINT('Ctrl Pts',(-50.,1.81990320787353,-15.9314881821968));
#57836=CARTESIAN_POINT('Ctrl Pts',(-66.,1.79236675521062,-16.047171421572));
#57837=CARTESIAN_POINT('Ctrl Pts',(-50.,1.79236675521062,-16.047171421572));
#57838=CARTESIAN_POINT('Ctrl Pts',(-66.,1.75962656360386,-16.1634991659178));
#57839=CARTESIAN_POINT('Ctrl Pts',(-50.,1.75962656360386,-16.1634991659178));
#57840=CARTESIAN_POINT('Ctrl Pts',(-66.,1.71576415160101,-16.2823020281062));
#57841=CARTESIAN_POINT('Ctrl Pts',(-50.,1.71576415160101,-16.2823020281062));
#57842=CARTESIAN_POINT('Ctrl Pts',(-66.,1.65721731641851,-16.404699010131));
#57843=CARTESIAN_POINT('Ctrl Pts',(-50.,1.65721731641851,-16.404699010131));
#57844=CARTESIAN_POINT('Ctrl Pts',(-66.,1.58548533639917,-16.5302522193407));
#57845=CARTESIAN_POINT('Ctrl Pts',(-50.,1.58548533639917,-16.5302522193407));
#57846=CARTESIAN_POINT('Ctrl Pts',(-66.,1.51018311888448,-16.6560140258254));
#57847=CARTESIAN_POINT('Ctrl Pts',(-50.,1.51018311888448,-16.6560140258254));
#57848=CARTESIAN_POINT('Ctrl Pts',(-66.,1.44669461706905,-16.777251814139));
#57849=CARTESIAN_POINT('Ctrl Pts',(-50.,1.44669461706905,-16.777251814139));
#57850=CARTESIAN_POINT('Ctrl Pts',(-66.,1.4131868054492,-16.8883714873147));
#57851=CARTESIAN_POINT('Ctrl Pts',(-50.,1.4131868054492,-16.8883714873147));
#57852=CARTESIAN_POINT('Ctrl Pts',(-66.,1.42807075369374,-16.9837024010898));
#57853=CARTESIAN_POINT('Ctrl Pts',(-50.,1.42807075369374,-16.9837024010898));
#57854=CARTESIAN_POINT('Ctrl Pts',(-66.,1.5067972118416,-17.0584883928594));
#57855=CARTESIAN_POINT('Ctrl Pts',(-50.,1.5067972118416,-17.0584883928594));
#57856=CARTESIAN_POINT('Ctrl Pts',(-66.,1.66099491104707,-17.1091540005748));
#57857=CARTESIAN_POINT('Ctrl Pts',(-50.,1.66099491104707,-17.1091540005748));
#57858=CARTESIAN_POINT('Ctrl Pts',(-66.,1.89932882606092,-17.1330386239557));
#57859=CARTESIAN_POINT('Ctrl Pts',(-50.,1.89932882606092,-17.1330386239557));
#57860=CARTESIAN_POINT('Ctrl Pts',(-66.,2.22783736744731,-17.1282919455736));
#57861=CARTESIAN_POINT('Ctrl Pts',(-50.,2.22783736744731,-17.1282919455736));
#57862=CARTESIAN_POINT('Ctrl Pts',(-66.,2.65045905252241,-17.0937107865576));
#57863=CARTESIAN_POINT('Ctrl Pts',(-50.,2.65045905252241,-17.0937107865576));
#57864=CARTESIAN_POINT('Ctrl Pts',(-66.,3.16945462184284,-17.028608359459));
#57865=CARTESIAN_POINT('Ctrl Pts',(-50.,3.16945462184284,-17.028608359459));
#57866=CARTESIAN_POINT('Ctrl Pts',(-66.,3.78585284120834,-16.9326762428294));
#57867=CARTESIAN_POINT('Ctrl Pts',(-50.,3.78585284120834,-16.9326762428294));
#57868=CARTESIAN_POINT('Ctrl Pts',(-66.,4.35706408125165,-16.8312196509802));
#57869=CARTESIAN_POINT('Ctrl Pts',(-50.,4.35706408125165,-16.8312196509802));
#57870=CARTESIAN_POINT('Ctrl Pts',(-66.,4.82931405494557,-16.741255681377));
#57871=CARTESIAN_POINT('Ctrl Pts',(-50.,4.82931405494557,-16.741255681377));
#57872=CARTESIAN_POINT('Ctrl Pts',(-66.,5.1636065849309,-16.675122778911));
#57873=CARTESIAN_POINT('Ctrl Pts',(-50.,5.1636065849309,-16.675122778911));
#57874=CARTESIAN_POINT('Ctrl Pts',(-66.,5.33561765563024,-16.6405170963203));
#57875=CARTESIAN_POINT('Ctrl Pts',(-50.,5.33561765563024,-16.6405170963203));
#57876=CARTESIAN_POINT('',(-65.5,1.44007540176665,-16.8134412847943));
#57877=CARTESIAN_POINT('Ctrl Pts',(-66.,1.71121724218688,-16.2853418923289));
#57878=CARTESIAN_POINT('Ctrl Pts',(-65.793328015403,1.61830628338315,-16.5029145172019));
#57879=CARTESIAN_POINT('Ctrl Pts',(-65.6370761749494,1.48519684004577,-16.671998573255));
#57880=CARTESIAN_POINT('Ctrl Pts',(-65.5,1.44007540176665,-16.8134412847943));
#57881=CARTESIAN_POINT('',(-66.,1.94795475120472,-13.9269299753125));
#57882=CARTESIAN_POINT('',(-50.5,1.44007540176665,-16.8134412847943));
#57883=CARTESIAN_POINT('Ctrl Pts',(-50.5,1.44007540176665,-16.8134412847943));
#57884=CARTESIAN_POINT('Ctrl Pts',(-50.4518618349121,1.45592106747543,-16.763769687224));
#57885=CARTESIAN_POINT('Ctrl Pts',(-50.4012423593882,1.48238889525558,-16.7106565643805));
#57886=CARTESIAN_POINT('Ctrl Pts',(-50.2441129793797,1.57401177915707,-16.5445613074064));
#57887=CARTESIAN_POINT('Ctrl Pts',(-50.1366827452939,1.64977047695671,-16.4292337881098));
#57888=CARTESIAN_POINT('Ctrl Pts',(-50.,1.71121724218688,-16.2853418923289));
#57889=CARTESIAN_POINT('Ctrl Pts',(-65.5,1.44007540176665,-16.8134412847943));
#57890=CARTESIAN_POINT('Ctrl Pts',(-60.5,1.44007540176665,-16.8134412847943));
#57891=CARTESIAN_POINT('Ctrl Pts',(-55.5,1.44007540176665,-16.8134412847943));
#57892=CARTESIAN_POINT('Ctrl Pts',(-50.5,1.44007540176665,-16.8134412847943));
#57893=CARTESIAN_POINT('Origin',(-66.,0.,0.));
#57894=CARTESIAN_POINT('',(-66.,3.31568234418831,-13.6660219830951));
#57895=CARTESIAN_POINT('Ctrl Pts',(-66.,5.33561765563024,-16.6405170963203));
#57896=CARTESIAN_POINT('Ctrl Pts',(-50.,5.33561765563024,-16.6405170963203));
#57897=CARTESIAN_POINT('Ctrl Pts',(-66.,5.3182047658335,-16.6262530840302));
#57898=CARTESIAN_POINT('Ctrl Pts',(-50.,5.3182047658335,-16.6262530840302));
#57899=CARTESIAN_POINT('Ctrl Pts',(-66.,5.28350576102771,-16.5976489598374));
#57900=CARTESIAN_POINT('Ctrl Pts',(-50.,5.28350576102771,-16.5976489598374));
#57901=CARTESIAN_POINT('Ctrl Pts',(-66.,5.23183757757387,-16.5545144750063));
#57902=CARTESIAN_POINT('Ctrl Pts',(-50.,5.23183757757387,-16.5545144750063));
#57903=CARTESIAN_POINT('Ctrl Pts',(-66.,5.16370833063597,-16.4965446216971));
#57904=CARTESIAN_POINT('Ctrl Pts',(-50.,5.16370833063597,-16.4965446216971));
#57905=CARTESIAN_POINT('Ctrl Pts',(-66.,5.07982156975354,-16.4233174400873));
#57906=CARTESIAN_POINT('Ctrl Pts',(-50.,5.07982156975354,-16.4233174400873));
#57907=CARTESIAN_POINT('Ctrl Pts',(-66.,4.99721554914146,-16.349322925718));
#57908=CARTESIAN_POINT('Ctrl Pts',(-50.,4.99721554914146,-16.349322925718));
#57909=CARTESIAN_POINT('Ctrl Pts',(-66.,4.91589421430013,-16.2745608937911));
#57910=CARTESIAN_POINT('Ctrl Pts',(-50.,4.91589421430013,-16.2745608937911));
#57911=CARTESIAN_POINT('Ctrl Pts',(-66.,4.83585737041464,-16.1990351518568));
#57912=CARTESIAN_POINT('Ctrl Pts',(-50.,4.83585737041464,-16.1990351518568));
#57913=CARTESIAN_POINT('Ctrl Pts',(-66.,4.7570970006683,-16.1227559570515));
#57914=CARTESIAN_POINT('Ctrl Pts',(-50.,4.7570970006683,-16.1227559570515));
#57915=CARTESIAN_POINT('Ctrl Pts',(-66.,4.67960615208147,-16.0457364830242));
#57916=CARTESIAN_POINT('Ctrl Pts',(-50.,4.67960615208147,-16.0457364830242));
#57917=CARTESIAN_POINT('Ctrl Pts',(-66.,4.60338916466408,-15.967988601377));
#57918=CARTESIAN_POINT('Ctrl Pts',(-50.,4.60338916466408,-15.967988601377));
#57919=CARTESIAN_POINT('Ctrl Pts',(-66.,4.52847216948537,-15.8895187122264));
#57920=CARTESIAN_POINT('Ctrl Pts',(-50.,4.52847216948537,-15.8895187122264));
#57921=CARTESIAN_POINT('Ctrl Pts',(-66.,4.45491152782849,-15.8103242397366));
#57922=CARTESIAN_POINT('Ctrl Pts',(-50.,4.45491152782849,-15.8103242397366));
#57923=CARTESIAN_POINT('Ctrl Pts',(-66.,4.38280804392589,-15.7303882811948));
#57924=CARTESIAN_POINT('Ctrl Pts',(-50.,4.38280804392589,-15.7303882811948));
#57925=CARTESIAN_POINT('Ctrl Pts',(-66.,4.31228554455994,-15.6496859840807));
#57926=CARTESIAN_POINT('Ctrl Pts',(-50.,4.31228554455994,-15.6496859840807));
#57927=CARTESIAN_POINT('Ctrl Pts',(-66.,4.24346069213056,-15.5681938729551));
#57928=CARTESIAN_POINT('Ctrl Pts',(-50.,4.24346069213056,-15.5681938729551));
#57929=CARTESIAN_POINT('Ctrl Pts',(-66.,4.17641309355012,-15.4858989998248));
#57930=CARTESIAN_POINT('Ctrl Pts',(-50.,4.17641309355012,-15.4858989998248));
#57931=CARTESIAN_POINT('Ctrl Pts',(-66.,4.11116052066234,-15.4028066461541));
#57932=CARTESIAN_POINT('Ctrl Pts',(-50.,4.11116052066234,-15.4028066461541));
#57933=CARTESIAN_POINT('Ctrl Pts',(-66.,4.04761717203886,-15.3189530593075));
#57934=CARTESIAN_POINT('Ctrl Pts',(-50.,4.04761717203886,-15.3189530593075));
#57935=CARTESIAN_POINT('Ctrl Pts',(-66.,3.98564361314731,-15.2343910171469));
#57936=CARTESIAN_POINT('Ctrl Pts',(-50.,3.98564361314731,-15.2343910171469));
#57937=CARTESIAN_POINT('Ctrl Pts',(-66.,3.92512698668427,-15.1491664279643));
#57938=CARTESIAN_POINT('Ctrl Pts',(-50.,3.92512698668427,-15.1491664279643));
#57939=CARTESIAN_POINT('Ctrl Pts',(-66.,3.8660560521067,-15.0632964960055));
#57940=CARTESIAN_POINT('Ctrl Pts',(-50.,3.8660560521067,-15.0632964960055));
#57941=CARTESIAN_POINT('Ctrl Pts',(-66.,3.80858764637521,-14.9767504442745));
#57942=CARTESIAN_POINT('Ctrl Pts',(-50.,3.80858764637521,-14.9767504442745));
#57943=CARTESIAN_POINT('Ctrl Pts',(-66.,3.75314559090774,-14.8894206676529));
#57944=CARTESIAN_POINT('Ctrl Pts',(-50.,3.75314559090774,-14.8894206676529));
#57945=CARTESIAN_POINT('Ctrl Pts',(-66.,3.7003355991968,-14.801148312913));
#57946=CARTESIAN_POINT('Ctrl Pts',(-50.,3.7003355991968,-14.801148312913));
#57947=CARTESIAN_POINT('Ctrl Pts',(-66.,3.65079792075207,-14.7117672540732));
#57948=CARTESIAN_POINT('Ctrl Pts',(-50.,3.65079792075207,-14.7117672540732));
#57949=CARTESIAN_POINT('Ctrl Pts',(-66.,3.60507534944737,-14.6211436324314));
#57950=CARTESIAN_POINT('Ctrl Pts',(-50.,3.60507534944737,-14.6211436324314));
#57951=CARTESIAN_POINT('Ctrl Pts',(-66.,3.56348590797974,-14.5292138499942));
#57952=CARTESIAN_POINT('Ctrl Pts',(-50.,3.56348590797974,-14.5292138499942));
#57953=CARTESIAN_POINT('Ctrl Pts',(-66.,3.52596156208203,-14.436033113783));
#57954=CARTESIAN_POINT('Ctrl Pts',(-50.,3.52596156208203,-14.436033113783));
#57955=CARTESIAN_POINT('Ctrl Pts',(-66.,3.49212193962963,-14.3417513965941));
#57956=CARTESIAN_POINT('Ctrl Pts',(-50.,3.49212193962963,-14.3417513965941));
#57957=CARTESIAN_POINT('Ctrl Pts',(-66.,3.46140835460361,-14.246570799961));
#57958=CARTESIAN_POINT('Ctrl Pts',(-50.,3.46140835460361,-14.246570799961));
#57959=CARTESIAN_POINT('Ctrl Pts',(-66.,3.43319765990381,-14.1507090838548));
#57960=CARTESIAN_POINT('Ctrl Pts',(-50.,3.43319765990381,-14.1507090838548));
#57961=CARTESIAN_POINT('Ctrl Pts',(-66.,3.40691934362888,-14.0543622734568));
#57962=CARTESIAN_POINT('Ctrl Pts',(-50.,3.40691934362888,-14.0543622734568));
#57963=CARTESIAN_POINT('Ctrl Pts',(-66.,3.38218236859189,-13.9576639685687));
#57964=CARTESIAN_POINT('Ctrl Pts',(-50.,3.38218236859189,-13.9576639685687));
#57965=CARTESIAN_POINT('Ctrl Pts',(-66.,3.35875127854871,-13.860694068957));
#57966=CARTESIAN_POINT('Ctrl Pts',(-50.,3.35875127854871,-13.860694068957));
#57967=CARTESIAN_POINT('Ctrl Pts',(-66.,3.34095358960791,-13.7829335399729));
#57968=CARTESIAN_POINT('Ctrl Pts',(-50.,3.34095358960791,-13.7829335399729));
#57969=CARTESIAN_POINT('Ctrl Pts',(-66.,3.3281186287285,-13.7245156284827));
#57970=CARTESIAN_POINT('Ctrl Pts',(-50.,3.3281186287285,-13.7245156284827));
#57971=CARTESIAN_POINT('Ctrl Pts',(-66.,3.31978980257722,-13.6855270778435));
#57972=CARTESIAN_POINT('Ctrl Pts',(-50.,3.31978980257722,-13.6855270778435));
#57973=CARTESIAN_POINT('Ctrl Pts',(-66.,3.31568234418832,-13.6660219830951));
#57974=CARTESIAN_POINT('Ctrl Pts',(-50.,3.31568234418832,-13.6660219830951));
#57975=CARTESIAN_POINT('Origin',(-65.75,0.,0.));
#57976=CARTESIAN_POINT('',(-65.5,0.637367823683143,-16.8629590302928));
#57977=CARTESIAN_POINT('Origin',(-65.5,0.,0.));
#57978=CARTESIAN_POINT('Ctrl Pts',(-65.5,0.637367823683148,-16.8629590302928));
#57979=CARTESIAN_POINT('Ctrl Pts',(-65.5824396971602,0.587667004731077,
-16.7823408476978));
#57980=CARTESIAN_POINT('Ctrl Pts',(-65.6660036204853,0.539005134923334,
-16.7003659612199));
#57981=CARTESIAN_POINT('Ctrl Pts',(-65.7496756578578,0.492037124098817,
-16.6180469545161));
#57982=CARTESIAN_POINT('Ctrl Pts',(-65.8190041635689,0.45312063408684,-16.5498395353398));
#57983=CARTESIAN_POINT('Ctrl Pts',(-65.8884068934103,0.415362256265888,
-16.4813977166555));
#57984=CARTESIAN_POINT('Ctrl Pts',(-65.9573058363633,0.379170886061448,
-16.4133154040527));
#57985=CARTESIAN_POINT('Ctrl Pts',(-65.9715604948122,0.371683171461654,
-16.3992297001077));
#57986=CARTESIAN_POINT('Ctrl Pts',(-65.9857935889606,0.364262713372718,
-16.385159414606));
#57987=CARTESIAN_POINT('Ctrl Pts',(-66.,0.35691323813583,-16.3711098567093));
#57988=CARTESIAN_POINT('Origin',(-58.,0.,0.));
#57989=CARTESIAN_POINT('',(-50.5,0.637367823683145,-16.8629590302928));
#57990=CARTESIAN_POINT('Origin',(-50.5,0.,0.));
#57991=CARTESIAN_POINT('Ctrl Pts',(-50.5,0.637367823683145,-16.8629590302928));
#57992=CARTESIAN_POINT('Ctrl Pts',(-55.5,0.637367823683145,-16.8629590302928));
#57993=CARTESIAN_POINT('Ctrl Pts',(-60.5,0.637367823683144,-16.8629590302928));
#57994=CARTESIAN_POINT('Ctrl Pts',(-65.5,0.637367823683144,-16.8629590302928));
#57995=CARTESIAN_POINT('Origin',(-50.25,0.,0.));
#57996=CARTESIAN_POINT('Ctrl Pts',(-50.,0.356913238135828,-16.3711098567093));
#57997=CARTESIAN_POINT('Ctrl Pts',(-50.0728233300466,0.394587303694001,
-16.4431291435567));
#57998=CARTESIAN_POINT('Ctrl Pts',(-50.1463478065558,0.434124407382829,
-16.5156921628394));
#57999=CARTESIAN_POINT('Ctrl Pts',(-50.2198839404944,0.47502746617852,-16.5880885420746));
#58000=CARTESIAN_POINT('Ctrl Pts',(-50.3051443233005,0.52245191269314,-16.6720274531483));
#58001=CARTESIAN_POINT('Ctrl Pts',(-50.3904203770725,0.571717341873418,
-16.7557397783304));
#58002=CARTESIAN_POINT('Ctrl Pts',(-50.4746374523709,0.622131372875589,
-16.8381489075303));
#58003=CARTESIAN_POINT('Ctrl Pts',(-50.4831026982763,0.627198838921015,
-16.8464324241576));
#58004=CARTESIAN_POINT('Ctrl Pts',(-50.4915572446203,0.632277898913462,
-16.8547028185617));
#58005=CARTESIAN_POINT('Ctrl Pts',(-50.5,0.637367823683148,-16.8629590302928));
#58006=CARTESIAN_POINT('Ctrl Pts',(-66.,-1.57673047345591,-13.9738265075847));
#58007=CARTESIAN_POINT('Ctrl Pts',(-50.,-1.57673047345591,-13.9738265075847));
#58008=CARTESIAN_POINT('Ctrl Pts',(-66.,-1.57839446687451,-13.997139284115));
#58009=CARTESIAN_POINT('Ctrl Pts',(-50.,-1.57839446687451,-13.997139284115));
#58010=CARTESIAN_POINT('Ctrl Pts',(-66.,-1.58194744165485,-14.0437579089631));
#58011=CARTESIAN_POINT('Ctrl Pts',(-50.,-1.58194744165485,-14.0437579089631));
#58012=CARTESIAN_POINT('Ctrl Pts',(-66.,-1.58795185663835,-14.1136650691543));
#58013=CARTESIAN_POINT('Ctrl Pts',(-50.,-1.58795185663835,-14.1136650691543));
#58014=CARTESIAN_POINT('Ctrl Pts',(-66.,-1.59730953904946,-14.2068329413785));
#58015=CARTESIAN_POINT('Ctrl Pts',(-50.,-1.59730953904946,-14.2068329413785));
#58016=CARTESIAN_POINT('Ctrl Pts',(-66.,-1.61131285168258,-14.3232027730338));
#58017=CARTESIAN_POINT('Ctrl Pts',(-50.,-1.61131285168258,-14.3232027730338));
#58018=CARTESIAN_POINT('Ctrl Pts',(-66.,-1.6277658288928,-14.4394201991873));
#58019=CARTESIAN_POINT('Ctrl Pts',(-50.,-1.6277658288928,-14.4394201991873));
#58020=CARTESIAN_POINT('Ctrl Pts',(-66.,-1.64693894753001,-14.5553627910342));
#58021=CARTESIAN_POINT('Ctrl Pts',(-50.,-1.64693894753001,-14.5553627910342));
#58022=CARTESIAN_POINT('Ctrl Pts',(-66.,-1.6692793032136,-14.6708208125467));
#58023=CARTESIAN_POINT('Ctrl Pts',(-50.,-1.6692793032136,-14.6708208125467));
#58024=CARTESIAN_POINT('Ctrl Pts',(-66.,-1.69536426015181,-14.7855460452371));
#58025=CARTESIAN_POINT('Ctrl Pts',(-50.,-1.69536426015181,-14.7855460452371));
#58026=CARTESIAN_POINT('Ctrl Pts',(-66.,-1.72584315874106,-14.8993186269813));
#58027=CARTESIAN_POINT('Ctrl Pts',(-50.,-1.72584315874106,-14.8993186269813));
#58028=CARTESIAN_POINT('Ctrl Pts',(-66.,-1.76137347040452,-15.0119998487957));
#58029=CARTESIAN_POINT('Ctrl Pts',(-50.,-1.76137347040452,-15.0119998487957));
#58030=CARTESIAN_POINT('Ctrl Pts',(-66.,-1.80258340663877,-15.1236107380773));
#58031=CARTESIAN_POINT('Ctrl Pts',(-50.,-1.80258340663877,-15.1236107380773));
#58032=CARTESIAN_POINT('Ctrl Pts',(-66.,-1.84987755047685,-15.2342972131845));
#58033=CARTESIAN_POINT('Ctrl Pts',(-50.,-1.84987755047685,-15.2342972131845));
#58034=CARTESIAN_POINT('Ctrl Pts',(-66.,-1.90311710851519,-15.3442359664661));
#58035=CARTESIAN_POINT('Ctrl Pts',(-50.,-1.90311710851519,-15.3442359664661));
#58036=CARTESIAN_POINT('Ctrl Pts',(-66.,-1.96141617445265,-15.4535687378813));
#58037=CARTESIAN_POINT('Ctrl Pts',(-50.,-1.96141617445265,-15.4535687378813));
#58038=CARTESIAN_POINT('Ctrl Pts',(-66.,-2.02269912351901,-15.5623029350202));
#58039=CARTESIAN_POINT('Ctrl Pts',(-50.,-2.02269912351901,-15.5623029350202));
#58040=CARTESIAN_POINT('Ctrl Pts',(-66.,-2.08405759848474,-15.6703081575233));
#58041=CARTESIAN_POINT('Ctrl Pts',(-50.,-2.08405759848474,-15.6703081575233));
#58042=CARTESIAN_POINT('Ctrl Pts',(-66.,-2.14315912151332,-15.777429229659));
#58043=CARTESIAN_POINT('Ctrl Pts',(-50.,-2.14315912151332,-15.777429229659));
#58044=CARTESIAN_POINT('Ctrl Pts',(-66.,-2.19927239636847,-15.8835627084126));
#58045=CARTESIAN_POINT('Ctrl Pts',(-50.,-2.19927239636847,-15.8835627084126));
#58046=CARTESIAN_POINT('Ctrl Pts',(-66.,-2.25471299248206,-15.9887635087906));
#58047=CARTESIAN_POINT('Ctrl Pts',(-50.,-2.25471299248206,-15.9887635087906));
#58048=CARTESIAN_POINT('Ctrl Pts',(-66.,-2.31535412437999,-16.0932944485795));
#58049=CARTESIAN_POINT('Ctrl Pts',(-50.,-2.31535412437999,-16.0932944485795));
#58050=CARTESIAN_POINT('Ctrl Pts',(-66.,-2.38738358844493,-16.1974567620974));
#58051=CARTESIAN_POINT('Ctrl Pts',(-50.,-2.38738358844493,-16.1974567620974));
#58052=CARTESIAN_POINT('Ctrl Pts',(-66.,-2.47452995878914,-16.3014484120242));
#58053=CARTESIAN_POINT('Ctrl Pts',(-50.,-2.47452995878914,-16.3014484120242));
#58054=CARTESIAN_POINT('Ctrl Pts',(-66.,-2.57523216018184,-16.4052181182732));
#58055=CARTESIAN_POINT('Ctrl Pts',(-50.,-2.57523216018184,-16.4052181182732));
#58056=CARTESIAN_POINT('Ctrl Pts',(-66.,-2.67944430952652,-16.5083019863704));
#58057=CARTESIAN_POINT('Ctrl Pts',(-50.,-2.67944430952652,-16.5083019863704));
#58058=CARTESIAN_POINT('Ctrl Pts',(-66.,-2.77108881520607,-16.6099419182707));
#58059=CARTESIAN_POINT('Ctrl Pts',(-50.,-2.77108881520607,-16.6099419182707));
#58060=CARTESIAN_POINT('Ctrl Pts',(-66.,-2.83117825629119,-16.7092375086879));
#58061=CARTESIAN_POINT('Ctrl Pts',(-50.,-2.83117825629119,-16.7092375086879));
#58062=CARTESIAN_POINT('Ctrl Pts',(-66.,-2.84046974884046,-16.805274913915));
#58063=CARTESIAN_POINT('Ctrl Pts',(-50.,-2.84046974884046,-16.805274913915));
#58064=CARTESIAN_POINT('Ctrl Pts',(-66.,-2.78281514699786,-16.8972898402251));
#58065=CARTESIAN_POINT('Ctrl Pts',(-50.,-2.78281514699786,-16.8972898402251));
#58066=CARTESIAN_POINT('Ctrl Pts',(-66.,-2.64606187632854,-16.984711103123));
#58067=CARTESIAN_POINT('Ctrl Pts',(-50.,-2.64606187632854,-16.984711103123));
#58068=CARTESIAN_POINT('Ctrl Pts',(-66.,-2.42115552381383,-17.067116581572));
#58069=CARTESIAN_POINT('Ctrl Pts',(-50.,-2.42115552381383,-17.067116581572));
#58070=CARTESIAN_POINT('Ctrl Pts',(-66.,-2.10178723142879,-17.1442157809099));
#58071=CARTESIAN_POINT('Ctrl Pts',(-50.,-2.10178723142879,-17.1442157809099));
#58072=CARTESIAN_POINT('Ctrl Pts',(-66.,-1.68384299920352,-17.2158227917694));
#58073=CARTESIAN_POINT('Ctrl Pts',(-50.,-1.68384299920352,-17.2158227917694));
#58074=CARTESIAN_POINT('Ctrl Pts',(-66.,-1.16496231481007,-17.2818346267064));
#58075=CARTESIAN_POINT('Ctrl Pts',(-50.,-1.16496231481007,-17.2818346267064));
#58076=CARTESIAN_POINT('Ctrl Pts',(-66.,-0.544072031722875,-17.3422083975502));
#58077=CARTESIAN_POINT('Ctrl Pts',(-50.,-0.544072031722875,-17.3422083975502));
#58078=CARTESIAN_POINT('Ctrl Pts',(-66.,0.0344247852095814,-17.3859937099332));
#58079=CARTESIAN_POINT('Ctrl Pts',(-50.,0.0344247852095814,-17.3859937099332));
#58080=CARTESIAN_POINT('Ctrl Pts',(-66.,0.51421128702247,-17.4162999165388));
#58081=CARTESIAN_POINT('Ctrl Pts',(-50.,0.51421128702247,-17.4162999165388));
#58082=CARTESIAN_POINT('Ctrl Pts',(-66.,0.854447986509492,-17.4353798723759));
#58083=CARTESIAN_POINT('Ctrl Pts',(-50.,0.854447986509492,-17.4353798723759));
#58084=CARTESIAN_POINT('Ctrl Pts',(-66.,1.02966109641534,-17.4446388047024));
#58085=CARTESIAN_POINT('Ctrl Pts',(-50.,1.02966109641534,-17.4446388047024));
#58086=CARTESIAN_POINT('',(-65.5,-2.7865000310617,-16.643348298251));
#58087=CARTESIAN_POINT('Ctrl Pts',(-66.,-2.39254363182917,-16.1992703530064));
#58088=CARTESIAN_POINT('Ctrl Pts',(-65.8407752276778,-2.50356161005854,
-16.3438256470978));
#58089=CARTESIAN_POINT('Ctrl Pts',(-65.7187076779594,-2.62552396821496,
-16.448224027428));
#58090=CARTESIAN_POINT('Ctrl Pts',(-65.5661348005199,-2.74402943200492,
-16.5833869839835));
#58091=CARTESIAN_POINT('Ctrl Pts',(-65.532379579053,-2.76786749699358,-16.6136375795362));
#58092=CARTESIAN_POINT('Ctrl Pts',(-65.5,-2.7865000310617,-16.643348298251));
#58093=CARTESIAN_POINT('',(-66.,-1.57673047345591,-13.9738265075847));
#58094=CARTESIAN_POINT('',(-50.5,-2.7865000310617,-16.643348298251));
#58095=CARTESIAN_POINT('Ctrl Pts',(-50.5,-2.78650003106167,-16.6433482982509));
#58096=CARTESIAN_POINT('Ctrl Pts',(-50.4645575966417,-2.76610413878685,
-16.6108257966901));
#58097=CARTESIAN_POINT('Ctrl Pts',(-50.4275078925308,-2.7394921488981,-16.5776894595399));
#58098=CARTESIAN_POINT('Ctrl Pts',(-50.3892199354571,-2.70928763483811,
-16.5438395577443));
#58099=CARTESIAN_POINT('Ctrl Pts',(-50.3627387584052,-2.68839722579765,
-16.5204278818245));
#58100=CARTESIAN_POINT('Ctrl Pts',(-50.3356652570434,-2.66578887888934,
-16.4966747434728));
#58101=CARTESIAN_POINT('Ctrl Pts',(-50.3081215291836,-2.64231600067803,
-16.4725441298628));
#58102=CARTESIAN_POINT('Ctrl Pts',(-50.287625293614,-2.62484902439342,-16.454587710038));
#58103=CARTESIAN_POINT('Ctrl Pts',(-50.2671206064011,-2.60711322773141,
-16.4366340223856));
#58104=CARTESIAN_POINT('Ctrl Pts',(-50.2463806710782,-2.58922579273126,
-16.4184483377371));
#58105=CARTESIAN_POINT('Ctrl Pts',(-50.2161613181612,-2.56316270706432,
-16.3919506841102));
#58106=CARTESIAN_POINT('Ctrl Pts',(-50.1854425271455,-2.53676748651398,
-16.3649610373556));
#58107=CARTESIAN_POINT('Ctrl Pts',(-50.153522730352,-2.51032301522503,-16.3367318371129));
#58108=CARTESIAN_POINT('Ctrl Pts',(-50.1248133742721,-2.486538285407,-16.3113418834469));
#58109=CARTESIAN_POINT('Ctrl Pts',(-50.0951324534083,-2.46271628719235,
-16.2849492581259));
#58110=CARTESIAN_POINT('Ctrl Pts',(-50.0639695102777,-2.43910032977209,
-16.2569947639715));
#58111=CARTESIAN_POINT('Ctrl Pts',(-50.0433448280462,-2.42347049611539,
-16.2384935410138));
#58112=CARTESIAN_POINT('Ctrl Pts',(-50.0220709849552,-2.40793241896019,
-16.2193079242621));
#58113=CARTESIAN_POINT('Ctrl Pts',(-50.,-2.39254363182917,-16.1992703530065));
#58114=CARTESIAN_POINT('Ctrl Pts',(-65.5,-2.7865000310617,-16.643348298251));
#58115=CARTESIAN_POINT('Ctrl Pts',(-60.5,-2.7865000310617,-16.643348298251));
#58116=CARTESIAN_POINT('Ctrl Pts',(-55.5,-2.7865000310617,-16.643348298251));
#58117=CARTESIAN_POINT('Ctrl Pts',(-50.5,-2.7865000310617,-16.643348298251));
#58118=CARTESIAN_POINT('Origin',(-66.,0.,0.));
#58119=CARTESIAN_POINT('',(-66.,-0.187087378736044,-14.0612554404903));
#58120=CARTESIAN_POINT('Ctrl Pts',(-66.,1.02966109641534,-17.4446388047024));
#58121=CARTESIAN_POINT('Ctrl Pts',(-50.,1.02966109641534,-17.4446388047024));
#58122=CARTESIAN_POINT('Ctrl Pts',(-66.,1.01634258017856,-17.4264925129894));
#58123=CARTESIAN_POINT('Ctrl Pts',(-50.,1.01634258017856,-17.4264925129894));
#58124=CARTESIAN_POINT('Ctrl Pts',(-66.,0.989847264833719,-17.3901577483675));
#58125=CARTESIAN_POINT('Ctrl Pts',(-50.,0.989847264833719,-17.3901577483675));
#58126=CARTESIAN_POINT('Ctrl Pts',(-66.,0.950529442539783,-17.335529057983));
#58127=CARTESIAN_POINT('Ctrl Pts',(-50.,0.950529442539783,-17.335529057983));
#58128=CARTESIAN_POINT('Ctrl Pts',(-66.,0.898957117453771,-17.262437379481));
#58129=CARTESIAN_POINT('Ctrl Pts',(-50.,0.898957117453771,-17.262437379481));
#58130=CARTESIAN_POINT('Ctrl Pts',(-66.,0.835916672953383,-17.1706489753383));
#58131=CARTESIAN_POINT('Ctrl Pts',(-50.,0.835916672953383,-17.1706489753383));
#58132=CARTESIAN_POINT('Ctrl Pts',(-66.,0.774307559809985,-17.0784358527592));
#58133=CARTESIAN_POINT('Ctrl Pts',(-50.,0.774307559809985,-17.0784358527592));
#58134=CARTESIAN_POINT('Ctrl Pts',(-66.,0.714133645526303,-16.9857988139572));
#58135=CARTESIAN_POINT('Ctrl Pts',(-50.,0.714133645526303,-16.9857988139572));
#58136=CARTESIAN_POINT('Ctrl Pts',(-66.,0.655393794508624,-16.892741498413));
#58137=CARTESIAN_POINT('Ctrl Pts',(-50.,0.655393794508624,-16.892741498413));
#58138=CARTESIAN_POINT('Ctrl Pts',(-66.,0.598077690957197,-16.7992718473149));
#58139=CARTESIAN_POINT('Ctrl Pts',(-50.,0.598077690957197,-16.7992718473149));
#58140=CARTESIAN_POINT('Ctrl Pts',(-66.,0.542175324179779,-16.7054008913016));
#58141=CARTESIAN_POINT('Ctrl Pts',(-50.,0.542175324179779,-16.7054008913016));
#58142=CARTESIAN_POINT('Ctrl Pts',(-66.,0.487687945489481,-16.6111412083239));
#58143=CARTESIAN_POINT('Ctrl Pts',(-50.,0.487687945489481,-16.6111412083239));
#58144=CARTESIAN_POINT('Ctrl Pts',(-66.,0.434639273355722,-16.5165054959593));
#58145=CARTESIAN_POINT('Ctrl Pts',(-50.,0.434639273355722,-16.5165054959593));
#58146=CARTESIAN_POINT('Ctrl Pts',(-66.,0.383084538952625,-16.4215052757778));
#58147=CARTESIAN_POINT('Ctrl Pts',(-50.,0.383084538952625,-16.4215052757778));
#58148=CARTESIAN_POINT('Ctrl Pts',(-66.,0.333125583096024,-16.3261492450896));
#58149=CARTESIAN_POINT('Ctrl Pts',(-50.,0.333125583096024,-16.3261492450896));
#58150=CARTESIAN_POINT('Ctrl Pts',(-66.,0.284888522892723,-16.2304441266305));
#58151=CARTESIAN_POINT('Ctrl Pts',(-50.,0.284888522892723,-16.2304441266305));
#58152=CARTESIAN_POINT('Ctrl Pts',(-66.,0.238492193683111,-16.1343961952447));
#58153=CARTESIAN_POINT('Ctrl Pts',(-50.,0.238492193683111,-16.1343961952447));
#58154=CARTESIAN_POINT('Ctrl Pts',(-66.,0.194016921417006,-16.0380127071578));
#58155=CARTESIAN_POINT('Ctrl Pts',(-50.,0.194016921417006,-16.0380127071578));
#58156=CARTESIAN_POINT('Ctrl Pts',(-66.,0.151478606156202,-15.9413031975852));
#58157=CARTESIAN_POINT('Ctrl Pts',(-50.,0.151478606156202,-15.9413031975852));
#58158=CARTESIAN_POINT('Ctrl Pts',(-66.,0.110785127729046,-15.844281437166));
#58159=CARTESIAN_POINT('Ctrl Pts',(-50.,0.110785127729046,-15.844281437166));
#58160=CARTESIAN_POINT('Ctrl Pts',(-66.,0.0717883068748032,-15.7469638696907));
#58161=CARTESIAN_POINT('Ctrl Pts',(-50.,0.0717883068748032,-15.7469638696907));
#58162=CARTESIAN_POINT('Ctrl Pts',(-66.,0.0343674149818962,-15.6493668946876));
#58163=CARTESIAN_POINT('Ctrl Pts',(-50.,0.0343674149818962,-15.6493668946876));
#58164=CARTESIAN_POINT('Ctrl Pts',(-66.,-0.00149271387238248,-15.5515043804903));
#58165=CARTESIAN_POINT('Ctrl Pts',(-50.,-0.00149271387238248,-15.5515043804903));
#58166=CARTESIAN_POINT('Ctrl Pts',(-66.,-0.0356325161212601,-15.4533855207845));
#58167=CARTESIAN_POINT('Ctrl Pts',(-50.,-0.0356325161212601,-15.4533855207845));
#58168=CARTESIAN_POINT('Ctrl Pts',(-66.,-0.0676147251712506,-15.3550114911653));
#58169=CARTESIAN_POINT('Ctrl Pts',(-50.,-0.0676147251712506,-15.3550114911653));
#58170=CARTESIAN_POINT('Ctrl Pts',(-66.,-0.0968131519417803,-15.2563790638913));
#58171=CARTESIAN_POINT('Ctrl Pts',(-50.,-0.0968131519417803,-15.2563790638913));
#58172=CARTESIAN_POINT('Ctrl Pts',(-66.,-0.122566347687195,-15.1574865557124));
#58173=CARTESIAN_POINT('Ctrl Pts',(-50.,-0.122566347687195,-15.1574865557124));
#58174=CARTESIAN_POINT('Ctrl Pts',(-66.,-0.144315282095873,-15.058339300691));
#58175=CARTESIAN_POINT('Ctrl Pts',(-50.,-0.144315282095873,-15.058339300691));
#58176=CARTESIAN_POINT('Ctrl Pts',(-66.,-0.161736107560775,-14.9589547879103));
#58177=CARTESIAN_POINT('Ctrl Pts',(-50.,-0.161736107560775,-14.9589547879103));
#58178=CARTESIAN_POINT('Ctrl Pts',(-66.,-0.174908450355344,-14.8593695705273));
#58179=CARTESIAN_POINT('Ctrl Pts',(-50.,-0.174908450355344,-14.8593695705273));
#58180=CARTESIAN_POINT('Ctrl Pts',(-66.,-0.184238029232279,-14.7596343149665));
#58181=CARTESIAN_POINT('Ctrl Pts',(-50.,-0.184238029232279,-14.7596343149665));
#58182=CARTESIAN_POINT('Ctrl Pts',(-66.,-0.190316238669402,-14.6598058338069));
#58183=CARTESIAN_POINT('Ctrl Pts',(-50.,-0.190316238669402,-14.6598058338069));
#58184=CARTESIAN_POINT('Ctrl Pts',(-66.,-0.19380080315749,-14.5599400753078));
#58185=CARTESIAN_POINT('Ctrl Pts',(-50.,-0.19380080315749,-14.5599400753078));
#58186=CARTESIAN_POINT('Ctrl Pts',(-66.,-0.195293060397626,-14.4600850256186));
#58187=CARTESIAN_POINT('Ctrl Pts',(-50.,-0.195293060397626,-14.4600850256186));
#58188=CARTESIAN_POINT('Ctrl Pts',(-66.,-0.195204987344071,-14.3602728402636));
#58189=CARTESIAN_POINT('Ctrl Pts',(-50.,-0.195204987344071,-14.3602728402636));
#58190=CARTESIAN_POINT('Ctrl Pts',(-66.,-0.193784513213942,-14.2605223532243));
#58191=CARTESIAN_POINT('Ctrl Pts',(-50.,-0.193784513213942,-14.2605223532243));
#58192=CARTESIAN_POINT('Ctrl Pts',(-66.,-0.191684797850075,-14.1807787089954));
#58193=CARTESIAN_POINT('Ctrl Pts',(-50.,-0.191684797850075,-14.1807787089954));
#58194=CARTESIAN_POINT('Ctrl Pts',(-66.,-0.189588581014708,-14.1210041786448));
#58195=CARTESIAN_POINT('Ctrl Pts',(-50.,-0.189588581014708,-14.1210041786448));
#58196=CARTESIAN_POINT('Ctrl Pts',(-66.,-0.187959683517641,-14.0811692301831));
#58197=CARTESIAN_POINT('Ctrl Pts',(-50.,-0.187959683517641,-14.0811692301831));
#58198=CARTESIAN_POINT('Ctrl Pts',(-66.,-0.187087378736032,-14.0612554404903));
#58199=CARTESIAN_POINT('Ctrl Pts',(-50.,-0.187087378736032,-14.0612554404903));
#58200=CARTESIAN_POINT('Origin',(-65.75,0.,0.));
#58201=CARTESIAN_POINT('',(-65.5,-3.57630363704438,-16.4916850956979));
#58202=CARTESIAN_POINT('Origin',(-65.5,0.,0.));
#58203=CARTESIAN_POINT('Ctrl Pts',(-65.5,-3.57630363704438,-16.4916850956979));
#58204=CARTESIAN_POINT('Ctrl Pts',(-65.6677203872149,-3.63345385098673,
-16.3076730899736));
#58205=CARTESIAN_POINT('Ctrl Pts',(-65.8346640232699,-3.68344582376579,
-16.1251870335913));
#58206=CARTESIAN_POINT('Ctrl Pts',(-66.,-3.72562931058621,-15.9455420491152));
#58207=CARTESIAN_POINT('Origin',(-58.,0.,0.));
#58208=CARTESIAN_POINT('',(-50.5,-3.57630363704438,-16.4916850956979));
#58209=CARTESIAN_POINT('Origin',(-50.5,0.,0.));
#58210=CARTESIAN_POINT('Ctrl Pts',(-50.5,-3.57630363704438,-16.4916850956979));
#58211=CARTESIAN_POINT('Ctrl Pts',(-55.5,-3.57630363704438,-16.4916850956979));
#58212=CARTESIAN_POINT('Ctrl Pts',(-60.5,-3.57630363704438,-16.4916850956979));
#58213=CARTESIAN_POINT('Ctrl Pts',(-65.5,-3.57630363704438,-16.4916850956979));
#58214=CARTESIAN_POINT('Origin',(-50.25,0.,0.));
#58215=CARTESIAN_POINT('Ctrl Pts',(-50.,-3.7256293105862,-15.9455420491152));
#58216=CARTESIAN_POINT('Ctrl Pts',(-50.1653359767302,-3.68344582376579,
-16.1251870335914));
#58217=CARTESIAN_POINT('Ctrl Pts',(-50.3322796127843,-3.633453850987,-16.3076730899727));
#58218=CARTESIAN_POINT('Ctrl Pts',(-50.5,-3.57630363704438,-16.4916850956979));
#58219=CARTESIAN_POINT('Ctrl Pts',(-66.,-5.00234392366024,-13.1426961282463));
#58220=CARTESIAN_POINT('Ctrl Pts',(-50.,-5.00234392366024,-13.1426961282463));
#58221=CARTESIAN_POINT('Ctrl Pts',(-66.,-5.00975329143057,-13.1648626726972));
#58222=CARTESIAN_POINT('Ctrl Pts',(-50.,-5.00975329143057,-13.1648626726972));
#58223=CARTESIAN_POINT('Ctrl Pts',(-66.,-5.02478822352796,-13.2091330988228));
#58224=CARTESIAN_POINT('Ctrl Pts',(-50.,-5.02478822352796,-13.2091330988228));
#58225=CARTESIAN_POINT('Ctrl Pts',(-66.,-5.04798920255339,-13.2753507597416));
#58226=CARTESIAN_POINT('Ctrl Pts',(-50.,-5.04798920255339,-13.2753507597416));
#58227=CARTESIAN_POINT('Ctrl Pts',(-66.,-5.08022280379478,-13.3632644309532));
#58228=CARTESIAN_POINT('Ctrl Pts',(-50.,-5.08022280379478,-13.3632644309532));
#58229=CARTESIAN_POINT('Ctrl Pts',(-66.,-5.12272617691501,-13.4724958081193));
#58230=CARTESIAN_POINT('Ctrl Pts',(-50.,-5.12272617691501,-13.4724958081193));
#58231=CARTESIAN_POINT('Ctrl Pts',(-66.,-5.16756435218796,-13.5809703610753));
#58232=CARTESIAN_POINT('Ctrl Pts',(-50.,-5.16756435218796,-13.5809703610753));
#58233=CARTESIAN_POINT('Ctrl Pts',(-66.,-5.21496886213029,-13.6885022424853));
#58234=CARTESIAN_POINT('Ctrl Pts',(-50.,-5.21496886213029,-13.6885022424853));
#58235=CARTESIAN_POINT('Ctrl Pts',(-66.,-5.26532059680125,-13.7947771174053));
#58236=CARTESIAN_POINT('Ctrl Pts',(-50.,-5.26532059680125,-13.7947771174053));
#58237=CARTESIAN_POINT('Ctrl Pts',(-66.,-5.31911705202313,-13.8994109809482));
#58238=CARTESIAN_POINT('Ctrl Pts',(-50.,-5.31911705202313,-13.8994109809482));
#58239=CARTESIAN_POINT('Ctrl Pts',(-66.,-5.37693249048282,-14.0020293939727));
#58240=CARTESIAN_POINT('Ctrl Pts',(-50.,-5.37693249048282,-14.0020293939727));
#58241=CARTESIAN_POINT('Ctrl Pts',(-66.,-5.43936923240832,-14.102334498799));
#58242=CARTESIAN_POINT('Ctrl Pts',(-50.,-5.43936923240832,-14.102334498799));
#58243=CARTESIAN_POINT('Ctrl Pts',(-66.,-5.50704098217782,-14.2001904323636));
#58244=CARTESIAN_POINT('Ctrl Pts',(-50.,-5.50704098217782,-14.2001904323636));
#58245=CARTESIAN_POINT('Ctrl Pts',(-66.,-5.58037590052447,-14.2956379130225));
#58246=CARTESIAN_POINT('Ctrl Pts',(-50.,-5.58037590052447,-14.2956379130225));
#58247=CARTESIAN_POINT('Ctrl Pts',(-66.,-5.65928349609497,-14.3888825985252));
#58248=CARTESIAN_POINT('Ctrl Pts',(-50.,-5.65928349609497,-14.3888825985252));
#58249=CARTESIAN_POINT('Ctrl Pts',(-66.,-5.7429409442582,-14.4802820917477));
#58250=CARTESIAN_POINT('Ctrl Pts',(-50.,-5.7429409442582,-14.4802820917477));
#58251=CARTESIAN_POINT('Ctrl Pts',(-66.,-5.8293396720056,-14.5703597544468));
#58252=CARTESIAN_POINT('Ctrl Pts',(-50.,-5.8293396720056,-14.5703597544468));
#58253=CARTESIAN_POINT('Ctrl Pts',(-66.,-5.91563026424745,-14.6597125620614));
#58254=CARTESIAN_POINT('Ctrl Pts',(-50.,-5.91563026424745,-14.6597125620614));
#58255=CARTESIAN_POINT('Ctrl Pts',(-66.,-5.99951493159239,-14.7487702776409));
#58256=CARTESIAN_POINT('Ctrl Pts',(-50.,-5.99951493159239,-14.7487702776409));
#58257=CARTESIAN_POINT('Ctrl Pts',(-66.,-6.08025962758854,-14.8376145740015));
#58258=CARTESIAN_POINT('Ctrl Pts',(-50.,-6.08025962758854,-14.8376145740015));
#58259=CARTESIAN_POINT('Ctrl Pts',(-66.,-6.16012083060275,-14.925722782193));
#58260=CARTESIAN_POINT('Ctrl Pts',(-50.,-6.16012083060275,-14.925722782193));
#58261=CARTESIAN_POINT('Ctrl Pts',(-66.,-6.2448525974522,-15.0118888540403));
#58262=CARTESIAN_POINT('Ctrl Pts',(-50.,-6.2448525974522,-15.0118888540403));
#58263=CARTESIAN_POINT('Ctrl Pts',(-66.,-6.34052323744621,-15.094865717647));
#58264=CARTESIAN_POINT('Ctrl Pts',(-50.,-6.34052323744621,-15.094865717647));
#58265=CARTESIAN_POINT('Ctrl Pts',(-66.,-6.45079341600148,-15.1739178576564));
#58266=CARTESIAN_POINT('Ctrl Pts',(-50.,-6.45079341600148,-15.1739178576564));
#58267=CARTESIAN_POINT('Ctrl Pts',(-66.,-6.57413834909723,-15.2493838286629));
#58268=CARTESIAN_POINT('Ctrl Pts',(-50.,-6.57413834909723,-15.2493838286629));
#58269=CARTESIAN_POINT('Ctrl Pts',(-66.,-6.70071239766311,-15.323312619824));
#58270=CARTESIAN_POINT('Ctrl Pts',(-50.,-6.70071239766311,-15.323312619824));
#58271=CARTESIAN_POINT('Ctrl Pts',(-66.,-6.81475454587001,-15.3989682845842));
#58272=CARTESIAN_POINT('Ctrl Pts',(-50.,-6.81475454587001,-15.3989682845842));
#58273=CARTESIAN_POINT('Ctrl Pts',(-66.,-6.89764997584352,-15.4802006851134));
#58274=CARTESIAN_POINT('Ctrl Pts',(-50.,-6.89764997584352,-15.4802006851134));
#58275=CARTESIAN_POINT('Ctrl Pts',(-66.,-6.93053309053802,-15.5709101984212));
#58276=CARTESIAN_POINT('Ctrl Pts',(-50.,-6.93053309053802,-15.5709101984212));
#58277=CARTESIAN_POINT('Ctrl Pts',(-66.,-6.89757299567323,-15.6743724230443));
#58278=CARTESIAN_POINT('Ctrl Pts',(-50.,-6.89757299567323,-15.6743724230443));
#58279=CARTESIAN_POINT('Ctrl Pts',(-66.,-6.78685686447956,-15.7930563416641));
#58280=CARTESIAN_POINT('Ctrl Pts',(-50.,-6.78685686447956,-15.7930563416641));
#58281=CARTESIAN_POINT('Ctrl Pts',(-66.,-6.58950976774019,-15.928804835904));
#58282=CARTESIAN_POINT('Ctrl Pts',(-50.,-6.58950976774019,-15.928804835904));
#58283=CARTESIAN_POINT('Ctrl Pts',(-66.,-6.29934880872149,-16.0829054867165));
#58284=CARTESIAN_POINT('Ctrl Pts',(-50.,-6.29934880872149,-16.0829054867165));
#58285=CARTESIAN_POINT('Ctrl Pts',(-66.,-5.91234300254812,-16.2562013356071));
#58286=CARTESIAN_POINT('Ctrl Pts',(-50.,-5.91234300254812,-16.2562013356071));
#58287=CARTESIAN_POINT('Ctrl Pts',(-66.,-5.42618038479175,-16.4491796662161));
#58288=CARTESIAN_POINT('Ctrl Pts',(-50.,-5.42618038479175,-16.4491796662161));
#58289=CARTESIAN_POINT('Ctrl Pts',(-66.,-4.83981085794396,-16.6620658184719));
#58290=CARTESIAN_POINT('Ctrl Pts',(-50.,-4.83981085794396,-16.6620658184719));
#58291=CARTESIAN_POINT('Ctrl Pts',(-66.,-4.29037754669269,-16.8483418428791));
#58292=CARTESIAN_POINT('Ctrl Pts',(-50.,-4.29037754669269,-16.8483418428791));
#58293=CARTESIAN_POINT('Ctrl Pts',(-66.,-3.83320126720106,-16.997013975274));
#58294=CARTESIAN_POINT('Ctrl Pts',(-50.,-3.83320126720106,-16.997013975274));
#58295=CARTESIAN_POINT('Ctrl Pts',(-66.,-3.50839872134417,-17.1001079256176));
#58296=CARTESIAN_POINT('Ctrl Pts',(-50.,-3.50839872134417,-17.1001079256176));
#58297=CARTESIAN_POINT('Ctrl Pts',(-66.,-3.34099285631593,-17.1526497000914));
#58298=CARTESIAN_POINT('Ctrl Pts',(-50.,-3.34099285631593,-17.1526497000914));
#58299=CARTESIAN_POINT('',(-65.5,-6.83798941890817,-15.4274925281751));
#58300=CARTESIAN_POINT('Ctrl Pts',(-66.,-6.34597219029741,-15.0953390806557));
#58301=CARTESIAN_POINT('Ctrl Pts',(-65.793328015403,-6.53220709556297,-15.2412392294586));
#58302=CARTESIAN_POINT('Ctrl Pts',(-65.6370761749492,-6.73030865517213,
-15.3252827538815));
#58303=CARTESIAN_POINT('Ctrl Pts',(-65.5,-6.83798941890817,-15.4274925281751));
#58304=CARTESIAN_POINT('',(-66.,-5.00234392366024,-13.1426961282463));
#58305=CARTESIAN_POINT('',(-50.5,-6.83798941890817,-15.4274925281751));
#58306=CARTESIAN_POINT('Ctrl Pts',(-50.5,-6.83798941890817,-15.4274925281751));
#58307=CARTESIAN_POINT('Ctrl Pts',(-50.4442803165968,-6.79421858808209,
-15.3859455834456));
#58308=CARTESIAN_POINT('Ctrl Pts',(-50.3845456174402,-6.73516562112925,
-15.3467194221617));
#58309=CARTESIAN_POINT('Ctrl Pts',(-50.2235302462153,-6.56816980859925,
-15.2438530879325));
#58310=CARTESIAN_POINT('Ctrl Pts',(-50.1242297628299,-6.45791730059814,
-15.1830391185586));
#58311=CARTESIAN_POINT('Ctrl Pts',(-50.,-6.34597219029741,-15.0953390806557));
#58312=CARTESIAN_POINT('Ctrl Pts',(-65.5,-6.83798941890817,-15.4274925281751));
#58313=CARTESIAN_POINT('Ctrl Pts',(-60.5,-6.83798941890817,-15.4274925281751));
#58314=CARTESIAN_POINT('Ctrl Pts',(-55.5,-6.83798941890817,-15.4274925281751));
#58315=CARTESIAN_POINT('Ctrl Pts',(-50.5,-6.83798941890817,-15.4274925281751));
#58316=CARTESIAN_POINT('Origin',(-66.,0.,0.));
#58317=CARTESIAN_POINT('',(-66.,-3.67810171359515,-13.5729685048794));
#58318=CARTESIAN_POINT('Ctrl Pts',(-66.,-3.34099285631593,-17.1526497000914));
#58319=CARTESIAN_POINT('Ctrl Pts',(-50.,-3.34099285631593,-17.1526497000914));
#58320=CARTESIAN_POINT('Ctrl Pts',(-66.,-3.34938014763553,-17.1317613272011));
#58321=CARTESIAN_POINT('Ctrl Pts',(-50.,-3.34938014763553,-17.1317613272011));
#58322=CARTESIAN_POINT('Ctrl Pts',(-66.,-3.36600697541335,-17.0899789690413));
#58323=CARTESIAN_POINT('Ctrl Pts',(-50.,-3.36600697541335,-17.0899789690413));
#58324=CARTESIAN_POINT('Ctrl Pts',(-66.,-3.39050395317181,-17.0272885946305));
#58325=CARTESIAN_POINT('Ctrl Pts',(-50.,-3.39050395317181,-17.0272885946305));
#58326=CARTESIAN_POINT('Ctrl Pts',(-66.,-3.42227887755104,-16.9436677099084));
#58327=CARTESIAN_POINT('Ctrl Pts',(-50.,-3.42227887755104,-16.9436677099084));
#58328=CARTESIAN_POINT('Ctrl Pts',(-66.,-3.46051194269489,-16.8390854862393));
#58329=CARTESIAN_POINT('Ctrl Pts',(-50.,-3.46051194269489,-16.8390854862393));
#58330=CARTESIAN_POINT('Ctrl Pts',(-66.,-3.49725302120834,-16.7344478450781));
#58331=CARTESIAN_POINT('Ctrl Pts',(-50.,-3.49725302120834,-16.7344478450781));
#58332=CARTESIAN_POINT('Ctrl Pts',(-66.,-3.53249856659576,-16.6297565252442));
#58333=CARTESIAN_POINT('Ctrl Pts',(-50.,-3.53249856659576,-16.6297565252442));
#58334=CARTESIAN_POINT('Ctrl Pts',(-66.,-3.56625058387612,-16.5250147694666));
#58335=CARTESIAN_POINT('Ctrl Pts',(-50.,-3.56625058387612,-16.5250147694666));
#58336=CARTESIAN_POINT('Ctrl Pts',(-66.,-3.59852103965262,-16.4202277040114));
#58337=CARTESIAN_POINT('Ctrl Pts',(-50.,-3.59852103965262,-16.4202277040114));
#58338=CARTESIAN_POINT('Ctrl Pts',(-66.,-3.62932237332147,-16.3154035234118));
#58339=CARTESIAN_POINT('Ctrl Pts',(-50.,-3.62932237332147,-16.3154035234118));
#58340=CARTESIAN_POINT('Ctrl Pts',(-66.,-3.658656500891,-16.2105547216479));
#58341=CARTESIAN_POINT('Ctrl Pts',(-50.,-3.658656500891,-16.2105547216479));
#58342=CARTESIAN_POINT('Ctrl Pts',(-66.,-3.68650360681028,-16.1056994959229));
#58343=CARTESIAN_POINT('Ctrl Pts',(-50.,-3.68650360681028,-16.1056994959229));
#58344=CARTESIAN_POINT('Ctrl Pts',(-66.,-3.712813060392,-16.0008627412701));
#58345=CARTESIAN_POINT('Ctrl Pts',(-50.,-3.712813060392,-16.0008627412701));
#58346=CARTESIAN_POINT('Ctrl Pts',(-66.,-3.73748838326994,-15.8960782085386));
#58347=CARTESIAN_POINT('Ctrl Pts',(-50.,-3.73748838326994,-15.8960782085386));
#58348=CARTESIAN_POINT('Ctrl Pts',(-66.,-3.76040909241452,-15.7913837733062));
#58349=CARTESIAN_POINT('Ctrl Pts',(-50.,-3.76040909241452,-15.7913837733062));
#58350=CARTESIAN_POINT('Ctrl Pts',(-66.,-3.78146164640637,-15.6868150664286));
#58351=CARTESIAN_POINT('Ctrl Pts',(-50.,-3.78146164640637,-15.6868150664286));
#58352=CARTESIAN_POINT('Ctrl Pts',(-66.,-3.80057004743305,-15.5823990924153));
#58353=CARTESIAN_POINT('Ctrl Pts',(-50.,-3.80057004743305,-15.5823990924153));
#58354=CARTESIAN_POINT('Ctrl Pts',(-66.,-3.81772126627406,-15.4781490410999));
#58355=CARTESIAN_POINT('Ctrl Pts',(-50.,-3.81772126627406,-15.4781490410999));
#58356=CARTESIAN_POINT('Ctrl Pts',(-66.,-3.83300795359517,-15.3740553411364));
#58357=CARTESIAN_POINT('Ctrl Pts',(-50.,-3.83300795359517,-15.3740553411364));
#58358=CARTESIAN_POINT('Ctrl Pts',(-66.,-3.84657772273756,-15.2700970690198));
#58359=CARTESIAN_POINT('Ctrl Pts',(-50.,-3.84657772273756,-15.2700970690198));
#58360=CARTESIAN_POINT('Ctrl Pts',(-66.,-3.85855158779829,-15.1662600850723));
#58361=CARTESIAN_POINT('Ctrl Pts',(-50.,-3.85855158779829,-15.1662600850723));
#58362=CARTESIAN_POINT('Ctrl Pts',(-66.,-3.86894768714904,-15.0625540503165));
#58363=CARTESIAN_POINT('Ctrl Pts',(-50.,-3.86894768714904,-15.0625540503165));
#58364=CARTESIAN_POINT('Ctrl Pts',(-66.,-3.87761375658259,-14.9590275514473));
#58365=CARTESIAN_POINT('Ctrl Pts',(-50.,-3.87761375658259,-14.9590275514473));
#58366=CARTESIAN_POINT('Ctrl Pts',(-66.,-3.88412655939816,-14.8557904709058));
#58367=CARTESIAN_POINT('Ctrl Pts',(-50.,-3.88412655939816,-14.8557904709058));
#58368=CARTESIAN_POINT('Ctrl Pts',(-66.,-3.88787877668998,-14.7529954092481));
#58369=CARTESIAN_POINT('Ctrl Pts',(-50.,-3.88787877668998,-14.7529954092481));
#58370=CARTESIAN_POINT('Ctrl Pts',(-66.,-3.88822932173376,-14.6508052317201));
#58371=CARTESIAN_POINT('Ctrl Pts',(-50.,-3.88822932173376,-14.6508052317201));
#58372=CARTESIAN_POINT('Ctrl Pts',(-66.,-3.88463805371054,-14.5493641299902));
#58373=CARTESIAN_POINT('Ctrl Pts',(-50.,-3.88463805371054,-14.5493641299902));
#58374=CARTESIAN_POINT('Ctrl Pts',(-66.,-3.87679564863944,-14.4487695813147));
#58375=CARTESIAN_POINT('Ctrl Pts',(-50.,-3.87679564863944,-14.4487695813147));
#58376=CARTESIAN_POINT('Ctrl Pts',(-66.,-3.86478832158859,-14.3490371882169));
#58377=CARTESIAN_POINT('Ctrl Pts',(-50.,-3.86478832158859,-14.3490371882169));
#58378=CARTESIAN_POINT('Ctrl Pts',(-66.,-3.84902164513744,-14.2501151271916));
#58379=CARTESIAN_POINT('Ctrl Pts',(-50.,-3.84902164513744,-14.2501151271916));
#58380=CARTESIAN_POINT('Ctrl Pts',(-66.,-3.83008256273264,-14.1519113521203));
#58381=CARTESIAN_POINT('Ctrl Pts',(-50.,-3.83008256273264,-14.1519113521203));
#58382=CARTESIAN_POINT('Ctrl Pts',(-66.,-3.8086220490069,-14.0543164841154));
#58383=CARTESIAN_POINT('Ctrl Pts',(-50.,-3.8086220490069,-14.0543164841154));
#58384=CARTESIAN_POINT('Ctrl Pts',(-66.,-3.7852344832017,-13.9572274551481));
#58385=CARTESIAN_POINT('Ctrl Pts',(-50.,-3.7852344832017,-13.9572274551481));
#58386=CARTESIAN_POINT('Ctrl Pts',(-66.,-3.76032689601146,-13.8605729560155));
#58387=CARTESIAN_POINT('Ctrl Pts',(-50.,-3.76032689601146,-13.8605729560155));
#58388=CARTESIAN_POINT('Ctrl Pts',(-66.,-3.73414411132176,-13.764309571506));
#58389=CARTESIAN_POINT('Ctrl Pts',(-50.,-3.73414411132176,-13.764309571506));
#58390=CARTESIAN_POINT('Ctrl Pts',(-66.,-3.71227892449176,-13.6875933984758));
#58391=CARTESIAN_POINT('Ctrl Pts',(-50.,-3.71227892449176,-13.6875933984758));
#58392=CARTESIAN_POINT('Ctrl Pts',(-66.,-3.69538324295473,-13.6302181028421));
#58393=CARTESIAN_POINT('Ctrl Pts',(-50.,-3.69538324295473,-13.6302181028421));
#58394=CARTESIAN_POINT('Ctrl Pts',(-66.,-3.68389897142971,-13.5920397328724));
#58395=CARTESIAN_POINT('Ctrl Pts',(-50.,-3.68389897142971,-13.5920397328724));
#58396=CARTESIAN_POINT('Ctrl Pts',(-66.,-3.67810171359514,-13.5729685048794));
#58397=CARTESIAN_POINT('Ctrl Pts',(-50.,-3.67810171359514,-13.5729685048794));
#58398=CARTESIAN_POINT('Origin',(-65.75,0.,0.));
#58399=CARTESIAN_POINT('',(-65.5,-7.56526278753169,-15.0841779343651));
#58400=CARTESIAN_POINT('Origin',(-65.5,0.,0.));
#58401=CARTESIAN_POINT('Ctrl Pts',(-65.5,-7.56526278753169,-15.0841779343651));
#58402=CARTESIAN_POINT('Ctrl Pts',(-65.6931595476753,-7.57631059668304,
-14.8625452434075));
#58403=CARTESIAN_POINT('Ctrl Pts',(-65.8611256967106,-7.57728353276941,
-14.6730213958903));
#58404=CARTESIAN_POINT('Ctrl Pts',(-66.,-7.57407686781798,-14.5180571909737));
#58405=CARTESIAN_POINT('Origin',(-58.,0.,0.));
#58406=CARTESIAN_POINT('',(-50.5,-7.56526278753169,-15.0841779343651));
#58407=CARTESIAN_POINT('Origin',(-50.5,0.,0.));
#58408=CARTESIAN_POINT('Ctrl Pts',(-50.5,-7.56526278753169,-15.0841779343651));
#58409=CARTESIAN_POINT('Ctrl Pts',(-55.5,-7.56526278753169,-15.0841779343651));
#58410=CARTESIAN_POINT('Ctrl Pts',(-60.5,-7.56526278753169,-15.0841779343651));
#58411=CARTESIAN_POINT('Ctrl Pts',(-65.5,-7.56526278753169,-15.0841779343651));
#58412=CARTESIAN_POINT('Origin',(-50.25,0.,0.));
#58413=CARTESIAN_POINT('Ctrl Pts',(-50.,-7.57407686781798,-14.5180571909737));
#58414=CARTESIAN_POINT('Ctrl Pts',(-50.1388743032875,-7.57728353276935,
-14.6730213958882));
#58415=CARTESIAN_POINT('Ctrl Pts',(-50.3068404523229,-7.57631059668312,
-14.8625452434055));
#58416=CARTESIAN_POINT('Ctrl Pts',(-50.5,-7.56526278753169,-15.0841779343651));
#58417=CARTESIAN_POINT('Ctrl Pts',(-66.,-8.11364170780698,-11.4857618157149));
#58418=CARTESIAN_POINT('Ctrl Pts',(-50.,-8.11364170780698,-11.4857618157149));
#58419=CARTESIAN_POINT('Ctrl Pts',(-66.,-8.12633089210227,-11.5053893225758));
#58420=CARTESIAN_POINT('Ctrl Pts',(-50.,-8.12633089210227,-11.5053893225758));
#58421=CARTESIAN_POINT('Ctrl Pts',(-66.,-8.15190308143842,-11.5445298762901));
#58422=CARTESIAN_POINT('Ctrl Pts',(-50.,-8.15190308143842,-11.5445298762901));
#58423=CARTESIAN_POINT('Ctrl Pts',(-66.,-8.19084282166638,-11.6028973387695));
#58424=CARTESIAN_POINT('Ctrl Pts',(-50.,-8.19084282166638,-11.6028973387695));
#58425=CARTESIAN_POINT('Ctrl Pts',(-66.,-8.24392698602517,-11.6800328696824));
#58426=CARTESIAN_POINT('Ctrl Pts',(-50.,-8.24392698602517,-11.6800328696824));
#58427=CARTESIAN_POINT('Ctrl Pts',(-66.,-8.3122597763829,-11.775262383207));
#58428=CARTESIAN_POINT('Ctrl Pts',(-50.,-8.3122597763829,-11.775262383207));
#58429=CARTESIAN_POINT('Ctrl Pts',(-66.,-8.3826658022629,-11.8691782078618));
#58430=CARTESIAN_POINT('Ctrl Pts',(-50.,-8.3826658022629,-11.8691782078618));
#58431=CARTESIAN_POINT('Ctrl Pts',(-66.,-8.45532310380908,-11.9615427552514));
#58432=CARTESIAN_POINT('Ctrl Pts',(-50.,-8.45532310380908,-11.9615427552514));
#58433=CARTESIAN_POINT('Ctrl Pts',(-66.,-8.53052243279731,-12.0519568423361));
#58434=CARTESIAN_POINT('Ctrl Pts',(-50.,-8.53052243279731,-12.0519568423361));
#58435=CARTESIAN_POINT('Ctrl Pts',(-66.,-8.60865015717173,-12.1399248062686));
#58436=CARTESIAN_POINT('Ctrl Pts',(-50.,-8.60865015717173,-12.1399248062686));
#58437=CARTESIAN_POINT('Ctrl Pts',(-66.,-8.69016937887314,-12.2249411582788));
#58438=CARTESIAN_POINT('Ctrl Pts',(-50.,-8.69016937887314,-12.2249411582788));
#58439=CARTESIAN_POINT('Ctrl Pts',(-66.,-8.77558942093922,-12.3065676074844));
#58440=CARTESIAN_POINT('Ctrl Pts',(-50.,-8.77558942093922,-12.3065676074844));
#58441=CARTESIAN_POINT('Ctrl Pts',(-66.,-8.86547091932666,-12.3845199371372));
#58442=CARTESIAN_POINT('Ctrl Pts',(-50.,-8.86547091932666,-12.3845199371372));
#58443=CARTESIAN_POINT('Ctrl Pts',(-66.,-8.96023870955522,-12.4587311071067));
#58444=CARTESIAN_POINT('Ctrl Pts',(-50.,-8.96023870955522,-12.4587311071067));
#58445=CARTESIAN_POINT('Ctrl Pts',(-66.,-9.05985628822634,-12.5294228183105));
#58446=CARTESIAN_POINT('Ctrl Pts',(-50.,-9.05985628822634,-12.5294228183105));
#58447=CARTESIAN_POINT('Ctrl Pts',(-66.,-9.16361561347667,-12.5971460670373));
#58448=CARTESIAN_POINT('Ctrl Pts',(-50.,-9.16361561347667,-12.5971460670373));
#58449=CARTESIAN_POINT('Ctrl Pts',(-66.,-9.26970137008846,-12.6629072844668));
#58450=CARTESIAN_POINT('Ctrl Pts',(-50.,-9.26970137008846,-12.6629072844668));
#58451=CARTESIAN_POINT('Ctrl Pts',(-66.,-9.37550212434126,-12.7279933116739));
#58452=CARTESIAN_POINT('Ctrl Pts',(-50.,-9.37550212434126,-12.7279933116739));
#58453=CARTESIAN_POINT('Ctrl Pts',(-66.,-9.47889915384706,-12.7933918468958));
#58454=CARTESIAN_POINT('Ctrl Pts',(-50.,-9.47889915384706,-12.7933918468958));
#58455=CARTESIAN_POINT('Ctrl Pts',(-66.,-9.57920178477654,-12.8593645469766));
#58456=CARTESIAN_POINT('Ctrl Pts',(-50.,-9.57920178477654,-12.8593645469766));
#58457=CARTESIAN_POINT('Ctrl Pts',(-66.,-9.67846562159703,-12.9248440002217));
#58458=CARTESIAN_POINT('Ctrl Pts',(-50.,-9.67846562159703,-12.9248440002217));
#58459=CARTESIAN_POINT('Ctrl Pts',(-66.,-9.78196401486522,-12.9872310729365));
#58460=CARTESIAN_POINT('Ctrl Pts',(-50.,-9.78196401486522,-12.9872310729365));
#58461=CARTESIAN_POINT('Ctrl Pts',(-66.,-9.89526449262547,-13.0438087451241));
#58462=CARTESIAN_POINT('Ctrl Pts',(-50.,-9.89526449262547,-13.0438087451241));
#58463=CARTESIAN_POINT('Ctrl Pts',(-66.,-10.0217297985278,-13.0929542385258));
#58464=CARTESIAN_POINT('Ctrl Pts',(-50.,-10.0217297985278,-13.0929542385258));
#58465=CARTESIAN_POINT('Ctrl Pts',(-66.,-10.1599672475493,-13.135374669787));
#58466=CARTESIAN_POINT('Ctrl Pts',(-50.,-10.1599672475493,-13.135374669787));
#58467=CARTESIAN_POINT('Ctrl Pts',(-66.,-10.3009500823582,-13.1755031661724));
#58468=CARTESIAN_POINT('Ctrl Pts',(-50.,-10.3009500823582,-13.1755031661724));
#58469=CARTESIAN_POINT('Ctrl Pts',(-66.,-10.4302241855029,-13.2204208401335));
#58470=CARTESIAN_POINT('Ctrl Pts',(-50.,-10.4302241855029,-13.2204208401335));
#58471=CARTESIAN_POINT('Ctrl Pts',(-66.,-10.5307169796315,-13.2784859202976));
#58472=CARTESIAN_POINT('Ctrl Pts',(-50.,-10.5307169796315,-13.2784859202976));
#58473=CARTESIAN_POINT('Ctrl Pts',(-66.,-10.5851255494393,-13.3581679293586));
#58474=CARTESIAN_POINT('Ctrl Pts',(-50.,-10.5851255494393,-13.3581679293586));
#58475=CARTESIAN_POINT('Ctrl Pts',(-66.,-10.5789309655315,-13.4665765402144));
#58476=CARTESIAN_POINT('Ctrl Pts',(-50.,-10.5789309655315,-13.4665765402144));
#58477=CARTESIAN_POINT('Ctrl Pts',(-66.,-10.5012086755218,-13.6090657674601));
#58478=CARTESIAN_POINT('Ctrl Pts',(-50.,-10.5012086755218,-13.6090657674601));
#58479=CARTESIAN_POINT('Ctrl Pts',(-66.,-10.3438208784378,-13.7896277003499));
#58480=CARTESIAN_POINT('Ctrl Pts',(-50.,-10.3438208784378,-13.7896277003499));
#58481=CARTESIAN_POINT('Ctrl Pts',(-66.,-10.1010991329779,-14.0110470920039));
#58482=CARTESIAN_POINT('Ctrl Pts',(-50.,-10.1010991329779,-14.0110470920039));
#58483=CARTESIAN_POINT('Ctrl Pts',(-66.,-9.76934875096609,-14.2751429634022));
#58484=CARTESIAN_POINT('Ctrl Pts',(-50.,-9.76934875096609,-14.2751429634022));
#58485=CARTESIAN_POINT('Ctrl Pts',(-66.,-9.34645158510148,-14.5829622514464));
#58486=CARTESIAN_POINT('Ctrl Pts',(-50.,-9.34645158510148,-14.5829622514464));
#58487=CARTESIAN_POINT('Ctrl Pts',(-66.,-8.83144656838121,-14.9349843652275));
#58488=CARTESIAN_POINT('Ctrl Pts',(-50.,-8.83144656838121,-14.9349843652275));
#58489=CARTESIAN_POINT('Ctrl Pts',(-66.,-8.34559967843141,-15.25204669397));
#58490=CARTESIAN_POINT('Ctrl Pts',(-50.,-8.34559967843141,-15.25204669397));
#58491=CARTESIAN_POINT('Ctrl Pts',(-66.,-7.93975968827824,-15.509743135298));
#58492=CARTESIAN_POINT('Ctrl Pts',(-50.,-7.93975968827824,-15.509743135298));
#58493=CARTESIAN_POINT('Ctrl Pts',(-66.,-7.65079983454787,-15.6903733080951));
#58494=CARTESIAN_POINT('Ctrl Pts',(-50.,-7.65079983454787,-15.6903733080951));
#58495=CARTESIAN_POINT('Ctrl Pts',(-66.,-7.50171994057268,-15.7828965317908));
#58496=CARTESIAN_POINT('Ctrl Pts',(-50.,-7.50171994057268,-15.7828965317908));
#58497=CARTESIAN_POINT('',(-65.5,-10.4598227831987,-13.2422706642055));
#58498=CARTESIAN_POINT('Ctrl Pts',(-66.,-9.90065997719615,-13.0429121370937));
#58499=CARTESIAN_POINT('Ctrl Pts',(-65.7933280154041,-10.1173278619927,
-13.1379138268532));
#58500=CARTESIAN_POINT('Ctrl Pts',(-65.6370761749487,-10.3301064714307,
-13.1700511149055));
#58501=CARTESIAN_POINT('Ctrl Pts',(-65.5,-10.4598227831987,-13.2422706642055));
#58502=CARTESIAN_POINT('',(-66.,-8.11364170780698,-11.4857618157149));
#58503=CARTESIAN_POINT('',(-50.5,-10.4598227831987,-13.2422706642055));
#58504=CARTESIAN_POINT('Ctrl Pts',(-50.5,-10.4598227831987,-13.2422706642055));
#58505=CARTESIAN_POINT('Ctrl Pts',(-50.4518618349117,-10.4142692416525,
-13.2169087325051));
#58506=CARTESIAN_POINT('Ctrl Pts',(-50.4012423593874,-10.3586165910348,
-13.1963094071548));
#58507=CARTESIAN_POINT('Ctrl Pts',(-50.2441129793791,-10.1781263556467,
-13.1379513556689));
#58508=CARTESIAN_POINT('Ctrl Pts',(-50.1366827452935,-10.0439535221284,
-13.105741609551));
#58509=CARTESIAN_POINT('Ctrl Pts',(-50.,-9.90065997719615,-13.0429121370937));
#58510=CARTESIAN_POINT('Ctrl Pts',(-65.5,-10.4598227831987,-13.2422706642055));
#58511=CARTESIAN_POINT('Ctrl Pts',(-60.5,-10.4598227831987,-13.2422706642055));
#58512=CARTESIAN_POINT('Ctrl Pts',(-55.5,-10.4598227831987,-13.2422706642055));
#58513=CARTESIAN_POINT('Ctrl Pts',(-50.5,-10.4598227831987,-13.2422706642055));
#58514=CARTESIAN_POINT('Origin',(-66.,0.,0.));
#58515=CARTESIAN_POINT('',(-66.,-6.93800739067722,-12.2318420402206));
#58516=CARTESIAN_POINT('Ctrl Pts',(-66.,-7.50171994057268,-15.7828965317908));
#58517=CARTESIAN_POINT('Ctrl Pts',(-50.,-7.50171994057268,-15.7828965317908));
#58518=CARTESIAN_POINT('Ctrl Pts',(-66.,-7.50464900261518,-15.760578571014));
#58519=CARTESIAN_POINT('Ctrl Pts',(-50.,-7.50464900261518,-15.760578571014));
#58520=CARTESIAN_POINT('Ctrl Pts',(-66.,-7.5103626180875,-15.7159739585441));
#58521=CARTESIAN_POINT('Ctrl Pts',(-50.,-7.5103626180875,-15.7159739585441));
#58522=CARTESIAN_POINT('Ctrl Pts',(-66.,-7.51849951610435,-15.6491609668904));
#58523=CARTESIAN_POINT('Ctrl Pts',(-50.,-7.51849951610435,-15.6491609668904));
#58524=CARTESIAN_POINT('Ctrl Pts',(-66.,-7.52848050441805,-15.5602650836714));
#58525=CARTESIAN_POINT('Ctrl Pts',(-50.,-7.52848050441805,-15.5602650836714));
#58526=CARTESIAN_POINT('Ctrl Pts',(-66.,-7.53950386611099,-15.4494603262155));
#58527=CARTESIAN_POINT('Ctrl Pts',(-50.,-7.53950386611099,-15.4494603262155));
#58528=CARTESIAN_POINT('Ctrl Pts',(-66.,-7.54906833290726,-15.3389729342967));
#58529=CARTESIAN_POINT('Ctrl Pts',(-50.,-7.54906833290726,-15.3389729342967));
#58530=CARTESIAN_POINT('Ctrl Pts',(-66.,-7.55717090215767,-15.2288054740838));
#58531=CARTESIAN_POINT('Ctrl Pts',(-50.,-7.55717090215767,-15.2288054740838));
#58532=CARTESIAN_POINT('Ctrl Pts',(-66.,-7.56381432232377,-15.1189605878015));
#58533=CARTESIAN_POINT('Ctrl Pts',(-50.,-7.56381432232377,-15.1189605878015));
#58534=CARTESIAN_POINT('Ctrl Pts',(-66.,-7.56901145890645,-15.0094402646918));
#58535=CARTESIAN_POINT('Ctrl Pts',(-50.,-7.56901145890645,-15.0094402646918));
#58536=CARTESIAN_POINT('Ctrl Pts',(-66.,-7.57277639839295,-14.9002493482892));
#58537=CARTESIAN_POINT('Ctrl Pts',(-50.,-7.57277639839295,-14.9002493482892));
#58538=CARTESIAN_POINT('Ctrl Pts',(-66.,-7.57511410372315,-14.7913994635608));
#58539=CARTESIAN_POINT('Ctrl Pts',(-50.,-7.57511410372315,-14.7913994635608));
#58540=CARTESIAN_POINT('Ctrl Pts',(-66.,-7.57600990734854,-14.6829131639384));
#58541=CARTESIAN_POINT('Ctrl Pts',(-50.,-7.57600990734854,-14.6829131639384));
#58542=CARTESIAN_POINT('Ctrl Pts',(-66.,-7.57542096038094,-14.5748271536716));
#58543=CARTESIAN_POINT('Ctrl Pts',(-50.,-7.57542096038094,-14.5748271536716));
#58544=CARTESIAN_POINT('Ctrl Pts',(-66.,-7.57326220899431,-14.4671981164589));
#58545=CARTESIAN_POINT('Ctrl Pts',(-50.,-7.57326220899431,-14.4671981164589));
#58546=CARTESIAN_POINT('Ctrl Pts',(-66.,-7.56942637462814,-14.360092700858));
#58547=CARTESIAN_POINT('Ctrl Pts',(-50.,-7.56942637462814,-14.360092700858));
#58548=CARTESIAN_POINT('Ctrl Pts',(-66.,-7.56381234400904,-14.2535736549186));
#58549=CARTESIAN_POINT('Ctrl Pts',(-50.,-7.56381234400904,-14.2535736549186));
#58550=CARTESIAN_POINT('Ctrl Pts',(-66.,-7.556353222684,-14.1476860346413));
#58551=CARTESIAN_POINT('Ctrl Pts',(-50.,-7.556353222684,-14.1476860346413));
#58552=CARTESIAN_POINT('Ctrl Pts',(-66.,-7.54703967094767,-14.0424458557121));
#58553=CARTESIAN_POINT('Ctrl Pts',(-50.,-7.54703967094767,-14.0424458557121));
#58554=CARTESIAN_POINT('Ctrl Pts',(-66.,-7.53595904837785,-13.9378208062029));
#58555=CARTESIAN_POINT('Ctrl Pts',(-50.,-7.53595904837785,-13.9378208062029));
#58556=CARTESIAN_POINT('Ctrl Pts',(-66.,-7.52324912730704,-13.8337539100138));
#58557=CARTESIAN_POINT('Ctrl Pts',(-50.,-7.52324912730704,-13.8337539100138));
#58558=CARTESIAN_POINT('Ctrl Pts',(-66.,-7.50902360355704,-13.730201376709));
#58559=CARTESIAN_POINT('Ctrl Pts',(-50.,-7.50902360355704,-13.730201376709));
#58560=CARTESIAN_POINT('Ctrl Pts',(-66.,-7.49330244824787,-13.6271680529626));
#58561=CARTESIAN_POINT('Ctrl Pts',(-50.,-7.49330244824787,-13.6271680529626));
#58562=CARTESIAN_POINT('Ctrl Pts',(-66.,-7.47595026385202,-13.5247388655977));
#58563=CARTESIAN_POINT('Ctrl Pts',(-50.,-7.47595026385202,-13.5247388655977));
#58564=CARTESIAN_POINT('Ctrl Pts',(-66.,-7.45658443707985,-13.4231254995838));
#58565=CARTESIAN_POINT('Ctrl Pts',(-50.,-7.45658443707985,-13.4231254995838));
#58566=CARTESIAN_POINT('Ctrl Pts',(-66.,-7.43465467928082,-13.32262679532));
#58567=CARTESIAN_POINT('Ctrl Pts',(-50.,-7.43465467928082,-13.32262679532));
#58568=CARTESIAN_POINT('Ctrl Pts',(-66.,-7.40958054758866,-13.2235599331263));
#58569=CARTESIAN_POINT('Ctrl Pts',(-50.,-7.40958054758866,-13.2235599331263));
#58570=CARTESIAN_POINT('Ctrl Pts',(-66.,-7.38087472971119,-13.1261989021839));
#58571=CARTESIAN_POINT('Ctrl Pts',(-50.,-7.38087472971119,-13.1261989021839));
#58572=CARTESIAN_POINT('Ctrl Pts',(-66.,-7.34826186125705,-13.0307150430677));
#58573=CARTESIAN_POINT('Ctrl Pts',(-50.,-7.34826186125705,-13.0307150430677));
#58574=CARTESIAN_POINT('Ctrl Pts',(-66.,-7.31182932887926,-12.9371020273035));
#58575=CARTESIAN_POINT('Ctrl Pts',(-50.,-7.31182932887926,-12.9371020273035));
#58576=CARTESIAN_POINT('Ctrl Pts',(-66.,-7.27195707536722,-12.8452087977179));
#58577=CARTESIAN_POINT('Ctrl Pts',(-50.,-7.27195707536722,-12.8452087977179));
#58578=CARTESIAN_POINT('Ctrl Pts',(-66.,-7.22919071332107,-12.7548002330908));
#58579=CARTESIAN_POINT('Ctrl Pts',(-50.,-7.22919071332107,-12.7548002330908));
#58580=CARTESIAN_POINT('Ctrl Pts',(-66.,-7.18413356438513,-12.6656085000656));
#58581=CARTESIAN_POINT('Ctrl Pts',(-50.,-7.18413356438513,-12.6656085000656));
#58582=CARTESIAN_POINT('Ctrl Pts',(-66.,-7.13733570230759,-12.5773859525787));
#58583=CARTESIAN_POINT('Ctrl Pts',(-50.,-7.13733570230759,-12.5773859525787));
#58584=CARTESIAN_POINT('Ctrl Pts',(-66.,-7.08917363628753,-12.4899622973194));
#58585=CARTESIAN_POINT('Ctrl Pts',(-50.,-7.08917363628753,-12.4899622973194));
#58586=CARTESIAN_POINT('Ctrl Pts',(-66.,-7.03987370169386,-12.4032345978205));
#58587=CARTESIAN_POINT('Ctrl Pts',(-50.,-7.03987370169386,-12.4032345978205));
#58588=CARTESIAN_POINT('Ctrl Pts',(-66.,-6.99961691350077,-12.3343662552827));
#58589=CARTESIAN_POINT('Ctrl Pts',(-50.,-6.99961691350077,-12.3343662552827));
#58590=CARTESIAN_POINT('Ctrl Pts',(-66.,-6.96898338507103,-12.2829952952022));
#58591=CARTESIAN_POINT('Ctrl Pts',(-50.,-6.96898338507103,-12.2829952952022));
#58592=CARTESIAN_POINT('Ctrl Pts',(-66.,-6.94836533853418,-12.24887239112));
#58593=CARTESIAN_POINT('Ctrl Pts',(-50.,-6.94836533853418,-12.24887239112));
#58594=CARTESIAN_POINT('Ctrl Pts',(-66.,-6.93800739067721,-12.2318420402206));
#58595=CARTESIAN_POINT('Ctrl Pts',(-50.,-6.93800739067721,-12.2318420402206));
#58596=CARTESIAN_POINT('Origin',(-65.75,0.,0.));
#58597=CARTESIAN_POINT('',(-65.5,-11.0788686539881,-12.7288763976904));
#58598=CARTESIAN_POINT('Origin',(-65.5,0.,0.));
#58599=CARTESIAN_POINT('Ctrl Pts',(-65.5,-11.0788686539881,-12.7288763976904));
#58600=CARTESIAN_POINT('Ctrl Pts',(-65.693159547666,-11.0344515669953,-12.5114592268724));
#58601=CARTESIAN_POINT('Ctrl Pts',(-65.8611256966936,-10.9882612722543,
-12.3276476601772));
#58602=CARTESIAN_POINT('Ctrl Pts',(-66.,-10.9466173199385,-12.178349405844));
#58603=CARTESIAN_POINT('Origin',(-58.,0.,0.));
#58604=CARTESIAN_POINT('',(-50.5,-11.0788686539881,-12.7288763976904));
#58605=CARTESIAN_POINT('Origin',(-50.5,0.,0.));
#58606=CARTESIAN_POINT('Ctrl Pts',(-50.5,-11.0788686539881,-12.7288763976904));
#58607=CARTESIAN_POINT('Ctrl Pts',(-55.5,-11.0788686539881,-12.7288763976904));
#58608=CARTESIAN_POINT('Ctrl Pts',(-60.5,-11.0788686539881,-12.7288763976904));
#58609=CARTESIAN_POINT('Ctrl Pts',(-65.5,-11.0788686539881,-12.7288763976904));
#58610=CARTESIAN_POINT('Origin',(-50.25,0.,0.));
#58611=CARTESIAN_POINT('Ctrl Pts',(-50.,-10.9466173199385,-12.178349405844));
#58612=CARTESIAN_POINT('Ctrl Pts',(-50.1388743032945,-10.9882612722507,
-12.3276476601644));
#58613=CARTESIAN_POINT('Ctrl Pts',(-50.3068404523294,-11.0344515669942,
-12.5114592268673));
#58614=CARTESIAN_POINT('Ctrl Pts',(-50.5,-11.0788686539881,-12.7288763976904));
#58615=CARTESIAN_POINT('Ctrl Pts',(-66.,-10.7151295435653,-9.10713484662511));
#58616=CARTESIAN_POINT('Ctrl Pts',(-50.,-10.7151295435653,-9.10713484662511));
#58617=CARTESIAN_POINT('Ctrl Pts',(-66.,-10.7323012362688,-9.12299004745485));
#58618=CARTESIAN_POINT('Ctrl Pts',(-50.,-10.7323012362688,-9.12299004745485));
#58619=CARTESIAN_POINT('Ctrl Pts',(-66.,-10.7668038881397,-9.15454138381928));
#58620=CARTESIAN_POINT('Ctrl Pts',(-50.,-10.7668038881397,-9.15454138381928));
#58621=CARTESIAN_POINT('Ctrl Pts',(-66.,-10.8190356624814,-9.20139120553108));
#58622=CARTESIAN_POINT('Ctrl Pts',(-50.,-10.8190356624814,-9.20139120553108));
#58623=CARTESIAN_POINT('Ctrl Pts',(-66.,-10.889634916681,-9.26290188705335));
#58624=CARTESIAN_POINT('Ctrl Pts',(-50.,-10.889634916681,-9.26290188705335));
#58625=CARTESIAN_POINT('Ctrl Pts',(-66.,-10.9795035237476,-9.33814591637203));
#58626=CARTESIAN_POINT('Ctrl Pts',(-50.,-10.9795035237476,-9.33814591637203));
#58627=CARTESIAN_POINT('Ctrl Pts',(-66.,-11.0710535306934,-9.4116019360644));
#58628=CARTESIAN_POINT('Ctrl Pts',(-50.,-11.0710535306934,-9.4116019360644));
#58629=CARTESIAN_POINT('Ctrl Pts',(-66.,-11.1643982983724,-9.48299554522798));
#58630=CARTESIAN_POINT('Ctrl Pts',(-50.,-11.1643982983724,-9.48299554522798));
#58631=CARTESIAN_POINT('Ctrl Pts',(-66.,-11.2597201712738,-9.55186779486609));
#58632=CARTESIAN_POINT('Ctrl Pts',(-50.,-11.2597201712738,-9.55186779486609));
#58633=CARTESIAN_POINT('Ctrl Pts',(-66.,-11.3572701125446,-9.61764250849074));
#58634=CARTESIAN_POINT('Ctrl Pts',(-50.,-11.3572701125446,-9.61764250849074));
#58635=CARTESIAN_POINT('Ctrl Pts',(-66.,-11.4573709649815,-9.6797149094218));
#58636=CARTESIAN_POINT('Ctrl Pts',(-50.,-11.4573709649815,-9.6797149094218));
#58637=CARTESIAN_POINT('Ctrl Pts',(-66.,-11.5604070517922,-9.73753381300202));
#58638=CARTESIAN_POINT('Ctrl Pts',(-50.,-11.5604070517922,-9.73753381300202));
#58639=CARTESIAN_POINT('Ctrl Pts',(-66.,-11.6668507136929,-9.79068450718227));
#58640=CARTESIAN_POINT('Ctrl Pts',(-50.,-11.6668507136929,-9.79068450718227));
#58641=CARTESIAN_POINT('Ctrl Pts',(-66.,-11.7770967670118,-9.83899640572359));
#58642=CARTESIAN_POINT('Ctrl Pts',(-50.,-11.7770967670118,-9.83899640572359));
#58643=CARTESIAN_POINT('Ctrl Pts',(-66.,-11.8911649899478,-9.88269332242761));
#58644=CARTESIAN_POINT('Ctrl Pts',(-50.,-11.8911649899478,-9.88269332242761));
#58645=CARTESIAN_POINT('Ctrl Pts',(-66.,-12.0085066122796,-9.9224850258725));
#58646=CARTESIAN_POINT('Ctrl Pts',(-50.,-12.0085066122796,-9.9224850258725));
#58647=CARTESIAN_POINT('Ctrl Pts',(-66.,-12.1276136395118,-9.95979777888845));
#58648=CARTESIAN_POINT('Ctrl Pts',(-50.,-12.1276136395118,-9.95979777888845));
#58649=CARTESIAN_POINT('Ctrl Pts',(-66.,-12.2462767052779,-9.99652743122885));
#58650=CARTESIAN_POINT('Ctrl Pts',(-50.,-12.2462767052779,-9.99652743122885));
#58651=CARTESIAN_POINT('Ctrl Pts',(-66.,-12.362689281313,-10.0341575556064));
#58652=CARTESIAN_POINT('Ctrl Pts',(-50.,-12.362689281313,-10.0341575556064));
#58653=CARTESIAN_POINT('Ctrl Pts',(-66.,-12.4762474639872,-10.0731133520306));
#58654=CARTESIAN_POINT('Ctrl Pts',(-50.,-12.4762474639872,-10.0731133520306));
#58655=CARTESIAN_POINT('Ctrl Pts',(-66.,-12.5886768226797,-10.1118497354652));
#58656=CARTESIAN_POINT('Ctrl Pts',(-50.,-12.5886768226797,-10.1118497354652));
#58657=CARTESIAN_POINT('Ctrl Pts',(-66.,-12.7044386576771,-10.1465377998253));
#58658=CARTESIAN_POINT('Ctrl Pts',(-50.,-12.7044386576771,-10.1465377998253));
#58659=CARTESIAN_POINT('Ctrl Pts',(-66.,-12.8282498874959,-10.1731612973722));
#58660=CARTESIAN_POINT('Ctrl Pts',(-50.,-12.8282498874959,-10.1731612973722));
#58661=CARTESIAN_POINT('Ctrl Pts',(-66.,-12.9629640404687,-10.1893121520713));
#58662=CARTESIAN_POINT('Ctrl Pts',(-50.,-12.9629640404687,-10.1893121520713));
#58663=CARTESIAN_POINT('Ctrl Pts',(-66.,-13.1074080380921,-10.1960216118796));
#58664=CARTESIAN_POINT('Ctrl Pts',(-50.,-13.1074080380921,-10.1960216118796));
#58665=CARTESIAN_POINT('Ctrl Pts',(-66.,-13.2539411891343,-10.1998283924791));
#58666=CARTESIAN_POINT('Ctrl Pts',(-50.,-13.2539411891343,-10.1998283924791));
#58667=CARTESIAN_POINT('Ctrl Pts',(-66.,-13.3903244798794,-10.2111857329905));
#58668=CARTESIAN_POINT('Ctrl Pts',(-50.,-13.3903244798794,-10.2111857329905));
#58669=CARTESIAN_POINT('Ctrl Pts',(-66.,-13.5021003063213,-10.2424350502543));
#58670=CARTESIAN_POINT('Ctrl Pts',(-50.,-13.5021003063213,-10.2424350502543));
#58671=CARTESIAN_POINT('Ctrl Pts',(-66.,-13.5746156407008,-10.3060828413894));
#58672=CARTESIAN_POINT('Ctrl Pts',(-50.,-13.5746156407008,-10.3060828413894));
#58673=CARTESIAN_POINT('Ctrl Pts',(-66.,-13.5955757962388,-10.4126261267587));
#58674=CARTESIAN_POINT('Ctrl Pts',(-50.,-13.5955757962388,-10.4126261267587));
#58675=CARTESIAN_POINT('Ctrl Pts',(-66.,-13.5557309247371,-10.5699675404438));
#58676=CARTESIAN_POINT('Ctrl Pts',(-50.,-13.5557309247371,-10.5699675404438));
#58677=CARTESIAN_POINT('Ctrl Pts',(-66.,-13.448191681431,-10.7839975416797));
#58678=CARTESIAN_POINT('Ctrl Pts',(-50.,-13.448191681431,-10.7839975416797));
#58679=CARTESIAN_POINT('Ctrl Pts',(-66.,-13.2681602494653,-11.0588230794739));
#58680=CARTESIAN_POINT('Ctrl Pts',(-50.,-13.2681602494653,-11.0588230794739));
#58681=CARTESIAN_POINT('Ctrl Pts',(-66.,-13.0125103882094,-11.3971248585033));
#58682=CARTESIAN_POINT('Ctrl Pts',(-50.,-13.0125103882094,-11.3971248585033));
#58683=CARTESIAN_POINT('Ctrl Pts',(-66.,-12.6794508584748,-11.8004436860348));
#58684=CARTESIAN_POINT('Ctrl Pts',(-50.,-12.6794508584748,-11.8004436860348));
#58685=CARTESIAN_POINT('Ctrl Pts',(-66.,-12.2681700111386,-12.2694829172856));
#58686=CARTESIAN_POINT('Ctrl Pts',(-50.,-12.2681700111386,-12.2694829172856));
#58687=CARTESIAN_POINT('Ctrl Pts',(-66.,-11.8764370894057,-12.6974093581748));
#58688=CARTESIAN_POINT('Ctrl Pts',(-50.,-11.8764370894057,-12.6974093581748));
#58689=CARTESIAN_POINT('Ctrl Pts',(-66.,-11.5474338077474,-13.0479380932861));
#58690=CARTESIAN_POINT('Ctrl Pts',(-50.,-11.5474338077474,-13.0479380932861));
#58691=CARTESIAN_POINT('Ctrl Pts',(-66.,-11.3124730564734,-13.2947548304684));
#58692=CARTESIAN_POINT('Ctrl Pts',(-50.,-11.3124730564734,-13.2947548304684));
#58693=CARTESIAN_POINT('Ctrl Pts',(-66.,-11.1910863715672,-13.4214459289647));
#58694=CARTESIAN_POINT('Ctrl Pts',(-50.,-11.1910863715672,-13.4214459289647));
#58695=CARTESIAN_POINT('',(-65.5,-13.4244270134836,-10.224988232739));
#58696=CARTESIAN_POINT('Ctrl Pts',(-66.,-12.8332528856473,-10.1709510554827));
#58697=CARTESIAN_POINT('Ctrl Pts',(-65.7933280154042,-13.0667397099252,
-10.2090849806402));
#58698=CARTESIAN_POINT('Ctrl Pts',(-65.6370761749484,-13.2808257066153,
-10.1872967283199));
#58699=CARTESIAN_POINT('Ctrl Pts',(-65.5,-13.4244270134836,-10.224988232739));
#58700=CARTESIAN_POINT('',(-66.,-10.7151295435653,-9.10713484662511));
#58701=CARTESIAN_POINT('',(-50.5,-13.4244270134836,-10.224988232739));
#58702=CARTESIAN_POINT('Ctrl Pts',(-50.5,-13.4244270134836,-10.224988232739));
#58703=CARTESIAN_POINT('Ctrl Pts',(-50.4518618349118,-13.3739973642794,
-10.2117517978674));
#58704=CARTESIAN_POINT('Ctrl Pts',(-50.4012423593876,-13.3149703001221,
-10.205639889605));
#58705=CARTESIAN_POINT('Ctrl Pts',(-50.2441129793791,-13.1256374401377,
-10.1940013598926));
#58706=CARTESIAN_POINT('Ctrl Pts',(-50.1366827452936,-12.9876696547833,
-10.1961709690068));
#58707=CARTESIAN_POINT('Ctrl Pts',(-50.,-12.8332528856473,-10.1709510554827));
#58708=CARTESIAN_POINT('Ctrl Pts',(-65.5,-13.4244270134836,-10.224988232739));
#58709=CARTESIAN_POINT('Ctrl Pts',(-60.5,-13.4244270134836,-10.224988232739));
#58710=CARTESIAN_POINT('Ctrl Pts',(-55.5,-13.4244270134836,-10.224988232739));
#58711=CARTESIAN_POINT('Ctrl Pts',(-50.5,-13.4244270134836,-10.224988232739));
#58712=CARTESIAN_POINT('Origin',(-66.,0.,0.));
#58713=CARTESIAN_POINT('',(-66.,-9.76197254719673,-10.1221439546065));
#58714=CARTESIAN_POINT('Ctrl Pts',(-66.,-11.1910863715672,-13.4214459289647));
#58715=CARTESIAN_POINT('Ctrl Pts',(-50.,-11.1910863715672,-13.4214459289647));
#58716=CARTESIAN_POINT('Ctrl Pts',(-66.,-11.1883731605921,-13.3991006998567));
#58717=CARTESIAN_POINT('Ctrl Pts',(-50.,-11.1883731605921,-13.3991006998567));
#58718=CARTESIAN_POINT('Ctrl Pts',(-66.,-11.1828145562856,-13.3544765049226));
#58719=CARTESIAN_POINT('Ctrl Pts',(-50.,-11.1828145562856,-13.3544765049226));
#58720=CARTESIAN_POINT('Ctrl Pts',(-66.,-11.1740801033331,-13.2877390020125));
#58721=CARTESIAN_POINT('Ctrl Pts',(-50.,-11.1740801033331,-13.2877390020125));
#58722=CARTESIAN_POINT('Ctrl Pts',(-66.,-11.161640013378,-13.1991537755753));
#58723=CARTESIAN_POINT('Ctrl Pts',(-50.,-11.161640013378,-13.1991537755753));
#58724=CARTESIAN_POINT('Ctrl Pts',(-66.,-11.1447610332637,-13.089088754755));
#58725=CARTESIAN_POINT('Ctrl Pts',(-50.,-11.1447610332637,-13.089088754755));
#58726=CARTESIAN_POINT('Ctrl Pts',(-66.,-11.1265479177184,-12.9796939412571));
#58727=CARTESIAN_POINT('Ctrl Pts',(-50.,-11.1265479177184,-12.9796939412571));
#58728=CARTESIAN_POINT('Ctrl Pts',(-66.,-11.1069983966066,-12.870972567358));
#58729=CARTESIAN_POINT('Ctrl Pts',(-50.,-11.1069983966066,-12.870972567358));
#58730=CARTESIAN_POINT('Ctrl Pts',(-66.,-11.0861157891366,-12.7629265087573));
#58731=CARTESIAN_POINT('Ctrl Pts',(-50.,-11.0861157891366,-12.7629265087573));
#58732=CARTESIAN_POINT('Ctrl Pts',(-66.,-11.0639130513203,-12.6555544926816));
#58733=CARTESIAN_POINT('Ctrl Pts',(-50.,-11.0639130513203,-12.6555544926816));
#58734=CARTESIAN_POINT('Ctrl Pts',(-66.,-11.04040503163,-12.5488577073298));
#58735=CARTESIAN_POINT('Ctrl Pts',(-50.,-11.04040503163,-12.5488577073298));
#58736=CARTESIAN_POINT('Ctrl Pts',(-66.,-11.0155994280975,-12.4428461782163));
#58737=CARTESIAN_POINT('Ctrl Pts',(-50.,-11.0155994280975,-12.4428461782163));
#58738=CARTESIAN_POINT('Ctrl Pts',(-66.,-10.9894876427927,-12.3375453978863));
#58739=CARTESIAN_POINT('Ctrl Pts',(-50.,-10.9894876427927,-12.3375453978863));
#58740=CARTESIAN_POINT('Ctrl Pts',(-66.,-10.9620373009797,-12.2330015735433));
#58741=CARTESIAN_POINT('Ctrl Pts',(-50.,-10.9620373009797,-12.2330015735433));
#58742=CARTESIAN_POINT('Ctrl Pts',(-66.,-10.9331801176175,-12.1292907600893));
#58743=CARTESIAN_POINT('Ctrl Pts',(-50.,-10.9331801176175,-12.1292907600893));
#58744=CARTESIAN_POINT('Ctrl Pts',(-66.,-10.902828759321,-12.0265041912883));
#58745=CARTESIAN_POINT('Ctrl Pts',(-50.,-10.902828759321,-12.0265041912883));
#58746=CARTESIAN_POINT('Ctrl Pts',(-66.,-10.8709008942817,-11.9247277896931));
#58747=CARTESIAN_POINT('Ctrl Pts',(-50.,-10.8709008942817,-11.9247277896931));
#58748=CARTESIAN_POINT('Ctrl Pts',(-66.,-10.8373429346305,-11.8240218317612));
#58749=CARTESIAN_POINT('Ctrl Pts',(-50.,-10.8373429346305,-11.8240218317612));
#58750=CARTESIAN_POINT('Ctrl Pts',(-66.,-10.8021498170253,-11.7244041527066));
#58751=CARTESIAN_POINT('Ctrl Pts',(-50.,-10.8021498170253,-11.7244041527066));
#58752=CARTESIAN_POINT('Ctrl Pts',(-66.,-10.7653981208323,-11.6258217302963));
#58753=CARTESIAN_POINT('Ctrl Pts',(-50.,-10.7653981208323,-11.6258217302963));
#58754=CARTESIAN_POINT('Ctrl Pts',(-66.,-10.727207120633,-11.5281851158537));
#58755=CARTESIAN_POINT('Ctrl Pts',(-50.,-10.727207120633,-11.5281851158537));
#58756=CARTESIAN_POINT('Ctrl Pts',(-66.,-10.6876760500473,-11.4314236196986));
#58757=CARTESIAN_POINT('Ctrl Pts',(-50.,-10.6876760500473,-11.4314236196986));
#58758=CARTESIAN_POINT('Ctrl Pts',(-66.,-10.6468254580846,-11.3355369696227));
#58759=CARTESIAN_POINT('Ctrl Pts',(-50.,-10.6468254580846,-11.3355369696227));
#58760=CARTESIAN_POINT('Ctrl Pts',(-66.,-10.6045453214218,-11.2406410963124));
#58761=CARTESIAN_POINT('Ctrl Pts',(-50.,-10.6045453214218,-11.2406410963124));
#58762=CARTESIAN_POINT('Ctrl Pts',(-66.,-10.5605176911805,-11.1470361863206));
#58763=CARTESIAN_POINT('Ctrl Pts',(-50.,-10.5605176911805,-11.1470361863206));
#58764=CARTESIAN_POINT('Ctrl Pts',(-66.,-10.5142838856252,-11.055148542648));
#58765=CARTESIAN_POINT('Ctrl Pts',(-50.,-10.5142838856252,-11.055148542648));
#58766=CARTESIAN_POINT('Ctrl Pts',(-66.,-10.4653605771075,-10.9654297310826));
#58767=CARTESIAN_POINT('Ctrl Pts',(-50.,-10.4653605771075,-10.9654297310826));
#58768=CARTESIAN_POINT('Ctrl Pts',(-66.,-10.4133439014856,-10.8782663225706));
#58769=CARTESIAN_POINT('Ctrl Pts',(-50.,-10.4133439014856,-10.8782663225706));
#58770=CARTESIAN_POINT('Ctrl Pts',(-66.,-10.3580097561152,-10.7938927550471));
#58771=CARTESIAN_POINT('Ctrl Pts',(-50.,-10.3580097561152,-10.7938927550471));
#58772=CARTESIAN_POINT('Ctrl Pts',(-66.,-10.2994412084092,-10.7122811666816));
#58773=CARTESIAN_POINT('Ctrl Pts',(-50.,-10.2994412084092,-10.7122811666816));
#58774=CARTESIAN_POINT('Ctrl Pts',(-66.,-10.2379686981643,-10.6331907581101));
#58775=CARTESIAN_POINT('Ctrl Pts',(-50.,-10.2379686981643,-10.6331907581101));
#58776=CARTESIAN_POINT('Ctrl Pts',(-66.,-10.1740622242879,-10.5562581065423));
#58777=CARTESIAN_POINT('Ctrl Pts',(-50.,-10.1740622242879,-10.5562581065423));
#58778=CARTESIAN_POINT('Ctrl Pts',(-66.,-10.108239546518,-10.4810737531071));
#58779=CARTESIAN_POINT('Ctrl Pts',(-50.,-10.108239546518,-10.4810737531071));
#58780=CARTESIAN_POINT('Ctrl Pts',(-66.,-10.0409718699529,-10.4072610342189));
#58781=CARTESIAN_POINT('Ctrl Pts',(-50.,-10.0409718699529,-10.4072610342189));
#58782=CARTESIAN_POINT('Ctrl Pts',(-66.,-9.97258152483879,-10.3345613726147));
#58783=CARTESIAN_POINT('Ctrl Pts',(-50.,-9.97258152483879,-10.3345613726147));
#58784=CARTESIAN_POINT('Ctrl Pts',(-66.,-9.90326213654415,-10.2628187784479));
#58785=CARTESIAN_POINT('Ctrl Pts',(-50.,-9.90326213654415,-10.2628187784479));
#58786=CARTESIAN_POINT('Ctrl Pts',(-66.,-9.84714322904426,-10.2061255176443));
#58787=CARTESIAN_POINT('Ctrl Pts',(-50.,-9.84714322904426,-10.2061255176443));
#58788=CARTESIAN_POINT('Ctrl Pts',(-66.,-9.80469667097528,-10.163986719468));
#58789=CARTESIAN_POINT('Ctrl Pts',(-50.,-9.80469667097528,-10.163986719468));
#58790=CARTESIAN_POINT('Ctrl Pts',(-66.,-9.77624035711837,-10.1360633488319));
#58791=CARTESIAN_POINT('Ctrl Pts',(-50.,-9.77624035711837,-10.1360633488319));
#58792=CARTESIAN_POINT('Ctrl Pts',(-66.,-9.76197254719672,-10.1221439546065));
#58793=CARTESIAN_POINT('Ctrl Pts',(-50.,-9.76197254719672,-10.1221439546065));
#58794=CARTESIAN_POINT('Origin',(-65.75,0.,0.));
#58795=CARTESIAN_POINT('',(-65.5,-13.8963484576857,-9.57377274341605));
#58796=CARTESIAN_POINT('Origin',(-65.5,0.,0.));
#58797=CARTESIAN_POINT('Ctrl Pts',(-65.5,-13.8963484576857,-9.57377274341605));
#58798=CARTESIAN_POINT('Ctrl Pts',(-65.6931595476708,-13.7992573634772,
-9.37423221316899));
#58799=CARTESIAN_POINT('Ctrl Pts',(-65.8611256967054,-13.7088061439983,
-9.2076824840282));
#58800=CARTESIAN_POINT('Ctrl Pts',(-66.,-13.631341547005,-9.07343113870903));
#58801=CARTESIAN_POINT('Origin',(-58.,0.,0.));
#58802=CARTESIAN_POINT('',(-50.5,-13.8963484576857,-9.57377274341605));
#58803=CARTESIAN_POINT('Origin',(-50.5,0.,0.));
#58804=CARTESIAN_POINT('Ctrl Pts',(-50.5,-13.8963484576857,-9.57377274341605));
#58805=CARTESIAN_POINT('Ctrl Pts',(-55.5,-13.8963484576857,-9.57377274341605));
#58806=CARTESIAN_POINT('Ctrl Pts',(-60.5,-13.8963484576857,-9.57377274341605));
#58807=CARTESIAN_POINT('Ctrl Pts',(-65.5,-13.8963484576857,-9.57377274341605));
#58808=CARTESIAN_POINT('Origin',(-50.25,0.,0.));
#58809=CARTESIAN_POINT('Ctrl Pts',(-50.,-13.631341547005,-9.07343113870903));
#58810=CARTESIAN_POINT('Ctrl Pts',(-50.1388743032954,-13.7088061439988,
-9.20768248402894));
#58811=CARTESIAN_POINT('Ctrl Pts',(-50.3068404523299,-13.7992573634776,
-9.37423221316971));
#58812=CARTESIAN_POINT('Ctrl Pts',(-50.5,-13.8963484576857,-9.57377274341605));
#58813=CARTESIAN_POINT('Ctrl Pts',(-66.,-12.6433463826116,-6.1562731014228));
#58814=CARTESIAN_POINT('Ctrl Pts',(-50.,-12.6433463826116,-6.1562731014228));
#58815=CARTESIAN_POINT('Ctrl Pts',(-66.,-12.6639216231176,-6.16735975564195));
#58816=CARTESIAN_POINT('Ctrl Pts',(-50.,-12.6639216231176,-6.16735975564195));
#58817=CARTESIAN_POINT('Ctrl Pts',(-66.,-12.7051868090144,-6.18933938815496));
#58818=CARTESIAN_POINT('Ctrl Pts',(-50.,-12.7051868090144,-6.18933938815496));
#58819=CARTESIAN_POINT('Ctrl Pts',(-66.,-12.7674287029928,-6.22172782249946));
#58820=CARTESIAN_POINT('Ctrl Pts',(-50.,-12.7674287029928,-6.22172782249946));
#58821=CARTESIAN_POINT('Ctrl Pts',(-66.,-12.851107036246,-6.26374871229064));
#58822=CARTESIAN_POINT('Ctrl Pts',(-50.,-12.851107036246,-6.26374871229064));
#58823=CARTESIAN_POINT('Ctrl Pts',(-66.,-12.9568646849259,-6.31427939831312));
#58824=CARTESIAN_POINT('Ctrl Pts',(-50.,-12.9568646849259,-6.31427939831312));
#58825=CARTESIAN_POINT('Ctrl Pts',(-66.,-13.0638062493037,-6.3626601011734));
#58826=CARTESIAN_POINT('Ctrl Pts',(-50.,-13.0638062493037,-6.3626601011734));
#58827=CARTESIAN_POINT('Ctrl Pts',(-66.,-13.1719732880642,-6.40859684907992));
#58828=CARTESIAN_POINT('Ctrl Pts',(-50.,-13.1719732880642,-6.40859684907992));
#58829=CARTESIAN_POINT('Ctrl Pts',(-66.,-13.281428281035,-6.45159976453225));
#58830=CARTESIAN_POINT('Ctrl Pts',(-50.,-13.281428281035,-6.45159976453225));
#58831=CARTESIAN_POINT('Ctrl Pts',(-66.,-13.3922710176287,-6.49104836068956));
#58832=CARTESIAN_POINT('Ctrl Pts',(-50.,-13.3922710176287,-6.49104836068956));
#58833=CARTESIAN_POINT('Ctrl Pts',(-66.,-13.5046637960973,-6.52627657330457));
#58834=CARTESIAN_POINT('Ctrl Pts',(-50.,-13.5046637960973,-6.52627657330457));
#58835=CARTESIAN_POINT('Ctrl Pts',(-66.,-13.6188417913781,-6.55665495690443));
#58836=CARTESIAN_POINT('Ctrl Pts',(-50.,-13.6188417913781,-6.55665495690443));
#58837=CARTESIAN_POINT('Ctrl Pts',(-66.,-13.7351593700424,-6.58166436202222));
#58838=CARTESIAN_POINT('Ctrl Pts',(-50.,-13.7351593700424,-6.58166436202222));
#58839=CARTESIAN_POINT('Ctrl Pts',(-66.,-13.8539565214648,-6.60104137487127));
#58840=CARTESIAN_POINT('Ctrl Pts',(-50.,-13.8539565214648,-6.60104137487127));
#58841=CARTESIAN_POINT('Ctrl Pts',(-66.,-13.9753080627051,-6.61499785909296));
#58842=CARTESIAN_POINT('Ctrl Pts',(-50.,-13.9753080627051,-6.61499785909296));
#58843=CARTESIAN_POINT('Ctrl Pts',(-66.,-14.0988589764351,-6.62435775818486));
#58844=CARTESIAN_POINT('Ctrl Pts',(-50.,-14.0988589764351,-6.62435775818486));
#58845=CARTESIAN_POINT('Ctrl Pts',(-66.,-14.2235033417215,-6.63087754928856));
#58846=CARTESIAN_POINT('Ctrl Pts',(-50.,-14.2235033417215,-6.63087754928856));
#58847=CARTESIAN_POINT('Ctrl Pts',(-66.,-14.3475726821666,-6.63694296762358));
#58848=CARTESIAN_POINT('Ctrl Pts',(-50.,-14.3475726821666,-6.63694296762358));
#58849=CARTESIAN_POINT('Ctrl Pts',(-66.,-14.4696861744433,-6.64444024204806));
#58850=CARTESIAN_POINT('Ctrl Pts',(-50.,-14.4696861744433,-6.64444024204806));
#58851=CARTESIAN_POINT('Ctrl Pts',(-66.,-14.5893646306071,-6.65393139885702));
#58852=CARTESIAN_POINT('Ctrl Pts',(-50.,-14.5893646306071,-6.65393139885702));
#58853=CARTESIAN_POINT('Ctrl Pts',(-66.,-14.7078951610787,-6.6634907630476));
#58854=CARTESIAN_POINT('Ctrl Pts',(-50.,-14.7078951610787,-6.6634907630476));
#58855=CARTESIAN_POINT('Ctrl Pts',(-66.,-14.8286466959702,-6.66830024039538));
#58856=CARTESIAN_POINT('Ctrl Pts',(-50.,-14.8286466959702,-6.66830024039538));
#58857=CARTESIAN_POINT('Ctrl Pts',(-66.,-14.9551891629322,-6.66329671103626));
#58858=CARTESIAN_POINT('Ctrl Pts',(-50.,-14.9551891629322,-6.66329671103626));
#58859=CARTESIAN_POINT('Ctrl Pts',(-66.,-15.0896875773,-6.64543810943336));
#58860=CARTESIAN_POINT('Ctrl Pts',(-50.,-15.0896875773,-6.64543810943336));
#58861=CARTESIAN_POINT('Ctrl Pts',(-66.,-15.2312621759268,-6.61601501775332));
#58862=CARTESIAN_POINT('Ctrl Pts',(-50.,-15.2312621759268,-6.61601501775332));
#58863=CARTESIAN_POINT('Ctrl Pts',(-66.,-15.3741384264112,-6.58326088854155));
#58864=CARTESIAN_POINT('Ctrl Pts',(-50.,-15.3741384264112,-6.58326088854155));
#58865=CARTESIAN_POINT('Ctrl Pts',(-66.,-15.5090614410165,-6.56034427212951));
#58866=CARTESIAN_POINT('Ctrl Pts',(-50.,-15.5090614410165,-6.56034427212951));
#58867=CARTESIAN_POINT('Ctrl Pts',(-66.,-15.6250970135137,-6.56281431696235));
#58868=CARTESIAN_POINT('Ctrl Pts',(-50.,-15.6250970135137,-6.56281431696235));
#58869=CARTESIAN_POINT('Ctrl Pts',(-66.,-15.7111627073129,-6.60642866537431));
#58870=CARTESIAN_POINT('Ctrl Pts',(-50.,-15.7111627073129,-6.60642866537431));
#58871=CARTESIAN_POINT('Ctrl Pts',(-66.,-15.7579605986384,-6.70441211879867));
#58872=CARTESIAN_POINT('Ctrl Pts',(-50.,-15.7579605986384,-6.70441211879867));
#58873=CARTESIAN_POINT('Ctrl Pts',(-66.,-15.7584967454601,-6.86671937924014));
#58874=CARTESIAN_POINT('Ctrl Pts',(-50.,-15.7584967454601,-6.86671937924014));
#58875=CARTESIAN_POINT('Ctrl Pts',(-66.,-15.7075631420906,-7.10076915669713));
#58876=CARTESIAN_POINT('Ctrl Pts',(-50.,-15.7075631420906,-7.10076915669713));
#58877=CARTESIAN_POINT('Ctrl Pts',(-66.,-15.6015340605988,-7.41173254135438));
#58878=CARTESIAN_POINT('Ctrl Pts',(-50.,-15.6015340605988,-7.41173254135438));
#58879=CARTESIAN_POINT('Ctrl Pts',(-66.,-15.438048141096,-7.80298348305155));
#58880=CARTESIAN_POINT('Ctrl Pts',(-50.,-15.438048141096,-7.80298348305155));
#58881=CARTESIAN_POINT('Ctrl Pts',(-66.,-15.2157536026519,-8.27645984483354));
#58882=CARTESIAN_POINT('Ctrl Pts',(-50.,-15.2157536026519,-8.27645984483354));
#58883=CARTESIAN_POINT('Ctrl Pts',(-66.,-14.9340392129229,-8.83304473364892));
#58884=CARTESIAN_POINT('Ctrl Pts',(-50.,-14.9340392129229,-8.83304473364892));
#58885=CARTESIAN_POINT('Ctrl Pts',(-66.,-14.6610342795723,-9.34494709460039));
#58886=CARTESIAN_POINT('Ctrl Pts',(-50.,-14.6610342795723,-9.34494709460039));
#58887=CARTESIAN_POINT('Ctrl Pts',(-66.,-14.4295401925849,-9.76628311391338));
#58888=CARTESIAN_POINT('Ctrl Pts',(-50.,-14.4295401925849,-9.76628311391338));
#58889=CARTESIAN_POINT('Ctrl Pts',(-66.,-14.2633419918951,-10.0637780121554));
#58890=CARTESIAN_POINT('Ctrl Pts',(-50.,-14.2633419918951,-10.0637780121554));
#58891=CARTESIAN_POINT('Ctrl Pts',(-66.,-14.1772756878995,-10.2166765177964));
#58892=CARTESIAN_POINT('Ctrl Pts',(-50.,-14.1772756878995,-10.2166765177964));
#58893=CARTESIAN_POINT('',(-65.5,-15.5455251229224,-6.56523218573333));
#58894=CARTESIAN_POINT('Ctrl Pts',(-66.,-14.9594853178907,-6.65991171291435));
#58895=CARTESIAN_POINT('Ctrl Pts',(-65.7933280154027,-15.195120245778,-6.63878177870532));
#58896=CARTESIAN_POINT('Ctrl Pts',(-65.6370761749496,-15.3970618191913,
-6.56443702203716));
#58897=CARTESIAN_POINT('Ctrl Pts',(-65.5,-15.5455251229224,-6.56523218573333));
#58898=CARTESIAN_POINT('',(-66.,-12.6433463826116,-6.1562731014228));
#58899=CARTESIAN_POINT('',(-50.5,-15.5455251229224,-6.56523218573333));
#58900=CARTESIAN_POINT('Ctrl Pts',(-50.5,-15.5455251229224,-6.56523218573333));
#58901=CARTESIAN_POINT('Ctrl Pts',(-50.4518618349121,-15.4933880463872,
-6.56495294157371));
#58902=CARTESIAN_POINT('Ctrl Pts',(-50.4012423593883,-15.4346954562179,
-6.57371248407322));
#58903=CARTESIAN_POINT('Ctrl Pts',(-50.24411297938,-15.248416451548,-6.60952476775937));
#58904=CARTESIAN_POINT('Ctrl Pts',(-50.1366827452942,-15.1153227377209,
-6.64593740758603));
#58905=CARTESIAN_POINT('Ctrl Pts',(-50.,-14.9594853178907,-6.65991171291435));
#58906=CARTESIAN_POINT('Ctrl Pts',(-65.5,-15.5455251229224,-6.56523218573333));
#58907=CARTESIAN_POINT('Ctrl Pts',(-60.5,-15.5455251229224,-6.56523218573333));
#58908=CARTESIAN_POINT('Ctrl Pts',(-55.5,-15.5455251229224,-6.56523218573333));
#58909=CARTESIAN_POINT('Ctrl Pts',(-50.5,-15.5455251229224,-6.56523218573333));
#58910=CARTESIAN_POINT('Origin',(-66.,0.,0.));
#58911=CARTESIAN_POINT('',(-66.,-11.9725570665522,-7.37643433768308));
#58912=CARTESIAN_POINT('Ctrl Pts',(-66.,-14.1772756878995,-10.2166765177964));
#58913=CARTESIAN_POINT('Ctrl Pts',(-50.,-14.1772756878995,-10.2166765177964));
#58914=CARTESIAN_POINT('Ctrl Pts',(-66.,-14.169090684931,-10.1957080532821));
#58915=CARTESIAN_POINT('Ctrl Pts',(-50.,-14.169090684931,-10.1957080532821));
#58916=CARTESIAN_POINT('Ctrl Pts',(-66.,-14.1526091283973,-10.1538681781678));
#58917=CARTESIAN_POINT('Ctrl Pts',(-50.,-14.1526091283973,-10.1538681781678));
#58918=CARTESIAN_POINT('Ctrl Pts',(-66.,-14.1275521422774,-10.0913995267525));
#58919=CARTESIAN_POINT('Ctrl Pts',(-50.,-14.1275521422774,-10.0913995267525));
#58920=CARTESIAN_POINT('Ctrl Pts',(-66.,-14.0934726306568,-10.008691092668));
#58921=CARTESIAN_POINT('Ctrl Pts',(-50.,-14.0934726306568,-10.008691092668));
#58922=CARTESIAN_POINT('Ctrl Pts',(-66.,-14.0497518771326,-9.9062815985322));
#58923=CARTESIAN_POINT('Ctrl Pts',(-50.,-14.0497518771326,-9.9062815985322));
#58924=CARTESIAN_POINT('Ctrl Pts',(-66.,-14.0049055762784,-9.80485304191326));
#58925=CARTESIAN_POINT('Ctrl Pts',(-50.,-14.0049055762784,-9.80485304191326));
#58926=CARTESIAN_POINT('Ctrl Pts',(-66.,-13.9589323331141,-9.70440911809916));
#58927=CARTESIAN_POINT('Ctrl Pts',(-50.,-13.9589323331141,-9.70440911809916));
#58928=CARTESIAN_POINT('Ctrl Pts',(-66.,-13.9118358290362,-9.60495081840769));
#58929=CARTESIAN_POINT('Ctrl Pts',(-50.,-13.9118358290362,-9.60495081840769));
#58930=CARTESIAN_POINT('Ctrl Pts',(-66.,-13.8636282964938,-9.50647368802256));
#58931=CARTESIAN_POINT('Ctrl Pts',(-50.,-13.8636282964938,-9.50647368802256));
#58932=CARTESIAN_POINT('Ctrl Pts',(-66.,-13.8143244129603,-9.40897518514854));
#58933=CARTESIAN_POINT('Ctrl Pts',(-50.,-13.8143244129603,-9.40897518514854));
#58934=CARTESIAN_POINT('Ctrl Pts',(-66.,-13.7639341278636,-9.31246310590722));
#58935=CARTESIAN_POINT('Ctrl Pts',(-50.,-13.7639341278636,-9.31246310590722));
#58936=CARTESIAN_POINT('Ctrl Pts',(-66.,-13.7124554531318,-9.21696428016702));
#58937=CARTESIAN_POINT('Ctrl Pts',(-50.,-13.7124554531318,-9.21696428016702));
#58938=CARTESIAN_POINT('Ctrl Pts',(-66.,-13.6598685224049,-9.12253151471647));
#58939=CARTESIAN_POINT('Ctrl Pts',(-50.,-13.6598685224049,-9.12253151471647));
#58940=CARTESIAN_POINT('Ctrl Pts',(-66.,-13.606126110027,-9.02925545685226));
#58941=CARTESIAN_POINT('Ctrl Pts',(-50.,-13.606126110027,-9.02925545685226));
#58942=CARTESIAN_POINT('Ctrl Pts',(-66.,-13.5511663152664,-8.93724619299147));
#58943=CARTESIAN_POINT('Ctrl Pts',(-50.,-13.5511663152664,-8.93724619299147));
#58944=CARTESIAN_POINT('Ctrl Pts',(-66.,-13.4949307609898,-8.84660742136017));
#58945=CARTESIAN_POINT('Ctrl Pts',(-50.,-13.4949307609898,-8.84660742136017));
#58946=CARTESIAN_POINT('Ctrl Pts',(-66.,-13.4373825330349,-8.7574108514811));
#58947=CARTESIAN_POINT('Ctrl Pts',(-50.,-13.4373825330349,-8.7574108514811));
#58948=CARTESIAN_POINT('Ctrl Pts',(-66.,-13.3785211625712,-8.66967501744431));
#58949=CARTESIAN_POINT('Ctrl Pts',(-50.,-13.3785211625712,-8.66967501744431));
#58950=CARTESIAN_POINT('Ctrl Pts',(-66.,-13.3184076369901,-8.58332951829382));
#58951=CARTESIAN_POINT('Ctrl Pts',(-50.,-13.3184076369901,-8.58332951829382));
#58952=CARTESIAN_POINT('Ctrl Pts',(-66.,-13.2571352386615,-8.49825805316535));
#58953=CARTESIAN_POINT('Ctrl Pts',(-50.,-13.2571352386615,-8.49825805316535));
#58954=CARTESIAN_POINT('Ctrl Pts',(-66.,-13.1947825037901,-8.41436747482742));
#58955=CARTESIAN_POINT('Ctrl Pts',(-50.,-13.1947825037901,-8.41436747482742));
#58956=CARTESIAN_POINT('Ctrl Pts',(-66.,-13.1313692681049,-8.3316524092927));
#58957=CARTESIAN_POINT('Ctrl Pts',(-50.,-13.1313692681049,-8.3316524092927));
#58958=CARTESIAN_POINT('Ctrl Pts',(-66.,-13.0668177956572,-8.25025250675973));
#58959=CARTESIAN_POINT('Ctrl Pts',(-50.,-13.0668177956572,-8.25025250675973));
#58960=CARTESIAN_POINT('Ctrl Pts',(-66.,-13.0008947798771,-8.17053759353955));
#58961=CARTESIAN_POINT('Ctrl Pts',(-50.,-13.0008947798771,-8.17053759353955));
#58962=CARTESIAN_POINT('Ctrl Pts',(-66.,-12.9332619666045,-8.09303464904925));
#58963=CARTESIAN_POINT('Ctrl Pts',(-50.,-12.9332619666045,-8.09303464904925));
#58964=CARTESIAN_POINT('Ctrl Pts',(-66.,-12.8635635126628,-8.01830125100551));
#58965=CARTESIAN_POINT('Ctrl Pts',(-50.,-12.8635635126628,-8.01830125100551));
#58966=CARTESIAN_POINT('Ctrl Pts',(-66.,-12.7915043783298,-7.9468122624453));
#58967=CARTESIAN_POINT('Ctrl Pts',(-50.,-12.7915043783298,-7.9468122624453));
#58968=CARTESIAN_POINT('Ctrl Pts',(-66.,-12.7169258039014,-7.87885048806616));
#58969=CARTESIAN_POINT('Ctrl Pts',(-50.,-12.7169258039014,-7.87885048806616));
#58970=CARTESIAN_POINT('Ctrl Pts',(-66.,-12.6399013181197,-7.81436828334278));
#58971=CARTESIAN_POINT('Ctrl Pts',(-50.,-12.6399013181197,-7.81436828334278));
#58972=CARTESIAN_POINT('Ctrl Pts',(-66.,-12.5606910950408,-7.75305023703025));
#58973=CARTESIAN_POINT('Ctrl Pts',(-50.,-12.5606910950408,-7.75305023703025));
#58974=CARTESIAN_POINT('Ctrl Pts',(-66.,-12.4796599881192,-7.69442745995809));
#58975=CARTESIAN_POINT('Ctrl Pts',(-50.,-12.4796599881192,-7.69442745995809));
#58976=CARTESIAN_POINT('Ctrl Pts',(-66.,-12.3972076624386,-7.63797459554787));
#58977=CARTESIAN_POINT('Ctrl Pts',(-50.,-12.3972076624386,-7.63797459554787));
#58978=CARTESIAN_POINT('Ctrl Pts',(-66.,-12.3136968468978,-7.58320962985052));
#58979=CARTESIAN_POINT('Ctrl Pts',(-50.,-12.3136968468978,-7.58320962985052));
#58980=CARTESIAN_POINT('Ctrl Pts',(-66.,-12.2293754395952,-7.5298019490105));
#58981=CARTESIAN_POINT('Ctrl Pts',(-50.,-12.2293754395952,-7.5298019490105));
#58982=CARTESIAN_POINT('Ctrl Pts',(-66.,-12.144392189705,-7.47755231121817));
#58983=CARTESIAN_POINT('Ctrl Pts',(-50.,-12.144392189705,-7.47755231121817));
#58984=CARTESIAN_POINT('Ctrl Pts',(-66.,-12.0759373202474,-7.43659637822836));
#58985=CARTESIAN_POINT('Ctrl Pts',(-50.,-12.0759373202474,-7.43659637822836));
#58986=CARTESIAN_POINT('Ctrl Pts',(-66.,-12.0243448058902,-7.40633747762124));
#58987=CARTESIAN_POINT('Ctrl Pts',(-50.,-12.0243448058902,-7.40633747762124));
#58988=CARTESIAN_POINT('Ctrl Pts',(-66.,-11.9898382395678,-7.38636816850343));
#58989=CARTESIAN_POINT('Ctrl Pts',(-50.,-11.9898382395678,-7.38636816850343));
#58990=CARTESIAN_POINT('Ctrl Pts',(-66.,-11.9725570665522,-7.37643433768309));
#58991=CARTESIAN_POINT('Ctrl Pts',(-50.,-11.9725570665522,-7.37643433768309));
#58992=CARTESIAN_POINT('Origin',(-65.75,0.,0.));
#58993=CARTESIAN_POINT('',(-65.5,-15.8406695805923,-5.81711373779967));
#58994=CARTESIAN_POINT('Origin',(-65.5,0.,0.));
#58995=CARTESIAN_POINT('Ctrl Pts',(-65.5,-15.8406695805923,-5.81711373779968));
#58996=CARTESIAN_POINT('Ctrl Pts',(-65.6931595476752,-15.6970050696912,
-5.64798771349928));
#58997=CARTESIAN_POINT('Ctrl Pts',(-65.8611256967103,-15.5679763082525,
-5.509164753929));
#58998=CARTESIAN_POINT('Ctrl Pts',(-66.,-15.4595584521058,-5.39839582338346));
#58999=CARTESIAN_POINT('Origin',(-58.,0.,0.));
#59000=CARTESIAN_POINT('',(-50.5,-15.8406695805923,-5.81711373779967));
#59001=CARTESIAN_POINT('Origin',(-50.5,0.,0.));
#59002=CARTESIAN_POINT('Ctrl Pts',(-50.5,-15.8406695805923,-5.81711373779967));
#59003=CARTESIAN_POINT('Ctrl Pts',(-55.5,-15.8406695805923,-5.81711373779967));
#59004=CARTESIAN_POINT('Ctrl Pts',(-60.5,-15.8406695805923,-5.81711373779967));
#59005=CARTESIAN_POINT('Ctrl Pts',(-65.5,-15.8406695805923,-5.81711373779967));
#59006=CARTESIAN_POINT('Origin',(-50.25,0.,0.));
#59007=CARTESIAN_POINT('Ctrl Pts',(-50.,-15.4595584521058,-5.39839582338346));
#59008=CARTESIAN_POINT('Ctrl Pts',(-50.1388743032875,-15.5679763082507,
-5.50916475392723));
#59009=CARTESIAN_POINT('Ctrl Pts',(-50.3068404523245,-15.697005069691,-5.64798771349904));
#59010=CARTESIAN_POINT('Ctrl Pts',(-50.5,-15.8406695805923,-5.81711373779967));
#59011=CARTESIAN_POINT('Ctrl Pts',(-66.,-13.7771352694631,-2.8185900760694));
#59012=CARTESIAN_POINT('Ctrl Pts',(-50.,-13.7771352694631,-2.8185900760694));
#59013=CARTESIAN_POINT('Ctrl Pts',(-66.,-13.7998212397401,-2.82421156841951));
#59014=CARTESIAN_POINT('Ctrl Pts',(-50.,-13.7998212397401,-2.82421156841951));
#59015=CARTESIAN_POINT('Ctrl Pts',(-66.,-13.8452561162702,-2.83523843593487));
#59016=CARTESIAN_POINT('Ctrl Pts',(-50.,-13.8452561162702,-2.83523843593487));
#59017=CARTESIAN_POINT('Ctrl Pts',(-66.,-13.913597242777,-2.85113039846586));
#59018=CARTESIAN_POINT('Ctrl Pts',(-50.,-13.913597242777,-2.85113039846586));
#59019=CARTESIAN_POINT('Ctrl Pts',(-66.,-14.0050968376581,-2.87102116947837));
#59020=CARTESIAN_POINT('Ctrl Pts',(-50.,-14.0050968376581,-2.87102116947837));
#59021=CARTESIAN_POINT('Ctrl Pts',(-66.,-14.1200983859353,-2.89366348336299));
#59022=CARTESIAN_POINT('Ctrl Pts',(-50.,-14.1200983859353,-2.89366348336299));
#59023=CARTESIAN_POINT('Ctrl Pts',(-66.,-14.2357119759516,-2.91392893189869));
#59024=CARTESIAN_POINT('Ctrl Pts',(-50.,-14.2357119759516,-2.91392893189869));
#59025=CARTESIAN_POINT('Ctrl Pts',(-66.,-14.3519047529378,-2.93152244373364));
#59026=CARTESIAN_POINT('Ctrl Pts',(-50.,-14.3519047529378,-2.93152244373364));
#59027=CARTESIAN_POINT('Ctrl Pts',(-66.,-14.4686154062224,-2.94595399366867));
#59028=CARTESIAN_POINT('Ctrl Pts',(-50.,-14.4686154062224,-2.94595399366867));
#59029=CARTESIAN_POINT('Ctrl Pts',(-66.,-14.5857862813476,-2.95659777198027));
#59030=CARTESIAN_POINT('Ctrl Pts',(-50.,-14.5857862813476,-2.95659777198027));
#59031=CARTESIAN_POINT('Ctrl Pts',(-66.,-14.703408934225,-2.96276827812033));
#59032=CARTESIAN_POINT('Ctrl Pts',(-50.,-14.703408934225,-2.96276827812033));
#59033=CARTESIAN_POINT('Ctrl Pts',(-66.,-14.8215546146151,-2.96379735617437));
#59034=CARTESIAN_POINT('Ctrl Pts',(-50.,-14.8215546146151,-2.96379735617437));
#59035=CARTESIAN_POINT('Ctrl Pts',(-66.,-14.9404374487894,-2.959094039328));
#59036=CARTESIAN_POINT('Ctrl Pts',(-50.,-14.9404374487894,-2.959094039328));
#59037=CARTESIAN_POINT('Ctrl Pts',(-66.,-15.0603212363863,-2.9483186375038));
#59038=CARTESIAN_POINT('Ctrl Pts',(-50.,-15.0603212363863,-2.9483186375038));
#59039=CARTESIAN_POINT('Ctrl Pts',(-66.,-15.181331132295,-2.93165775201116));
#59040=CARTESIAN_POINT('Ctrl Pts',(-50.,-15.181331132295,-2.93165775201116));
#59041=CARTESIAN_POINT('Ctrl Pts',(-66.,-15.3033281791249,-2.90999772986683));
#59042=CARTESIAN_POINT('Ctrl Pts',(-50.,-15.3033281791249,-2.90999772986683));
#59043=CARTESIAN_POINT('Ctrl Pts',(-66.,-15.4256780185848,-2.88531489660512));
#59044=CARTESIAN_POINT('Ctrl Pts',(-50.,-15.4256780185848,-2.88531489660512));
#59045=CARTESIAN_POINT('Ctrl Pts',(-66.,-15.5473579007536,-2.86033496839371));
#59046=CARTESIAN_POINT('Ctrl Pts',(-50.,-15.5473579007536,-2.86033496839371));
#59047=CARTESIAN_POINT('Ctrl Pts',(-66.,-15.6674994694501,-2.83722831154002));
#59048=CARTESIAN_POINT('Ctrl Pts',(-50.,-15.6674994694501,-2.83722831154002));
#59049=CARTESIAN_POINT('Ctrl Pts',(-66.,-15.7857783615561,-2.81665846444538));
#59050=CARTESIAN_POINT('Ctrl Pts',(-50.,-15.7857783615561,-2.81665846444538));
#59051=CARTESIAN_POINT('Ctrl Pts',(-66.,-15.9029623546524,-2.7964401593829));
#59052=CARTESIAN_POINT('Ctrl Pts',(-50.,-15.9029623546524,-2.7964401593829));
#59053=CARTESIAN_POINT('Ctrl Pts',(-66.,-16.0211163264077,-2.77106885256863));
#59054=CARTESIAN_POINT('Ctrl Pts',(-50.,-16.0211163264077,-2.77106885256863));
#59055=CARTESIAN_POINT('Ctrl Pts',(-66.,-16.1424389019231,-2.73475268645485));
#59056=CARTESIAN_POINT('Ctrl Pts',(-50.,-16.1424389019231,-2.73475268645485));
#59057=CARTESIAN_POINT('Ctrl Pts',(-66.,-16.2682705476607,-2.68400675016798));
#59058=CARTESIAN_POINT('Ctrl Pts',(-50.,-16.2682705476607,-2.68400675016798));
#59059=CARTESIAN_POINT('Ctrl Pts',(-66.,-16.3980800945842,-2.62029986806045));
#59060=CARTESIAN_POINT('Ctrl Pts',(-50.,-16.3980800945842,-2.62029986806045));
#59061=CARTESIAN_POINT('Ctrl Pts',(-66.,-16.5283220042307,-2.55304289143699));
#59062=CARTESIAN_POINT('Ctrl Pts',(-50.,-16.5283220042307,-2.55304289143699));
#59063=CARTESIAN_POINT('Ctrl Pts',(-66.,-16.6533070334764,-2.49729225339212));
#59064=CARTESIAN_POINT('Ctrl Pts',(-50.,-16.6533070334764,-2.49729225339212));
#59065=CARTESIAN_POINT('Ctrl Pts',(-66.,-16.7663114102599,-2.470827823793));
#59066=CARTESIAN_POINT('Ctrl Pts',(-50.,-16.7663114102599,-2.470827823793));
#59067=CARTESIAN_POINT('Ctrl Pts',(-66.,-16.86051963941,-2.49166827956873));
#59068=CARTESIAN_POINT('Ctrl Pts',(-50.,-16.86051963941,-2.49166827956873));
#59069=CARTESIAN_POINT('Ctrl Pts',(-66.,-16.9302147829003,-2.57493524031151));
#59070=CARTESIAN_POINT('Ctrl Pts',(-50.,-16.9302147829003,-2.57493524031151));
#59071=CARTESIAN_POINT('Ctrl Pts',(-66.,-16.971098259969,-2.73200998541143));
#59072=CARTESIAN_POINT('Ctrl Pts',(-50.,-16.971098259969,-2.73200998541143));
#59073=CARTESIAN_POINT('Ctrl Pts',(-66.,-16.9799706421563,-2.97137333079705));
#59074=CARTESIAN_POINT('Ctrl Pts',(-50.,-16.9799706421563,-2.97137333079705));
#59075=CARTESIAN_POINT('Ctrl Pts',(-66.,-16.9546061082763,-3.29893558921601));
#59076=CARTESIAN_POINT('Ctrl Pts',(-50.,-16.9546061082763,-3.29893558921601));
#59077=CARTESIAN_POINT('Ctrl Pts',(-66.,-16.8935565521081,-3.71855195799381));
#59078=CARTESIAN_POINT('Ctrl Pts',(-50.,-16.8935565521081,-3.71855195799381));
#59079=CARTESIAN_POINT('Ctrl Pts',(-66.,-16.795994588347,-4.23243559289131));
#59080=CARTESIAN_POINT('Ctrl Pts',(-50.,-16.795994588347,-4.23243559289131));
#59081=CARTESIAN_POINT('Ctrl Pts',(-66.,-16.6615478074051,-4.84159386373095));
#59082=CARTESIAN_POINT('Ctrl Pts',(-50.,-16.6615478074051,-4.84159386373095));
#59083=CARTESIAN_POINT('Ctrl Pts',(-66.,-16.5244247664411,-5.40530743676095));
#59084=CARTESIAN_POINT('Ctrl Pts',(-50.,-16.5244247664411,-5.40530743676095));
#59085=CARTESIAN_POINT('Ctrl Pts',(-66.,-16.4049854989856,-5.87097664861672));
#59086=CARTESIAN_POINT('Ctrl Pts',(-50.,-16.4049854989856,-5.87097664861672));
#59087=CARTESIAN_POINT('Ctrl Pts',(-66.,-16.3179926930635,-6.20045700935217));
#59088=CARTESIAN_POINT('Ctrl Pts',(-50.,-16.3179926930635,-6.20045700935217));
#59089=CARTESIAN_POINT('Ctrl Pts',(-66.,-16.2726546323884,-6.36995574670713));
#59090=CARTESIAN_POINT('Ctrl Pts',(-50.,-16.2726546323884,-6.36995574670713));
#59091=CARTESIAN_POINT('',(-65.5,-16.6898407164458,-2.49295845526303));
#59092=CARTESIAN_POINT('Ctrl Pts',(-66.,-16.1457582704724,-2.73040562398164));
#59093=CARTESIAN_POINT('Ctrl Pts',(-65.7933280154031,-16.3687354928431,
-2.65133950188281));
#59094=CARTESIAN_POINT('Ctrl Pts',(-65.6370761749492,-16.5458439112369,
-2.5291095953495));
#59095=CARTESIAN_POINT('Ctrl Pts',(-65.5,-16.6898407164458,-2.49295845526303));
#59096=CARTESIAN_POINT('',(-66.,-13.7771352694631,-2.8185900760694));
#59097=CARTESIAN_POINT('',(-50.5,-16.6898407164458,-2.49295845526303));
#59098=CARTESIAN_POINT('Ctrl Pts',(-50.5,-16.6898407164458,-2.49295845526304));
#59099=CARTESIAN_POINT('Ctrl Pts',(-50.451861834912,-16.6392721768446,-2.50565394775287));
#59100=CARTESIAN_POINT('Ctrl Pts',(-50.401242359388,-16.5846019319592,-2.52873454674382));
#59101=CARTESIAN_POINT('Ctrl Pts',(-50.2441129793792,-16.4130813775527,
-2.6097474263366));
#59102=CARTESIAN_POINT('Ctrl Pts',(-50.1366827452938,-16.293224502778,-2.67811515679866));
#59103=CARTESIAN_POINT('Ctrl Pts',(-50.,-16.1457582704724,-2.73040562398164));
#59104=CARTESIAN_POINT('Ctrl Pts',(-65.5,-16.6898407164458,-2.49295845526303));
#59105=CARTESIAN_POINT('Ctrl Pts',(-60.5,-16.6898407164458,-2.49295845526303));
#59106=CARTESIAN_POINT('Ctrl Pts',(-55.5,-16.6898407164458,-2.49295845526303));
#59107=CARTESIAN_POINT('Ctrl Pts',(-50.5,-16.6898407164458,-2.49295845526303));
#59108=CARTESIAN_POINT('Origin',(-66.,0.,0.));
#59109=CARTESIAN_POINT('',(-66.,-13.4308617934315,-4.16723622269519));
#59110=CARTESIAN_POINT('Ctrl Pts',(-66.,-16.2726546323884,-6.36995574670713));
#59111=CARTESIAN_POINT('Ctrl Pts',(-50.,-16.2726546323884,-6.36995574670713));
#59112=CARTESIAN_POINT('Ctrl Pts',(-66.,-16.2595121312652,-6.35168157252855));
#59113=CARTESIAN_POINT('Ctrl Pts',(-50.,-16.2595121312652,-6.35168157252855));
#59114=CARTESIAN_POINT('Ctrl Pts',(-66.,-16.2331432193164,-6.31525497046376));
#59115=CARTESIAN_POINT('Ctrl Pts',(-50.,-16.2331432193164,-6.31525497046376));
#59116=CARTESIAN_POINT('Ctrl Pts',(-66.,-16.1933381226201,-6.26098030565532));
#59117=CARTESIAN_POINT('Ctrl Pts',(-50.,-16.1933381226201,-6.26098030565532));
#59118=CARTESIAN_POINT('Ctrl Pts',(-66.,-16.1397605303849,-6.18934553901729));
#59119=CARTESIAN_POINT('Ctrl Pts',(-50.,-16.1397605303849,-6.18934553901729));
#59120=CARTESIAN_POINT('Ctrl Pts',(-66.,-16.0719451391882,-6.1010263367184));
#59121=CARTESIAN_POINT('Ctrl Pts',(-50.,-16.0719451391882,-6.1010263367184));
#59122=CARTESIAN_POINT('Ctrl Pts',(-66.,-16.0032835110412,-6.01393716621888));
#59123=CARTESIAN_POINT('Ctrl Pts',(-50.,-16.0032835110412,-6.01393716621888));
#59124=CARTESIAN_POINT('Ctrl Pts',(-66.,-15.9337752137699,-5.92808195363001));
#59125=CARTESIAN_POINT('Ctrl Pts',(-50.,-15.9337752137699,-5.92808195363001));
#59126=CARTESIAN_POINT('Ctrl Pts',(-66.,-15.8634240596442,-5.84346074359936));
#59127=CARTESIAN_POINT('Ctrl Pts',(-50.,-15.8634240596442,-5.84346074359936));
#59128=CARTESIAN_POINT('Ctrl Pts',(-66.,-15.7922407889403,-5.76006617918052));
#59129=CARTESIAN_POINT('Ctrl Pts',(-50.,-15.7922407889403,-5.76006617918052));
#59130=CARTESIAN_POINT('Ctrl Pts',(-66.,-15.720238985893,-5.67789214829422));
#59131=CARTESIAN_POINT('Ctrl Pts',(-50.,-15.720238985893,-5.67789214829422));
#59132=CARTESIAN_POINT('Ctrl Pts',(-66.,-15.6474302261674,-5.59694372781046));
#59133=CARTESIAN_POINT('Ctrl Pts',(-50.,-15.6474302261674,-5.59694372781046));
#59134=CARTESIAN_POINT('Ctrl Pts',(-66.,-15.5738192564671,-5.5172473991014));
#59135=CARTESIAN_POINT('Ctrl Pts',(-50.,-15.5738192564671,-5.5172473991014));
#59136=CARTESIAN_POINT('Ctrl Pts',(-66.,-15.4993999670851,-5.43885925049602));
#59137=CARTESIAN_POINT('Ctrl Pts',(-50.,-15.4993999670851,-5.43885925049602));
#59138=CARTESIAN_POINT('Ctrl Pts',(-66.,-15.424149159112,-5.36187882598251));
#59139=CARTESIAN_POINT('Ctrl Pts',(-50.,-15.424149159112,-5.36187882598251));
#59140=CARTESIAN_POINT('Ctrl Pts',(-66.,-15.3480342539202,-5.28642814749671));
#59141=CARTESIAN_POINT('Ctrl Pts',(-50.,-15.3480342539202,-5.28642814749671));
#59142=CARTESIAN_POINT('Ctrl Pts',(-66.,-15.2710244971014,-5.21262217319695));
#59143=CARTESIAN_POINT('Ctrl Pts',(-50.,-15.2710244971014,-5.21262217319695));
#59144=CARTESIAN_POINT('Ctrl Pts',(-66.,-15.1931019676527,-5.14053953989829));
#59145=CARTESIAN_POINT('Ctrl Pts',(-50.,-15.1931019676527,-5.14053953989829));
#59146=CARTESIAN_POINT('Ctrl Pts',(-66.,-15.1142708207137,-5.07019831600168));
#59147=CARTESIAN_POINT('Ctrl Pts',(-50.,-15.1142708207137,-5.07019831600168));
#59148=CARTESIAN_POINT('Ctrl Pts',(-66.,-15.0345726196388,-5.00151514537911));
#59149=CARTESIAN_POINT('Ctrl Pts',(-50.,-15.0345726196388,-5.00151514537911));
#59150=CARTESIAN_POINT('Ctrl Pts',(-66.,-14.954068793312,-4.9343541825898));
#59151=CARTESIAN_POINT('Ctrl Pts',(-50.,-14.954068793312,-4.9343541825898));
#59152=CARTESIAN_POINT('Ctrl Pts',(-66.,-14.8728122458042,-4.86860567563393));
#59153=CARTESIAN_POINT('Ctrl Pts',(-50.,-14.8728122458042,-4.86860567563393));
#59154=CARTESIAN_POINT('Ctrl Pts',(-66.,-14.7908208532122,-4.80425948641264));
#59155=CARTESIAN_POINT('Ctrl Pts',(-50.,-14.7908208532122,-4.80425948641264));
#59156=CARTESIAN_POINT('Ctrl Pts',(-66.,-14.7080540513971,-4.74147020990105));
#59157=CARTESIAN_POINT('Ctrl Pts',(-50.,-14.7080540513971,-4.74147020990105));
#59158=CARTESIAN_POINT('Ctrl Pts',(-66.,-14.6243778356077,-4.68065407462106));
#59159=CARTESIAN_POINT('Ctrl Pts',(-50.,-14.6243778356077,-4.68065407462106));
#59160=CARTESIAN_POINT('Ctrl Pts',(-66.,-14.5395956330118,-4.62240562435127));
#59161=CARTESIAN_POINT('Ctrl Pts',(-50.,-14.5395956330118,-4.62240562435127));
#59162=CARTESIAN_POINT('Ctrl Pts',(-66.,-14.4535014438403,-4.56735341407851));
#59163=CARTESIAN_POINT('Ctrl Pts',(-50.,-14.4535014438403,-4.56735341407851));
#59164=CARTESIAN_POINT('Ctrl Pts',(-66.,-14.3659275912213,-4.51603076153944));
#59165=CARTESIAN_POINT('Ctrl Pts',(-50.,-14.3659275912213,-4.51603076153944));
#59166=CARTESIAN_POINT('Ctrl Pts',(-66.,-14.2767906338471,-4.4687510685349));
#59167=CARTESIAN_POINT('Ctrl Pts',(-50.,-14.2767906338471,-4.4687510685349));
#59168=CARTESIAN_POINT('Ctrl Pts',(-66.,-14.1861499417075,-4.42544990152536));
#59169=CARTESIAN_POINT('Ctrl Pts',(-50.,-14.1861499417075,-4.42544990152536));
#59170=CARTESIAN_POINT('Ctrl Pts',(-66.,-14.0941790754254,-4.38575705583354));
#59171=CARTESIAN_POINT('Ctrl Pts',(-50.,-14.0941790754254,-4.38575705583354));
#59172=CARTESIAN_POINT('Ctrl Pts',(-66.,-14.0011148179182,-4.34912763794002));
#59173=CARTESIAN_POINT('Ctrl Pts',(-50.,-14.0011148179182,-4.34912763794002));
#59174=CARTESIAN_POINT('Ctrl Pts',(-66.,-13.9072136271877,-4.31495340364481));
#59175=CARTESIAN_POINT('Ctrl Pts',(-50.,-13.9072136271877,-4.31495340364481));
#59176=CARTESIAN_POINT('Ctrl Pts',(-66.,-13.8127069643429,-4.28267727534445));
#59177=CARTESIAN_POINT('Ctrl Pts',(-50.,-13.8127069643429,-4.28267727534445));
#59178=CARTESIAN_POINT('Ctrl Pts',(-66.,-13.717752718985,-4.25191737627554));
#59179=CARTESIAN_POINT('Ctrl Pts',(-50.,-13.717752718985,-4.25191737627554));
#59180=CARTESIAN_POINT('Ctrl Pts',(-66.,-13.6224454176364,-4.22244373176092));
#59181=CARTESIAN_POINT('Ctrl Pts',(-50.,-13.6224454176364,-4.22244373176092));
#59182=CARTESIAN_POINT('Ctrl Pts',(-66.,-13.5459558574286,-4.19979853847996));
#59183=CARTESIAN_POINT('Ctrl Pts',(-50.,-13.5459558574286,-4.19979853847996));
#59184=CARTESIAN_POINT('Ctrl Pts',(-66.,-13.4884591342042,-4.1833208134517));
#59185=CARTESIAN_POINT('Ctrl Pts',(-50.,-13.4884591342042,-4.1833208134517));
#59186=CARTESIAN_POINT('Ctrl Pts',(-66.,-13.4500704898848,-4.17256031098595));
#59187=CARTESIAN_POINT('Ctrl Pts',(-50.,-13.4500704898848,-4.17256031098595));
#59188=CARTESIAN_POINT('Ctrl Pts',(-66.,-13.4308617934315,-4.1672362226952));
#59189=CARTESIAN_POINT('Ctrl Pts',(-50.,-13.4308617934315,-4.1672362226952));
#59190=CARTESIAN_POINT('Origin',(-65.75,0.,0.));
#59191=CARTESIAN_POINT('',(-65.5,-16.7896631758428,-1.69494408218955));
#59192=CARTESIAN_POINT('Origin',(-65.5,0.,0.));
#59193=CARTESIAN_POINT('Ctrl Pts',(-65.5,-16.7896631758444,-1.69494408219071));
#59194=CARTESIAN_POINT('Ctrl Pts',(-65.5831526942313,-16.7116597831043,
-1.63980921666946));
#59195=CARTESIAN_POINT('Ctrl Pts',(-65.6668642214866,-16.632756953137,-1.58602207616305));
#59196=CARTESIAN_POINT('Ctrl Pts',(-65.7504318115564,-16.5536453909681,
-1.53405266616925));
#59197=CARTESIAN_POINT('Ctrl Pts',(-65.8128644036996,-16.4945418570434,
-1.49522678911148));
#59198=CARTESIAN_POINT('Ctrl Pts',(-65.8752166580337,-16.4353232089395,
-1.45741341708658));
#59199=CARTESIAN_POINT('Ctrl Pts',(-65.9371955299004,-16.3762823874727,
-1.42085043219345));
#59200=CARTESIAN_POINT('Ctrl Pts',(-65.9581769321365,-16.3562955889681,
-1.40847294499675));
#59201=CARTESIAN_POINT('Ctrl Pts',(-65.9791155450307,-16.3363291519437,
-1.39623925385214));
#59202=CARTESIAN_POINT('Ctrl Pts',(-66.,-16.3163944433819,-1.38415944456368));
#59203=CARTESIAN_POINT('Origin',(-58.,0.,0.));
#59204=CARTESIAN_POINT('',(-50.5,-16.7896631758428,-1.69494408218955));
#59205=CARTESIAN_POINT('Origin',(-50.5,0.,0.));
#59206=CARTESIAN_POINT('Ctrl Pts',(-50.5,-16.7896631758428,-1.69494408218955));
#59207=CARTESIAN_POINT('Ctrl Pts',(-55.5,-16.7896631758428,-1.69494408218955));
#59208=CARTESIAN_POINT('Ctrl Pts',(-60.5,-16.7896631758428,-1.69494408218955));
#59209=CARTESIAN_POINT('Ctrl Pts',(-65.5,-16.7896631758428,-1.69494408218955));
#59210=CARTESIAN_POINT('Origin',(-50.25,0.,0.));
#59211=CARTESIAN_POINT('Ctrl Pts',(-50.,-16.3163944433819,-1.38415944456368));
#59212=CARTESIAN_POINT('Ctrl Pts',(-50.0654889940711,-16.3789052444887,
-1.42203903299602));
#59213=CARTESIAN_POINT('Ctrl Pts',(-50.1315105283009,-16.4417279886672,
-1.46142918595527));
#59214=CARTESIAN_POINT('Ctrl Pts',(-50.1977140592374,-16.5045125667653,
-1.50202867177275));
#59215=CARTESIAN_POINT('Ctrl Pts',(-50.271970484712,-16.5749341632954,-1.54756661590145));
#59216=CARTESIAN_POINT('Ctrl Pts',(-50.346455875293,-16.6453067355572,-1.59462664329308));
#59217=CARTESIAN_POINT('Ctrl Pts',(-50.4206755781269,-16.715139000376,-1.64286733678613));
#59218=CARTESIAN_POINT('Ctrl Pts',(-50.4471583693976,-16.7400562827491,
-1.66008039703497));
#59219=CARTESIAN_POINT('Ctrl Pts',(-50.4736073338915,-16.7649048980886,
-1.67744427523805));
#59220=CARTESIAN_POINT('Ctrl Pts',(-50.5,-16.7896631758444,-1.69494408219072));
#59221=CARTESIAN_POINT('Ctrl Pts',(-66.,-14.045256078575,0.696195329812624));
#59222=CARTESIAN_POINT('Ctrl Pts',(-50.,-14.045256078575,0.696195329812624));
#59223=CARTESIAN_POINT('Ctrl Pts',(-66.,-14.0686273356774,0.696392218370307));
#59224=CARTESIAN_POINT('Ctrl Pts',(-50.,-14.0686273356774,0.696392218370307));
#59225=CARTESIAN_POINT('Ctrl Pts',(-66.,-14.1153770624506,0.697010974492569));
#59226=CARTESIAN_POINT('Ctrl Pts',(-50.,-14.1153770624506,0.697010974492569));
#59227=CARTESIAN_POINT('Ctrl Pts',(-66.,-14.1855232971663,0.698614034227448));
#59228=CARTESIAN_POINT('Ctrl Pts',(-50.,-14.1855232971663,0.698614034227448));
#59229=CARTESIAN_POINT('Ctrl Pts',(-66.,-14.279094897617,0.702103192289484));
#59230=CARTESIAN_POINT('Ctrl Pts',(-50.,-14.279094897617,0.702103192289484));
#59231=CARTESIAN_POINT('Ctrl Pts',(-66.,-14.3961143752671,0.708771950396692));
#59232=CARTESIAN_POINT('Ctrl Pts',(-50.,-14.3961143752671,0.708771950396692));
#59233=CARTESIAN_POINT('Ctrl Pts',(-66.,-14.5131355638642,0.717895108848178));
#59234=CARTESIAN_POINT('Ctrl Pts',(-50.,-14.5131355638642,0.717895108848178));
#59235=CARTESIAN_POINT('Ctrl Pts',(-66.,-14.6300532595709,0.7297502981378));
#59236=CARTESIAN_POINT('Ctrl Pts',(-50.,-14.6300532595709,0.7297502981378));
#59237=CARTESIAN_POINT('Ctrl Pts',(-66.,-14.7466862135917,0.744796901078022));
#59238=CARTESIAN_POINT('Ctrl Pts',(-50.,-14.7466862135917,0.744796901078022));
#59239=CARTESIAN_POINT('Ctrl Pts',(-66.,-14.8628229502399,0.763626728348506));
#59240=CARTESIAN_POINT('Ctrl Pts',(-50.,-14.8628229502399,0.763626728348506));
#59241=CARTESIAN_POINT('Ctrl Pts',(-66.,-14.97828481366,0.786901644277719));
#59242=CARTESIAN_POINT('Ctrl Pts',(-50.,-14.97828481366,0.786901644277719));
#59243=CARTESIAN_POINT('Ctrl Pts',(-66.,-15.0929746515511,0.81528653252832));
#59244=CARTESIAN_POINT('Ctrl Pts',(-50.,-15.0929746515511,0.81528653252832));
#59245=CARTESIAN_POINT('Ctrl Pts',(-66.,-15.2069528955437,0.849407044643804));
#59246=CARTESIAN_POINT('Ctrl Pts',(-50.,-15.2069528955437,0.849407044643804));
#59247=CARTESIAN_POINT('Ctrl Pts',(-66.,-15.3203905800386,0.889657803015486));
#59248=CARTESIAN_POINT('Ctrl Pts',(-50.,-15.3203905800386,0.889657803015486));
#59249=CARTESIAN_POINT('Ctrl Pts',(-66.,-15.4334553338124,0.935889193512498));
#59250=CARTESIAN_POINT('Ctrl Pts',(-50.,-15.4334553338124,0.935889193512498));
#59251=CARTESIAN_POINT('Ctrl Pts',(-66.,-15.5462329906162,0.987208158041752));
#59252=CARTESIAN_POINT('Ctrl Pts',(-50.,-15.5462329906162,0.987208158041752));
#59253=CARTESIAN_POINT('Ctrl Pts',(-66.,-15.6586006138651,1.04154270247793));
#59254=CARTESIAN_POINT('Ctrl Pts',(-50.,-15.6586006138651,1.04154270247793));
#59255=CARTESIAN_POINT('Ctrl Pts',(-66.,-15.7702454432537,1.09599839647648));
#59256=CARTESIAN_POINT('Ctrl Pts',(-50.,-15.7702454432537,1.09599839647648));
#59257=CARTESIAN_POINT('Ctrl Pts',(-66.,-15.8808661517589,1.14825710837788));
#59258=CARTESIAN_POINT('Ctrl Pts',(-50.,-15.8808661517589,1.14825710837788));
#59259=CARTESIAN_POINT('Ctrl Pts',(-66.,-15.9903135820168,1.19759548023257));
#59260=CARTESIAN_POINT('Ctrl Pts',(-50.,-15.9903135820168,1.19759548023257));
#59261=CARTESIAN_POINT('Ctrl Pts',(-66.,-16.0987879364791,1.2463210640833));
#59262=CARTESIAN_POINT('Ctrl Pts',(-50.,-16.0987879364791,1.2463210640833));
#59263=CARTESIAN_POINT('Ctrl Pts',(-66.,-16.2069202965129,1.30027898254334));
#59264=CARTESIAN_POINT('Ctrl Pts',(-50.,-16.2069202965129,1.30027898254334));
#59265=CARTESIAN_POINT('Ctrl Pts',(-66.,-16.3153998369687,1.36562590713335));
#59266=CARTESIAN_POINT('Ctrl Pts',(-50.,-16.3153998369687,1.36562590713335));
#59267=CARTESIAN_POINT('Ctrl Pts',(-66.,-16.424658248998,1.44607062429677));
#59268=CARTESIAN_POINT('Ctrl Pts',(-50.,-16.424658248998,1.44607062429677));
#59269=CARTESIAN_POINT('Ctrl Pts',(-66.,-16.5345463329789,1.54005835913147));
#59270=CARTESIAN_POINT('Ctrl Pts',(-50.,-16.5345463329789,1.54005835913147));
#59271=CARTESIAN_POINT('Ctrl Pts',(-66.,-16.6439703236082,1.63759217997151));
#59272=CARTESIAN_POINT('Ctrl Pts',(-50.,-16.6439703236082,1.63759217997151));
#59273=CARTESIAN_POINT('Ctrl Pts',(-66.,-16.751164098444,1.72267382202435));
#59274=CARTESIAN_POINT('Ctrl Pts',(-50.,-16.751164098444,1.72267382202435));
#59275=CARTESIAN_POINT('Ctrl Pts',(-66.,-16.8540367989194,1.77640986861434));
#59276=CARTESIAN_POINT('Ctrl Pts',(-50.,-16.8540367989194,1.77640986861434));
#59277=CARTESIAN_POINT('Ctrl Pts',(-66.,-16.9504681139093,1.77965278795706));
#59278=CARTESIAN_POINT('Ctrl Pts',(-50.,-16.9504681139093,1.77965278795706));
#59279=CARTESIAN_POINT('Ctrl Pts',(-66.,-17.0386813073781,1.71633428927379));
#59280=CARTESIAN_POINT('Ctrl Pts',(-50.,-17.0386813073781,1.71633428927379));
#59281=CARTESIAN_POINT('Ctrl Pts',(-66.,-17.1173432554706,1.57436164343055));
#59282=CARTESIAN_POINT('Ctrl Pts',(-50.,-17.1173432554706,1.57436164343055));
#59283=CARTESIAN_POINT('Ctrl Pts',(-66.,-17.1854641388117,1.34472480942369));
#59284=CARTESIAN_POINT('Ctrl Pts',(-50.,-17.1854641388117,1.34472480942369));
#59285=CARTESIAN_POINT('Ctrl Pts',(-66.,-17.2423578994913,1.02114561862921));
#59286=CARTESIAN_POINT('Ctrl Pts',(-50.,-17.2423578994913,1.02114561862921));
#59287=CARTESIAN_POINT('Ctrl Pts',(-66.,-17.2875806747963,0.599529862462145));
#59288=CARTESIAN_POINT('Ctrl Pts',(-50.,-17.2875806747963,0.599529862462145));
#59289=CARTESIAN_POINT('Ctrl Pts',(-66.,-17.3208814627092,0.0775281531615438));
#59290=CARTESIAN_POINT('Ctrl Pts',(-50.,-17.3208814627092,0.0775281531615438));
#59291=CARTESIAN_POINT('Ctrl Pts',(-66.,-17.3421500762616,-0.545927845218096));
#59292=CARTESIAN_POINT('Ctrl Pts',(-50.,-17.3421500762616,-0.545927845218096));
#59293=CARTESIAN_POINT('Ctrl Pts',(-66.,-17.3495248726512,-1.12603243333965));
#59294=CARTESIAN_POINT('Ctrl Pts',(-50.,-17.3495248726512,-1.12603243333965));
#59295=CARTESIAN_POINT('Ctrl Pts',(-66.,-17.3496452331689,-1.60677512854574));
#59296=CARTESIAN_POINT('Ctrl Pts',(-50.,-17.3496452331689,-1.60677512854574));
#59297=CARTESIAN_POINT('Ctrl Pts',(-66.,-17.3473238999477,-1.94753848896561));
#59298=CARTESIAN_POINT('Ctrl Pts',(-50.,-17.3473238999477,-1.94753848896561));
#59299=CARTESIAN_POINT('Ctrl Pts',(-66.,-17.345562839687,-2.12298722899376));
#59300=CARTESIAN_POINT('Ctrl Pts',(-50.,-17.345562839687,-2.12298722899376));
#59301=CARTESIAN_POINT('',(-65.5,-16.7854722368145,1.73595702341129));
#59302=CARTESIAN_POINT('Ctrl Pts',(-66.,-16.3175338509752,1.37066189203528));
#59303=CARTESIAN_POINT('Ctrl Pts',(-65.8729887704777,-16.4381764834115,
1.45180418206711));
#59304=CARTESIAN_POINT('Ctrl Pts',(-65.7718691849107,-16.5316964789852,
1.54005558503416));
#59305=CARTESIAN_POINT('Ctrl Pts',(-65.6164770304283,-16.675938104789,1.66211853613209));
#59306=CARTESIAN_POINT('Ctrl Pts',(-65.5625284355056,-16.7261279559211,
1.70187129664813));
#59307=CARTESIAN_POINT('Ctrl Pts',(-65.5076868273056,-16.7781614587951,
1.73192223528954));
#59308=CARTESIAN_POINT('Ctrl Pts',(-65.5038549844531,-16.7818026870438,
1.73396519020203));
#59309=CARTESIAN_POINT('Ctrl Pts',(-65.5,-16.7854722368145,1.73595702341129));
#59310=CARTESIAN_POINT('',(-66.,-14.045256078575,0.696195329812624));
#59311=CARTESIAN_POINT('',(-50.5,-16.7854722368145,1.73595702341129));
#59312=CARTESIAN_POINT('Ctrl Pts',(-50.5,-16.7854722368145,1.73595702341129));
#59313=CARTESIAN_POINT('Ctrl Pts',(-50.4675027013721,-16.754538141962,1.71916598329007));
#59314=CARTESIAN_POINT('Ctrl Pts',(-50.4339845147439,-16.7230774265929,
1.6973772200423));
#59315=CARTESIAN_POINT('Ctrl Pts',(-50.2820350749108,-16.5813058210333,
1.58823427035107));
#59316=CARTESIAN_POINT('Ctrl Pts',(-50.1596733333234,-16.4692008439998,
1.47267066694127));
#59317=CARTESIAN_POINT('Ctrl Pts',(-50.,-16.3175338509752,1.37066189203528));
#59318=CARTESIAN_POINT('Ctrl Pts',(-65.5,-16.7854722368145,1.73595702341129));
#59319=CARTESIAN_POINT('Ctrl Pts',(-60.5,-16.7854722368145,1.73595702341129));
#59320=CARTESIAN_POINT('Ctrl Pts',(-55.5,-16.7854722368145,1.73595702341129));
#59321=CARTESIAN_POINT('Ctrl Pts',(-50.5,-16.7854722368145,1.73595702341129));
#59322=CARTESIAN_POINT('Origin',(-66.,0.,0.));
#59323=CARTESIAN_POINT('',(-66.,-14.045256078575,-0.696195329812616));
#59324=CARTESIAN_POINT('Ctrl Pts',(-66.,-17.345562839687,-2.12298722899376));
#59325=CARTESIAN_POINT('Ctrl Pts',(-50.,-17.345562839687,-2.12298722899376));
#59326=CARTESIAN_POINT('Ctrl Pts',(-66.,-17.3282886320894,-2.10855557872225));
#59327=CARTESIAN_POINT('Ctrl Pts',(-50.,-17.3282886320894,-2.10855557872225));
#59328=CARTESIAN_POINT('Ctrl Pts',(-66.,-17.2936892204412,-2.07983106708238));
#59329=CARTESIAN_POINT('Ctrl Pts',(-50.,-17.2936892204412,-2.07983106708238));
#59330=CARTESIAN_POINT('Ctrl Pts',(-66.,-17.241637113787,-2.03716066567899));
#59331=CARTESIAN_POINT('Ctrl Pts',(-50.,-17.241637113787,-2.03716066567899));
#59332=CARTESIAN_POINT('Ctrl Pts',(-66.,-17.1719279181019,-1.98110064232955));
#59333=CARTESIAN_POINT('Ctrl Pts',(-50.,-17.1719279181019,-1.98110064232955));
#59334=CARTESIAN_POINT('Ctrl Pts',(-66.,-17.0842789796692,-1.91242115216328));
#59335=CARTESIAN_POINT('Ctrl Pts',(-50.,-17.0842789796692,-1.91242115216328));
#59336=CARTESIAN_POINT('Ctrl Pts',(-66.,-16.9961162868454,-1.84514350065724));
#59337=CARTESIAN_POINT('Ctrl Pts',(-50.,-16.9961162868454,-1.84514350065724));
#59338=CARTESIAN_POINT('Ctrl Pts',(-66.,-16.9074403974186,-1.77927159805394));
#59339=CARTESIAN_POINT('Ctrl Pts',(-50.,-16.9074403974186,-1.77927159805394));
#59340=CARTESIAN_POINT('Ctrl Pts',(-66.,-16.8182550149921,-1.71480453952538));
#59341=CARTESIAN_POINT('Ctrl Pts',(-50.,-16.8182550149921,-1.71480453952538));
#59342=CARTESIAN_POINT('Ctrl Pts',(-66.,-16.7285687128188,-1.65173252825902));
#59343=CARTESIAN_POINT('Ctrl Pts',(-50.,-16.7285687128188,-1.65173252825902));
#59344=CARTESIAN_POINT('Ctrl Pts',(-66.,-16.6383931283473,-1.59004626593597));
#59345=CARTESIAN_POINT('Ctrl Pts',(-50.,-16.6383931283473,-1.59004626593597));
#59346=CARTESIAN_POINT('Ctrl Pts',(-66.,-16.5477407361381,-1.52974779117622));
#59347=CARTESIAN_POINT('Ctrl Pts',(-50.,-16.5477407361381,-1.52974779117622));
#59348=CARTESIAN_POINT('Ctrl Pts',(-66.,-16.456622719418,-1.4708615729337));
#59349=CARTESIAN_POINT('Ctrl Pts',(-50.,-16.456622719418,-1.4708615729337));
#59350=CARTESIAN_POINT('Ctrl Pts',(-66.,-16.3650471090276,-1.41344345684179));
#59351=CARTESIAN_POINT('Ctrl Pts',(-50.,-16.3650471090276,-1.41344345684179));
#59352=CARTESIAN_POINT('Ctrl Pts',(-66.,-16.2730161904774,-1.35759562886537));
#59353=CARTESIAN_POINT('Ctrl Pts',(-50.,-16.2730161904774,-1.35759562886537));
#59354=CARTESIAN_POINT('Ctrl Pts',(-66.,-16.1805287542786,-1.30344437937201));
#59355=CARTESIAN_POINT('Ctrl Pts',(-50.,-16.1805287542786,-1.30344437937201));
#59356=CARTESIAN_POINT('Ctrl Pts',(-66.,-16.0875836011606,-1.25110870320843));
#59357=CARTESIAN_POINT('Ctrl Pts',(-50.,-16.0875836011606,-1.25110870320843));
#59358=CARTESIAN_POINT('Ctrl Pts',(-66.,-15.9941829293225,-1.20066922344171));
#59359=CARTESIAN_POINT('Ctrl Pts',(-50.,-15.9941829293225,-1.20066922344171));
#59360=CARTESIAN_POINT('Ctrl Pts',(-66.,-15.900335256791,-1.15214240747963));
#59361=CARTESIAN_POINT('Ctrl Pts',(-50.,-15.900335256791,-1.15214240747963));
#59362=CARTESIAN_POINT('Ctrl Pts',(-66.,-15.8060601113054,-1.10543718159424));
#59363=CARTESIAN_POINT('Ctrl Pts',(-50.,-15.8060601113054,-1.10543718159424));
#59364=CARTESIAN_POINT('Ctrl Pts',(-66.,-15.7113832084608,-1.06040669143688));
#59365=CARTESIAN_POINT('Ctrl Pts',(-50.,-15.7113832084608,-1.06040669143688));
#59366=CARTESIAN_POINT('Ctrl Pts',(-66.,-15.6163284960372,-1.01693147636119));
#59367=CARTESIAN_POINT('Ctrl Pts',(-50.,-15.6163284960372,-1.01693147636119));
#59368=CARTESIAN_POINT('Ctrl Pts',(-66.,-15.5209107672782,-0.974997271170846));
#59369=CARTESIAN_POINT('Ctrl Pts',(-50.,-15.5209107672782,-0.974997271170846));
#59370=CARTESIAN_POINT('Ctrl Pts',(-66.,-15.4251291786488,-0.934763901846662));
#59371=CARTESIAN_POINT('Ctrl Pts',(-50.,-15.4251291786488,-0.934763901846662));
#59372=CARTESIAN_POINT('Ctrl Pts',(-66.,-15.3289574472276,-0.89666784595261));
#59373=CARTESIAN_POINT('Ctrl Pts',(-50.,-15.3289574472276,-0.89666784595261));
#59374=CARTESIAN_POINT('Ctrl Pts',(-66.,-15.2323530329047,-0.861333854256595));
#59375=CARTESIAN_POINT('Ctrl Pts',(-50.,-15.2323530329047,-0.861333854256595));
#59376=CARTESIAN_POINT('Ctrl Pts',(-66.,-15.1352727230412,-0.829421964594113));
#59377=CARTESIAN_POINT('Ctrl Pts',(-50.,-15.1352727230412,-0.829421964594113));
#59378=CARTESIAN_POINT('Ctrl Pts',(-66.,-15.0376867393704,-0.801490439086723));
#59379=CARTESIAN_POINT('Ctrl Pts',(-50.,-15.0376867393704,-0.801490439086723));
#59380=CARTESIAN_POINT('Ctrl Pts',(-66.,-14.939592201905,-0.777863584450799));
#59381=CARTESIAN_POINT('Ctrl Pts',(-50.,-14.939592201905,-0.777863584450799));
#59382=CARTESIAN_POINT('Ctrl Pts',(-66.,-14.8410305914479,-0.758464226728878));
#59383=CARTESIAN_POINT('Ctrl Pts',(-50.,-14.8410305914479,-0.758464226728878));
#59384=CARTESIAN_POINT('Ctrl Pts',(-66.,-14.7420779497362,-0.742890629132665));
#59385=CARTESIAN_POINT('Ctrl Pts',(-50.,-14.7420779497362,-0.742890629132665));
#59386=CARTESIAN_POINT('Ctrl Pts',(-66.,-14.6428281112089,-0.730556131457601));
#59387=CARTESIAN_POINT('Ctrl Pts',(-50.,-14.6428281112089,-0.730556131457601));
#59388=CARTESIAN_POINT('Ctrl Pts',(-66.,-14.5433782125866,-0.72080782010221));
#59389=CARTESIAN_POINT('Ctrl Pts',(-50.,-14.5433782125866,-0.72080782010221));
#59390=CARTESIAN_POINT('Ctrl Pts',(-66.,-14.4438139036356,-0.71304855704325));
#59391=CARTESIAN_POINT('Ctrl Pts',(-50.,-14.4438139036356,-0.71304855704325));
#59392=CARTESIAN_POINT('Ctrl Pts',(-66.,-14.3441931446757,-0.706869197330954));
#59393=CARTESIAN_POINT('Ctrl Pts',(-50.,-14.3441931446757,-0.706869197330954));
#59394=CARTESIAN_POINT('Ctrl Pts',(-66.,-14.2445503001281,-0.702023483575367));
#59395=CARTESIAN_POINT('Ctrl Pts',(-50.,-14.2445503001281,-0.702023483575367));
#59396=CARTESIAN_POINT('Ctrl Pts',(-66.,-14.1648321695468,-0.699111910780302));
#59397=CARTESIAN_POINT('Ctrl Pts',(-50.,-14.1648321695468,-0.699111910780302));
#59398=CARTESIAN_POINT('Ctrl Pts',(-66.,-14.1050439680336,-0.697450717395246));
#59399=CARTESIAN_POINT('Ctrl Pts',(-50.,-14.1050439680336,-0.697450717395246));
#59400=CARTESIAN_POINT('Ctrl Pts',(-66.,-14.0651853454231,-0.696575143525857));
#59401=CARTESIAN_POINT('Ctrl Pts',(-50.,-14.0651853454231,-0.696575143525857));
#59402=CARTESIAN_POINT('Ctrl Pts',(-66.,-14.045256078575,-0.696195329812629));
#59403=CARTESIAN_POINT('Ctrl Pts',(-50.,-14.045256078575,-0.696195329812629));
#59404=CARTESIAN_POINT('Origin',(-65.75,0.,0.));
#59405=CARTESIAN_POINT('',(-65.5,-16.6837004856932,2.53372514367283));
#59406=CARTESIAN_POINT('Origin',(-65.5,0.,0.));
#59407=CARTESIAN_POINT('Ctrl Pts',(-65.5,-16.6837004857171,2.53372514366373));
#59408=CARTESIAN_POINT('Ctrl Pts',(-65.5738810032737,-16.6043913553664,
2.56393691646143));
#59409=CARTESIAN_POINT('Ctrl Pts',(-65.647826758183,-16.5250605133332,2.59279124243202));
#59410=CARTESIAN_POINT('Ctrl Pts',(-65.7215770308288,-16.4460101931368,
2.6202092323328));
#59411=CARTESIAN_POINT('Ctrl Pts',(-65.7821649037802,-16.3810681856701,
2.64273386348462));
#59412=CARTESIAN_POINT('Ctrl Pts',(-65.842620844317,-16.3163158245858,2.6642910002248));
#59413=CARTESIAN_POINT('Ctrl Pts',(-65.9028005644781,-16.2519319156941,
2.68479258877889));
#59414=CARTESIAN_POINT('Ctrl Pts',(-65.935288443709,-16.2171744151459,2.6958603227465));
#59415=CARTESIAN_POINT('Ctrl Pts',(-65.967695822527,-16.1825245252962,2.70661906026748));
#59416=CARTESIAN_POINT('Ctrl Pts',(-66.,-16.1480113642792,2.71704876274038));
#59417=CARTESIAN_POINT('Origin',(-58.,0.,0.));
#59418=CARTESIAN_POINT('',(-50.5,-16.6837004856932,2.53372514367283));
#59419=CARTESIAN_POINT('Origin',(-50.5,0.,0.));
#59420=CARTESIAN_POINT('Ctrl Pts',(-50.5,-16.6837004856932,2.53372514367283));
#59421=CARTESIAN_POINT('Ctrl Pts',(-55.5,-16.6837004856932,2.53372514367283));
#59422=CARTESIAN_POINT('Ctrl Pts',(-60.5,-16.6837004856932,2.53372514367283));
#59423=CARTESIAN_POINT('Ctrl Pts',(-65.5,-16.6837004856932,2.53372514367283));
#59424=CARTESIAN_POINT('Origin',(-50.25,0.,0.));
#59425=CARTESIAN_POINT('Ctrl Pts',(-50.,-16.1480113642792,2.71704876274038));
#59426=CARTESIAN_POINT('Ctrl Pts',(-50.0601511103782,-16.2122756520658,
2.69762842042758));
#59427=CARTESIAN_POINT('Ctrl Pts',(-50.1206600330683,-16.2770136258072,
2.6770696979896));
#59428=CARTESIAN_POINT('Ctrl Pts',(-50.1813802137674,-16.3420386981439,
2.65549281295864));
#59429=CARTESIAN_POINT('Ctrl Pts',(-50.2450302523274,-16.4102013471008,
2.63287480444134));
#59430=CARTESIAN_POINT('Ctrl Pts',(-50.3089124279122,-16.4786791569631,
2.60913798457234));
#59431=CARTESIAN_POINT('Ctrl Pts',(-50.3728579315898,-16.5472689407516,
2.58435539231395));
#59432=CARTESIAN_POINT('Ctrl Pts',(-50.4152271869693,-16.5927154209358,
2.56793484794457));
#59433=CARTESIAN_POINT('Ctrl Pts',(-50.4576242444773,-16.638211331949,2.55105364004647));
#59434=CARTESIAN_POINT('Ctrl Pts',(-50.5,-16.6837004857171,2.53372514366373));
#59435=CARTESIAN_POINT('Ctrl Pts',(-66.,-13.4308617934315,4.1672362226952));
#59436=CARTESIAN_POINT('Ctrl Pts',(-50.,-13.4308617934315,4.1672362226952));
#59437=CARTESIAN_POINT('Ctrl Pts',(-66.,-13.4534498353221,4.1732391209285));
#59438=CARTESIAN_POINT('Ctrl Pts',(-50.,-13.4534498353221,4.1732391209285));
#59439=CARTESIAN_POINT('Ctrl Pts',(-66.,-13.4985769550718,4.18546462196559));
#59440=CARTESIAN_POINT('Ctrl Pts',(-50.,-13.4985769550718,4.18546462196559));
#59441=CARTESIAN_POINT('Ctrl Pts',(-66.,-13.5661207520894,4.20446197782756));
#59442=CARTESIAN_POINT('Ctrl Pts',(-50.,-13.5661207520894,4.20446197782756));
#59443=CARTESIAN_POINT('Ctrl Pts',(-66.,-13.655884910321,4.23111182833087));
#59444=CARTESIAN_POINT('Ctrl Pts',(-50.,-13.655884910321,4.23111182833087));
#59445=CARTESIAN_POINT('Ctrl Pts',(-66.,-13.7675695531958,4.26667263583206));
#59446=CARTESIAN_POINT('Ctrl Pts',(-50.,-13.7675695531958,4.26667263583206));
#59447=CARTESIAN_POINT('Ctrl Pts',(-66.,-13.8786454687203,4.30461115967259));
#59448=CARTESIAN_POINT('Ctrl Pts',(-50.,-13.8786454687203,4.30461115967259));
#59449=CARTESIAN_POINT('Ctrl Pts',(-66.,-13.988941714333,4.34517014494338));
#59450=CARTESIAN_POINT('Ctrl Pts',(-50.,-13.988941714333,4.34517014494338));
#59451=CARTESIAN_POINT('Ctrl Pts',(-66.,-14.0981684916428,4.38874946735859));
#59452=CARTESIAN_POINT('Ctrl Pts',(-50.,-14.0981684916428,4.38874946735859));
#59453=CARTESIAN_POINT('Ctrl Pts',(-66.,-14.2059737915295,4.4358697529125));
#59454=CARTESIAN_POINT('Ctrl Pts',(-50.,-14.2059737915295,4.4358697529125));
#59455=CARTESIAN_POINT('Ctrl Pts',(-66.,-14.3120199719745,4.48712764234399));
#59456=CARTESIAN_POINT('Ctrl Pts',(-50.,-14.3120199719745,4.48712764234399));
#59457=CARTESIAN_POINT('Ctrl Pts',(-66.,-14.4160475830522,4.54314296997813));
#59458=CARTESIAN_POINT('Ctrl Pts',(-50.,-14.4160475830522,4.54314296997813));
#59459=CARTESIAN_POINT('Ctrl Pts',(-66.,-14.5179595646104,4.60453676010005));
#59460=CARTESIAN_POINT('Ctrl Pts',(-50.,-14.5179595646104,4.60453676010005));
#59461=CARTESIAN_POINT('Ctrl Pts',(-66.,-14.6178234390918,4.67173377183878));
#59462=CARTESIAN_POINT('Ctrl Pts',(-50.,-14.6178234390918,4.67173377183878));
#59463=CARTESIAN_POINT('Ctrl Pts',(-66.,-14.7158387764281,4.74463077904808));
#59464=CARTESIAN_POINT('Ctrl Pts',(-50.,-14.7158387764281,4.74463077904808));
#59465=CARTESIAN_POINT('Ctrl Pts',(-66.,-14.8123108082616,4.82238412668293));
#59466=CARTESIAN_POINT('Ctrl Pts',(-50.,-14.8123108082616,4.82238412668293));
#59467=CARTESIAN_POINT('Ctrl Pts',(-66.,-14.9076357442716,4.90295634303817));
#59468=CARTESIAN_POINT('Ctrl Pts',(-50.,-14.9076357442716,4.90295634303817));
#59469=CARTESIAN_POINT('Ctrl Pts',(-66.,-15.0022304656484,4.98346615129592));
#59470=CARTESIAN_POINT('Ctrl Pts',(-50.,-15.0022304656484,4.98346615129592));
#59471=CARTESIAN_POINT('Ctrl Pts',(-66.,-15.0963796080126,5.06159331118216));
#59472=CARTESIAN_POINT('Ctrl Pts',(-50.,-15.0963796080126,5.06159331118216));
#59473=CARTESIAN_POINT('Ctrl Pts',(-66.,-15.1901185918597,5.13660009643943));
#59474=CARTESIAN_POINT('Ctrl Pts',(-50.,-15.1901185918597,5.13660009643943));
#59475=CARTESIAN_POINT('Ctrl Pts',(-66.,-15.2830674650563,5.2107713514449));
#59476=CARTESIAN_POINT('Ctrl Pts',(-50.,-15.2830674650563,5.2107713514449));
#59477=CARTESIAN_POINT('Ctrl Pts',(-66.,-15.3743838595047,5.28992550709052));
#59478=CARTESIAN_POINT('Ctrl Pts',(-50.,-15.3743838595047,5.28992550709052));
#59479=CARTESIAN_POINT('Ctrl Pts',(-66.,-15.4632041964143,5.3801972025556));
#59480=CARTESIAN_POINT('Ctrl Pts',(-50.,-15.4632041964143,5.3801972025556));
#59481=CARTESIAN_POINT('Ctrl Pts',(-66.,-15.5490242668831,5.48528606316123));
#59482=CARTESIAN_POINT('Ctrl Pts',(-50.,-15.5490242668831,5.48528606316123));
#59483=CARTESIAN_POINT('Ctrl Pts',(-66.,-15.6320862154648,5.6036490556807));
#59484=CARTESIAN_POINT('Ctrl Pts',(-50.,-15.6320862154648,5.6036490556807));
#59485=CARTESIAN_POINT('Ctrl Pts',(-66.,-15.7138167753124,5.72533131206965));
#59486=CARTESIAN_POINT('Ctrl Pts',(-50.,-15.7138167753124,5.72533131206965));
#59487=CARTESIAN_POINT('Ctrl Pts',(-66.,-15.7964839166342,5.83439796565188));
#59488=CARTESIAN_POINT('Ctrl Pts',(-50.,-15.7964839166342,5.83439796565188));
#59489=CARTESIAN_POINT('Ctrl Pts',(-66.,-15.8827610706914,5.91202919579815));
#59490=CARTESIAN_POINT('Ctrl Pts',(-50.,-15.8827610706914,5.91202919579815));
#59491=CARTESIAN_POINT('Ctrl Pts',(-66.,-15.9753563373507,5.9391517257104));
#59492=CARTESIAN_POINT('Ctrl Pts',(-50.,-15.9753563373507,5.9391517257104));
#59493=CARTESIAN_POINT('Ctrl Pts',(-66.,-16.0765448214269,5.89976022322805));
#59494=CARTESIAN_POINT('Ctrl Pts',(-50.,-16.0765448214269,5.89976022322805));
#59495=CARTESIAN_POINT('Ctrl Pts',(-66.,-16.1880426210461,5.78181034011869));
#59496=CARTESIAN_POINT('Ctrl Pts',(-50.,-16.1880426210461,5.78181034011869));
#59497=CARTESIAN_POINT('Ctrl Pts',(-66.,-16.3111317199096,5.57632894431644));
#59498=CARTESIAN_POINT('Ctrl Pts',(-50.,-16.3111317199096,5.57632894431644));
#59499=CARTESIAN_POINT('Ctrl Pts',(-66.,-16.4467089309247,5.27706449174507));
#59500=CARTESIAN_POINT('Ctrl Pts',(-50.,-16.4467089309247,5.27706449174507));
#59501=CARTESIAN_POINT('Ctrl Pts',(-66.,-16.5953625244127,4.879941016743));
#59502=CARTESIAN_POINT('Ctrl Pts',(-50.,-16.5953625244127,4.879941016743));
#59503=CARTESIAN_POINT('Ctrl Pts',(-66.,-16.7574336530234,4.38262052022265));
#59504=CARTESIAN_POINT('Ctrl Pts',(-50.,-16.7574336530234,4.38262052022265));
#59505=CARTESIAN_POINT('Ctrl Pts',(-66.,-16.93308127586,3.78404082759198));
#59506=CARTESIAN_POINT('Ctrl Pts',(-50.,-16.93308127586,3.78404082759198));
#59507=CARTESIAN_POINT('Ctrl Pts',(-66.,-17.0844905240235,3.22399532912598));
#59508=CARTESIAN_POINT('Ctrl Pts',(-50.,-17.0844905240235,3.22399532912598));
#59509=CARTESIAN_POINT('Ctrl Pts',(-66.,-17.2041629498203,2.75838598215733));
#59510=CARTESIAN_POINT('Ctrl Pts',(-50.,-17.2041629498203,2.75838598215733));
#59511=CARTESIAN_POINT('Ctrl Pts',(-66.,-17.2866589472037,2.4277510372282));
#59512=CARTESIAN_POINT('Ctrl Pts',(-50.,-17.2866589472037,2.4277510372282));
#59513=CARTESIAN_POINT('Ctrl Pts',(-66.,-17.3285855412502,2.25737638411816));
#59514=CARTESIAN_POINT('Ctrl Pts',(-50.,-17.3285855412502,2.25737638411816));
#59515=CARTESIAN_POINT('',(-65.5,-15.8264108038954,5.85579593790134));
#59516=CARTESIAN_POINT('Ctrl Pts',(-66.,-15.4640187679296,5.38560568043381));
#59517=CARTESIAN_POINT('Ctrl Pts',(-65.7933280154035,-15.6213248025723,
5.56231194751196));
#59518=CARTESIAN_POINT('Ctrl Pts',(-65.637076174949,-15.7176413861457,5.75474546238425));
#59519=CARTESIAN_POINT('Ctrl Pts',(-65.5,-15.8264108038954,5.85579593790134));
#59520=CARTESIAN_POINT('',(-66.,-13.4308617934315,4.1672362226952));
#59521=CARTESIAN_POINT('',(-50.5,-15.8264108038954,5.85579593790134));
#59522=CARTESIAN_POINT('Ctrl Pts',(-50.5,-15.8264108038954,5.85579593790134));
#59523=CARTESIAN_POINT('Ctrl Pts',(-50.4432204291973,-15.7813564327869,
5.81393890015279));
#59524=CARTESIAN_POINT('Ctrl Pts',(-50.3822807385572,-15.7377169583822,
5.75610061597894));
#59525=CARTESIAN_POINT('Ctrl Pts',(-50.2209130984549,-15.6244042480767,
5.59526303189522));
#59526=CARTESIAN_POINT('Ctrl Pts',(-50.1226480777072,-15.5573709598018,
5.49047080774294));
#59527=CARTESIAN_POINT('Ctrl Pts',(-50.,-15.4640187679296,5.38560568043381));
#59528=CARTESIAN_POINT('Ctrl Pts',(-65.5,-15.8264108038954,5.85579593790135));
#59529=CARTESIAN_POINT('Ctrl Pts',(-60.5,-15.8264108038954,5.85579593790135));
#59530=CARTESIAN_POINT('Ctrl Pts',(-55.5,-15.8264108038954,5.85579593790135));
#59531=CARTESIAN_POINT('Ctrl Pts',(-50.5,-15.8264108038954,5.85579593790135));
#59532=CARTESIAN_POINT('Origin',(-66.,0.,0.));
#59533=CARTESIAN_POINT('',(-66.,-13.7771352694631,2.8185900760694));
#59534=CARTESIAN_POINT('Ctrl Pts',(-66.,-17.3285855412502,2.25737638411816));
#59535=CARTESIAN_POINT('Ctrl Pts',(-50.,-17.3285855412502,2.25737638411816));
#59536=CARTESIAN_POINT('Ctrl Pts',(-66.,-17.3082650291717,2.26705871682014));
#59537=CARTESIAN_POINT('Ctrl Pts',(-50.,-17.3082650291717,2.26705871682014));
#59538=CARTESIAN_POINT('Ctrl Pts',(-66.,-17.2676091261057,2.28627627132739));
#59539=CARTESIAN_POINT('Ctrl Pts',(-50.,-17.2676091261057,2.28627627132739));
#59540=CARTESIAN_POINT('Ctrl Pts',(-66.,-17.2065806347889,2.31466127107479));
#59541=CARTESIAN_POINT('Ctrl Pts',(-50.,-17.2065806347889,2.31466127107479));
#59542=CARTESIAN_POINT('Ctrl Pts',(-66.,-17.1251199207912,2.35162409369425));
#59543=CARTESIAN_POINT('Ctrl Pts',(-50.,-17.1251199207912,2.35162409369425));
#59544=CARTESIAN_POINT('Ctrl Pts',(-66.,-17.0231447402746,2.39634848677526));
#59545=CARTESIAN_POINT('Ctrl Pts',(-50.,-17.0231447402746,2.39634848677526));
#59546=CARTESIAN_POINT('Ctrl Pts',(-66.,-16.921020569004,2.4395873170138));
#59547=CARTESIAN_POINT('Ctrl Pts',(-50.,-16.921020569004,2.4395873170138));
#59548=CARTESIAN_POINT('Ctrl Pts',(-66.,-16.8187489196813,2.48133693573106));
#59549=CARTESIAN_POINT('Ctrl Pts',(-50.,-16.8187489196813,2.48133693573106));
#59550=CARTESIAN_POINT('Ctrl Pts',(-66.,-16.7163331545329,2.52159914037693));
#59551=CARTESIAN_POINT('Ctrl Pts',(-50.,-16.7163331545329,2.52159914037693));
#59552=CARTESIAN_POINT('Ctrl Pts',(-66.,-16.6137791410988,2.56038555206031));
#59553=CARTESIAN_POINT('Ctrl Pts',(-50.,-16.6137791410988,2.56038555206031));
#59554=CARTESIAN_POINT('Ctrl Pts',(-66.,-16.511095838818,2.59770807109214));
#59555=CARTESIAN_POINT('Ctrl Pts',(-50.,-16.511095838818,2.59770807109214));
#59556=CARTESIAN_POINT('Ctrl Pts',(-66.,-16.408295837324,2.63356782519645));
#59557=CARTESIAN_POINT('Ctrl Pts',(-50.,-16.408295837324,2.63356782519645));
#59558=CARTESIAN_POINT('Ctrl Pts',(-66.,-16.3053960536831,2.66794389531189));
#59559=CARTESIAN_POINT('Ctrl Pts',(-50.,-16.3053960536831,2.66794389531189));
#59560=CARTESIAN_POINT('Ctrl Pts',(-66.,-16.2024181546768,2.70078418748721));
#59561=CARTESIAN_POINT('Ctrl Pts',(-50.,-16.2024181546768,2.70078418748721));
#59562=CARTESIAN_POINT('Ctrl Pts',(-66.,-16.099389766628,2.73199029450084));
#59563=CARTESIAN_POINT('Ctrl Pts',(-50.,-16.099389766628,2.73199029450084));
#59564=CARTESIAN_POINT('Ctrl Pts',(-66.,-15.9963411251835,2.76143959284173));
#59565=CARTESIAN_POINT('Ctrl Pts',(-50.,-15.9963411251835,2.76143959284173));
#59566=CARTESIAN_POINT('Ctrl Pts',(-66.,-15.8933006615651,2.78901652785862));
#59567=CARTESIAN_POINT('Ctrl Pts',(-50.,-15.8933006615651,2.78901652785862));
#59568=CARTESIAN_POINT('Ctrl Pts',(-66.,-15.7902905550528,2.81464355607623));
#59569=CARTESIAN_POINT('Ctrl Pts',(-50.,-15.7902905550528,2.81464355607623));
#59570=CARTESIAN_POINT('Ctrl Pts',(-66.,-15.6873231513416,2.83830684578773));
#59571=CARTESIAN_POINT('Ctrl Pts',(-50.,-15.6873231513416,2.83830684578773));
#59572=CARTESIAN_POINT('Ctrl Pts',(-66.,-15.5843947155558,2.86009946582377));
#59573=CARTESIAN_POINT('Ctrl Pts',(-50.,-15.5843947155558,2.86009946582377));
#59574=CARTESIAN_POINT('Ctrl Pts',(-66.,-15.4814936341966,2.88017005204204));
#59575=CARTESIAN_POINT('Ctrl Pts',(-50.,-15.4814936341966,2.88017005204204));
#59576=CARTESIAN_POINT('Ctrl Pts',(-66.,-15.3786133940255,2.89864026758367));
#59577=CARTESIAN_POINT('Ctrl Pts',(-50.,-15.3786133940255,2.89864026758367));
#59578=CARTESIAN_POINT('Ctrl Pts',(-66.,-15.2757647759192,2.91552760840775));
#59579=CARTESIAN_POINT('Ctrl Pts',(-50.,-15.2757647759192,2.91552760840775));
#59580=CARTESIAN_POINT('Ctrl Pts',(-66.,-15.1729867099492,2.9306770599819));
#59581=CARTESIAN_POINT('Ctrl Pts',(-50.,-15.1729867099492,2.9306770599819));
#59582=CARTESIAN_POINT('Ctrl Pts',(-66.,-15.0703622864763,2.94365932119071));
#59583=CARTESIAN_POINT('Ctrl Pts',(-50.,-15.0703622864763,2.94365932119071));
#59584=CARTESIAN_POINT('Ctrl Pts',(-66.,-14.9680056710645,2.95385868966535));
#59585=CARTESIAN_POINT('Ctrl Pts',(-50.,-14.9680056710645,2.95385868966535));
#59586=CARTESIAN_POINT('Ctrl Pts',(-66.,-14.8660391534142,2.96062511732634));
#59587=CARTESIAN_POINT('Ctrl Pts',(-50.,-14.8660391534142,2.96062511732634));
#59588=CARTESIAN_POINT('Ctrl Pts',(-66.,-14.7645727249416,2.96341047532946));
#59589=CARTESIAN_POINT('Ctrl Pts',(-50.,-14.7645727249416,2.96341047532946));
#59590=CARTESIAN_POINT('Ctrl Pts',(-66.,-14.6636842479405,2.96189992942649));
#59591=CARTESIAN_POINT('Ctrl Pts',(-50.,-14.6636842479405,2.96189992942649));
#59592=CARTESIAN_POINT('Ctrl Pts',(-66.,-14.5633947076351,2.95617854486928));
#59593=CARTESIAN_POINT('Ctrl Pts',(-50.,-14.5633947076351,2.95617854486928));
#59594=CARTESIAN_POINT('Ctrl Pts',(-66.,-14.463677848895,2.94665434795724));
#59595=CARTESIAN_POINT('Ctrl Pts',(-50.,-14.463677848895,2.94665434795724));
#59596=CARTESIAN_POINT('Ctrl Pts',(-66.,-14.3644786617177,2.93391890356181));
#59597=CARTESIAN_POINT('Ctrl Pts',(-50.,-14.3644786617177,2.93391890356181));
#59598=CARTESIAN_POINT('Ctrl Pts',(-66.,-14.2657288580852,2.91862876972314));
#59599=CARTESIAN_POINT('Ctrl Pts',(-50.,-14.2657288580852,2.91862876972314));
#59600=CARTESIAN_POINT('Ctrl Pts',(-66.,-14.1673628947312,2.90138362450613));
#59601=CARTESIAN_POINT('Ctrl Pts',(-50.,-14.1673628947312,2.90138362450613));
#59602=CARTESIAN_POINT('Ctrl Pts',(-66.,-14.0693351608341,2.882594172965));
#59603=CARTESIAN_POINT('Ctrl Pts',(-50.,-14.0693351608341,2.882594172965));
#59604=CARTESIAN_POINT('Ctrl Pts',(-66.,-13.9716176994713,2.862507481945));
#59605=CARTESIAN_POINT('Ctrl Pts',(-50.,-13.9716176994713,2.862507481945));
#59606=CARTESIAN_POINT('Ctrl Pts',(-66.,-13.8936799818437,2.84550248942744));
#59607=CARTESIAN_POINT('Ctrl Pts',(-50.,-13.8936799818437,2.84550248942744));
#59608=CARTESIAN_POINT('Ctrl Pts',(-66.,-13.8353570146283,2.83224277227946));
#59609=CARTESIAN_POINT('Ctrl Pts',(-50.,-13.8353570146283,2.83224277227946));
#59610=CARTESIAN_POINT('Ctrl Pts',(-66.,-13.7965328775753,2.82317840202614));
#59611=CARTESIAN_POINT('Ctrl Pts',(-50.,-13.7965328775753,2.82317840202614));
#59612=CARTESIAN_POINT('Ctrl Pts',(-66.,-13.7771352694631,2.81859007606939));
#59613=CARTESIAN_POINT('Ctrl Pts',(-50.,-13.7771352694631,2.81859007606939));
#59614=CARTESIAN_POINT('Origin',(-65.75,0.,0.));
#59615=CARTESIAN_POINT('',(-65.5,-15.5294395356693,6.60319110036901));
#59616=CARTESIAN_POINT('Origin',(-65.5,0.,0.));
#59617=CARTESIAN_POINT('Ctrl Pts',(-65.5,-15.5294395356693,6.60319110036901));
#59618=CARTESIAN_POINT('Ctrl Pts',(-65.6931595476704,-15.308937883882,6.62813354100189));
#59619=CARTESIAN_POINT('Ctrl Pts',(-65.8611256967045,-15.1198491095487,
6.6410048580703));
#59620=CARTESIAN_POINT('Ctrl Pts',(-66.,-14.9649893429273,6.64753480367511));
#59621=CARTESIAN_POINT('Origin',(-58.,0.,0.));
#59622=CARTESIAN_POINT('',(-50.5,-15.5294395356693,6.60319110036901));
#59623=CARTESIAN_POINT('Origin',(-50.5,0.,0.));
#59624=CARTESIAN_POINT('Ctrl Pts',(-50.5,-15.5294395356693,6.60319110036901));
#59625=CARTESIAN_POINT('Ctrl Pts',(-55.5,-15.5294395356693,6.60319110036901));
#59626=CARTESIAN_POINT('Ctrl Pts',(-60.5,-15.5294395356693,6.60319110036901));
#59627=CARTESIAN_POINT('Ctrl Pts',(-65.5,-15.5294395356693,6.60319110036901));
#59628=CARTESIAN_POINT('Origin',(-50.25,0.,0.));
#59629=CARTESIAN_POINT('Ctrl Pts',(-50.,-14.9649893429273,6.64753480367511));
#59630=CARTESIAN_POINT('Ctrl Pts',(-50.1388743032925,-15.1198491095454,
6.64100485807044));
#59631=CARTESIAN_POINT('Ctrl Pts',(-50.3068404523269,-15.3089378838789,
6.62813354100223));
#59632=CARTESIAN_POINT('Ctrl Pts',(-50.5,-15.5294395356693,6.60319110036901));
#59633=CARTESIAN_POINT('Ctrl Pts',(-66.,-11.9725570665522,7.37643433768309));
#59634=CARTESIAN_POINT('Ctrl Pts',(-50.,-11.9725570665522,7.37643433768309));
#59635=CARTESIAN_POINT('Ctrl Pts',(-66.,-11.9929426034861,7.38786606141889));
#59636=CARTESIAN_POINT('Ctrl Pts',(-50.,-11.9929426034861,7.38786606141889));
#59637=CARTESIAN_POINT('Ctrl Pts',(-66.,-12.0336116133124,7.4109301341784));
#59638=CARTESIAN_POINT('Ctrl Pts',(-50.,-12.0336116133124,7.4109301341784));
#59639=CARTESIAN_POINT('Ctrl Pts',(-66.,-12.0943089474566,7.44612811243127));
#59640=CARTESIAN_POINT('Ctrl Pts',(-50.,-12.0943089474566,7.44612811243127));
#59641=CARTESIAN_POINT('Ctrl Pts',(-66.,-12.174625451278,7.49426414725743));
#59642=CARTESIAN_POINT('Ctrl Pts',(-50.,-12.174625451278,7.49426414725743));
#59643=CARTESIAN_POINT('Ctrl Pts',(-66.,-12.2739577025182,7.5564825878338));
#59644=CARTESIAN_POINT('Ctrl Pts',(-50.,-12.2739577025182,7.5564825878338));
#59645=CARTESIAN_POINT('Ctrl Pts',(-66.,-12.3721090366891,7.62085266008235));
#59646=CARTESIAN_POINT('Ctrl Pts',(-50.,-12.3721090366891,7.62085266008235));
#59647=CARTESIAN_POINT('Ctrl Pts',(-66.,-12.4688535134548,7.68756697112423));
#59648=CARTESIAN_POINT('Ctrl Pts',(-50.,-12.4688535134548,7.68756697112423));
#59649=CARTESIAN_POINT('Ctrl Pts',(-66.,-12.5638109939272,7.75694076391353));
#59650=CARTESIAN_POINT('Ctrl Pts',(-50.,-12.5638109939272,7.75694076391353));
#59651=CARTESIAN_POINT('Ctrl Pts',(-66.,-12.6565110535803,7.82939076691323));
#59652=CARTESIAN_POINT('Ctrl Pts',(-50.,-12.6565110535803,7.82939076691323));
#59653=CARTESIAN_POINT('Ctrl Pts',(-66.,-12.7464782795223,7.9054109081407));
#59654=CARTESIAN_POINT('Ctrl Pts',(-50.,-12.7464782795223,7.9054109081407));
#59655=CARTESIAN_POINT('Ctrl Pts',(-66.,-12.8333072263957,7.98553702611316));
#59656=CARTESIAN_POINT('Ctrl Pts',(-50.,-12.8333072263957,7.98553702611316));
#59657=CARTESIAN_POINT('Ctrl Pts',(-66.,-12.9167494409123,8.07034649661759));
#59658=CARTESIAN_POINT('Ctrl Pts',(-50.,-12.9167494409123,8.07034649661759));
#59659=CARTESIAN_POINT('Ctrl Pts',(-66.,-12.9967646908729,8.16026752634251));
#59660=CARTESIAN_POINT('Ctrl Pts',(-50.,-12.9967646908729,8.16026752634251));
#59661=CARTESIAN_POINT('Ctrl Pts',(-66.,-13.0735719476516,8.2552497632047));
#59662=CARTESIAN_POINT('Ctrl Pts',(-50.,-13.0735719476516,8.2552497632047));
#59663=CARTESIAN_POINT('Ctrl Pts',(-66.,-13.1476766619554,8.35455196515643));
#59664=CARTESIAN_POINT('Ctrl Pts',(-50.,-13.1476766619554,8.35455196515643));
#59665=CARTESIAN_POINT('Ctrl Pts',(-66.,-13.2199692944164,8.45629920475326));
#59666=CARTESIAN_POINT('Ctrl Pts',(-50.,-13.2199692944164,8.45629920475326));
#59667=CARTESIAN_POINT('Ctrl Pts',(-66.,-13.2915701735423,8.557804399923));
#59668=CARTESIAN_POINT('Ctrl Pts',(-50.,-13.2915701735423,8.557804399923));
#59669=CARTESIAN_POINT('Ctrl Pts',(-66.,-13.3633320128944,8.65689099100683));
#59670=CARTESIAN_POINT('Ctrl Pts',(-50.,-13.3633320128944,8.65689099100683));
#59671=CARTESIAN_POINT('Ctrl Pts',(-66.,-13.4354725852278,8.7528532374933));
#59672=CARTESIAN_POINT('Ctrl Pts',(-50.,-13.4354725852278,8.7528532374933));
#59673=CARTESIAN_POINT('Ctrl Pts',(-66.,-13.5070556576137,8.84780971091874));
#59674=CARTESIAN_POINT('Ctrl Pts',(-50.,-13.5070556576137,8.84780971091874));
#59675=CARTESIAN_POINT('Ctrl Pts',(-66.,-13.5758183415752,8.9471865570421));
#59676=CARTESIAN_POINT('Ctrl Pts',(-50.,-13.5758183415752,8.9471865570421));
#59677=CARTESIAN_POINT('Ctrl Pts',(-66.,-13.6393985665122,9.0567109207601));
#59678=CARTESIAN_POINT('Ctrl Pts',(-50.,-13.6393985665122,9.0567109207601));
#59679=CARTESIAN_POINT('Ctrl Pts',(-66.,-13.6963879047689,9.17984080520628));
#59680=CARTESIAN_POINT('Ctrl Pts',(-50.,-13.6963879047689,9.17984080520628));
#59681=CARTESIAN_POINT('Ctrl Pts',(-66.,-13.7474046302415,9.31514187328191));
#59682=CARTESIAN_POINT('Ctrl Pts',(-50.,-13.7474046302415,9.31514187328191));
#59683=CARTESIAN_POINT('Ctrl Pts',(-66.,-13.7963063276482,9.4533268215348));
#59684=CARTESIAN_POINT('Ctrl Pts',(-50.,-13.7963063276482,9.4533268215348));
#59685=CARTESIAN_POINT('Ctrl Pts',(-66.,-13.8492525549383,9.57952542768277));
#59686=CARTESIAN_POINT('Ctrl Pts',(-50.,-13.8492525549383,9.57952542768277));
#59687=CARTESIAN_POINT('Ctrl Pts',(-66.,-13.9135130516827,9.67617398568753));
#59688=CARTESIAN_POINT('Ctrl Pts',(-50.,-13.9135130516827,9.67617398568753));
#59689=CARTESIAN_POINT('Ctrl Pts',(-66.,-13.9964541688655,9.72547191786523));
#59690=CARTESIAN_POINT('Ctrl Pts',(-50.,-13.9964541688655,9.72547191786523));
#59691=CARTESIAN_POINT('Ctrl Pts',(-66.,-14.1042598989495,9.71248252455659));
#59692=CARTESIAN_POINT('Ctrl Pts',(-50.,-14.1042598989495,9.71248252455659));
#59693=CARTESIAN_POINT('Ctrl Pts',(-66.,-14.2415877332851,9.62596662912619));
#59694=CARTESIAN_POINT('Ctrl Pts',(-50.,-14.2415877332851,9.62596662912619));
#59695=CARTESIAN_POINT('Ctrl Pts',(-66.,-14.4119109068994,9.45755182333451));
#59696=CARTESIAN_POINT('Ctrl Pts',(-50.,-14.4119109068994,9.45755182333451));
#59697=CARTESIAN_POINT('Ctrl Pts',(-66.,-14.6176527534638,9.20140599515898));
#59698=CARTESIAN_POINT('Ctrl Pts',(-50.,-14.6176527534638,9.20140599515898));
#59699=CARTESIAN_POINT('Ctrl Pts',(-66.,-14.8603967131463,8.85372752977427));
#59700=CARTESIAN_POINT('Ctrl Pts',(-50.,-14.8603967131463,8.85372752977427));
#59701=CARTESIAN_POINT('Ctrl Pts',(-66.,-15.1410546573881,8.41233672184739));
#59702=CARTESIAN_POINT('Ctrl Pts',(-50.,-15.1410546573881,8.41233672184739));
#59703=CARTESIAN_POINT('Ctrl Pts',(-66.,-15.4600447033794,7.87624429847578));
#59704=CARTESIAN_POINT('Ctrl Pts',(-50.,-15.4600447033794,7.87624429847578));
#59705=CARTESIAN_POINT('Ctrl Pts',(-66.,-15.7459748034105,7.37144760803722));
#59706=CARTESIAN_POINT('Ctrl Pts',(-50.,-15.7459748034105,7.37144760803722));
#59707=CARTESIAN_POINT('Ctrl Pts',(-66.,-15.9776798358492,6.95022755696745));
#59708=CARTESIAN_POINT('Ctrl Pts',(-50.,-15.9776798358492,6.95022755696745));
#59709=CARTESIAN_POINT('Ctrl Pts',(-66.,-16.1398096369224,6.65049603710921));
#59710=CARTESIAN_POINT('Ctrl Pts',(-50.,-16.1398096369224,6.65049603710921));
#59711=CARTESIAN_POINT('Ctrl Pts',(-66.,-16.2227894831771,6.49590073696634));
#59712=CARTESIAN_POINT('Ctrl Pts',(-50.,-16.2227894831771,6.49590073696634));
#59713=CARTESIAN_POINT('',(-65.5,-13.8729177747003,9.60769365750208));
#59714=CARTESIAN_POINT('Ctrl Pts',(-66.,-13.6388425130122,9.0621520570585));
#59715=CARTESIAN_POINT('Ctrl Pts',(-65.7933280154028,-13.7472614276904,
9.27242719182262));
#59716=CARTESIAN_POINT('Ctrl Pts',(-65.6370761749494,-13.7926957795761,
9.48276801426461));
#59717=CARTESIAN_POINT('Ctrl Pts',(-65.5,-13.8729177747003,9.60769365750208));
#59718=CARTESIAN_POINT('',(-66.,-11.9725570665522,7.37643433768309));
#59719=CARTESIAN_POINT('',(-50.5,-13.8729177747003,9.60769365750209));
#59720=CARTESIAN_POINT('Ctrl Pts',(-50.5,-13.8729177747003,9.60769365750208));
#59721=CARTESIAN_POINT('Ctrl Pts',(-50.4518618349123,-13.8447455584389,
9.56382249433257));
#59722=CARTESIAN_POINT('Ctrl Pts',(-50.4012423593885,-13.8206924223065,
9.50957310384971));
#59723=CARTESIAN_POINT('Ctrl Pts',(-50.2441129793801,-13.7511164514545,
9.33310335708368));
#59724=CARTESIAN_POINT('Ctrl Pts',(-50.1366827452943,-13.7105454819895,
9.20121774969557));
#59725=CARTESIAN_POINT('Ctrl Pts',(-50.,-13.6388425130122,9.0621520570585));
#59726=CARTESIAN_POINT('Ctrl Pts',(-65.5,-13.8729177747003,9.60769365750208));
#59727=CARTESIAN_POINT('Ctrl Pts',(-60.5,-13.8729177747003,9.60769365750208));
#59728=CARTESIAN_POINT('Ctrl Pts',(-55.5,-13.8729177747003,9.60769365750208));
#59729=CARTESIAN_POINT('Ctrl Pts',(-50.5,-13.8729177747003,9.60769365750208));
#59730=CARTESIAN_POINT('Origin',(-66.,0.,0.));
#59731=CARTESIAN_POINT('',(-66.,-12.6433463826116,6.15627310142281));
#59732=CARTESIAN_POINT('Ctrl Pts',(-66.,-16.2227894831771,6.49590073696634));
#59733=CARTESIAN_POINT('Ctrl Pts',(-50.,-16.2227894831771,6.49590073696634));
#59734=CARTESIAN_POINT('Ctrl Pts',(-66.,-16.2006994791252,6.50022537552599));
#59735=CARTESIAN_POINT('Ctrl Pts',(-50.,-16.2006994791252,6.50022537552599));
#59736=CARTESIAN_POINT('Ctrl Pts',(-66.,-16.156541644553,6.50872846327372));
#59737=CARTESIAN_POINT('Ctrl Pts',(-50.,-16.156541644553,6.50872846327372));
#59738=CARTESIAN_POINT('Ctrl Pts',(-66.,-16.0903714131301,6.52104452743828));
#59739=CARTESIAN_POINT('Ctrl Pts',(-50.,-16.0903714131301,6.52104452743828));
#59740=CARTESIAN_POINT('Ctrl Pts',(-66.,-16.0022776570719,6.53658763924282));
#59741=CARTESIAN_POINT('Ctrl Pts',(-50.,-16.0022776570719,6.53658763924282));
#59742=CARTESIAN_POINT('Ctrl Pts',(-66.,-15.8923837101016,6.55454673713648));
#59743=CARTESIAN_POINT('Ctrl Pts',(-50.,-15.8923837101016,6.55454673713648));
#59744=CARTESIAN_POINT('Ctrl Pts',(-66.,-15.7827148976515,6.57102989138234));
#59745=CARTESIAN_POINT('Ctrl Pts',(-50.,-15.7827148976515,6.57102989138234));
#59746=CARTESIAN_POINT('Ctrl Pts',(-66.,-15.6732735922887,6.58603394412518));
#59747=CARTESIAN_POINT('Ctrl Pts',(-50.,-15.6732735922887,6.58603394412518));
#59748=CARTESIAN_POINT('Ctrl Pts',(-66.,-15.5640626036015,6.59956147249643));
#59749=CARTESIAN_POINT('Ctrl Pts',(-50.,-15.5640626036015,6.59956147249643));
#59750=CARTESIAN_POINT('Ctrl Pts',(-66.,-15.4550847247379,6.61162519170432));
#59751=CARTESIAN_POINT('Ctrl Pts',(-50.,-15.4550847247379,6.61162519170432));
#59752=CARTESIAN_POINT('Ctrl Pts',(-66.,-15.346345674173,6.62223885631155));
#59753=CARTESIAN_POINT('Ctrl Pts',(-50.,-15.346345674173,6.62223885631155));
#59754=CARTESIAN_POINT('Ctrl Pts',(-66.,-15.2378573655599,6.63140668952709));
#59755=CARTESIAN_POINT('Ctrl Pts',(-50.,-15.2378573655599,6.63140668952709));
#59756=CARTESIAN_POINT('Ctrl Pts',(-66.,-15.1296413868434,6.63911263660376));
#59757=CARTESIAN_POINT('Ctrl Pts',(-50.,-15.1296413868434,6.63911263660376));
#59758=CARTESIAN_POINT('Ctrl Pts',(-66.,-15.021731679342,6.64531162852697));
#59759=CARTESIAN_POINT('Ctrl Pts',(-50.,-15.021731679342,6.64531162852697));
#59760=CARTESIAN_POINT('Ctrl Pts',(-66.,-14.9141794743276,6.64991522010611));
#59761=CARTESIAN_POINT('Ctrl Pts',(-50.,-14.9141794743276,6.64991522010611));
#59762=CARTESIAN_POINT('Ctrl Pts',(-66.,-14.8070445527658,6.65281215957283));
#59763=CARTESIAN_POINT('Ctrl Pts',(-50.,-14.8070445527658,6.65281215957283));
#59764=CARTESIAN_POINT('Ctrl Pts',(-66.,-14.7003831899324,6.65389759319505));
#59765=CARTESIAN_POINT('Ctrl Pts',(-50.,-14.7003831899324,6.65389759319505));
#59766=CARTESIAN_POINT('Ctrl Pts',(-66.,-14.5942361525827,6.65310192943101));
#59767=CARTESIAN_POINT('Ctrl Pts',(-50.,-14.5942361525827,6.65310192943101));
#59768=CARTESIAN_POINT('Ctrl Pts',(-66.,-14.4886188383546,6.65041484137187));
#59769=CARTESIAN_POINT('Ctrl Pts',(-50.,-14.4886188383546,6.65041484137187));
#59770=CARTESIAN_POINT('Ctrl Pts',(-66.,-14.3835044844334,6.64592554509403));
#59771=CARTESIAN_POINT('Ctrl Pts',(-50.,-14.3835044844334,6.64592554509403));
#59772=CARTESIAN_POINT('Ctrl Pts',(-66.,-14.278844877945,6.63977511862666));
#59773=CARTESIAN_POINT('Ctrl Pts',(-50.,-14.278844877945,6.63977511862666));
#59774=CARTESIAN_POINT('Ctrl Pts',(-66.,-14.1746034538834,6.63207978306306));
#59775=CARTESIAN_POINT('Ctrl Pts',(-50.,-14.1746034538834,6.63207978306306));
#59776=CARTESIAN_POINT('Ctrl Pts',(-66.,-14.0707863033563,6.6228591657896));
#59777=CARTESIAN_POINT('Ctrl Pts',(-50.,-14.0707863033563,6.6228591657896));
#59778=CARTESIAN_POINT('Ctrl Pts',(-66.,-13.9674696839217,6.61197280385553));
#59779=CARTESIAN_POINT('Ctrl Pts',(-50.,-13.9674696839217,6.61197280385553));
#59780=CARTESIAN_POINT('Ctrl Pts',(-66.,-13.8648408383502,6.59902554716193));
#59781=CARTESIAN_POINT('Ctrl Pts',(-50.,-13.8648408383502,6.59902554716193));
#59782=CARTESIAN_POINT('Ctrl Pts',(-66.,-13.7631634644371,6.58344942858329));
#59783=CARTESIAN_POINT('Ctrl Pts',(-50.,-13.7631634644371,6.58344942858329));
#59784=CARTESIAN_POINT('Ctrl Pts',(-66.,-13.6627176703106,6.56464523470766));
#59785=CARTESIAN_POINT('Ctrl Pts',(-50.,-13.6627176703106,6.56464523470766));
#59786=CARTESIAN_POINT('Ctrl Pts',(-66.,-13.5637463059047,6.54210941091933));
#59787=CARTESIAN_POINT('Ctrl Pts',(-50.,-13.5637463059047,6.54210941091933));
#59788=CARTESIAN_POINT('Ctrl Pts',(-66.,-13.4664030834197,6.51555637763196));
#59789=CARTESIAN_POINT('Ctrl Pts',(-50.,-13.4664030834197,6.51555637763196));
#59790=CARTESIAN_POINT('Ctrl Pts',(-66.,-13.3706871739224,6.48507374642914));
#59791=CARTESIAN_POINT('Ctrl Pts',(-50.,-13.3706871739224,6.48507374642914));
#59792=CARTESIAN_POINT('Ctrl Pts',(-66.,-13.2764716751216,6.45105019532836));
#59793=CARTESIAN_POINT('Ctrl Pts',(-50.,-13.2764716751216,6.45105019532836));
#59794=CARTESIAN_POINT('Ctrl Pts',(-66.,-13.1835561890537,6.41404502367149));
#59795=CARTESIAN_POINT('Ctrl Pts',(-50.,-13.1835561890537,6.41404502367149));
#59796=CARTESIAN_POINT('Ctrl Pts',(-66.,-13.0917112937495,6.37467717998103));
#59797=CARTESIAN_POINT('Ctrl Pts',(-50.,-13.0917112937495,6.37467717998103));
#59798=CARTESIAN_POINT('Ctrl Pts',(-66.,-13.0007243712348,6.33351120238525));
#59799=CARTESIAN_POINT('Ctrl Pts',(-50.,-13.0007243712348,6.33351120238525));
#59800=CARTESIAN_POINT('Ctrl Pts',(-66.,-12.9104491054422,6.29093354993378));
#59801=CARTESIAN_POINT('Ctrl Pts',(-50.,-12.9104491054422,6.29093354993378));
#59802=CARTESIAN_POINT('Ctrl Pts',(-66.,-12.8207969747412,6.24717657480866));
#59803=CARTESIAN_POINT('Ctrl Pts',(-50.,-12.8207969747412,6.24717657480866));
#59804=CARTESIAN_POINT('Ctrl Pts',(-66.,-12.7495367835008,6.21132350319834));
#59805=CARTESIAN_POINT('Ctrl Pts',(-50.,-12.7495367835008,6.21132350319834));
#59806=CARTESIAN_POINT('Ctrl Pts',(-66.,-12.6963436971102,6.18397603231157));
#59807=CARTESIAN_POINT('Ctrl Pts',(-50.,-12.6963436971102,6.18397603231157));
#59808=CARTESIAN_POINT('Ctrl Pts',(-66.,-12.6609935089309,6.16554126565498));
#59809=CARTESIAN_POINT('Ctrl Pts',(-50.,-12.6609935089309,6.16554126565498));
#59810=CARTESIAN_POINT('Ctrl Pts',(-66.,-12.6433463826116,6.1562731014228));
#59811=CARTESIAN_POINT('Ctrl Pts',(-50.,-12.6433463826116,6.1562731014228));
#59812=CARTESIAN_POINT('Origin',(-65.75,0.,0.));
#59813=CARTESIAN_POINT('',(-65.5,-13.3994067863357,10.2577542753909));
#59814=CARTESIAN_POINT('Origin',(-65.5,0.,0.));
#59815=CARTESIAN_POINT('Ctrl Pts',(-65.5,-13.3994067863357,10.2577542753909));
#59816=CARTESIAN_POINT('Ctrl Pts',(-65.6931595476697,-13.1796296666677,
10.2270765724828));
#59817=CARTESIAN_POINT('Ctrl Pts',(-65.8611256967046,-12.9932804974997,
10.1925190475036));
#59818=CARTESIAN_POINT('Ctrl Pts',(-66.,-12.8416620037784,10.1603317849721));
#59819=CARTESIAN_POINT('Origin',(-58.,0.,0.));
#59820=CARTESIAN_POINT('',(-50.5,-13.3994067863357,10.2577542753909));
#59821=CARTESIAN_POINT('Origin',(-50.5,0.,0.));
#59822=CARTESIAN_POINT('Ctrl Pts',(-50.5,-13.3994067863357,10.2577542753909));
#59823=CARTESIAN_POINT('Ctrl Pts',(-55.5,-13.3994067863357,10.2577542753909));
#59824=CARTESIAN_POINT('Ctrl Pts',(-60.5,-13.3994067863357,10.2577542753909));
#59825=CARTESIAN_POINT('Ctrl Pts',(-65.5,-13.3994067863357,10.2577542753909));
#59826=CARTESIAN_POINT('Origin',(-50.25,0.,0.));
#59827=CARTESIAN_POINT('Ctrl Pts',(-50.,-12.8416620037784,10.1603317849721));
#59828=CARTESIAN_POINT('Ctrl Pts',(-50.1388743032962,-12.9932804975006,
10.1925190475038));
#59829=CARTESIAN_POINT('Ctrl Pts',(-50.3068404523311,-13.1796296666686,
10.2270765724829));
#59830=CARTESIAN_POINT('Ctrl Pts',(-50.5,-13.3994067863357,10.2577542753909));
#59831=CARTESIAN_POINT('Ctrl Pts',(-66.,-9.76197254719673,10.1221439546065));
#59832=CARTESIAN_POINT('Ctrl Pts',(-50.,-9.76197254719673,10.1221439546065));
#59833=CARTESIAN_POINT('Ctrl Pts',(-66.,-9.77887468091545,10.1382862065996));
#59834=CARTESIAN_POINT('Ctrl Pts',(-50.,-9.77887468091545,10.1382862065996));
#59835=CARTESIAN_POINT('Ctrl Pts',(-66.,-9.8125301973609,10.1707396505663));
#59836=CARTESIAN_POINT('Ctrl Pts',(-50.,-9.8125301973609,10.1707396505663));
#59837=CARTESIAN_POINT('Ctrl Pts',(-66.,-9.86256723189823,10.2199266327873));
#59838=CARTESIAN_POINT('Ctrl Pts',(-50.,-9.86256723189823,10.2199266327873));
#59839=CARTESIAN_POINT('Ctrl Pts',(-66.,-9.92838949999087,10.2865242878363));
#59840=CARTESIAN_POINT('Ctrl Pts',(-50.,-9.92838949999087,10.2865242878363));
#59841=CARTESIAN_POINT('Ctrl Pts',(-66.,-10.0091279489326,10.371490948043));
#59842=CARTESIAN_POINT('Ctrl Pts',(-50.,-10.0091279489326,10.371490948043));
#59843=CARTESIAN_POINT('Ctrl Pts',(-66.,-10.0881874924486,10.4582479603236));
#59844=CARTESIAN_POINT('Ctrl Pts',(-50.,-10.0881874924486,10.4582479603236));
#59845=CARTESIAN_POINT('Ctrl Pts',(-66.,-10.1653013890907,10.5469256916157));
#59846=CARTESIAN_POINT('Ctrl Pts',(-50.,-10.1653013890907,10.5469256916157));
#59847=CARTESIAN_POINT('Ctrl Pts',(-66.,-10.2400230449985,10.6377349442392));
#59848=CARTESIAN_POINT('Ctrl Pts',(-50.,-10.2400230449985,10.6377349442392));
#59849=CARTESIAN_POINT('Ctrl Pts',(-66.,-10.3117931787431,10.7309623645438));
#59850=CARTESIAN_POINT('Ctrl Pts',(-50.,-10.3117931787431,10.7309623645438));
#59851=CARTESIAN_POINT('Ctrl Pts',(-66.,-10.3800284784999,10.8269681325114));
#59852=CARTESIAN_POINT('Ctrl Pts',(-50.,-10.3800284784999,10.8269681325114));
#59853=CARTESIAN_POINT('Ctrl Pts',(-66.,-10.4442029791024,10.9261704221467));
#59854=CARTESIAN_POINT('Ctrl Pts',(-50.,-10.4442029791024,10.9261704221467));
#59855=CARTESIAN_POINT('Ctrl Pts',(-66.,-10.5039324453602,11.0290666820944));
#59856=CARTESIAN_POINT('Ctrl Pts',(-50.,-10.5039324453602,11.0290666820944));
#59857=CARTESIAN_POINT('Ctrl Pts',(-66.,-10.5590714183695,11.1360616608015));
#59858=CARTESIAN_POINT('Ctrl Pts',(-50.,-10.5590714183695,11.1360616608015));
#59859=CARTESIAN_POINT('Ctrl Pts',(-66.,-10.6098445121699,11.2471610440543));
#59860=CARTESIAN_POINT('Ctrl Pts',(-50.,-10.6098445121699,11.2471610440543));
#59861=CARTESIAN_POINT('Ctrl Pts',(-66.,-10.6569256372063,11.3617725777663));
#59862=CARTESIAN_POINT('Ctrl Pts',(-50.,-10.6569256372063,11.3617725777663));
#59863=CARTESIAN_POINT('Ctrl Pts',(-66.,-10.7016435541469,11.4783016873407));
#59864=CARTESIAN_POINT('Ctrl Pts',(-50.,-10.7016435541469,11.4783016873407));
#59865=CARTESIAN_POINT('Ctrl Pts',(-66.,-10.7457516444569,11.5944243246999));
#59866=CARTESIAN_POINT('Ctrl Pts',(-50.,-10.7457516444569,11.5944243246999));
#59867=CARTESIAN_POINT('Ctrl Pts',(-66.,-10.7906171205087,11.7082443720486));
#59868=CARTESIAN_POINT('Ctrl Pts',(-50.,-10.7906171205087,11.7082443720486));
#59869=CARTESIAN_POINT('Ctrl Pts',(-66.,-10.8366264238543,11.819132418893));
#59870=CARTESIAN_POINT('Ctrl Pts',(-50.,-10.8366264238543,11.819132418893));
#59871=CARTESIAN_POINT('Ctrl Pts',(-66.,-10.8823458677273,11.9289076462876));
#59872=CARTESIAN_POINT('Ctrl Pts',(-50.,-10.8823458677273,11.9289076462876));
#59873=CARTESIAN_POINT('Ctrl Pts',(-66.,-10.9242342288773,12.0422629701643));
#59874=CARTESIAN_POINT('Ctrl Pts',(-50.,-10.9242342288773,12.0422629701643));
#59875=CARTESIAN_POINT('Ctrl Pts',(-66.,-10.9585793624772,12.1641581835604));
#59876=CARTESIAN_POINT('Ctrl Pts',(-50.,-10.9585793624772,12.1641581835604));
#59877=CARTESIAN_POINT('Ctrl Pts',(-66.,-10.983157118807,12.2975923883674));
#59878=CARTESIAN_POINT('Ctrl Pts',(-50.,-10.983157118807,12.2975923883674));
#59879=CARTESIAN_POINT('Ctrl Pts',(-66.,-10.9989230526826,12.4413300682894));
#59880=CARTESIAN_POINT('Ctrl Pts',(-50.,-10.9989230526826,12.4413300682894));
#59881=CARTESIAN_POINT('Ctrl Pts',(-66.,-11.0119232141524,12.5873350398988));
#59882=CARTESIAN_POINT('Ctrl Pts',(-50.,-11.0119232141524,12.5873350398988));
#59883=CARTESIAN_POINT('Ctrl Pts',(-66.,-11.0318217212277,12.7227360760623));
#59884=CARTESIAN_POINT('Ctrl Pts',(-50.,-11.0318217212277,12.7227360760623));
#59885=CARTESIAN_POINT('Ctrl Pts',(-66.,-11.0700278373151,12.8323291775776));
#59886=CARTESIAN_POINT('Ctrl Pts',(-50.,-11.0700278373151,12.8323291775776));
#59887=CARTESIAN_POINT('Ctrl Pts',(-66.,-11.1381033095929,12.9007049416369));
#59888=CARTESIAN_POINT('Ctrl Pts',(-50.,-11.1381033095929,12.9007049416369));
#59889=CARTESIAN_POINT('Ctrl Pts',(-66.,-11.2457524551817,12.9149338288552));
#59890=CARTESIAN_POINT('Ctrl Pts',(-50.,-11.2457524551817,12.9149338288552));
#59891=CARTESIAN_POINT('Ctrl Pts',(-66.,-11.400281511346,12.8652880329968));
#59892=CARTESIAN_POINT('Ctrl Pts',(-50.,-11.400281511346,12.8652880329968));
#59893=CARTESIAN_POINT('Ctrl Pts',(-66.,-11.607136728308,12.7445219388499));
#59894=CARTESIAN_POINT('Ctrl Pts',(-50.,-11.607136728308,12.7445219388499));
#59895=CARTESIAN_POINT('Ctrl Pts',(-66.,-11.8701156935365,12.547589319493));
#59896=CARTESIAN_POINT('Ctrl Pts',(-50.,-11.8701156935365,12.547589319493));
#59897=CARTESIAN_POINT('Ctrl Pts',(-66.,-12.1916975236769,12.2712017803777));
#59898=CARTESIAN_POINT('Ctrl Pts',(-50.,-12.1916975236769,12.2712017803777));
#59899=CARTESIAN_POINT('Ctrl Pts',(-66.,-12.5733075127254,11.9134748688282));
#59900=CARTESIAN_POINT('Ctrl Pts',(-50.,-12.5733075127254,11.9134748688282));
#59901=CARTESIAN_POINT('Ctrl Pts',(-66.,-13.0155966641184,11.4735543732861));
#59902=CARTESIAN_POINT('Ctrl Pts',(-50.,-13.0155966641184,11.4735543732861));
#59903=CARTESIAN_POINT('Ctrl Pts',(-66.,-13.4180815762547,11.0557247234476));
#59904=CARTESIAN_POINT('Ctrl Pts',(-50.,-13.4180815762547,11.0557247234476));
#59905=CARTESIAN_POINT('Ctrl Pts',(-66.,-13.7472603359957,10.7053607732244));
#59906=CARTESIAN_POINT('Ctrl Pts',(-50.,-13.7472603359957,10.7053607732244));
#59907=CARTESIAN_POINT('Ctrl Pts',(-66.,-13.9788367290857,10.4553659121651));
#59908=CARTESIAN_POINT('Ctrl Pts',(-50.,-13.9788367290857,10.4553659121651));
#59909=CARTESIAN_POINT('Ctrl Pts',(-66.,-14.0976558986297,10.3262637562592));
#59910=CARTESIAN_POINT('Ctrl Pts',(-50.,-14.0976558986297,10.3262637562592));
#59911=CARTESIAN_POINT('',(-65.5,-11.0477383006981,12.7559046499764));
#59912=CARTESIAN_POINT('Ctrl Pts',(-66.,-10.9566876228483,12.1692900916743));
#59913=CARTESIAN_POINT('Ctrl Pts',(-65.7933280154032,-11.0094070584153,
12.3999217340683));
#59914=CARTESIAN_POINT('Ctrl Pts',(-65.6370761749493,-11.0011043711894,
12.6149533766279));
#59915=CARTESIAN_POINT('Ctrl Pts',(-65.5,-11.0477383006981,12.7559046499764));
#59916=CARTESIAN_POINT('',(-66.,-9.76197254719673,10.1221439546065));
#59917=CARTESIAN_POINT('',(-50.5,-11.0477383006981,12.7559046499764));
#59918=CARTESIAN_POINT('Ctrl Pts',(-50.5,-11.0477383006981,12.7559046499764));
#59919=CARTESIAN_POINT('Ctrl Pts',(-50.4518618349123,-11.0313614810341,
12.706405634788));
#59920=CARTESIAN_POINT('Ctrl Pts',(-50.4012423593886,-11.0215552932018,
12.6478788169541));
#59921=CARTESIAN_POINT('Ctrl Pts',(-50.2441129793802,-10.9980514208266,
12.4596503514474));
#59922=CARTESIAN_POINT('Ctrl Pts',(-50.1366827452942,-10.9915536797922,
12.3218185831175));
#59923=CARTESIAN_POINT('Ctrl Pts',(-50.,-10.9566876228483,12.1692900916743));
#59924=CARTESIAN_POINT('Ctrl Pts',(-65.5,-11.0477383006981,12.7559046499764));
#59925=CARTESIAN_POINT('Ctrl Pts',(-60.5,-11.0477383006981,12.7559046499764));
#59926=CARTESIAN_POINT('Ctrl Pts',(-55.5,-11.0477383006981,12.7559046499764));
#59927=CARTESIAN_POINT('Ctrl Pts',(-50.5,-11.0477383006981,12.7559046499764));
#59928=CARTESIAN_POINT('Origin',(-66.,0.,0.));
#59929=CARTESIAN_POINT('',(-66.,-10.7151295435653,9.10713484662512));
#59930=CARTESIAN_POINT('Ctrl Pts',(-66.,-14.0976558986297,10.3262637562592));
#59931=CARTESIAN_POINT('Ctrl Pts',(-50.,-14.0976558986297,10.3262637562592));
#59932=CARTESIAN_POINT('Ctrl Pts',(-66.,-14.0751843988004,10.3249589677309));
#59933=CARTESIAN_POINT('Ctrl Pts',(-50.,-14.0751843988004,10.3249589677309));
#59934=CARTESIAN_POINT('Ctrl Pts',(-66.,-14.0302992318693,10.3222133084437));
#59935=CARTESIAN_POINT('Ctrl Pts',(-50.,-14.0302992318693,10.3222133084437));
#59936=CARTESIAN_POINT('Ctrl Pts',(-66.,-13.9631449793377,10.3176865734186));
#59937=CARTESIAN_POINT('Ctrl Pts',(-50.,-13.9631449793377,10.3176865734186));
#59938=CARTESIAN_POINT('Ctrl Pts',(-66.,-13.8739534358983,10.31083334353));
#59939=CARTESIAN_POINT('Ctrl Pts',(-50.,-13.8739534358983,10.31083334353));
#59940=CARTESIAN_POINT('Ctrl Pts',(-66.,-13.7630457633241,10.3008987100667));
#59941=CARTESIAN_POINT('Ctrl Pts',(-50.,-13.7630457633241,10.3008987100667));
#59942=CARTESIAN_POINT('Ctrl Pts',(-66.,-13.6527232045145,10.2895904911179));
#59943=CARTESIAN_POINT('Ctrl Pts',(-50.,-13.6527232045145,10.2895904911179));
#59944=CARTESIAN_POINT('Ctrl Pts',(-66.,-13.5429888428245,10.2769062180714));
#59945=CARTESIAN_POINT('Ctrl Pts',(-50.,-13.5429888428245,10.2769062180714));
#59946=CARTESIAN_POINT('Ctrl Pts',(-66.,-13.4338447586676,10.2628490858097));
#59947=CARTESIAN_POINT('Ctrl Pts',(-50.,-13.4338447586676,10.2628490858097));
#59948=CARTESIAN_POINT('Ctrl Pts',(-66.,-13.3252904952962,10.247432104697));
#59949=CARTESIAN_POINT('Ctrl Pts',(-50.,-13.3252904952962,10.247432104697));
#59950=CARTESIAN_POINT('Ctrl Pts',(-66.,-13.2173281709084,10.230670019298));
#59951=CARTESIAN_POINT('Ctrl Pts',(-50.,-13.2173281709084,10.230670019298));
#59952=CARTESIAN_POINT('Ctrl Pts',(-66.,-13.1099682745984,10.2125698829469));
#59953=CARTESIAN_POINT('Ctrl Pts',(-50.,-13.1099682745984,10.2125698829469));
#59954=CARTESIAN_POINT('Ctrl Pts',(-66.,-13.0032357087396,10.1931215139895));
#59955=CARTESIAN_POINT('Ctrl Pts',(-50.,-13.0032357087396,10.1931215139895));
#59956=CARTESIAN_POINT('Ctrl Pts',(-66.,-12.8971745565295,10.1722897001998));
#59957=CARTESIAN_POINT('Ctrl Pts',(-50.,-12.8971745565295,10.1722897001998));
#59958=CARTESIAN_POINT('Ctrl Pts',(-66.,-12.7918564351399,10.1500015157547));
#59959=CARTESIAN_POINT('Ctrl Pts',(-50.,-12.7918564351399,10.1500015157547));
#59960=CARTESIAN_POINT('Ctrl Pts',(-66.,-12.6873669145973,10.1261640709864));
#59961=CARTESIAN_POINT('Ctrl Pts',(-50.,-12.6873669145973,10.1261640709864));
#59962=CARTESIAN_POINT('Ctrl Pts',(-66.,-12.5837865782488,10.1006898014275));
#59963=CARTESIAN_POINT('Ctrl Pts',(-50.,-12.5837865782488,10.1006898014275));
#59964=CARTESIAN_POINT('Ctrl Pts',(-66.,-12.4811722187999,10.0735214401623));
#59965=CARTESIAN_POINT('Ctrl Pts',(-50.,-12.4811722187999,10.0735214401623));
#59966=CARTESIAN_POINT('Ctrl Pts',(-66.,-12.3795413183411,10.0446528139577));
#59967=CARTESIAN_POINT('Ctrl Pts',(-50.,-12.3795413183411,10.0446528139577));
#59968=CARTESIAN_POINT('Ctrl Pts',(-66.,-12.2788457677249,10.0141636803616));
#59969=CARTESIAN_POINT('Ctrl Pts',(-50.,-12.2788457677249,10.0141636803616));
#59970=CARTESIAN_POINT('Ctrl Pts',(-66.,-12.179003784094,9.98217869512325));
#59971=CARTESIAN_POINT('Ctrl Pts',(-50.,-12.179003784094,9.98217869512325));
#59972=CARTESIAN_POINT('Ctrl Pts',(-66.,-12.079951048189,9.94880133468933));
#59973=CARTESIAN_POINT('Ctrl Pts',(-50.,-12.079951048189,9.94880133468933));
#59974=CARTESIAN_POINT('Ctrl Pts',(-66.,-11.9816885786214,9.91405212461268));
#59975=CARTESIAN_POINT('Ctrl Pts',(-50.,-11.9816885786214,9.91405212461268));
#59976=CARTESIAN_POINT('Ctrl Pts',(-66.,-11.8843251688933,9.87781397932795));
#59977=CARTESIAN_POINT('Ctrl Pts',(-50.,-11.8843251688933,9.87781397932795));
#59978=CARTESIAN_POINT('Ctrl Pts',(-66.,-11.7881404490329,9.83975072848667));
#59979=CARTESIAN_POINT('Ctrl Pts',(-50.,-11.7881404490329,9.83975072848667));
#59980=CARTESIAN_POINT('Ctrl Pts',(-66.,-11.6935310799647,9.79937782767));
#59981=CARTESIAN_POINT('Ctrl Pts',(-50.,-11.6935310799647,9.79937782767));
#59982=CARTESIAN_POINT('Ctrl Pts',(-66.,-11.6009173880207,9.75618454891596));
#59983=CARTESIAN_POINT('Ctrl Pts',(-50.,-11.6009173880207,9.75618454891596));
#59984=CARTESIAN_POINT('Ctrl Pts',(-66.,-11.5106598224983,9.70974355202577));
#59985=CARTESIAN_POINT('Ctrl Pts',(-50.,-11.5106598224983,9.70974355202577));
#59986=CARTESIAN_POINT('Ctrl Pts',(-66.,-11.4229782872014,9.65981645609066));
#59987=CARTESIAN_POINT('Ctrl Pts',(-50.,-11.4229782872014,9.65981645609066));
#59988=CARTESIAN_POINT('Ctrl Pts',(-66.,-11.3378501911246,9.60648791406797));
#59989=CARTESIAN_POINT('Ctrl Pts',(-50.,-11.3378501911246,9.60648791406797));
#59990=CARTESIAN_POINT('Ctrl Pts',(-66.,-11.255055958553,9.55010283362399));
#59991=CARTESIAN_POINT('Ctrl Pts',(-50.,-11.255055958553,9.55010283362399));
#59992=CARTESIAN_POINT('Ctrl Pts',(-66.,-11.1742623953034,9.49115310573639));
#59993=CARTESIAN_POINT('Ctrl Pts',(-50.,-11.1742623953034,9.49115310573639));
#59994=CARTESIAN_POINT('Ctrl Pts',(-66.,-11.0950933608815,9.43018117859799));
#59995=CARTESIAN_POINT('Ctrl Pts',(-50.,-11.0950933608815,9.43018117859799));
#59996=CARTESIAN_POINT('Ctrl Pts',(-66.,-11.0172025221741,9.36768097839366));
#59997=CARTESIAN_POINT('Ctrl Pts',(-50.,-11.0172025221741,9.36768097839366));
#59998=CARTESIAN_POINT('Ctrl Pts',(-66.,-10.9403520514449,9.30399043552504));
#59999=CARTESIAN_POINT('Ctrl Pts',(-50.,-10.9403520514449,9.30399043552504));
#60000=CARTESIAN_POINT('Ctrl Pts',(-66.,-10.8643984244951,9.23931258796881));
#60001=CARTESIAN_POINT('Ctrl Pts',(-50.,-10.8643984244951,9.23931258796881));
#60002=CARTESIAN_POINT('Ctrl Pts',(-66.,-10.8042932995341,9.18686421761339));
#60003=CARTESIAN_POINT('Ctrl Pts',(-50.,-10.8042932995341,9.18686421761339));
#60004=CARTESIAN_POINT('Ctrl Pts',(-66.,-10.7595724112169,9.14714733516059));
#60005=CARTESIAN_POINT('Ctrl Pts',(-50.,-10.7595724112169,9.14714733516059));
#60006=CARTESIAN_POINT('Ctrl Pts',(-66.,-10.7299173542433,9.1205004962881));
#60007=CARTESIAN_POINT('Ctrl Pts',(-50.,-10.7299173542433,9.1205004962881));
#60008=CARTESIAN_POINT('Ctrl Pts',(-66.,-10.7151295435653,9.10713484662511));
#60009=CARTESIAN_POINT('Ctrl Pts',(-50.,-10.7151295435653,9.10713484662511));
#60010=CARTESIAN_POINT('Origin',(-65.75,0.,0.));
#60011=CARTESIAN_POINT('',(-65.5,-10.4274400290457,13.2677850239087));
#60012=CARTESIAN_POINT('Origin',(-65.5,0.,0.));
#60013=CARTESIAN_POINT('Ctrl Pts',(-65.5,-10.4274400290457,13.2677850239087));
#60014=CARTESIAN_POINT('Ctrl Pts',(-65.6931595476722,-10.222196846206,13.183414770357));
#60015=CARTESIAN_POINT('Ctrl Pts',(-65.861125696707,-10.0502962858477,13.1035997797182));
#60016=CARTESIAN_POINT('Ctrl Pts',(-66.,-9.91144581260293,13.0347177531328));
#60017=CARTESIAN_POINT('Origin',(-58.,0.,0.));
#60018=CARTESIAN_POINT('',(-50.5,-10.4274400290457,13.2677850239087));
#60019=CARTESIAN_POINT('Origin',(-50.5,0.,0.));
#60020=CARTESIAN_POINT('Ctrl Pts',(-50.5,-10.4274400290457,13.2677850239087));
#60021=CARTESIAN_POINT('Ctrl Pts',(-55.5,-10.4274400290457,13.2677850239087));
#60022=CARTESIAN_POINT('Ctrl Pts',(-60.5,-10.4274400290457,13.2677850239087));
#60023=CARTESIAN_POINT('Ctrl Pts',(-65.5,-10.4274400290457,13.2677850239087));
#60024=CARTESIAN_POINT('Origin',(-50.25,0.,0.));
#60025=CARTESIAN_POINT('Ctrl Pts',(-50.,-9.91144581260292,13.0347177531328));
#60026=CARTESIAN_POINT('Ctrl Pts',(-50.1388743032951,-10.0502962858498,
13.1035997797192));
#60027=CARTESIAN_POINT('Ctrl Pts',(-50.3068404523279,-10.2221968462061,
13.1834147703571));
#60028=CARTESIAN_POINT('Ctrl Pts',(-50.5,-10.4274400290457,13.2677850239087));
#60029=CARTESIAN_POINT('Ctrl Pts',(-66.,-6.93800739067721,12.2318420402206));
#60030=CARTESIAN_POINT('Ctrl Pts',(-50.,-6.93800739067721,12.2318420402206));
#60031=CARTESIAN_POINT('Ctrl Pts',(-66.,-6.95036409795758,12.2516805434111));
#60032=CARTESIAN_POINT('Ctrl Pts',(-50.,-6.95036409795758,12.2516805434111));
#60033=CARTESIAN_POINT('Ctrl Pts',(-66.,-6.97489142114752,12.2914841893452));
#60034=CARTESIAN_POINT('Ctrl Pts',(-50.,-6.97489142114752,12.2914841893452));
#60035=CARTESIAN_POINT('Ctrl Pts',(-66.,-7.01112414517467,12.3515695765444));
#60036=CARTESIAN_POINT('Ctrl Pts',(-50.,-7.01112414517467,12.3515695765444));
#60037=CARTESIAN_POINT('Ctrl Pts',(-66.,-7.05831632235693,12.4324442762203));
#60038=CARTESIAN_POINT('Ctrl Pts',(-50.,-7.05831632235693,12.4324442762203));
#60039=CARTESIAN_POINT('Ctrl Pts',(-66.,-7.11538787531798,12.5348203883111));
#60040=CARTESIAN_POINT('Ctrl Pts',(-50.,-7.11538787531798,12.5348203883111));
#60041=CARTESIAN_POINT('Ctrl Pts',(-66.,-7.17038802629925,12.6385130784722));
#60042=CARTESIAN_POINT('Ctrl Pts',(-50.,-7.17038802629925,12.6385130784722));
#60043=CARTESIAN_POINT('Ctrl Pts',(-66.,-7.22302599308674,12.7435822820237));
#60044=CARTESIAN_POINT('Ctrl Pts',(-50.,-7.22302599308674,12.7435822820237));
#60045=CARTESIAN_POINT('Ctrl Pts',(-66.,-7.27281678798223,12.8501211151659));
#60046=CARTESIAN_POINT('Ctrl Pts',(-50.,-7.27281678798223,12.8501211151659));
#60047=CARTESIAN_POINT('Ctrl Pts',(-66.,-7.31914741436296,12.9582681310911));
#60048=CARTESIAN_POINT('Ctrl Pts',(-50.,-7.31914741436296,12.9582681310911));
#60049=CARTESIAN_POINT('Ctrl Pts',(-66.,-7.36136331309888,13.0682271303129));
#60050=CARTESIAN_POINT('Ctrl Pts',(-50.,-7.36136331309888,13.0682271303129));
#60051=CARTESIAN_POINT('Ctrl Pts',(-66.,-7.39885104754049,13.1802723469128));
#60052=CARTESIAN_POINT('Ctrl Pts',(-50.,-7.39885104754049,13.1802723469128));
#60053=CARTESIAN_POINT('Ctrl Pts',(-66.,-7.43111474350486,13.2947900458654));
#60054=CARTESIAN_POINT('Ctrl Pts',(-50.,-7.43111474350486,13.2947900458654));
#60055=CARTESIAN_POINT('Ctrl Pts',(-66.,-7.45791285510172,13.4121360855424));
#60056=CARTESIAN_POINT('Ctrl Pts',(-50.,-7.45791285510172,13.4121360855424));
#60057=CARTESIAN_POINT('Ctrl Pts',(-66.,-7.47946152571002,13.5323718323411));
#60058=CARTESIAN_POINT('Ctrl Pts',(-50.,-7.47946152571002,13.5323718323411));
#60059=CARTESIAN_POINT('Ctrl Pts',(-66.,-7.49656078124055,13.6550912336386));
#60060=CARTESIAN_POINT('Ctrl Pts',(-50.,-7.49656078124055,13.6550912336386));
#60061=CARTESIAN_POINT('Ctrl Pts',(-66.,-7.51089419147856,13.7790802606718));
#60062=CARTESIAN_POINT('Ctrl Pts',(-50.,-7.51089419147856,13.7790802606718));
#60063=CARTESIAN_POINT('Ctrl Pts',(-66.,-7.52473801944021,13.9025239278461));
#60064=CARTESIAN_POINT('Ctrl Pts',(-50.,-7.52473801944021,13.9025239278461));
#60065=CARTESIAN_POINT('Ctrl Pts',(-66.,-7.53988806932779,14.0239256992838));
#60066=CARTESIAN_POINT('Ctrl Pts',(-50.,-7.53988806932779,14.0239256992838));
#60067=CARTESIAN_POINT('Ctrl Pts',(-66.,-7.55687516994583,14.1427720426853));
#60068=CARTESIAN_POINT('Ctrl Pts',(-50.,-7.55687516994583,14.1427720426853));
#60069=CARTESIAN_POINT('Ctrl Pts',(-66.,-7.5738582645032,14.2604684427868));
#60070=CARTESIAN_POINT('Ctrl Pts',(-50.,-7.5738582645032,14.2604684427868));
#60071=CARTESIAN_POINT('Ctrl Pts',(-66.,-7.58624030305585,14.380679712526));
#60072=CARTESIAN_POINT('Ctrl Pts',(-50.,-7.58624030305585,14.380679712526));
#60073=CARTESIAN_POINT('Ctrl Pts',(-66.,-7.58919231426205,14.5072866510432));
#60074=CARTESIAN_POINT('Ctrl Pts',(-50.,-7.58919231426205,14.5072866510432));
#60075=CARTESIAN_POINT('Ctrl Pts',(-66.,-7.57981417784402,14.6426410143862));
#60076=CARTESIAN_POINT('Ctrl Pts',(-50.,-7.57981417784402,14.6426410143862));
#60077=CARTESIAN_POINT('Ctrl Pts',(-66.,-7.55933868851428,14.785783739095));
#60078=CARTESIAN_POINT('Ctrl Pts',(-50.,-7.55933868851428,14.785783739095));
#60079=CARTESIAN_POINT('Ctrl Pts',(-66.,-7.53562046609085,14.930434704726));
#60080=CARTESIAN_POINT('Ctrl Pts',(-50.,-7.53562046609085,14.930434704726));
#60081=CARTESIAN_POINT('Ctrl Pts',(-66.,-7.52122095657002,15.0665304258326));
#60082=CARTESIAN_POINT('Ctrl Pts',(-50.,-7.52122095657002,15.0665304258326));
#60083=CARTESIAN_POINT('Ctrl Pts',(-66.,-7.53097206121459,15.1821819332349));
#60084=CARTESIAN_POINT('Ctrl Pts',(-50.,-7.53097206121459,15.1821819332349));
#60085=CARTESIAN_POINT('Ctrl Pts',(-66.,-7.57990445630002,15.2653392284515));
#60086=CARTESIAN_POINT('Ctrl Pts',(-50.,-7.57990445630002,15.2653392284515));
#60087=CARTESIAN_POINT('Ctrl Pts',(-66.,-7.68063302567044,15.3058923428827));
#60088=CARTESIAN_POINT('Ctrl Pts',(-50.,-7.68063302567044,15.3058923428827));
#60089=CARTESIAN_POINT('Ctrl Pts',(-66.,-7.84265367474648,15.2962360745346));
#60090=CARTESIAN_POINT('Ctrl Pts',(-50.,-7.84265367474648,15.2962360745346));
#60091=CARTESIAN_POINT('Ctrl Pts',(-66.,-8.07304346101417,15.2307068698744));
#60092=CARTESIAN_POINT('Ctrl Pts',(-50.,-8.07304346101417,15.2307068698744));
#60093=CARTESIAN_POINT('Ctrl Pts',(-66.,-8.37673560935255,15.1053614600777));
#60094=CARTESIAN_POINT('Ctrl Pts',(-50.,-8.37673560935255,15.1053614600777));
#60095=CARTESIAN_POINT('Ctrl Pts',(-66.,-8.75694914086774,14.9176312927967));
#60096=CARTESIAN_POINT('Ctrl Pts',(-50.,-8.75694914086774,14.9176312927967));
#60097=CARTESIAN_POINT('Ctrl Pts',(-66.,-9.2155332156477,14.6660455751048));
#60098=CARTESIAN_POINT('Ctrl Pts',(-50.,-9.2155332156477,14.6660455751048));
#60099=CARTESIAN_POINT('Ctrl Pts',(-66.,-9.75333081843477,14.3499388300415));
#60100=CARTESIAN_POINT('Ctrl Pts',(-50.,-9.75333081843477,14.3499388300415));
#60101=CARTESIAN_POINT('Ctrl Pts',(-66.,-10.2470809354107,14.0453299943724));
#60102=CARTESIAN_POINT('Ctrl Pts',(-50.,-10.2470809354107,14.0453299943724));
#60103=CARTESIAN_POINT('Ctrl Pts',(-66.,-10.6530499103448,13.7878368005368));
#60104=CARTESIAN_POINT('Ctrl Pts',(-50.,-10.6530499103448,13.7878368005368));
#60105=CARTESIAN_POINT('Ctrl Pts',(-66.,-10.9395220989952,13.6032866948137));
#60106=CARTESIAN_POINT('Ctrl Pts',(-50.,-10.9395220989952,13.6032866948137));
#60107=CARTESIAN_POINT('Ctrl Pts',(-66.,-11.0867147464198,13.5077896464047));
#60108=CARTESIAN_POINT('Ctrl Pts',(-50.,-11.0867147464198,13.5077896464047));
#60109=CARTESIAN_POINT('',(-65.5,-7.52838879852371,15.102615240357));
#60110=CARTESIAN_POINT('Ctrl Pts',(-66.,-7.58608375346252,14.5117868743119));
#60111=CARTESIAN_POINT('Ctrl Pts',(-65.793328015403,-7.57979115389329,14.748283590041));
#60112=CARTESIAN_POINT('Ctrl Pts',(-65.6370761749494,-7.51827311592916,
14.9544948237843));
#60113=CARTESIAN_POINT('Ctrl Pts',(-65.5,-7.52838879852371,15.102615240357));
#60114=CARTESIAN_POINT('',(-66.,-6.93800739067721,12.2318420402206));
#60115=CARTESIAN_POINT('',(-50.5,-7.52838879852371,15.102615240357));
#60116=CARTESIAN_POINT('Ctrl Pts',(-50.5,-7.52838879852371,15.102615240357));
#60117=CARTESIAN_POINT('Ctrl Pts',(-50.4518618349125,-7.5248363912663,15.050598578319));
#60118=CARTESIAN_POINT('Ctrl Pts',(-50.401242359389,-7.52989331058026,14.9914717883454));
#60119=CARTESIAN_POINT('Ctrl Pts',(-50.2441129793808,-7.55393837142435,
14.8033116908419));
#60120=CARTESIAN_POINT('Ctrl Pts',(-50.1366827452945,-7.58192213578687,
14.6681942384838));
#60121=CARTESIAN_POINT('Ctrl Pts',(-50.,-7.58608375346252,14.5117868743119));
#60122=CARTESIAN_POINT('Ctrl Pts',(-65.5,-7.52838879852371,15.102615240357));
#60123=CARTESIAN_POINT('Ctrl Pts',(-60.5,-7.52838879852371,15.102615240357));
#60124=CARTESIAN_POINT('Ctrl Pts',(-55.5,-7.52838879852371,15.102615240357));
#60125=CARTESIAN_POINT('Ctrl Pts',(-50.5,-7.52838879852371,15.102615240357));
#60126=CARTESIAN_POINT('Origin',(-66.,0.,0.));
#60127=CARTESIAN_POINT('',(-66.,-8.11364170780697,11.4857618157149));
#60128=CARTESIAN_POINT('Ctrl Pts',(-66.,-11.0867147464198,13.5077896464047));
#60129=CARTESIAN_POINT('Ctrl Pts',(-50.,-11.0867147464198,13.5077896464047));
#60130=CARTESIAN_POINT('Ctrl Pts',(-66.,-11.0652737177917,13.5009374154504));
#60131=CARTESIAN_POINT('Ctrl Pts',(-50.,-11.0652737177917,13.5009374154504));
#60132=CARTESIAN_POINT('Ctrl Pts',(-66.,-11.0224815186161,13.4871155289992));
#60133=CARTESIAN_POINT('Ctrl Pts',(-50.,-11.0224815186161,13.4871155289992));
#60134=CARTESIAN_POINT('Ctrl Pts',(-66.,-10.9585627936384,13.4660304261943));
#60135=CARTESIAN_POINT('Ctrl Pts',(-50.,-10.9585627936384,13.4660304261943));
#60136=CARTESIAN_POINT('Ctrl Pts',(-66.,-10.8738776955157,13.4372114682508));
#60137=CARTESIAN_POINT('Ctrl Pts',(-50.,-10.8738776955157,13.4372114682508));
#60138=CARTESIAN_POINT('Ctrl Pts',(-66.,-10.7689250342954,13.4000073329881));
#60139=CARTESIAN_POINT('Ctrl Pts',(-50.,-10.7689250342954,13.4000073329881));
#60140=CARTESIAN_POINT('Ctrl Pts',(-66.,-10.6648807012342,13.3616182778297));
#60141=CARTESIAN_POINT('Ctrl Pts',(-50.,-10.6648807012342,13.3616182778297));
#60142=CARTESIAN_POINT('Ctrl Pts',(-66.,-10.5617482967368,13.322042678519));
#60143=CARTESIAN_POINT('Ctrl Pts',(-50.,-10.5617482967368,13.322042678519));
#60144=CARTESIAN_POINT('Ctrl Pts',(-66.,-10.4595290413216,13.2812841469428));
#60145=CARTESIAN_POINT('Ctrl Pts',(-50.,-10.4595290413216,13.2812841469428));
#60146=CARTESIAN_POINT('Ctrl Pts',(-66.,-10.3582192570447,13.2393551711326));
#60147=CARTESIAN_POINT('Ctrl Pts',(-50.,-10.3582192570447,13.2393551711326));
#60148=CARTESIAN_POINT('Ctrl Pts',(-66.,-10.2578173287328,13.1962705591997));
#60149=CARTESIAN_POINT('Ctrl Pts',(-50.,-10.2578173287328,13.1962705591997));
#60150=CARTESIAN_POINT('Ctrl Pts',(-66.,-10.1583316618534,13.1520397514165));
#60151=CARTESIAN_POINT('Ctrl Pts',(-50.,-10.1583316618534,13.1520397514165));
#60152=CARTESIAN_POINT('Ctrl Pts',(-66.,-10.0597889085,13.1066590789727));
#60153=CARTESIAN_POINT('Ctrl Pts',(-50.,-10.0597889085,13.1066590789727));
#60154=CARTESIAN_POINT('Ctrl Pts',(-66.,-9.9622405238402,13.0601053989445));
#60155=CARTESIAN_POINT('Ctrl Pts',(-50.,-9.9622405238402,13.0601053989445));
#60156=CARTESIAN_POINT('Ctrl Pts',(-66.,-9.86577401097532,13.012325887074));
#60157=CARTESIAN_POINT('Ctrl Pts',(-50.,-9.86577401097532,13.012325887074));
#60158=CARTESIAN_POINT('Ctrl Pts',(-66.,-9.77049535231301,12.9632518523934));
#60159=CARTESIAN_POINT('Ctrl Pts',(-50.,-9.77049535231301,12.9632518523934));
#60160=CARTESIAN_POINT('Ctrl Pts',(-66.,-9.67650437592402,12.9128185216976));
#60161=CARTESIAN_POINT('Ctrl Pts',(-50.,-9.67650437592402,12.9128185216976));
#60162=CARTESIAN_POINT('Ctrl Pts',(-66.,-9.58387033196931,12.8609845509879));
#60163=CARTESIAN_POINT('Ctrl Pts',(-50.,-9.58387033196931,12.8609845509879));
#60164=CARTESIAN_POINT('Ctrl Pts',(-66.,-9.49261168852801,12.8077483085937));
#60165=CARTESIAN_POINT('Ctrl Pts',(-50.,-9.49261168852801,12.8077483085937));
#60166=CARTESIAN_POINT('Ctrl Pts',(-66.,-9.40266201299437,12.7531750820743));
#60167=CARTESIAN_POINT('Ctrl Pts',(-50.,-9.40266201299437,12.7531750820743));
#60168=CARTESIAN_POINT('Ctrl Pts',(-66.,-9.31391109124575,12.69736527232));
#60169=CARTESIAN_POINT('Ctrl Pts',(-50.,-9.31391109124575,12.69736527232));
#60170=CARTESIAN_POINT('Ctrl Pts',(-66.,-9.22627089118454,12.6404031093252));
#60171=CARTESIAN_POINT('Ctrl Pts',(-50.,-9.22627089118454,12.6404031093252));
#60172=CARTESIAN_POINT('Ctrl Pts',(-66.,-9.13973729492348,12.5823087271131));
#60173=CARTESIAN_POINT('Ctrl Pts',(-50.,-9.13973729492348,12.5823087271131));
#60174=CARTESIAN_POINT('Ctrl Pts',(-66.,-9.05444479601274,12.5229957744206));
#60175=CARTESIAN_POINT('Ctrl Pts',(-50.,-9.05444479601274,12.5229957744206));
#60176=CARTESIAN_POINT('Ctrl Pts',(-66.,-8.9707478415549,12.4622081834688));
#60177=CARTESIAN_POINT('Ctrl Pts',(-50.,-8.9707478415549,12.4622081834688));
#60178=CARTESIAN_POINT('Ctrl Pts',(-66.,-8.88915113193907,12.3995752782536));
#60179=CARTESIAN_POINT('Ctrl Pts',(-50.,-8.88915113193907,12.3995752782536));
#60180=CARTESIAN_POINT('Ctrl Pts',(-66.,-8.81018880105177,12.334706907179));
#60181=CARTESIAN_POINT('Ctrl Pts',(-50.,-8.81018880105177,12.334706907179));
#60182=CARTESIAN_POINT('Ctrl Pts',(-66.,-8.73431624919877,12.2672787958196));
#60183=CARTESIAN_POINT('Ctrl Pts',(-50.,-8.73431624919877,12.2672787958196));
#60184=CARTESIAN_POINT('Ctrl Pts',(-66.,-8.66180575442286,12.1971147402934));
#60185=CARTESIAN_POINT('Ctrl Pts',(-50.,-8.66180575442286,12.1971147402934));
#60186=CARTESIAN_POINT('Ctrl Pts',(-66.,-8.59261438312223,12.1242911158748));
#60187=CARTESIAN_POINT('Ctrl Pts',(-50.,-8.59261438312223,12.1242911158748));
#60188=CARTESIAN_POINT('Ctrl Pts',(-66.,-8.52644368290816,12.0490873880617));
#60189=CARTESIAN_POINT('Ctrl Pts',(-50.,-8.52644368290816,12.0490873880617));
#60190=CARTESIAN_POINT('Ctrl Pts',(-66.,-8.46284859919381,11.9718971321485));
#60191=CARTESIAN_POINT('Ctrl Pts',(-50.,-8.46284859919381,11.9718971321485));
#60192=CARTESIAN_POINT('Ctrl Pts',(-66.,-8.40132990725019,11.8931522119833));
#60193=CARTESIAN_POINT('Ctrl Pts',(-50.,-8.40132990725019,11.8931522119833));
#60194=CARTESIAN_POINT('Ctrl Pts',(-66.,-8.34142932020866,11.8132449066089));
#60195=CARTESIAN_POINT('Ctrl Pts',(-50.,-8.34142932020866,11.8132449066089));
#60196=CARTESIAN_POINT('Ctrl Pts',(-66.,-8.28283244225497,11.732443384369));
#60197=CARTESIAN_POINT('Ctrl Pts',(-50.,-8.28283244225497,11.732443384369));
#60198=CARTESIAN_POINT('Ctrl Pts',(-66.,-8.22534976477564,11.6509086114121));
#60199=CARTESIAN_POINT('Ctrl Pts',(-50.,-8.22534976477564,11.6509086114121));
#60200=CARTESIAN_POINT('Ctrl Pts',(-66.,-8.18017633214654,11.5851604663126));
#60201=CARTESIAN_POINT('Ctrl Pts',(-50.,-8.18017633214654,11.5851604663126));
#60202=CARTESIAN_POINT('Ctrl Pts',(-66.,-8.14673761978747,11.5355697300868));
#60203=CARTESIAN_POINT('Ctrl Pts',(-50.,-8.14673761978747,11.5355697300868));
#60204=CARTESIAN_POINT('Ctrl Pts',(-66.,-8.12464103031309,11.502385137885));
#60205=CARTESIAN_POINT('Ctrl Pts',(-50.,-8.12464103031309,11.502385137885));
#60206=CARTESIAN_POINT('Ctrl Pts',(-66.,-8.11364170780698,11.4857618157149));
#60207=CARTESIAN_POINT('Ctrl Pts',(-50.,-8.11364170780698,11.4857618157149));
#60208=CARTESIAN_POINT('Origin',(-65.75,0.,0.));
#60209=CARTESIAN_POINT('',(-65.5,-6.80027886528895,15.4441520438742));
#60210=CARTESIAN_POINT('Origin',(-65.5,0.,0.));
#60211=CARTESIAN_POINT('Ctrl Pts',(-65.5,-6.80027886528895,15.4441520438742));
#60212=CARTESIAN_POINT('Ctrl Pts',(-65.6931595476699,-6.62246580329175,
15.3113905330037));
#60213=CARTESIAN_POINT('Ctrl Pts',(-65.8611256967037,-6.4758149961569,15.1913331461071));
#60214=CARTESIAN_POINT('Ctrl Pts',(-66.,-6.35845702927375,15.0900844665257));
#60215=CARTESIAN_POINT('Origin',(-58.,0.,0.));
#60216=CARTESIAN_POINT('',(-50.5,-6.80027886528895,15.4441520438742));
#60217=CARTESIAN_POINT('Origin',(-50.5,0.,0.));
#60218=CARTESIAN_POINT('Ctrl Pts',(-50.5,-6.80027886528895,15.4441520438742));
#60219=CARTESIAN_POINT('Ctrl Pts',(-55.5,-6.80027886528895,15.4441520438742));
#60220=CARTESIAN_POINT('Ctrl Pts',(-60.5,-6.80027886528895,15.4441520438742));
#60221=CARTESIAN_POINT('Ctrl Pts',(-65.5,-6.80027886528895,15.4441520438742));
#60222=CARTESIAN_POINT('Origin',(-50.25,0.,0.));
#60223=CARTESIAN_POINT('Ctrl Pts',(-50.,-6.35845702927375,15.0900844665257));
#60224=CARTESIAN_POINT('Ctrl Pts',(-50.1388743032885,-6.47581499615029,
15.1913331461014));
#60225=CARTESIAN_POINT('Ctrl Pts',(-50.306840452323,-6.62246580328526,15.3113905329989));
#60226=CARTESIAN_POINT('Ctrl Pts',(-50.5,-6.80027886528894,15.4441520438742));
#60227=CARTESIAN_POINT('Ctrl Pts',(-66.,-3.67810171359515,13.5729685048794));
#60228=CARTESIAN_POINT('Ctrl Pts',(-50.,-3.67810171359515,13.5729685048794));
#60229=CARTESIAN_POINT('Ctrl Pts',(-66.,-3.68513657707394,13.595256733151));
#60230=CARTESIAN_POINT('Ctrl Pts',(-50.,-3.68513657707394,13.595256733151));
#60231=CARTESIAN_POINT('Ctrl Pts',(-66.,-3.69899456508718,13.6399095715909));
#60232=CARTESIAN_POINT('Ctrl Pts',(-50.,-3.69899456508718,13.6399095715909));
#60233=CARTESIAN_POINT('Ctrl Pts',(-66.,-3.71914634329887,13.7071179779119));
#60234=CARTESIAN_POINT('Ctrl Pts',(-50.,-3.71914634329887,13.7071179779119));
#60235=CARTESIAN_POINT('Ctrl Pts',(-66.,-3.7447431715177,13.7971880673979));
#60236=CARTESIAN_POINT('Ctrl Pts',(-50.,-3.7447431715177,13.7971880673979));
#60237=CARTESIAN_POINT('Ctrl Pts',(-66.,-3.77456181293102,13.910540963737));
#60238=CARTESIAN_POINT('Ctrl Pts',(-50.,-3.77456181293102,13.910540963737));
#60239=CARTESIAN_POINT('Ctrl Pts',(-66.,-3.80204670961501,14.0246539387008));
#60240=CARTESIAN_POINT('Ctrl Pts',(-50.,-3.80204670961501,14.0246539387008));
#60241=CARTESIAN_POINT('Ctrl Pts',(-66.,-3.82690130950572,14.1395127300348));
#60242=CARTESIAN_POINT('Ctrl Pts',(-50.,-3.82690130950572,14.1395127300348));
#60243=CARTESIAN_POINT('Ctrl Pts',(-66.,-3.84863270462788,14.2550869169872));
#60244=CARTESIAN_POINT('Ctrl Pts',(-50.,-3.84863270462788,14.2550869169872));
#60245=CARTESIAN_POINT('Ctrl Pts',(-66.,-3.86661269999714,14.3713582537855));
#60246=CARTESIAN_POINT('Ctrl Pts',(-50.,-3.86661269999714,14.3713582537855));
#60247=CARTESIAN_POINT('Ctrl Pts',(-66.,-3.88015661753544,14.4883613559395));
#60248=CARTESIAN_POINT('Ctrl Pts',(-50.,-3.88015661753544,14.4883613559395));
#60249=CARTESIAN_POINT('Ctrl Pts',(-66.,-3.88860209359085,14.6062092864715));
#60250=CARTESIAN_POINT('Ctrl Pts',(-50.,-3.88860209359085,14.6062092864715));
#60251=CARTESIAN_POINT('Ctrl Pts',(-66.,-3.89137277258683,14.725152856237));
#60252=CARTESIAN_POINT('Ctrl Pts',(-50.,-3.89137277258683,14.725152856237));
#60253=CARTESIAN_POINT('Ctrl Pts',(-66.,-3.88814619886307,14.8454766736426));
#60254=CARTESIAN_POINT('Ctrl Pts',(-50.,-3.88814619886307,14.8454766736426));
#60255=CARTESIAN_POINT('Ctrl Pts',(-66.,-3.87911646405442,14.9672939298197));
#60256=CARTESIAN_POINT('Ctrl Pts',(-50.,-3.87911646405442,14.9672939298197));
#60257=CARTESIAN_POINT('Ctrl Pts',(-66.,-3.86515944096752,15.0904102873887));
#60258=CARTESIAN_POINT('Ctrl Pts',(-50.,-3.86515944096752,15.0904102873887));
#60259=CARTESIAN_POINT('Ctrl Pts',(-66.,-3.84820772362302,15.2140685453126));
#60260=CARTESIAN_POINT('Ctrl Pts',(-50.,-3.84820772362302,15.2140685453126));
#60261=CARTESIAN_POINT('Ctrl Pts',(-66.,-3.83091743061146,15.3370768226993));
#60262=CARTESIAN_POINT('Ctrl Pts',(-50.,-3.83091743061146,15.3370768226993));
#60263=CARTESIAN_POINT('Ctrl Pts',(-66.,-3.81540012098238,15.4584321984421));
#60264=CARTESIAN_POINT('Ctrl Pts',(-50.,-3.81540012098238,15.4584321984421));
#60265=CARTESIAN_POINT('Ctrl Pts',(-66.,-3.80229765686693,15.5777692855585));
#60266=CARTESIAN_POINT('Ctrl Pts',(-50.,-3.80229765686693,15.5777692855585));
#60267=CARTESIAN_POINT('Ctrl Pts',(-66.,-3.7894772918181,15.6959915606914));
#60268=CARTESIAN_POINT('Ctrl Pts',(-50.,-3.7894772918181,15.6959915606914));
#60269=CARTESIAN_POINT('Ctrl Pts',(-66.,-3.77157499875327,15.8155054601092));
#60270=CARTESIAN_POINT('Ctrl Pts',(-50.,-3.77157499875327,15.8155054601092));
#60271=CARTESIAN_POINT('Ctrl Pts',(-66.,-3.74294840184491,15.9388689441728));
#60272=CARTESIAN_POINT('Ctrl Pts',(-50.,-3.74294840184491,15.9388689441728));
#60273=CARTESIAN_POINT('Ctrl Pts',(-66.,-3.70020363548059,16.0676386536046));
#60274=CARTESIAN_POINT('Ctrl Pts',(-50.,-3.70020363548059,16.0676386536046));
#60275=CARTESIAN_POINT('Ctrl Pts',(-66.,-3.64477327324364,16.2011922392645));
#60276=CARTESIAN_POINT('Ctrl Pts',(-50.,-3.64477327324364,16.2011922392645));
#60277=CARTESIAN_POINT('Ctrl Pts',(-66.,-3.58582697007134,16.3354002467575));
#60278=CARTESIAN_POINT('Ctrl Pts',(-50.,-3.58582697007134,16.3354002467575));
#60279=CARTESIAN_POINT('Ctrl Pts',(-66.,-3.53803421809535,16.4636392581249));
#60280=CARTESIAN_POINT('Ctrl Pts',(-50.,-3.53803421809535,16.4636392581249));
#60281=CARTESIAN_POINT('Ctrl Pts',(-66.,-3.51871761353015,16.5780823618678));
#60282=CARTESIAN_POINT('Ctrl Pts',(-50.,-3.51871761353015,16.5780823618678));
#60283=CARTESIAN_POINT('Ctrl Pts',(-66.,-3.54543232907923,16.6707961095521));
#60284=CARTESIAN_POINT('Ctrl Pts',(-50.,-3.54543232907923,16.6707961095521));
#60285=CARTESIAN_POINT('Ctrl Pts',(-66.,-3.63291117576394,16.7351253498724));
#60286=CARTESIAN_POINT('Ctrl Pts',(-50.,-3.63291117576394,16.7351253498724));
#60287=CARTESIAN_POINT('Ctrl Pts',(-66.,-3.79224306450002,16.7660653478883));
#60288=CARTESIAN_POINT('Ctrl Pts',(-50.,-3.79224306450002,16.7660653478883));
#60289=CARTESIAN_POINT('Ctrl Pts',(-66.,-4.03169118248789,16.7598904736431));
#60290=CARTESIAN_POINT('Ctrl Pts',(-50.,-4.03169118248789,16.7598904736431));
#60291=CARTESIAN_POINT('Ctrl Pts',(-66.,-4.35701441935439,16.7140081864924));
#60292=CARTESIAN_POINT('Ctrl Pts',(-50.,-4.35701441935439,16.7140081864924));
#60293=CARTESIAN_POINT('Ctrl Pts',(-66.,-4.77196943773181,16.6267311678792));
#60294=CARTESIAN_POINT('Ctrl Pts',(-50.,-4.77196943773181,16.6267311678792));
#60295=CARTESIAN_POINT('Ctrl Pts',(-66.,-5.27871307427053,16.497094699955));
#60296=CARTESIAN_POINT('Ctrl Pts',(-50.,-5.27871307427053,16.497094699955));
#60297=CARTESIAN_POINT('Ctrl Pts',(-66.,-5.87822732718726,16.3246638547222));
#60298=CARTESIAN_POINT('Ctrl Pts',(-50.,-5.87822732718726,16.3246638547222));
#60299=CARTESIAN_POINT('Ctrl Pts',(-66.,-6.43221851326742,16.1524155266404));
#60300=CARTESIAN_POINT('Ctrl Pts',(-50.,-6.43221851326742,16.1524155266404));
#60301=CARTESIAN_POINT('Ctrl Pts',(-66.,-6.88946917964989,16.0039723335548));
#60302=CARTESIAN_POINT('Ctrl Pts',(-50.,-6.88946917964989,16.0039723335548));
#60303=CARTESIAN_POINT('Ctrl Pts',(-66.,-7.21283706267689,15.8964629450382));
#60304=CARTESIAN_POINT('Ctrl Pts',(-50.,-7.21283706267689,15.8964629450382));
#60305=CARTESIAN_POINT('Ctrl Pts',(-66.,-7.37915453260775,15.8405714348913));
#60306=CARTESIAN_POINT('Ctrl Pts',(-50.,-7.37915453260775,15.8405714348913));
#60307=CARTESIAN_POINT('',(-65.5,-3.53600294066089,16.5003729716524));
#60308=CARTESIAN_POINT('Ctrl Pts',(-66.,-3.73881834218223,15.9424547170178));
#60309=CARTESIAN_POINT('Ctrl Pts',(-65.7933280154032,-3.67390909465031,
16.1699565476581));
#60310=CARTESIAN_POINT('Ctrl Pts',(-65.6370761749492,-3.56304111052069,
16.3543903623781));
#60311=CARTESIAN_POINT('Ctrl Pts',(-65.5,-3.53600294066089,16.5003729716524));
#60312=CARTESIAN_POINT('',(-66.,-3.67810171359515,13.5729685048794));
#60313=CARTESIAN_POINT('',(-50.5,-3.53600294066089,16.5003729716524));
#60314=CARTESIAN_POINT('Ctrl Pts',(-50.5,-3.53600294066089,16.5003729716524));
#60315=CARTESIAN_POINT('Ctrl Pts',(-50.4518618349121,-3.54549815662287,
16.4491070609439));
#60316=CARTESIAN_POINT('Ctrl Pts',(-50.4012423593883,-3.5651004382447,16.3930954524971));
#60317=CARTESIAN_POINT('Ctrl Pts',(-50.2441129793802,-3.63518359270379,
16.2168265139271));
#60318=CARTESIAN_POINT('Ctrl Pts',(-50.1366827452941,-3.69589053963102,
16.0929133040005));
#60319=CARTESIAN_POINT('Ctrl Pts',(-50.,-3.73881834218223,15.9424547170178));
#60320=CARTESIAN_POINT('Ctrl Pts',(-65.5,-3.53600294066089,16.5003729716524));
#60321=CARTESIAN_POINT('Ctrl Pts',(-60.5,-3.53600294066089,16.5003729716524));
#60322=CARTESIAN_POINT('Ctrl Pts',(-55.5,-3.53600294066089,16.5003729716524));
#60323=CARTESIAN_POINT('Ctrl Pts',(-50.5,-3.53600294066089,16.5003729716524));
#60324=CARTESIAN_POINT('Origin',(-66.,0.,0.));
#60325=CARTESIAN_POINT('',(-66.,-5.00234392366024,13.1426961282463));
#60326=CARTESIAN_POINT('Ctrl Pts',(-66.,-7.37915453260775,15.8405714348913));
#60327=CARTESIAN_POINT('Ctrl Pts',(-50.,-7.37915453260775,15.8405714348913));
#60328=CARTESIAN_POINT('Ctrl Pts',(-66.,-7.36009119386413,15.8286023123826));
#60329=CARTESIAN_POINT('Ctrl Pts',(-50.,-7.36009119386413,15.8286023123826));
#60330=CARTESIAN_POINT('Ctrl Pts',(-66.,-7.32208075369696,15.8045726787264));
#60331=CARTESIAN_POINT('Ctrl Pts',(-50.,-7.32208075369696,15.8045726787264));
#60332=CARTESIAN_POINT('Ctrl Pts',(-66.,-7.26541380484018,15.7682540626965));
#60333=CARTESIAN_POINT('Ctrl Pts',(-50.,-7.26541380484018,15.7682540626965));
#60334=CARTESIAN_POINT('Ctrl Pts',(-66.,-7.19055622819912,15.7192801778145));
#60335=CARTESIAN_POINT('Ctrl Pts',(-50.,-7.19055622819912,15.7192801778145));
#60336=CARTESIAN_POINT('Ctrl Pts',(-66.,-7.09815314002604,15.6571442133981));
#60337=CARTESIAN_POINT('Ctrl Pts',(-50.,-7.09815314002604,15.6571442133981));
#60338=CARTESIAN_POINT('Ctrl Pts',(-66.,-7.00692452080779,15.594086447551));
#60339=CARTESIAN_POINT('Ctrl Pts',(-50.,-7.00692452080779,15.594086447551));
#60340=CARTESIAN_POINT('Ctrl Pts',(-66.,-6.91687426177195,15.5301062024295));
#60341=CARTESIAN_POINT('Ctrl Pts',(-50.,-6.91687426177195,15.5301062024295));
#60342=CARTESIAN_POINT('Ctrl Pts',(-66.,-6.82800264685238,15.4652072799773));
#60343=CARTESIAN_POINT('Ctrl Pts',(-50.,-6.82800264685238,15.4652072799773));
#60344=CARTESIAN_POINT('Ctrl Pts',(-66.,-6.74030300800744,15.3994008612236));
#60345=CARTESIAN_POINT('Ctrl Pts',(-50.,-6.74030300800744,15.3994008612236));
#60346=CARTESIAN_POINT('Ctrl Pts',(-66.,-6.65377009817984,15.3327008873786));
#60347=CARTESIAN_POINT('Ctrl Pts',(-50.,-6.65377009817984,15.3327008873786));
#60348=CARTESIAN_POINT('Ctrl Pts',(-66.,-6.56840971106354,15.2651185924859));
#60349=CARTESIAN_POINT('Ctrl Pts',(-50.,-6.56840971106354,15.2651185924859));
#60350=CARTESIAN_POINT('Ctrl Pts',(-66.,-6.48424857382376,15.1966570511038));
#60351=CARTESIAN_POINT('Ctrl Pts',(-50.,-6.48424857382376,15.1966570511038));
#60352=CARTESIAN_POINT('Ctrl Pts',(-66.,-6.40134228048028,15.1273066437657));
#60353=CARTESIAN_POINT('Ctrl Pts',(-50.,-6.40134228048028,15.1273066437657));
#60354=CARTESIAN_POINT('Ctrl Pts',(-66.,-6.31978872192241,15.0570379669215));
#60355=CARTESIAN_POINT('Ctrl Pts',(-50.,-6.31978872192241,15.0570379669215));
#60356=CARTESIAN_POINT('Ctrl Pts',(-66.,-6.23970763367462,14.9858108444093));
#60357=CARTESIAN_POINT('Ctrl Pts',(-50.,-6.23970763367462,14.9858108444093));
#60358=CARTESIAN_POINT('Ctrl Pts',(-66.,-6.16121181596629,14.913587364225));
#60359=CARTESIAN_POINT('Ctrl Pts',(-50.,-6.16121181596629,14.913587364225));
#60360=CARTESIAN_POINT('Ctrl Pts',(-66.,-6.08437862517161,14.8403447030824));
#60361=CARTESIAN_POINT('Ctrl Pts',(-50.,-6.08437862517161,14.8403447030824));
#60362=CARTESIAN_POINT('Ctrl Pts',(-66.,-6.00922635494104,14.7660858733973));
#60363=CARTESIAN_POINT('Ctrl Pts',(-50.,-6.00922635494104,14.7660858733973));
#60364=CARTESIAN_POINT('Ctrl Pts',(-66.,-5.93567442341548,14.6908575904833));
#60365=CARTESIAN_POINT('Ctrl Pts',(-50.,-5.93567442341548,14.6908575904833));
#60366=CARTESIAN_POINT('Ctrl Pts',(-66.,-5.86359111036561,14.614729691814));
#60367=CARTESIAN_POINT('Ctrl Pts',(-50.,-5.86359111036561,14.614729691814));
#60368=CARTESIAN_POINT('Ctrl Pts',(-66.,-5.79287020223623,14.5377618684515));
#60369=CARTESIAN_POINT('Ctrl Pts',(-50.,-5.79287020223623,14.5377618684515));
#60370=CARTESIAN_POINT('Ctrl Pts',(-66.,-5.72350270338309,14.4599725977946));
#60371=CARTESIAN_POINT('Ctrl Pts',(-50.,-5.72350270338309,14.4599725977946));
#60372=CARTESIAN_POINT('Ctrl Pts',(-66.,-5.6556403566801,14.3813116886496));
#60373=CARTESIAN_POINT('Ctrl Pts',(-50.,-5.6556403566801,14.3813116886496));
#60374=CARTESIAN_POINT('Ctrl Pts',(-66.,-5.5896901550893,14.301619265488));
#60375=CARTESIAN_POINT('Ctrl Pts',(-50.,-5.5896901550893,14.301619265488));
#60376=CARTESIAN_POINT('Ctrl Pts',(-66.,-5.52623312628269,14.2206618116565));
#60377=CARTESIAN_POINT('Ctrl Pts',(-50.,-5.52623312628269,14.2206618116565));
#60378=CARTESIAN_POINT('Ctrl Pts',(-66.,-5.46588365010489,14.1381942665852));
#60379=CARTESIAN_POINT('Ctrl Pts',(-50.,-5.46588365010489,14.1381942665852));
#60380=CARTESIAN_POINT('Ctrl Pts',(-66.,-5.40916346339393,14.0540157969766));
#60381=CARTESIAN_POINT('Ctrl Pts',(-50.,-5.40916346339393,14.0540157969766));
#60382=CARTESIAN_POINT('Ctrl Pts',(-66.,-5.35638011020072,13.9680234475133));
#60383=CARTESIAN_POINT('Ctrl Pts',(-50.,-5.35638011020072,13.9680234475133));
#60384=CARTESIAN_POINT('Ctrl Pts',(-66.,-5.30747301200313,13.8802805168475));
#60385=CARTESIAN_POINT('Ctrl Pts',(-50.,-5.30747301200313,13.8802805168475));
#60386=CARTESIAN_POINT('Ctrl Pts',(-66.,-5.2620835925999,13.7909834684638));
#60387=CARTESIAN_POINT('Ctrl Pts',(-50.,-5.2620835925999,13.7909834684638));
#60388=CARTESIAN_POINT('Ctrl Pts',(-66.,-5.21968290141691,13.7004028321899));
#60389=CARTESIAN_POINT('Ctrl Pts',(-50.,-5.21968290141691,13.7004028321899));
#60390=CARTESIAN_POINT('Ctrl Pts',(-66.,-5.17967999761633,13.6088327519355));
#60391=CARTESIAN_POINT('Ctrl Pts',(-50.,-5.17967999761633,13.6088327519355));
#60392=CARTESIAN_POINT('Ctrl Pts',(-66.,-5.14153343642338,13.5165392112663));
#60393=CARTESIAN_POINT('Ctrl Pts',(-50.,-5.14153343642338,13.5165392112663));
#60394=CARTESIAN_POINT('Ctrl Pts',(-66.,-5.10487200859133,13.4237037664646));
#60395=CARTESIAN_POINT('Ctrl Pts',(-50.,-5.10487200859133,13.4237037664646));
#60396=CARTESIAN_POINT('Ctrl Pts',(-66.,-5.06947212861492,13.3304351977558));
#60397=CARTESIAN_POINT('Ctrl Pts',(-50.,-5.06947212861492,13.3304351977558));
#60398=CARTESIAN_POINT('Ctrl Pts',(-66.,-5.04206880122609,13.2555184756737));
#60399=CARTESIAN_POINT('Ctrl Pts',(-50.,-5.04206880122609,13.2555184756737));
#60400=CARTESIAN_POINT('Ctrl Pts',(-66.,-5.02201334210169,13.1991698540138));
#60401=CARTESIAN_POINT('Ctrl Pts',(-50.,-5.02201334210169,13.1991698540138));
#60402=CARTESIAN_POINT('Ctrl Pts',(-66.,-5.00886363010872,13.1615326184551));
#60403=CARTESIAN_POINT('Ctrl Pts',(-50.,-5.00886363010872,13.1615326184551));
#60404=CARTESIAN_POINT('Ctrl Pts',(-66.,-5.00234392366025,13.1426961282463));
#60405=CARTESIAN_POINT('Ctrl Pts',(-50.,-5.00234392366025,13.1426961282463));
#60406=CARTESIAN_POINT('Origin',(-65.75,0.,0.));
#60407=CARTESIAN_POINT('',(-65.5,-2.74583117074985,16.6501061913052));
#60408=CARTESIAN_POINT('Origin',(-65.5,0.,0.));
#60409=CARTESIAN_POINT('Ctrl Pts',(-65.5,-2.74583117077843,16.6501061913406));
#60410=CARTESIAN_POINT('Ctrl Pts',(-65.5715932578482,-2.69423901044128,
16.5860614560832));
#60411=CARTESIAN_POINT('Ctrl Pts',(-65.6431740852859,-2.64390488478764,
16.5216686692745));
#60412=CARTESIAN_POINT('Ctrl Pts',(-65.7145580549966,-2.59494005965581,
16.4571219801265));
#60413=CARTESIAN_POINT('Ctrl Pts',(-65.774031663176,-2.55414497868363,16.4033448574024));
#60414=CARTESIAN_POINT('Ctrl Pts',(-65.8333686244976,-2.51429886362145,
16.3494616552359));
#60415=CARTESIAN_POINT('Ctrl Pts',(-65.8924622803263,-2.47551032558372,
16.2955807679008));
#60416=CARTESIAN_POINT('Ctrl Pts',(-65.9284062038969,-2.45191706117835,
16.2628075290626));
#60417=CARTESIAN_POINT('Ctrl Pts',(-65.9642601111668,-2.42871664894537,
16.2300349028932));
#60418=CARTESIAN_POINT('Ctrl Pts',(-66.,-2.40594300602613,16.1972856754381));
#60419=CARTESIAN_POINT('Origin',(-58.,0.,0.));
#60420=CARTESIAN_POINT('',(-50.5,-2.74583117074985,16.6501061913052));
#60421=CARTESIAN_POINT('Origin',(-50.5,0.,0.));
#60422=CARTESIAN_POINT('Ctrl Pts',(-50.5,-2.74583117074984,16.6501061913052));
#60423=CARTESIAN_POINT('Ctrl Pts',(-55.5,-2.74583117074984,16.6501061913052));
#60424=CARTESIAN_POINT('Ctrl Pts',(-60.5,-2.74583117074984,16.6501061913052));
#60425=CARTESIAN_POINT('Ctrl Pts',(-65.5,-2.74583117074984,16.6501061913052));
#60426=CARTESIAN_POINT('Origin',(-50.25,0.,0.));
#60427=CARTESIAN_POINT('Ctrl Pts',(-50.,-2.40594300602613,16.1972856754381));
#60428=CARTESIAN_POINT('Ctrl Pts',(-50.0590457046711,-2.44356723592708,
16.2513905223095));
#60429=CARTESIAN_POINT('Ctrl Pts',(-50.1184026134405,-2.482354056013,16.3055596366217));
#60430=CARTESIAN_POINT('Ctrl Pts',(-50.177962494421,-2.52215873348076,16.3596887934234));
#60431=CARTESIAN_POINT('Ctrl Pts',(-50.2399196509175,-2.56356554273836,
16.4159966399769));
#60432=CARTESIAN_POINT('Ctrl Pts',(-50.3020964476471,-2.6060736528862,16.4722610173791));
#60433=CARTESIAN_POINT('Ctrl Pts',(-50.3643710506945,-2.64958385609203,
16.5283547796601));
#60434=CARTESIAN_POINT('Ctrl Pts',(-50.4095447363725,-2.68114593994685,
16.5690449143504));
#60435=CARTESIAN_POINT('Ctrl Pts',(-50.4547698875302,-2.71323705109809,
16.6096449710267));
#60436=CARTESIAN_POINT('Ctrl Pts',(-50.5,-2.74583117077843,16.6501061913406));
#60437=CARTESIAN_POINT('Ctrl Pts',(-66.,-0.187087378736033,14.0612554404903));
#60438=CARTESIAN_POINT('Ctrl Pts',(-50.,-0.187087378736033,14.0612554404903));
#60439=CARTESIAN_POINT('Ctrl Pts',(-66.,-0.188358372068459,14.0845929424903));
#60440=CARTESIAN_POINT('Ctrl Pts',(-50.,-0.188358372068459,14.0845929424903));
#60441=CARTESIAN_POINT('Ctrl Pts',(-66.,-0.190676276552008,14.1312892713751));
#60442=CARTESIAN_POINT('Ctrl Pts',(-50.,-0.190676276552008,14.1312892713751));
#60443=CARTESIAN_POINT('Ctrl Pts',(-66.,-0.193480898610155,14.2013977454735));
#60444=CARTESIAN_POINT('Ctrl Pts',(-50.,-0.193480898610155,14.2013977454735));
#60445=CARTESIAN_POINT('Ctrl Pts',(-66.,-0.195874035010017,14.2950037897925));
#60446=CARTESIAN_POINT('Ctrl Pts',(-50.,-0.195874035010017,14.2950037897925));
#60447=CARTESIAN_POINT('Ctrl Pts',(-66.,-0.196566149970303,14.4122110910203));
#60448=CARTESIAN_POINT('Ctrl Pts',(-50.,-0.196566149970303,14.4122110910203));
#60449=CARTESIAN_POINT('Ctrl Pts',(-66.,-0.194808815215985,14.5295742128916));
#60450=CARTESIAN_POINT('Ctrl Pts',(-50.,-0.194808815215985,14.5295742128916));
#60451=CARTESIAN_POINT('Ctrl Pts',(-66.,-0.190318342289957,14.6470055917277));
#60452=CARTESIAN_POINT('Ctrl Pts',(-50.,-0.190318342289957,14.6470055917277));
#60453=CARTESIAN_POINT('Ctrl Pts',(-66.,-0.182624874160768,14.7643531812717));
#60454=CARTESIAN_POINT('Ctrl Pts',(-50.,-0.182624874160768,14.7643531812717));
#60455=CARTESIAN_POINT('Ctrl Pts',(-66.,-0.171124489283723,14.8814430832361));
#60456=CARTESIAN_POINT('Ctrl Pts',(-50.,-0.171124489283723,14.8814430832361));
#60457=CARTESIAN_POINT('Ctrl Pts',(-66.,-0.155145411474415,14.9981385531066));
#60458=CARTESIAN_POINT('Ctrl Pts',(-50.,-0.155145411474415,14.9981385531066));
#60459=CARTESIAN_POINT('Ctrl Pts',(-66.,-0.13401796882278,15.1143843786811));
#60460=CARTESIAN_POINT('Ctrl Pts',(-50.,-0.13401796882278,15.1143843786811));
#60461=CARTESIAN_POINT('Ctrl Pts',(-66.,-0.107121538899203,15.2302801573274));
#60462=CARTESIAN_POINT('Ctrl Pts',(-50.,-0.107121538899203,15.2302801573274));
#60463=CARTESIAN_POINT('Ctrl Pts',(-66.,-0.0740730173483893,15.3460213644938));
#60464=CARTESIAN_POINT('Ctrl Pts',(-50.,-0.0740730173483893,15.3460213644938));
#60465=CARTESIAN_POINT('Ctrl Pts',(-66.,-0.035032248569878,15.4617659038311));
#60466=CARTESIAN_POINT('Ctrl Pts',(-50.,-0.035032248569878,15.4617659038311));
#60467=CARTESIAN_POINT('Ctrl Pts',(-66.,0.00910408204356977,15.5775433641354));
#60468=CARTESIAN_POINT('Ctrl Pts',(-50.,0.00910408204356977,15.5775433641354));
#60469=CARTESIAN_POINT('Ctrl Pts',(-66.,0.0562757882257695,15.6931009498213));
#60470=CARTESIAN_POINT('Ctrl Pts',(-50.,0.0562757882257695,15.6931009498213));
#60471=CARTESIAN_POINT('Ctrl Pts',(-66.,0.103613789511375,15.8079447749594));
#60472=CARTESIAN_POINT('Ctrl Pts',(-50.,0.103613789511375,15.8079447749594));
#60473=CARTESIAN_POINT('Ctrl Pts',(-66.,0.148823449024451,15.9216285504355));
#60474=CARTESIAN_POINT('Ctrl Pts',(-50.,0.148823449024451,15.9216285504355));
#60475=CARTESIAN_POINT('Ctrl Pts',(-66.,0.191192201865526,16.0339579931922));
#60476=CARTESIAN_POINT('Ctrl Pts',(-50.,0.191192201865526,16.0339579931922));
#60477=CARTESIAN_POINT('Ctrl Pts',(-66.,0.233010475834533,16.1452778030188));
#60478=CARTESIAN_POINT('Ctrl Pts',(-50.,0.233010475834533,16.1452778030188));
#60479=CARTESIAN_POINT('Ctrl Pts',(-66.,0.280072233603551,16.2565848342734));
#60480=CARTESIAN_POINT('Ctrl Pts',(-50.,0.280072233603551,16.2565848342734));
#60481=CARTESIAN_POINT('Ctrl Pts',(-66.,0.338478724261455,16.3689534824806));
#60482=CARTESIAN_POINT('Ctrl Pts',(-50.,0.338478724261455,16.3689534824806));
#60483=CARTESIAN_POINT('Ctrl Pts',(-66.,0.411904309697133,16.4830474635755));
#60484=CARTESIAN_POINT('Ctrl Pts',(-50.,0.411904309697133,16.4830474635755));
#60485=CARTESIAN_POINT('Ctrl Pts',(-66.,0.498806651323343,16.5986202472239));
#60486=CARTESIAN_POINT('Ctrl Pts',(-50.,0.498806651323343,16.5986202472239));
#60487=CARTESIAN_POINT('Ctrl Pts',(-66.,0.589277222226854,16.7139525138855));
#60488=CARTESIAN_POINT('Ctrl Pts',(-50.,0.589277222226854,16.7139525138855));
#60489=CARTESIAN_POINT('Ctrl Pts',(-66.,0.667460222281906,16.8262770867996));
#60490=CARTESIAN_POINT('Ctrl Pts',(-50.,0.667460222281906,16.8262770867996));
#60491=CARTESIAN_POINT('Ctrl Pts',(-66.,0.714630802750556,16.9323209057825));
#60492=CARTESIAN_POINT('Ctrl Pts',(-50.,0.714630802750556,16.9323209057825));
#60493=CARTESIAN_POINT('Ctrl Pts',(-66.,0.711812350565616,17.0287655601902));
#60494=CARTESIAN_POINT('Ctrl Pts',(-50.,0.711812350565616,17.0287655601902));
#60495=CARTESIAN_POINT('Ctrl Pts',(-66.,0.643079844228511,17.112828883644));
#60496=CARTESIAN_POINT('Ctrl Pts',(-50.,0.643079844228511,17.112828883644));
#60497=CARTESIAN_POINT('Ctrl Pts',(-66.,0.496448124383368,17.1824210741591));
#60498=CARTESIAN_POINT('Ctrl Pts',(-50.,0.496448124383368,17.1824210741591));
#60499=CARTESIAN_POINT('Ctrl Pts',(-66.,0.262987080557083,17.2359885203873));
#60500=CARTESIAN_POINT('Ctrl Pts',(-50.,0.262987080557083,17.2359885203873));
#60501=CARTESIAN_POINT('Ctrl Pts',(-66.,-0.0635259894100476,17.2724523087275));
#60502=CARTESIAN_POINT('Ctrl Pts',(-50.,-0.0635259894100476,17.2724523087275));
#60503=CARTESIAN_POINT('Ctrl Pts',(-66.,-0.487149344747227,17.2911123748441));
#60504=CARTESIAN_POINT('Ctrl Pts',(-50.,-0.487149344747227,17.2911123748441));
#60505=CARTESIAN_POINT('Ctrl Pts',(-66.,-1.01021197668826,17.2915706927367));
#60506=CARTESIAN_POINT('Ctrl Pts',(-50.,-1.01021197668826,17.2915706927367));
#60507=CARTESIAN_POINT('Ctrl Pts',(-66.,-1.6337731943647,17.2736502114967));
#60508=CARTESIAN_POINT('Ctrl Pts',(-50.,-1.6337731943647,17.2736502114967));
#60509=CARTESIAN_POINT('Ctrl Pts',(-66.,-2.21319614589061,17.2445853869407));
#60510=CARTESIAN_POINT('Ctrl Pts',(-50.,-2.21319614589061,17.2445853869407));
#60511=CARTESIAN_POINT('Ctrl Pts',(-66.,-2.69299776270237,17.2145194263625));
#60512=CARTESIAN_POINT('Ctrl Pts',(-50.,-2.69299776270237,17.2145194263625));
#60513=CARTESIAN_POINT('Ctrl Pts',(-66.,-3.03294294675148,17.1908059653249));
#60514=CARTESIAN_POINT('Ctrl Pts',(-50.,-3.03294294675148,17.1908059653249));
#60515=CARTESIAN_POINT('Ctrl Pts',(-66.,-3.20793490087994,17.1780318625772));
#60516=CARTESIAN_POINT('Ctrl Pts',(-50.,-3.20793490087994,17.1780318625772));
#60517=CARTESIAN_POINT('',(-65.5,0.678562986472808,16.8613515850121));
#60518=CARTESIAN_POINT('Ctrl Pts',(-66.,0.343370775949386,16.3713994976063));
#60519=CARTESIAN_POINT('Ctrl Pts',(-65.815380499579,0.450072808997186,16.5538216515551));
#60520=CARTESIAN_POINT('Ctrl Pts',(-65.6764528558945,0.580559344874713,
16.6885936485503));
#60521=CARTESIAN_POINT('Ctrl Pts',(-65.5311665204831,0.663332916123189,
16.8307690367319));
#60522=CARTESIAN_POINT('Ctrl Pts',(-65.5154842698951,0.671503698056154,
16.8461388731867));
#60523=CARTESIAN_POINT('Ctrl Pts',(-65.5,0.678562986472805,16.8613515850121));
#60524=CARTESIAN_POINT('',(-66.,-0.187087378736033,14.0612554404903));
#60525=CARTESIAN_POINT('',(-50.5,0.678562986472808,16.8613515850121));
#60526=CARTESIAN_POINT('Ctrl Pts',(-50.5,0.678562986472804,16.8613515850121));
#60527=CARTESIAN_POINT('Ctrl Pts',(-50.4432410236137,0.652686533320046,
16.8055880290214));
#60528=CARTESIAN_POINT('Ctrl Pts',(-50.3823247550295,0.611185010004192,
16.7462340757651));
#60529=CARTESIAN_POINT('Ctrl Pts',(-50.2209638885107,0.493245381173695,
16.5887724832778));
#60530=CARTESIAN_POINT('Ctrl Pts',(-50.1226787683011,0.414273762685218,
16.4926181397662));
#60531=CARTESIAN_POINT('Ctrl Pts',(-50.,0.343370775949384,16.3713994976063));
#60532=CARTESIAN_POINT('Ctrl Pts',(-65.5,0.678562986472805,16.8613515850121));
#60533=CARTESIAN_POINT('Ctrl Pts',(-60.5,0.678562986472805,16.8613515850121));
#60534=CARTESIAN_POINT('Ctrl Pts',(-55.5,0.678562986472804,16.8613515850121));
#60535=CARTESIAN_POINT('Ctrl Pts',(-50.5,0.678562986472804,16.8613515850121));
#60536=CARTESIAN_POINT('Origin',(-66.,0.,0.));
#60537=CARTESIAN_POINT('',(-66.,-1.57673047345589,13.9738265075847));
#60538=CARTESIAN_POINT('Ctrl Pts',(-66.,-3.20793490087994,17.1780318625772));
#60539=CARTESIAN_POINT('Ctrl Pts',(-50.,-3.20793490087994,17.1780318625772));
#60540=CARTESIAN_POINT('Ctrl Pts',(-66.,-3.19244707170413,17.1616979125006));
#60541=CARTESIAN_POINT('Ctrl Pts',(-50.,-3.19244707170413,17.1616979125006));
#60542=CARTESIAN_POINT('Ctrl Pts',(-66.,-3.16160672629369,17.1289704018969));
#60543=CARTESIAN_POINT('Ctrl Pts',(-50.,-3.16160672629369,17.1289704018969));
#60544=CARTESIAN_POINT('Ctrl Pts',(-66.,-3.11575214636094,17.0797003048576));
#60545=CARTESIAN_POINT('Ctrl Pts',(-50.,-3.11575214636094,17.0797003048576));
#60546=CARTESIAN_POINT('Ctrl Pts',(-66.,-3.05542566804884,17.0136487023376));
#60547=CARTESIAN_POINT('Ctrl Pts',(-50.,-3.05542566804884,17.0136487023376));
#60548=CARTESIAN_POINT('Ctrl Pts',(-66.,-2.9813781787877,16.930485139932));
#60549=CARTESIAN_POINT('Ctrl Pts',(-50.,-2.9813781787877,16.930485139932));
#60550=CARTESIAN_POINT('Ctrl Pts',(-66.,-2.90869750307329,16.8467208147344));
#60551=CARTESIAN_POINT('Ctrl Pts',(-50.,-2.90869750307329,16.8467208147344));
#60552=CARTESIAN_POINT('Ctrl Pts',(-66.,-2.83738757845593,16.7623560379061));
#60553=CARTESIAN_POINT('Ctrl Pts',(-50.,-2.83738757845593,16.7623560379061));
#60554=CARTESIAN_POINT('Ctrl Pts',(-66.,-2.7674477344443,16.6773945625569));
#60555=CARTESIAN_POINT('Ctrl Pts',(-50.,-2.7674477344443,16.6773945625569));
#60556=CARTESIAN_POINT('Ctrl Pts',(-66.,-2.69886873187661,16.5918455601692));
#60557=CARTESIAN_POINT('Ctrl Pts',(-50.,-2.69886873187661,16.5918455601692));
#60558=CARTESIAN_POINT('Ctrl Pts',(-66.,-2.63164202150355,16.5057212290741));
#60559=CARTESIAN_POINT('Ctrl Pts',(-50.,-2.63164202150355,16.5057212290741));
#60560=CARTESIAN_POINT('Ctrl Pts',(-66.,-2.56577042120647,16.4190338912104));
#60561=CARTESIAN_POINT('Ctrl Pts',(-50.,-2.56577042120647,16.4190338912104));
#60562=CARTESIAN_POINT('Ctrl Pts',(-66.,-2.50127905385604,16.3317931713189));
#60563=CARTESIAN_POINT('Ctrl Pts',(-50.,-2.50127905385604,16.3317931713189));
#60564=CARTESIAN_POINT('Ctrl Pts',(-66.,-2.43822415914769,16.244003577817));
#60565=CARTESIAN_POINT('Ctrl Pts',(-50.,-2.43822415914769,16.244003577817));
#60566=CARTESIAN_POINT('Ctrl Pts',(-66.,-2.37670786491403,16.1556609753953));
#60567=CARTESIAN_POINT('Ctrl Pts',(-50.,-2.37670786491403,16.1556609753953));
#60568=CARTESIAN_POINT('Ctrl Pts',(-66.,-2.31685613637301,16.0667562271139));
#60569=CARTESIAN_POINT('Ctrl Pts',(-50.,-2.31685613637301,16.0667562271139));
#60570=CARTESIAN_POINT('Ctrl Pts',(-66.,-2.25878765825938,15.9772806643205));
#60571=CARTESIAN_POINT('Ctrl Pts',(-50.,-2.25878765825938,15.9772806643205));
#60572=CARTESIAN_POINT('Ctrl Pts',(-66.,-2.20258303257508,15.8872314185123));
#60573=CARTESIAN_POINT('Ctrl Pts',(-50.,-2.20258303257508,15.8872314185123));
#60574=CARTESIAN_POINT('Ctrl Pts',(-66.,-2.14825922908453,15.7966159569104));
#60575=CARTESIAN_POINT('Ctrl Pts',(-50.,-2.14825922908453,15.7966159569104));
#60576=CARTESIAN_POINT('Ctrl Pts',(-66.,-2.09572657992989,15.7054594872874));
#60577=CARTESIAN_POINT('Ctrl Pts',(-50.,-2.09572657992989,15.7054594872874));
#60578=CARTESIAN_POINT('Ctrl Pts',(-66.,-2.04484013524158,15.6137968955554));
#60579=CARTESIAN_POINT('Ctrl Pts',(-50.,-2.04484013524158,15.6137968955554));
#60580=CARTESIAN_POINT('Ctrl Pts',(-66.,-1.99548217379509,15.5216595832348));
#60581=CARTESIAN_POINT('Ctrl Pts',(-50.,-1.99548217379509,15.5216595832348));
#60582=CARTESIAN_POINT('Ctrl Pts',(-66.,-1.94763938741864,15.4290632100973));
#60583=CARTESIAN_POINT('Ctrl Pts',(-50.,-1.94763938741864,15.4290632100973));
#60584=CARTESIAN_POINT('Ctrl Pts',(-66.,-1.901471233747,15.3359968987161));
#60585=CARTESIAN_POINT('Ctrl Pts',(-50.,-1.901471233747,15.3359968987161));
#60586=CARTESIAN_POINT('Ctrl Pts',(-66.,-1.85741167873706,15.2424070113801));
#60587=CARTESIAN_POINT('Ctrl Pts',(-50.,-1.85741167873706,15.2424070113801));
#60588=CARTESIAN_POINT('Ctrl Pts',(-66.,-1.81608156923822,15.1482118634974));
#60589=CARTESIAN_POINT('Ctrl Pts',(-50.,-1.81608156923822,15.1482118634974));
#60590=CARTESIAN_POINT('Ctrl Pts',(-66.,-1.77813692730802,15.0533268835806));
#60591=CARTESIAN_POINT('Ctrl Pts',(-50.,-1.77813692730802,15.0533268835806));
#60592=CARTESIAN_POINT('Ctrl Pts',(-66.,-1.74413304367239,14.957687298555));
#60593=CARTESIAN_POINT('Ctrl Pts',(-50.,-1.74413304367239,14.957687298555));
#60594=CARTESIAN_POINT('Ctrl Pts',(-66.,-1.71439340426661,14.8612698707291));
#60595=CARTESIAN_POINT('Ctrl Pts',(-50.,-1.71439340426661,14.8612698707291));
#60596=CARTESIAN_POINT('Ctrl Pts',(-66.,-1.68884359201954,14.7641208448459));
#60597=CARTESIAN_POINT('Ctrl Pts',(-50.,-1.68884359201954,14.7641208448459));
#60598=CARTESIAN_POINT('Ctrl Pts',(-66.,-1.66708743757887,14.6663413378531));
#60599=CARTESIAN_POINT('Ctrl Pts',(-50.,-1.66708743757887,14.6663413378531));
#60600=CARTESIAN_POINT('Ctrl Pts',(-66.,-1.64854533029309,14.5680618357278));
#60601=CARTESIAN_POINT('Ctrl Pts',(-50.,-1.64854533029309,14.5680618357278));
#60602=CARTESIAN_POINT('Ctrl Pts',(-66.,-1.63257174420173,14.4694202802978));
#60603=CARTESIAN_POINT('Ctrl Pts',(-50.,-1.63257174420173,14.4694202802978));
#60604=CARTESIAN_POINT('Ctrl Pts',(-66.,-1.61857609759037,14.3705396469258));
#60605=CARTESIAN_POINT('Ctrl Pts',(-50.,-1.61857609759037,14.3705396469258));
#60606=CARTESIAN_POINT('Ctrl Pts',(-66.,-1.60615369222193,14.2715034719842));
#60607=CARTESIAN_POINT('Ctrl Pts',(-50.,-1.60615369222193,14.2715034719842));
#60608=CARTESIAN_POINT('Ctrl Pts',(-66.,-1.59506091439902,14.1723615147133));
#60609=CARTESIAN_POINT('Ctrl Pts',(-50.,-1.59506091439902,14.1723615147133));
#60610=CARTESIAN_POINT('Ctrl Pts',(-66.,-1.58714954409268,14.0929835088213));
#60611=CARTESIAN_POINT('Ctrl Pts',(-50.,-1.58714954409268,14.0929835088213));
#60612=CARTESIAN_POINT('Ctrl Pts',(-66.,-1.58173749645856,14.0334175928621));
#60613=CARTESIAN_POINT('Ctrl Pts',(-50.,-1.58173749645856,14.0334175928621));
#60614=CARTESIAN_POINT('Ctrl Pts',(-66.,-1.57836090671277,13.9936925998767));
#60615=CARTESIAN_POINT('Ctrl Pts',(-50.,-1.57836090671277,13.9936925998767));
#60616=CARTESIAN_POINT('Ctrl Pts',(-66.,-1.57673047345591,13.9738265075847));
#60617=CARTESIAN_POINT('Ctrl Pts',(-50.,-1.57673047345591,13.9738265075847));
#60618=CARTESIAN_POINT('Origin',(-65.75,0.,0.));
#60619=CARTESIAN_POINT('',(-65.5,1.48114719470812,16.8098729319293));
#60620=CARTESIAN_POINT('Origin',(-65.5,0.,0.));
#60621=CARTESIAN_POINT('Ctrl Pts',(-65.5,1.48114719470739,16.8098729319309));
#60622=CARTESIAN_POINT('Ctrl Pts',(-65.5830891893357,1.52065903745123,16.7229860401592));
#60623=CARTESIAN_POINT('Ctrl Pts',(-65.6667904343355,1.55870578833828,16.6354130562452));
#60624=CARTESIAN_POINT('Ctrl Pts',(-65.7503687595015,1.59493615732831,16.5479535315511));
#60625=CARTESIAN_POINT('Ctrl Pts',(-65.8133591842207,1.62224187715319,16.4820379655801));
#60626=CARTESIAN_POINT('Ctrl Pts',(-65.8762797883185,1.64851836527279,16.4161878541729));
#60627=CARTESIAN_POINT('Ctrl Pts',(-65.9388159306751,1.6735755621829,16.3507588674798));
#60628=CARTESIAN_POINT('Ctrl Pts',(-65.959255352681,1.68176530019086,16.3293739431778));
#60629=CARTESIAN_POINT('Ctrl Pts',(-65.9796537043586,1.68982432280954,16.3080340818493));
#60630=CARTESIAN_POINT('Ctrl Pts',(-66.,1.69774526472952,16.2867518559131));
#60631=CARTESIAN_POINT('Origin',(-58.,0.,0.));
#60632=CARTESIAN_POINT('',(-50.5,1.48114719470812,16.8098729319293));
#60633=CARTESIAN_POINT('Origin',(-50.5,0.,0.));
#60634=CARTESIAN_POINT('Ctrl Pts',(-50.5,1.48114719470812,16.8098729319293));
#60635=CARTESIAN_POINT('Ctrl Pts',(-55.5,1.48114719470812,16.8098729319293));
#60636=CARTESIAN_POINT('Ctrl Pts',(-60.5,1.48114719470812,16.8098729319293));
#60637=CARTESIAN_POINT('Ctrl Pts',(-65.5,1.48114719470812,16.8098729319293));
#60638=CARTESIAN_POINT('Origin',(-50.25,0.,0.));
#60639=CARTESIAN_POINT('Ctrl Pts',(-50.,1.69774526472952,16.2867518559131));
#60640=CARTESIAN_POINT('Ctrl Pts',(-50.0661278995916,1.67200125406601,16.3559216411457));
#60641=CARTESIAN_POINT('Ctrl Pts',(-50.132805681623,1.64480114704281,16.4256996735367));
#60642=CARTESIAN_POINT('Ctrl Pts',(-50.1996561856134,1.61638854466487,16.4956567269383));
#60643=CARTESIAN_POINT('Ctrl Pts',(-50.275508769232,1.58414990517748,16.5750341874825));
#60644=CARTESIAN_POINT('Ctrl Pts',(-50.3515837242552,1.55034920906213,16.6546411368507));
#60645=CARTESIAN_POINT('Ctrl Pts',(-50.4273300866396,1.51525802335958,16.7338710346662));
#60646=CARTESIAN_POINT('Ctrl Pts',(-50.4515931423099,1.5040176236171,16.7592499355262));
#60647=CARTESIAN_POINT('Ctrl Pts',(-50.4758224828177,1.49264445763884,16.7845903490235));
#60648=CARTESIAN_POINT('Ctrl Pts',(-50.5,1.48114719470371,16.809872931939));
#60649=CARTESIAN_POINT('Ctrl Pts',(-66.,3.31568234418832,13.6660219830951));
#60650=CARTESIAN_POINT('Ctrl Pts',(-50.,3.31568234418832,13.6660219830951));
#60651=CARTESIAN_POINT('Ctrl Pts',(-66.,3.32025508218772,13.6889423777435));
#60652=CARTESIAN_POINT('Ctrl Pts',(-50.,3.32025508218772,13.6889423777435));
#60653=CARTESIAN_POINT('Ctrl Pts',(-66.,3.32962290369722,13.7347480949923));
#60654=CARTESIAN_POINT('Ctrl Pts',(-50.,3.32962290369722,13.7347480949923));
#60655=CARTESIAN_POINT('Ctrl Pts',(-66.,3.34434166251121,13.8033514635997));
#60656=CARTESIAN_POINT('Ctrl Pts',(-50.,3.34434166251121,13.8033514635997));
#60657=CARTESIAN_POINT('Ctrl Pts',(-66.,3.36530258749166,13.8946118507282));
#60658=CARTESIAN_POINT('Ctrl Pts',(-50.,3.36530258749166,13.8946118507282));
#60659=CARTESIAN_POINT('Ctrl Pts',(-66.,3.39378048711278,14.0083089910501));
#60660=CARTESIAN_POINT('Ctrl Pts',(-50.,3.39378048711278,14.0083089910501));
#60661=CARTESIAN_POINT('Ctrl Pts',(-66.,3.42466963349977,14.1215479032503));
#60662=CARTESIAN_POINT('Ctrl Pts',(-50.,3.42466963349977,14.1215479032503));
#60663=CARTESIAN_POINT('Ctrl Pts',(-66.,3.45822302631379,14.2341732241738));
#60664=CARTESIAN_POINT('Ctrl Pts',(-50.,3.45822302631379,14.2341732241738));
#60665=CARTESIAN_POINT('Ctrl Pts',(-66.,3.49485794879717,14.3459208356842));
#60666=CARTESIAN_POINT('Ctrl Pts',(-50.,3.49485794879717,14.3459208356842));
#60667=CARTESIAN_POINT('Ctrl Pts',(-66.,3.53511610244324,14.4564721136477));
#60668=CARTESIAN_POINT('Ctrl Pts',(-50.,3.53511610244324,14.4564721136477));
#60669=CARTESIAN_POINT('Ctrl Pts',(-66.,3.57961415137445,14.5655275456869));
#60670=CARTESIAN_POINT('Ctrl Pts',(-50.,3.57961415137445,14.5655275456869));
#60671=CARTESIAN_POINT('Ctrl Pts',(-66.,3.62898699781003,14.6728671135607));
#60672=CARTESIAN_POINT('Ctrl Pts',(-50.,3.62898699781003,14.6728671135607));
#60673=CARTESIAN_POINT('Ctrl Pts',(-66.,3.68386053504292,14.7784329430806));
#60674=CARTESIAN_POINT('Ctrl Pts',(-50.,3.68386053504292,14.7784329430806));
#60675=CARTESIAN_POINT('Ctrl Pts',(-66.,3.74465444426779,14.8823190942953));
#60676=CARTESIAN_POINT('Ctrl Pts',(-50.,3.74465444426779,14.8823190942953));
#60677=CARTESIAN_POINT('Ctrl Pts',(-66.,3.81125317193191,14.9847182617076));
#60678=CARTESIAN_POINT('Ctrl Pts',(-50.,3.81125317193191,14.9847182617076));
#60679=CARTESIAN_POINT('Ctrl Pts',(-66.,3.88279556209739,15.0858821011164));
#60680=CARTESIAN_POINT('Ctrl Pts',(-50.,3.88279556209739,15.0858821011164));
#60681=CARTESIAN_POINT('Ctrl Pts',(-66.,3.95722328533246,15.1860781064647));
#60682=CARTESIAN_POINT('Ctrl Pts',(-50.,3.95722328533246,15.1860781064647));
#60683=CARTESIAN_POINT('Ctrl Pts',(-66.,4.03163457417435,15.2855414194547));
#60684=CARTESIAN_POINT('Ctrl Pts',(-50.,4.03163457417435,15.2855414194547));
#60685=CARTESIAN_POINT('Ctrl Pts',(-66.,4.10369589439471,15.3844104249513));
#60686=CARTESIAN_POINT('Ctrl Pts',(-50.,4.10369589439471,15.3844104249513));
#60687=CARTESIAN_POINT('Ctrl Pts',(-66.,4.17266875139903,15.482674151341));
#60688=CARTESIAN_POINT('Ctrl Pts',(-50.,4.17266875139903,15.482674151341));
#60689=CARTESIAN_POINT('Ctrl Pts',(-66.,4.24085733833789,15.5800968628044));
#60690=CARTESIAN_POINT('Ctrl Pts',(-50.,4.24085733833789,15.5800968628044));
#60691=CARTESIAN_POINT('Ctrl Pts',(-66.,4.31412149748944,15.6762031957635));
#60692=CARTESIAN_POINT('Ctrl Pts',(-50.,4.31412149748944,15.6762031957635));
#60693=CARTESIAN_POINT('Ctrl Pts',(-66.,4.3986379872848,15.7705164726843));
#60694=CARTESIAN_POINT('Ctrl Pts',(-50.,4.3986379872848,15.7705164726843));
#60695=CARTESIAN_POINT('Ctrl Pts',(-66.,4.4981307922185,15.862765781002));
#60696=CARTESIAN_POINT('Ctrl Pts',(-50.,4.4981307922185,15.862765781002));
#60697=CARTESIAN_POINT('Ctrl Pts',(-66.,4.61104471950514,15.9530958995951));
#60698=CARTESIAN_POINT('Ctrl Pts',(-50.,4.61104471950514,15.9530958995951));
#60699=CARTESIAN_POINT('Ctrl Pts',(-66.,4.72735495944251,16.0423056749486));
#60700=CARTESIAN_POINT('Ctrl Pts',(-50.,4.72735495944251,16.0423056749486));
#60701=CARTESIAN_POINT('Ctrl Pts',(-66.,4.83101568214621,16.1316580433923));
#60702=CARTESIAN_POINT('Ctrl Pts',(-50.,4.83101568214621,16.1316580433923));
#60703=CARTESIAN_POINT('Ctrl Pts',(-66.,4.9030763374662,16.2226394544667));
#60704=CARTESIAN_POINT('Ctrl Pts',(-50.,4.9030763374662,16.2226394544667));
#60705=CARTESIAN_POINT('Ctrl Pts',(-66.,4.92433124236172,16.3167550432627));
#60706=CARTESIAN_POINT('Ctrl Pts',(-50.,4.92433124236172,16.3167550432627));
#60707=CARTESIAN_POINT('Ctrl Pts',(-66.,4.87866379252586,16.4152704420741));
#60708=CARTESIAN_POINT('Ctrl Pts',(-50.,4.87866379252586,16.4152704420741));
#60709=CARTESIAN_POINT('Ctrl Pts',(-66.,4.75394565180326,16.5191420918161));
#60710=CARTESIAN_POINT('Ctrl Pts',(-50.,4.75394565180326,16.5191420918161));
#60711=CARTESIAN_POINT('Ctrl Pts',(-66.,4.54114089813183,16.629086018864));
#60712=CARTESIAN_POINT('Ctrl Pts',(-50.,4.54114089813183,16.629086018864));
#60713=CARTESIAN_POINT('Ctrl Pts',(-66.,4.23395401208117,16.7456047287692));
#60714=CARTESIAN_POINT('Ctrl Pts',(-50.,4.23395401208117,16.7456047287692));
#60715=CARTESIAN_POINT('Ctrl Pts',(-66.,3.82828013317778,16.8690293990345));
#60716=CARTESIAN_POINT('Ctrl Pts',(-50.,3.82828013317778,16.8690293990345));
#60717=CARTESIAN_POINT('Ctrl Pts',(-66.,3.32176445468909,16.9995537049453));
#60718=CARTESIAN_POINT('Ctrl Pts',(-50.,3.32176445468909,16.9995537049453));
#60719=CARTESIAN_POINT('Ctrl Pts',(-66.,2.7133369168573,17.1372695974412));
#60720=CARTESIAN_POINT('Ctrl Pts',(-50.,2.7133369168573,17.1372695974412));
#60721=CARTESIAN_POINT('Ctrl Pts',(-66.,2.14488947489857,17.2532145262309));
#60722=CARTESIAN_POINT('Ctrl Pts',(-50.,2.14488947489857,17.2532145262309));
#60723=CARTESIAN_POINT('Ctrl Pts',(-66.,1.67268460782871,17.3434149530381));
#60724=CARTESIAN_POINT('Ctrl Pts',(-50.,1.67268460782871,17.3434149530381));
#60725=CARTESIAN_POINT('Ctrl Pts',(-66.,1.33752212890223,17.4049874234484));
#60726=CARTESIAN_POINT('Ctrl Pts',(-50.,1.33752212890223,17.4049874234484));
#60727=CARTESIAN_POINT('Ctrl Pts',(-66.,1.16485107862945,17.4361333719554));
#60728=CARTESIAN_POINT('Ctrl Pts',(-50.,1.16485107862945,17.4361333719554));
#60729=CARTESIAN_POINT('',(-65.5,4.85049230558631,16.1628694665721));
#60730=CARTESIAN_POINT('Ctrl Pts',(-66.,4.40398464539872,15.7716690379646));
#60731=CARTESIAN_POINT('Ctrl Pts',(-65.7933280154034,4.57046489538325,15.9397601433951));
#60732=CARTESIAN_POINT('Ctrl Pts',(-65.637076174949,4.75647091834925,16.0479696685658));
#60733=CARTESIAN_POINT('Ctrl Pts',(-65.5,4.85049230558631,16.1628694665721));
#60734=CARTESIAN_POINT('',(-66.,3.31568234418832,13.6660219830951));
#60735=CARTESIAN_POINT('',(-50.5,4.85049230558631,16.1628694665721));
#60736=CARTESIAN_POINT('Ctrl Pts',(-50.5,4.85049230558631,16.1628694665721));
#60737=CARTESIAN_POINT('Ctrl Pts',(-50.4457232578825,4.81326355602069,16.1173736923571));
#60738=CARTESIAN_POINT('Ctrl Pts',(-50.3881125476901,4.76170358838096,16.0726383675736));
#60739=CARTESIAN_POINT('Ctrl Pts',(-50.2297317785044,4.61214589079611,15.951491103014));
#60740=CARTESIAN_POINT('Ctrl Pts',(-50.1279794591276,4.50707579435166,15.8757576922597));
#60741=CARTESIAN_POINT('Ctrl Pts',(-50.,4.40398464539871,15.7716690379646));
#60742=CARTESIAN_POINT('Ctrl Pts',(-65.5,4.85049230558631,16.1628694665721));
#60743=CARTESIAN_POINT('Ctrl Pts',(-60.5,4.85049230558631,16.1628694665721));
#60744=CARTESIAN_POINT('Ctrl Pts',(-55.5,4.85049230558631,16.1628694665721));
#60745=CARTESIAN_POINT('Ctrl Pts',(-50.5,4.85049230558631,16.1628694665721));
#60746=CARTESIAN_POINT('Origin',(-66.,0.,0.));
#60747=CARTESIAN_POINT('',(-66.,1.94795475120473,13.9269299753125));
#60748=CARTESIAN_POINT('Ctrl Pts',(-66.,1.16485107862945,17.4361333719554));
#60749=CARTESIAN_POINT('Ctrl Pts',(-50.,1.16485107862945,17.4361333719554));
#60750=CARTESIAN_POINT('Ctrl Pts',(-66.,1.17579024097006,17.4164609164663));
#60751=CARTESIAN_POINT('Ctrl Pts',(-50.,1.17579024097006,17.4164609164663));
#60752=CARTESIAN_POINT('Ctrl Pts',(-66.,1.19752267929878,17.3770919187696));
#60753=CARTESIAN_POINT('Ctrl Pts',(-50.,1.19752267929878,17.3770919187696));
#60754=CARTESIAN_POINT('Ctrl Pts',(-66.,1.22968367840899,17.3179661621208));
#60755=CARTESIAN_POINT('Ctrl Pts',(-50.,1.22968367840899,17.3179661621208));
#60756=CARTESIAN_POINT('Ctrl Pts',(-66.,1.2716885238945,17.2389871070698));
#60757=CARTESIAN_POINT('Ctrl Pts',(-50.,1.2716885238945,17.2389871070698));
#60758=CARTESIAN_POINT('Ctrl Pts',(-66.,1.32272773816582,17.1400214191551));
#60759=CARTESIAN_POINT('Ctrl Pts',(-50.,1.32272773816582,17.1400214191551));
#60760=CARTESIAN_POINT('Ctrl Pts',(-66.,1.37229367622044,17.040813755223));
#60761=CARTESIAN_POINT('Ctrl Pts',(-50.,1.37229367622044,17.040813755223));
#60762=CARTESIAN_POINT('Ctrl Pts',(-66.,1.42038260159604,16.9413653958879));
#60763=CARTESIAN_POINT('Ctrl Pts',(-50.,1.42038260159604,16.9413653958879));
#60764=CARTESIAN_POINT('Ctrl Pts',(-66.,1.46699609707973,16.8416798096044));
#60765=CARTESIAN_POINT('Ctrl Pts',(-50.,1.46699609707973,16.8416798096044));
#60766=CARTESIAN_POINT('Ctrl Pts',(-66.,1.51214539242291,16.7417635820299));
#60767=CARTESIAN_POINT('Ctrl Pts',(-50.,1.51214539242291,16.7417635820299));
#60768=CARTESIAN_POINT('Ctrl Pts',(-66.,1.55584180188614,16.6416264021506));
#60769=CARTESIAN_POINT('Ctrl Pts',(-50.,1.55584180188614,16.6416264021506));
#60770=CARTESIAN_POINT('Ctrl Pts',(-66.,1.59808566045853,16.5412809055674));
#60771=CARTESIAN_POINT('Ctrl Pts',(-50.,1.59808566045853,16.5412809055674));
#60772=CARTESIAN_POINT('Ctrl Pts',(-66.,1.63885502812633,16.4407426624463));
#60773=CARTESIAN_POINT('Ctrl Pts',(-50.,1.63885502812633,16.4407426624463));
#60774=CARTESIAN_POINT('Ctrl Pts',(-66.,1.67809655326534,16.3400300258078));
#60775=CARTESIAN_POINT('Ctrl Pts',(-50.,1.67809655326534,16.3400300258078));
#60776=CARTESIAN_POINT('Ctrl Pts',(-66.,1.71571028816699,16.2391643884201));
#60777=CARTESIAN_POINT('Ctrl Pts',(-50.,1.71571028816699,16.2391643884201));
#60778=CARTESIAN_POINT('Ctrl Pts',(-66.,1.75157195277774,16.1381682266729));
#60779=CARTESIAN_POINT('Ctrl Pts',(-50.,1.75157195277774,16.1381682266729));
#60780=CARTESIAN_POINT('Ctrl Pts',(-66.,1.78556443525587,16.0370626599488));
#60781=CARTESIAN_POINT('Ctrl Pts',(-50.,1.78556443525587,16.0370626599488));
#60782=CARTESIAN_POINT('Ctrl Pts',(-66.,1.8176089524919,15.9358649547671));
#60783=CARTESIAN_POINT('Ctrl Pts',(-50.,1.8176089524919,15.9358649547671));
#60784=CARTESIAN_POINT('Ctrl Pts',(-66.,1.84769092488014,15.8345865639611));
#60785=CARTESIAN_POINT('Ctrl Pts',(-50.,1.84769092488014,15.8345865639611));
#60786=CARTESIAN_POINT('Ctrl Pts',(-66.,1.87590347211591,15.7332296038656));
#60787=CARTESIAN_POINT('Ctrl Pts',(-50.,1.87590347211591,15.7332296038656));
#60788=CARTESIAN_POINT('Ctrl Pts',(-66.,1.90239566597564,15.6317918168208));
#60789=CARTESIAN_POINT('Ctrl Pts',(-50.,1.90239566597564,15.6317918168208));
#60790=CARTESIAN_POINT('Ctrl Pts',(-66.,1.92728933849566,15.5302743417326));
#60791=CARTESIAN_POINT('Ctrl Pts',(-50.,1.92728933849566,15.5302743417326));
#60792=CARTESIAN_POINT('Ctrl Pts',(-66.,1.95060127417394,15.4286890367845));
#60793=CARTESIAN_POINT('Ctrl Pts',(-50.,1.95060127417394,15.4286890367845));
#60794=CARTESIAN_POINT('Ctrl Pts',(-66.,1.97217431992445,15.3270650217851));
#60795=CARTESIAN_POINT('Ctrl Pts',(-50.,1.97217431992445,15.3270650217851));
#60796=CARTESIAN_POINT('Ctrl Pts',(-66.,1.99157480447254,15.2254582670956));
#60797=CARTESIAN_POINT('Ctrl Pts',(-50.,1.99157480447254,15.2254582670956));
#60798=CARTESIAN_POINT('Ctrl Pts',(-66.,2.00818107188229,15.1239440527286));
#60799=CARTESIAN_POINT('Ctrl Pts',(-50.,2.00818107188229,15.1239440527286));
#60800=CARTESIAN_POINT('Ctrl Pts',(-66.,2.02133667816179,15.022603610217));
#60801=CARTESIAN_POINT('Ctrl Pts',(-50.,2.02133667816179,15.022603610217));
#60802=CARTESIAN_POINT('Ctrl Pts',(-66.,2.03048766965571,14.9215122966393));
#60803=CARTESIAN_POINT('Ctrl Pts',(-50.,2.03048766965571,14.9215122966393));
#60804=CARTESIAN_POINT('Ctrl Pts',(-66.,2.03531494435546,14.8207280520398));
#60805=CARTESIAN_POINT('Ctrl Pts',(-50.,2.03531494435546,14.8207280520398));
#60806=CARTESIAN_POINT('Ctrl Pts',(-66.,2.03590208198289,14.7202771615244));
#60807=CARTESIAN_POINT('Ctrl Pts',(-50.,2.03590208198289,14.7202771615244));
#60808=CARTESIAN_POINT('Ctrl Pts',(-66.,2.03265795226397,14.6201590419547));
#60809=CARTESIAN_POINT('Ctrl Pts',(-50.,2.03265795226397,14.6201590419547));
#60810=CARTESIAN_POINT('Ctrl Pts',(-66.,2.02617640685866,14.5203559365434));
#60811=CARTESIAN_POINT('Ctrl Pts',(-50.,2.02617640685866,14.5203559365434));
#60812=CARTESIAN_POINT('Ctrl Pts',(-66.,2.01711699607993,14.4208409176437));
#60813=CARTESIAN_POINT('Ctrl Pts',(-50.,2.01711699607993,14.4208409176437));
#60814=CARTESIAN_POINT('Ctrl Pts',(-66.,2.00608233016073,14.3215862254212));
#60815=CARTESIAN_POINT('Ctrl Pts',(-50.,2.00608233016073,14.3215862254212));
#60816=CARTESIAN_POINT('Ctrl Pts',(-66.,1.99348516764985,14.2225721274408));
#60817=CARTESIAN_POINT('Ctrl Pts',(-50.,1.99348516764985,14.2225721274408));
#60818=CARTESIAN_POINT('Ctrl Pts',(-66.,1.97957384329226,14.1237862354018));
#60819=CARTESIAN_POINT('Ctrl Pts',(-50.,1.97957384329226,14.1237862354018));
#60820=CARTESIAN_POINT('Ctrl Pts',(-66.,1.96749615602378,14.044934557742));
#60821=CARTESIAN_POINT('Ctrl Pts',(-50.,1.96749615602378,14.044934557742));
#60822=CARTESIAN_POINT('Ctrl Pts',(-66.,1.95792473331065,13.9858940930512));
#60823=CARTESIAN_POINT('Ctrl Pts',(-50.,1.95792473331065,13.9858940930512));
#60824=CARTESIAN_POINT('Ctrl Pts',(-66.,1.9513160372573,13.9465774100468));
#60825=CARTESIAN_POINT('Ctrl Pts',(-50.,1.9513160372573,13.9465774100468));
#60826=CARTESIAN_POINT('Ctrl Pts',(-66.,1.94795475120472,13.9269299753125));
#60827=CARTESIAN_POINT('Ctrl Pts',(-50.,1.94795475120472,13.9269299753125));
#60828=CARTESIAN_POINT('Origin',(-65.75,0.,0.));
#60829=CARTESIAN_POINT('',(-65.5,5.61505963464423,15.9134135338522));
#60830=CARTESIAN_POINT('Origin',(-65.5,0.,0.));
#60831=CARTESIAN_POINT('Ctrl Pts',(-65.5,5.61505963464423,15.9134135338522));
#60832=CARTESIAN_POINT('Ctrl Pts',(-65.6931595476746,5.65379827034173,15.6949131405067));
#60833=CARTESIAN_POINT('Ctrl Pts',(-65.861125696709,5.67851717118329,15.507005686362));
#60834=CARTESIAN_POINT('Ctrl Pts',(-66.,5.69475795663189,15.3528615187976));
#60835=CARTESIAN_POINT('Origin',(-58.,0.,0.));
#60836=CARTESIAN_POINT('',(-50.5,5.61505963464423,15.9134135338522));
#60837=CARTESIAN_POINT('Origin',(-50.5,0.,0.));
#60838=CARTESIAN_POINT('Ctrl Pts',(-50.5,5.61505963464423,15.9134135338522));
#60839=CARTESIAN_POINT('Ctrl Pts',(-55.5,5.61505963464423,15.9134135338522));
#60840=CARTESIAN_POINT('Ctrl Pts',(-60.5,5.61505963464423,15.9134135338522));
#60841=CARTESIAN_POINT('Ctrl Pts',(-65.5,5.61505963464423,15.9134135338522));
#60842=CARTESIAN_POINT('Origin',(-50.25,0.,0.));
#60843=CARTESIAN_POINT('Ctrl Pts',(-50.,5.69475795663189,15.3528615187977));
#60844=CARTESIAN_POINT('Ctrl Pts',(-50.1388743032898,5.67851717118344,15.5070056863606));
#60845=CARTESIAN_POINT('Ctrl Pts',(-50.3068404523242,5.65379827034194,15.6949131405054));
#60846=CARTESIAN_POINT('Ctrl Pts',(-50.5,5.61505963464423,15.9134135338522));
#60847=CARTESIAN_POINT('Ctrl Pts',(-66.,6.61011555120064,12.4121021043889));
#60848=CARTESIAN_POINT('Ctrl Pts',(-50.,6.61011555120064,12.4121021043889));
#60849=CARTESIAN_POINT('Ctrl Pts',(-66.,6.62024469858602,12.4331652189947));
#60850=CARTESIAN_POINT('Ctrl Pts',(-50.,6.62024469858602,12.4331652189947));
#60851=CARTESIAN_POINT('Ctrl Pts',(-66.,6.64070963141069,12.4752021829311));
#60852=CARTESIAN_POINT('Ctrl Pts',(-50.,6.64070963141069,12.4752021829311));
#60853=CARTESIAN_POINT('Ctrl Pts',(-66.,6.67202693734873,12.5379898440923));
#60854=CARTESIAN_POINT('Ctrl Pts',(-50.,6.67202693734873,12.5379898440923));
#60855=CARTESIAN_POINT('Ctrl Pts',(-66.,6.71502487170408,12.6211703482748));
#60856=CARTESIAN_POINT('Ctrl Pts',(-50.,6.71502487170408,12.6211703482748));
#60857=CARTESIAN_POINT('Ctrl Pts',(-66.,6.77088341473902,12.7242133182155));
#60858=CARTESIAN_POINT('Ctrl Pts',(-50.,6.77088341473902,12.7242133182155));
#60859=CARTESIAN_POINT('Ctrl Pts',(-66.,6.82896349408885,12.8262128034276));
#60860=CARTESIAN_POINT('Ctrl Pts',(-50.,6.82896349408885,12.8262128034276));
#60861=CARTESIAN_POINT('Ctrl Pts',(-66.,6.88947152371961,12.9269554033179));
#60862=CARTESIAN_POINT('Ctrl Pts',(-50.,6.88947152371961,12.9269554033179));
#60863=CARTESIAN_POINT('Ctrl Pts',(-66.,6.95274599364373,13.0260815233846));
#60864=CARTESIAN_POINT('Ctrl Pts',(-50.,6.95274599364373,13.0260815233846));
#60865=CARTESIAN_POINT('Ctrl Pts',(-66.,7.01923234820612,13.1231478339735));
#60866=CARTESIAN_POINT('Ctrl Pts',(-50.,7.01923234820612,13.1231478339735));
#60867=CARTESIAN_POINT('Ctrl Pts',(-66.,7.08945339219251,13.2177108743086));
#60868=CARTESIAN_POINT('Ctrl Pts',(-50.,7.08945339219251,13.2177108743086));
#60869=CARTESIAN_POINT('Ctrl Pts',(-66.,7.16396936488986,13.3093996446649));
#60870=CARTESIAN_POINT('Ctrl Pts',(-50.,7.16396936488986,13.3093996446649));
#60871=CARTESIAN_POINT('Ctrl Pts',(-66.,7.24337210327696,13.3980024357456));
#60872=CARTESIAN_POINT('Ctrl Pts',(-50.,7.24337210327696,13.3980024357456));
#60873=CARTESIAN_POINT('Ctrl Pts',(-66.,7.32809149527493,13.4835059820612));
#60874=CARTESIAN_POINT('Ctrl Pts',(-50.,7.32809149527493,13.4835059820612));
#60875=CARTESIAN_POINT('Ctrl Pts',(-66.,7.41806353883254,13.5661256612623));
#60876=CARTESIAN_POINT('Ctrl Pts',(-50.,7.41806353883254,13.5661256612623));
#60877=CARTESIAN_POINT('Ctrl Pts',(-66.,7.51251671706145,13.646319383691));
#60878=CARTESIAN_POINT('Ctrl Pts',(-50.,7.51251671706145,13.646319383691));
#60879=CARTESIAN_POINT('Ctrl Pts',(-66.,7.60952388977251,13.7248581251904));
#60880=CARTESIAN_POINT('Ctrl Pts',(-50.,7.60952388977251,13.7248581251904));
#60881=CARTESIAN_POINT('Ctrl Pts',(-66.,7.70633293122716,13.8026912802767));
#60882=CARTESIAN_POINT('Ctrl Pts',(-50.,7.70633293122716,13.8026912802767));
#60883=CARTESIAN_POINT('Ctrl Pts',(-66.,7.80071803438238,13.8805332125637));
#60884=CARTESIAN_POINT('Ctrl Pts',(-50.,7.80071803438238,13.8805332125637));
#60885=CARTESIAN_POINT('Ctrl Pts',(-66.,7.89196117727994,13.9585569512687));
#60886=CARTESIAN_POINT('Ctrl Pts',(-50.,7.89196117727994,13.9585569512687));
#60887=CARTESIAN_POINT('Ctrl Pts',(-66.,7.9822355374912,14.0359611371119));
#60888=CARTESIAN_POINT('Ctrl Pts',(-50.,7.9822355374912,14.0359611371119));
#60889=CARTESIAN_POINT('Ctrl Pts',(-66.,8.07709864145905,14.1108280574212));
#60890=CARTESIAN_POINT('Ctrl Pts',(-50.,8.07709864145905,14.1108280574212));
#60891=CARTESIAN_POINT('Ctrl Pts',(-66.,8.18241464850812,14.1811599130068));
#60892=CARTESIAN_POINT('Ctrl Pts',(-50.,8.18241464850812,14.1811599130068));
#60893=CARTESIAN_POINT('Ctrl Pts',(-66.,8.30172317409692,14.2457681852364));
#60894=CARTESIAN_POINT('Ctrl Pts',(-50.,8.30172317409692,14.2457681852364));
#60895=CARTESIAN_POINT('Ctrl Pts',(-66.,8.43355388972419,14.3051798652122));
#60896=CARTESIAN_POINT('Ctrl Pts',(-50.,8.43355388972419,14.3051798652122));
#60897=CARTESIAN_POINT('Ctrl Pts',(-66.,8.56839559856102,14.3626617709815));
#60898=CARTESIAN_POINT('Ctrl Pts',(-50.,8.56839559856102,14.3626617709815));
#60899=CARTESIAN_POINT('Ctrl Pts',(-66.,8.69102065946842,14.4234275970304));
#60900=CARTESIAN_POINT('Ctrl Pts',(-50.,8.69102065946842,14.4234275970304));
#60901=CARTESIAN_POINT('Ctrl Pts',(-66.,8.78344355364544,14.4936299035323));
#60902=CARTESIAN_POINT('Ctrl Pts',(-50.,8.78344355364544,14.4936299035323));
#60903=CARTESIAN_POINT('Ctrl Pts',(-66.,8.82743629177677,14.5795027981396));
#60904=CARTESIAN_POINT('Ctrl Pts',(-50.,8.82743629177677,14.5795027981396));
#60905=CARTESIAN_POINT('Ctrl Pts',(-66.,8.80770335226846,14.686280187487));
#60906=CARTESIAN_POINT('Ctrl Pts',(-50.,8.80770335226846,14.686280187487));
#60907=CARTESIAN_POINT('Ctrl Pts',(-66.,8.71273529013126,14.8179046586894));
#60908=CARTESIAN_POINT('Ctrl Pts',(-50.,8.71273529013126,14.8179046586894));
#60909=CARTESIAN_POINT('Ctrl Pts',(-66.,8.53395813192898,14.9773168852751));
#60910=CARTESIAN_POINT('Ctrl Pts',(-50.,8.53395813192898,14.9773168852751));
#60911=CARTESIAN_POINT('Ctrl Pts',(-66.,8.2653991115997,15.1665692176762));
#60912=CARTESIAN_POINT('Ctrl Pts',(-50.,8.2653991115997,15.1665692176762));
#60913=CARTESIAN_POINT('Ctrl Pts',(-66.,7.90316469090577,15.3870032661332));
#60914=CARTESIAN_POINT('Ctrl Pts',(-50.,7.90316469090577,15.3870032661332));
#60915=CARTESIAN_POINT('Ctrl Pts',(-66.,7.44502220878323,15.639392237887));
#60916=CARTESIAN_POINT('Ctrl Pts',(-50.,7.44502220878323,15.639392237887));
#60917=CARTESIAN_POINT('Ctrl Pts',(-66.,6.889958090638,15.9240913081097));
#60918=CARTESIAN_POINT('Ctrl Pts',(-50.,6.889958090638,15.9240913081097));
#60919=CARTESIAN_POINT('Ctrl Pts',(-66.,6.36820380162818,16.1777607439535));
#60920=CARTESIAN_POINT('Ctrl Pts',(-50.,6.36820380162818,16.1777607439535));
#60921=CARTESIAN_POINT('Ctrl Pts',(-66.,5.93326605274623,16.3825599335959));
#60922=CARTESIAN_POINT('Ctrl Pts',(-50.,5.93326605274623,16.3825599335959));
#60923=CARTESIAN_POINT('Ctrl Pts',(-66.,5.62394577013471,16.5255495106905));
#60924=CARTESIAN_POINT('Ctrl Pts',(-50.,5.62394577013471,16.5255495106905));
#60925=CARTESIAN_POINT('Ctrl Pts',(-66.,5.46444518084595,16.5986584959607));
#60926=CARTESIAN_POINT('Ctrl Pts',(-50.,5.46444518084595,16.5986584959607));
#60927=CARTESIAN_POINT('',(-65.5,8.71764735427698,14.4488148166716));
#60928=CARTESIAN_POINT('Ctrl Pts',(-66.,8.1878799628551,14.1809466085264));
#60929=CARTESIAN_POINT('Ctrl Pts',(-65.7933280154035,8.3909324876934,14.3023548681979));
#60930=CARTESIAN_POINT('Ctrl Pts',(-65.637076174949,8.59800540401177,14.3609069752887));
#60931=CARTESIAN_POINT('Ctrl Pts',(-65.5,8.71764735427698,14.4488148166716));
#60932=CARTESIAN_POINT('',(-66.,6.61011555120064,12.4121021043889));
#60933=CARTESIAN_POINT('',(-50.5,8.71764735427698,14.4488148166716));
#60934=CARTESIAN_POINT('Ctrl Pts',(-50.5,8.71764735427698,14.4488148166716));
#60935=CARTESIAN_POINT('Ctrl Pts',(-50.4518618349118,8.67563170892152,14.4179434987156));
#60936=CARTESIAN_POINT('Ctrl Pts',(-50.4012423593878,8.62299967613232,14.3905314785402));
#60937=CARTESIAN_POINT('Ctrl Pts',(-50.2441129793791,8.45124686345708,14.3100121728929));
#60938=CARTESIAN_POINT('Ctrl Pts',(-50.1366827452935,8.32216897443961,14.2612400951623));
#60939=CARTESIAN_POINT('Ctrl Pts',(-50.,8.1878799628551,14.1809466085264));
#60940=CARTESIAN_POINT('Ctrl Pts',(-65.5,8.71764735427698,14.4488148166716));
#60941=CARTESIAN_POINT('Ctrl Pts',(-60.5,8.71764735427698,14.4488148166716));
#60942=CARTESIAN_POINT('Ctrl Pts',(-55.5,8.71764735427698,14.4488148166716));
#60943=CARTESIAN_POINT('Ctrl Pts',(-50.5,8.71764735427698,14.4488148166716));
#60944=CARTESIAN_POINT('Origin',(-66.,0.,0.));
#60945=CARTESIAN_POINT('',(-66.,5.35024281477072,13.004953213026));
#60946=CARTESIAN_POINT('Ctrl Pts',(-66.,5.46444518084595,16.5986584959607));
#60947=CARTESIAN_POINT('Ctrl Pts',(-50.,5.46444518084595,16.5986584959607));
#60948=CARTESIAN_POINT('Ctrl Pts',(-66.,5.47014832855009,16.5768836277878));
#60949=CARTESIAN_POINT('Ctrl Pts',(-50.,5.47014832855009,16.5768836277878));
#60950=CARTESIAN_POINT('Ctrl Pts',(-66.,5.48140733077057,16.5333468419125));
#60951=CARTESIAN_POINT('Ctrl Pts',(-50.,5.48140733077057,16.5333468419125));
#60952=CARTESIAN_POINT('Ctrl Pts',(-66.,5.49785395520425,16.4680805143936));
#60953=CARTESIAN_POINT('Ctrl Pts',(-50.,5.49785395520425,16.4680805143936));
#60954=CARTESIAN_POINT('Ctrl Pts',(-66.,5.51889784893831,16.3811365513052));
#60955=CARTESIAN_POINT('Ctrl Pts',(-50.,5.51889784893831,16.3811365513052));
#60956=CARTESIAN_POINT('Ctrl Pts',(-66.,5.54372180667804,16.2725871160234));
#60957=CARTESIAN_POINT('Ctrl Pts',(-50.,5.54372180667804,16.2725871160234));
#60958=CARTESIAN_POINT('Ctrl Pts',(-66.,5.56705859689412,16.1641696957418));
#60959=CARTESIAN_POINT('Ctrl Pts',(-50.,5.56705859689412,16.1641696957418));
#60960=CARTESIAN_POINT('Ctrl Pts',(-66.,5.58890491898793,16.0558864600624));
#60961=CARTESIAN_POINT('Ctrl Pts',(-50.,5.58890491898793,16.0558864600624));
#60962=CARTESIAN_POINT('Ctrl Pts',(-66.,5.60926316858998,15.9477403748489));
#60963=CARTESIAN_POINT('Ctrl Pts',(-50.,5.60926316858998,15.9477403748489));
#60964=CARTESIAN_POINT('Ctrl Pts',(-66.,5.62814586043475,15.8397350261322));
#60965=CARTESIAN_POINT('Ctrl Pts',(-50.,5.62814586043475,15.8397350261322));
#60966=CARTESIAN_POINT('Ctrl Pts',(-66.,5.64556636287744,15.7318769847593));
#60967=CARTESIAN_POINT('Ctrl Pts',(-50.,5.64556636287744,15.7318769847593));
#60968=CARTESIAN_POINT('Ctrl Pts',(-66.,5.66152814272899,15.624178406052));
#60969=CARTESIAN_POINT('Ctrl Pts',(-50.,5.66152814272899,15.624178406052));
#60970=CARTESIAN_POINT('Ctrl Pts',(-66.,5.67601382140434,15.5166598272703));
#60971=CARTESIAN_POINT('Ctrl Pts',(-50.,5.67601382140434,15.5166598272703));
#60972=CARTESIAN_POINT('Ctrl Pts',(-66.,5.68897628762929,15.4093522928504));
#60973=CARTESIAN_POINT('Ctrl Pts',(-50.,5.68897628762929,15.4093522928504));
#60974=CARTESIAN_POINT('Ctrl Pts',(-66.,5.70032405390141,15.3023013794516));
#60975=CARTESIAN_POINT('Ctrl Pts',(-50.,5.70032405390141,15.3023013794516));
#60976=CARTESIAN_POINT('Ctrl Pts',(-66.,5.70994233430443,15.195559764519));
#60977=CARTESIAN_POINT('Ctrl Pts',(-50.,5.70994233430443,15.195559764519));
#60978=CARTESIAN_POINT('Ctrl Pts',(-66.,5.71772294845736,15.0891770284618));
#60979=CARTESIAN_POINT('Ctrl Pts',(-50.,5.71772294845736,15.0891770284618));
#60980=CARTESIAN_POINT('Ctrl Pts',(-66.,5.72359388237569,14.9831894879022));
#60981=CARTESIAN_POINT('Ctrl Pts',(-50.,5.72359388237569,14.9831894879022));
#60982=CARTESIAN_POINT('Ctrl Pts',(-66.,5.72754386270271,14.8776118616624));
#60983=CARTESIAN_POINT('Ctrl Pts',(-50.,5.72754386270271,14.8776118616624));
#60984=CARTESIAN_POINT('Ctrl Pts',(-66.,5.72966360991829,14.772423041662));
#60985=CARTESIAN_POINT('Ctrl Pts',(-50.,5.72966360991829,14.772423041662));
#60986=CARTESIAN_POINT('Ctrl Pts',(-66.,5.73009695097776,14.6675837685266));
#60987=CARTESIAN_POINT('Ctrl Pts',(-50.,5.73009695097776,14.6675837685266));
#60988=CARTESIAN_POINT('Ctrl Pts',(-66.,5.72896217357436,14.5630648469857));
#60989=CARTESIAN_POINT('Ctrl Pts',(-50.,5.72896217357436,14.5630648469857));
#60990=CARTESIAN_POINT('Ctrl Pts',(-66.,5.72627848390049,14.4588735885414));
#60991=CARTESIAN_POINT('Ctrl Pts',(-50.,5.72627848390049,14.4588735885414));
#60992=CARTESIAN_POINT('Ctrl Pts',(-66.,5.72190090792526,14.3550772805332));
#60993=CARTESIAN_POINT('Ctrl Pts',(-50.,5.72190090792526,14.3550772805332));
#60994=CARTESIAN_POINT('Ctrl Pts',(-66.,5.71542331821735,14.2518379845708));
#60995=CARTESIAN_POINT('Ctrl Pts',(-50.,5.71542331821735,14.2518379845708));
#60996=CARTESIAN_POINT('Ctrl Pts',(-66.,5.70626231068308,14.1493832151514));
#60997=CARTESIAN_POINT('Ctrl Pts',(-50.,5.70626231068308,14.1493832151514));
#60998=CARTESIAN_POINT('Ctrl Pts',(-66.,5.6938022661864,14.0479549027521));
#60999=CARTESIAN_POINT('Ctrl Pts',(-50.,5.6938022661864,14.0479549027521));
#61000=CARTESIAN_POINT('Ctrl Pts',(-66.,5.67752537508807,13.9477637996424));
#61001=CARTESIAN_POINT('Ctrl Pts',(-50.,5.67752537508807,13.9477637996424));
#61002=CARTESIAN_POINT('Ctrl Pts',(-66.,5.65713696965892,13.8489453830157));
#61003=CARTESIAN_POINT('Ctrl Pts',(-50.,5.65713696965892,13.8489453830157));
#61004=CARTESIAN_POINT('Ctrl Pts',(-66.,5.63272454065023,13.7515043267519));
#61005=CARTESIAN_POINT('Ctrl Pts',(-50.,5.63272454065023,13.7515043267519));
#61006=CARTESIAN_POINT('Ctrl Pts',(-66.,5.60468396737303,13.6553383842666));
#61007=CARTESIAN_POINT('Ctrl Pts',(-50.,5.60468396737303,13.6553383842666));
#61008=CARTESIAN_POINT('Ctrl Pts',(-66.,5.57358602861192,13.5602826717323));
#61009=CARTESIAN_POINT('Ctrl Pts',(-50.,5.57358602861192,13.5602826717323));
#61010=CARTESIAN_POINT('Ctrl Pts',(-66.,5.54006285706051,13.466147083991));
#61011=CARTESIAN_POINT('Ctrl Pts',(-50.,5.54006285706051,13.466147083991));
#61012=CARTESIAN_POINT('Ctrl Pts',(-66.,5.50469122725311,13.3727548702637));
#61013=CARTESIAN_POINT('Ctrl Pts',(-50.,5.50469122725311,13.3727548702637));
#61014=CARTESIAN_POINT('Ctrl Pts',(-66.,5.46786602291259,13.2799842691689));
#61015=CARTESIAN_POINT('Ctrl Pts',(-50.,5.46786602291259,13.2799842691689));
#61016=CARTESIAN_POINT('Ctrl Pts',(-66.,5.42982469604617,13.1877615232676));
#61017=CARTESIAN_POINT('Ctrl Pts',(-50.,5.42982469604617,13.1877615232676));
#61018=CARTESIAN_POINT('Ctrl Pts',(-66.,5.39851683671257,13.1143907147436));
#61019=CARTESIAN_POINT('Ctrl Pts',(-50.,5.39851683671257,13.1143907147436));
#61020=CARTESIAN_POINT('Ctrl Pts',(-66.,5.37456335134248,13.0595854308535));
#61021=CARTESIAN_POINT('Ctrl Pts',(-50.,5.37456335134248,13.0595854308535));
#61022=CARTESIAN_POINT('Ctrl Pts',(-66.,5.35838461816811,13.0231474696198));
#61023=CARTESIAN_POINT('Ctrl Pts',(-50.,5.35838461816811,13.0231474696198));
#61024=CARTESIAN_POINT('Ctrl Pts',(-66.,5.35024281477071,13.004953213026));
#61025=CARTESIAN_POINT('Ctrl Pts',(-50.,5.35024281477071,13.004953213026));
#61026=CARTESIAN_POINT('Origin',(-65.75,0.,0.));
#61027=CARTESIAN_POINT('',(-65.5,9.39615722699085,14.0170558380021));
#61028=CARTESIAN_POINT('Origin',(-65.5,0.,0.));
#61029=CARTESIAN_POINT('Ctrl Pts',(-65.5,9.39615722699085,14.0170558380021));
#61030=CARTESIAN_POINT('Ctrl Pts',(-65.693159547678,9.37933997904567,13.7957861293633));
#61031=CARTESIAN_POINT('Ctrl Pts',(-65.861125696713,9.3565516065934,13.6076347927665));
#61032=CARTESIAN_POINT('Ctrl Pts',(-66.,9.33394806226437,13.4542944285812));
#61033=CARTESIAN_POINT('Origin',(-58.,0.,0.));
#61034=CARTESIAN_POINT('',(-50.5,9.39615722699085,14.0170558380021));
#61035=CARTESIAN_POINT('Origin',(-50.5,0.,0.));
#61036=CARTESIAN_POINT('Ctrl Pts',(-50.5,9.39615722699085,14.0170558380021));
#61037=CARTESIAN_POINT('Ctrl Pts',(-55.5,9.39615722699085,14.0170558380021));
#61038=CARTESIAN_POINT('Ctrl Pts',(-60.5,9.39615722699085,14.0170558380021));
#61039=CARTESIAN_POINT('Ctrl Pts',(-65.5,9.39615722699085,14.0170558380021));
#61040=CARTESIAN_POINT('Origin',(-50.25,0.,0.));
#61041=CARTESIAN_POINT('Ctrl Pts',(-50.,9.33394806226437,13.4542944285812));
#61042=CARTESIAN_POINT('Ctrl Pts',(-50.1388743032948,9.35655160659466,13.6076347927751));
#61043=CARTESIAN_POINT('Ctrl Pts',(-50.3068404523291,9.3793399790463,13.7957861293714));
#61044=CARTESIAN_POINT('Ctrl Pts',(-50.5,9.39615722699085,14.0170558380021));
#61045=CARTESIAN_POINT('Ctrl Pts',(-66.,9.48921088782658,10.3782842019456));
#61046=CARTESIAN_POINT('Ctrl Pts',(-50.,9.48921088782658,10.3782842019456));
#61047=CARTESIAN_POINT('Ctrl Pts',(-66.,9.5042599930153,10.3961665635534));
#61048=CARTESIAN_POINT('Ctrl Pts',(-50.,9.5042599930153,10.3961665635534));
#61049=CARTESIAN_POINT('Ctrl Pts',(-66.,9.53453615016101,10.4317934371322));
#61050=CARTESIAN_POINT('Ctrl Pts',(-50.,9.53453615016101,10.4317934371322));
#61051=CARTESIAN_POINT('Ctrl Pts',(-66.,9.58048422171402,10.4848202111794));
#61052=CARTESIAN_POINT('Ctrl Pts',(-50.,9.58048422171402,10.4848202111794));
#61053=CARTESIAN_POINT('Ctrl Pts',(-66.,9.64281744709338,10.5546942954216));
#61054=CARTESIAN_POINT('Ctrl Pts',(-50.,9.64281744709338,10.5546942954216));
#61055=CARTESIAN_POINT('Ctrl Pts',(-66.,9.72254683584991,10.6406085262144));
#61056=CARTESIAN_POINT('Ctrl Pts',(-50.,9.72254683584991,10.6406085262144));
#61057=CARTESIAN_POINT('Ctrl Pts',(-66.,9.80416846317344,10.7249595816546));
#61058=CARTESIAN_POINT('Ctrl Pts',(-50.,9.80416846317344,10.7249595816546));
#61059=CARTESIAN_POINT('Ctrl Pts',(-66.,9.88782918758628,10.8074894324552));
#61060=CARTESIAN_POINT('Ctrl Pts',(-50.,9.88782918758628,10.8074894324552));
#61061=CARTESIAN_POINT('Ctrl Pts',(-66.,9.97376743729857,10.8877656023939));
#61062=CARTESIAN_POINT('Ctrl Pts',(-50.,9.97376743729857,10.8877656023939));
#61063=CARTESIAN_POINT('Ctrl Pts',(-66.,10.0623044106004,10.9652479123292));
#61064=CARTESIAN_POINT('Ctrl Pts',(-50.,10.0623044106004,10.9652479123292));
#61065=CARTESIAN_POINT('Ctrl Pts',(-66.,10.1538362031934,11.0393768173572));
#61066=CARTESIAN_POINT('Ctrl Pts',(-50.,10.1538362031934,11.0393768173572));
#61067=CARTESIAN_POINT('Ctrl Pts',(-66.,10.2488131895374,11.1096536475468));
#61068=CARTESIAN_POINT('Ctrl Pts',(-50.,10.2488131895374,11.1096536475468));
#61069=CARTESIAN_POINT('Ctrl Pts',(-66.,10.347755963003,11.1757261609666));
#61070=CARTESIAN_POINT('Ctrl Pts',(-50.,10.347755963003,11.1757261609666));
#61071=CARTESIAN_POINT('Ctrl Pts',(-66.,10.4510776067987,11.237474600108));
#61072=CARTESIAN_POINT('Ctrl Pts',(-50.,10.4510776067987,11.237474600108));
#61073=CARTESIAN_POINT('Ctrl Pts',(-66.,10.558769691859,11.2951234927996));
#61074=CARTESIAN_POINT('Ctrl Pts',(-50.,10.558769691859,11.2951234927996));
#61075=CARTESIAN_POINT('Ctrl Pts',(-66.,10.6701988175887,11.3493082317362));
#61076=CARTESIAN_POINT('Ctrl Pts',(-50.,10.6701988175887,11.3493082317362));
#61077=CARTESIAN_POINT('Ctrl Pts',(-66.,10.7836901223469,11.4012548314131));
#61078=CARTESIAN_POINT('Ctrl Pts',(-50.,10.7836901223469,11.4012548314131));
#61079=CARTESIAN_POINT('Ctrl Pts',(-66.,10.896814048301,11.4525672852113));
#61080=CARTESIAN_POINT('Ctrl Pts',(-50.,10.896814048301,11.4525672852113));
#61081=CARTESIAN_POINT('Ctrl Pts',(-66.,11.0075923712357,11.5044910494005));
#61082=CARTESIAN_POINT('Ctrl Pts',(-50.,11.0075923712357,11.5044910494005));
#61083=CARTESIAN_POINT('Ctrl Pts',(-66.,11.1153726577894,11.5573722819667));
#61084=CARTESIAN_POINT('Ctrl Pts',(-50.,11.1153726577894,11.5573722819667));
#61085=CARTESIAN_POINT('Ctrl Pts',(-66.,11.2220605212152,11.6098943525204));
#61086=CARTESIAN_POINT('Ctrl Pts',(-50.,11.2220605212152,11.6098943525204));
#61087=CARTESIAN_POINT('Ctrl Pts',(-66.,11.3325619722949,11.6588176962357));
#61088=CARTESIAN_POINT('Ctrl Pts',(-50.,11.3325619722949,11.6588176962357));
#61089=CARTESIAN_POINT('Ctrl Pts',(-66.,11.4520601045496,11.7007489213372));
#61090=CARTESIAN_POINT('Ctrl Pts',(-50.,11.4520601045496,11.7007489213372));
#61091=CARTESIAN_POINT('Ctrl Pts',(-66.,11.5836877573447,11.7336565821219));
#61092=CARTESIAN_POINT('Ctrl Pts',(-50.,11.5836877573447,11.7336565821219));
#61093=CARTESIAN_POINT('Ctrl Pts',(-66.,11.7261518526103,11.7584167691267));
#61094=CARTESIAN_POINT('Ctrl Pts',(-50.,11.7261518526103,11.7584167691267));
#61095=CARTESIAN_POINT('Ctrl Pts',(-66.,11.8710524298673,11.7805590057687));
#61096=CARTESIAN_POINT('Ctrl Pts',(-50.,11.8710524298673,11.7805590057687));
#61097=CARTESIAN_POINT('Ctrl Pts',(-66.,12.0049368454181,11.8089201490911));
#61098=CARTESIAN_POINT('Ctrl Pts',(-50.,12.0049368454181,11.8089201490911));
#61099=CARTESIAN_POINT('Ctrl Pts',(-66.,12.1119147081034,11.8539322819168));
#61100=CARTESIAN_POINT('Ctrl Pts',(-50.,12.1119147081034,11.8539322819168));
#61101=CARTESIAN_POINT('Ctrl Pts',(-66.,12.1758810539398,11.9261667725489));
#61102=CARTESIAN_POINT('Ctrl Pts',(-50.,12.1758810539398,11.9261667725489));
#61103=CARTESIAN_POINT('Ctrl Pts',(-66.,12.183322517921,12.0344969363598));
#61104=CARTESIAN_POINT('Ctrl Pts',(-50.,12.183322517921,12.0344969363598));
#61105=CARTESIAN_POINT('Ctrl Pts',(-66.,12.1240717269814,12.1856037794161));
#61106=CARTESIAN_POINT('Ctrl Pts',(-50.,12.1240717269814,12.1856037794161));
#61107=CARTESIAN_POINT('Ctrl Pts',(-66.,11.9905553905945,12.384467849066));
#61108=CARTESIAN_POINT('Ctrl Pts',(-50.,11.9905553905945,12.384467849066));
#61109=CARTESIAN_POINT('Ctrl Pts',(-66.,11.7774987869249,12.6345623838968));
#61110=CARTESIAN_POINT('Ctrl Pts',(-50.,11.7774987869249,12.6345623838968));
#61111=CARTESIAN_POINT('Ctrl Pts',(-66.,11.4814643452976,12.9381551285812));
#61112=CARTESIAN_POINT('Ctrl Pts',(-50.,11.4814643452976,12.9381551285812));
#61113=CARTESIAN_POINT('Ctrl Pts',(-66.,11.1004818366232,13.2965502388611));
#61114=CARTESIAN_POINT('Ctrl Pts',(-50.,11.1004818366232,13.2965502388611));
#61115=CARTESIAN_POINT('Ctrl Pts',(-66.,10.6336578580906,13.7103437971785));
#61116=CARTESIAN_POINT('Ctrl Pts',(-50.,10.6336578580906,13.7103437971785));
#61117=CARTESIAN_POINT('Ctrl Pts',(-66.,10.1913804628862,14.0857987564915));
#61118=CARTESIAN_POINT('Ctrl Pts',(-50.,10.1913804628862,14.0857987564915));
#61119=CARTESIAN_POINT('Ctrl Pts',(-66.,9.82103857054357,14.392328422685));
#61120=CARTESIAN_POINT('Ctrl Pts',(-50.,9.82103857054357,14.392328422685));
#61121=CARTESIAN_POINT('Ctrl Pts',(-66.,9.55699621520391,14.6077505454562));
#61122=CARTESIAN_POINT('Ctrl Pts',(-50.,9.55699621520391,14.6077505454562));
#61123=CARTESIAN_POINT('Ctrl Pts',(-66.,9.42068809552632,14.7182288610691));
#61124=CARTESIAN_POINT('Ctrl Pts',(-50.,9.42068809552632,14.7182288610691));
#61125=CARTESIAN_POINT('',(-65.5,12.0370405584342,11.8268879928158));
#61126=CARTESIAN_POINT('Ctrl Pts',(-66.,11.4573006693292,11.699183149801));
#61127=CARTESIAN_POINT('Ctrl Pts',(-65.7933280154038,11.6841669321105,11.7662800362502));
#61128=CARTESIAN_POINT('Ctrl Pts',(-65.6370761749488,11.8992955888885,11.7714956810329));
#61129=CARTESIAN_POINT('Ctrl Pts',(-65.5,12.0370405584342,11.8268879928158));
#61130=CARTESIAN_POINT('',(-66.,9.48921088782658,10.3782842019456));
#61131=CARTESIAN_POINT('',(-50.5,12.0370405584342,11.8268879928158));
#61132=CARTESIAN_POINT('Ctrl Pts',(-50.5,12.0370405584342,11.8268879928158));
#61133=CARTESIAN_POINT('Ctrl Pts',(-50.451861834912,11.98866752726,11.8074354201845));
#61134=CARTESIAN_POINT('Ctrl Pts',(-50.4012423593881,11.9308719343602,11.7939736533257));
#61135=CARTESIAN_POINT('Ctrl Pts',(-50.2441129793797,11.7444907150908,11.7586971973344));
#61136=CARTESIAN_POINT('Ctrl Pts',(-50.1366827452942,11.607338922807,11.7435577497667));
#61137=CARTESIAN_POINT('Ctrl Pts',(-50.,11.4573006693292,11.699183149801));
#61138=CARTESIAN_POINT('Ctrl Pts',(-65.5,12.0370405584342,11.8268879928158));
#61139=CARTESIAN_POINT('Ctrl Pts',(-60.5,12.0370405584342,11.8268879928158));
#61140=CARTESIAN_POINT('Ctrl Pts',(-55.5,12.0370405584342,11.8268879928158));
#61141=CARTESIAN_POINT('Ctrl Pts',(-50.5,12.0370405584342,11.8268879928158));
#61142=CARTESIAN_POINT('Origin',(-66.,0.,0.));
#61143=CARTESIAN_POINT('',(-66.,8.41635544546802,11.2658274114927));
#61144=CARTESIAN_POINT('Ctrl Pts',(-66.,9.42068809552632,14.7182288610691));
#61145=CARTESIAN_POINT('Ctrl Pts',(-50.,9.42068809552632,14.7182288610691));
#61146=CARTESIAN_POINT('Ctrl Pts',(-66.,9.42079687884903,14.695719775262));
#61147=CARTESIAN_POINT('Ctrl Pts',(-50.,9.42079687884903,14.695719775262));
#61148=CARTESIAN_POINT('Ctrl Pts',(-66.,9.42087500044404,14.6507507775818));
#61149=CARTESIAN_POINT('Ctrl Pts',(-50.,9.42087500044404,14.6507507775818));
#61150=CARTESIAN_POINT('Ctrl Pts',(-66.,9.42057384830158,14.5834448025836));
#61151=CARTESIAN_POINT('Ctrl Pts',(-50.,9.42057384830158,14.5834448025836));
#61152=CARTESIAN_POINT('Ctrl Pts',(-66.,9.41933452504685,14.4939989404162));
#61153=CARTESIAN_POINT('Ctrl Pts',(-50.,9.41933452504685,14.4939989404162));
#61154=CARTESIAN_POINT('Ctrl Pts',(-66.,9.41638344569407,14.3826863180029));
#61155=CARTESIAN_POINT('Ctrl Pts',(-50.,9.41638344569407,14.3826863180029));
#61156=CARTESIAN_POINT('Ctrl Pts',(-66.,9.41202475171563,14.2718714066195));
#61157=CARTESIAN_POINT('Ctrl Pts',(-50.,9.41202475171563,14.2718714066195));
#61158=CARTESIAN_POINT('Ctrl Pts',(-66.,9.40625578576533,14.1615571285314));
#61159=CARTESIAN_POINT('Ctrl Pts',(-50.,9.40625578576533,14.1615571285314));
#61160=CARTESIAN_POINT('Ctrl Pts',(-66.,9.39907960579085,14.0517457606552));
#61161=CARTESIAN_POINT('Ctrl Pts',(-50.,9.39907960579085,14.0517457606552));
#61162=CARTESIAN_POINT('Ctrl Pts',(-66.,9.39050922516292,13.9424376640721));
#61163=CARTESIAN_POINT('Ctrl Pts',(-50.,9.39050922516292,13.9424376640721));
#61164=CARTESIAN_POINT('Ctrl Pts',(-66.,9.38055922634845,13.8336358786192));
#61165=CARTESIAN_POINT('Ctrl Pts',(-50.,9.38055922634845,13.8336358786192));
#61166=CARTESIAN_POINT('Ctrl Pts',(-66.,9.36923599014777,13.7253513155756));
#61167=CARTESIAN_POINT('Ctrl Pts',(-50.,9.36923599014777,13.7253513155756));
#61168=CARTESIAN_POINT('Ctrl Pts',(-66.,9.35652779136491,13.6176081888639));
#61169=CARTESIAN_POINT('Ctrl Pts',(-50.,9.35652779136491,13.6176081888639));
#61170=CARTESIAN_POINT('Ctrl Pts',(-66.,9.34239671925027,13.5104482836997));
#61171=CARTESIAN_POINT('Ctrl Pts',(-50.,9.34239671925027,13.5104482836997));
#61172=CARTESIAN_POINT('Ctrl Pts',(-66.,9.32676549500383,13.4039384968844));
#61173=CARTESIAN_POINT('Ctrl Pts',(-50.,9.32676549500383,13.4039384968844));
#61174=CARTESIAN_POINT('Ctrl Pts',(-66.,9.30953603926783,13.2981583970009));
#61175=CARTESIAN_POINT('Ctrl Pts',(-50.,9.30953603926783,13.2981583970009));
#61176=CARTESIAN_POINT('Ctrl Pts',(-66.,9.29061590049322,13.1931829101653));
#61177=CARTESIAN_POINT('Ctrl Pts',(-50.,9.29061590049322,13.1931829101653));
#61178=CARTESIAN_POINT('Ctrl Pts',(-66.,9.26994435872398,13.0890651211961));
#61179=CARTESIAN_POINT('Ctrl Pts',(-50.,9.26994435872398,13.0890651211961));
#61180=CARTESIAN_POINT('Ctrl Pts',(-66.,9.24751415519882,12.9858220900665));
#61181=CARTESIAN_POINT('Ctrl Pts',(-50.,9.24751415519882,12.9858220900665));
#61182=CARTESIAN_POINT('Ctrl Pts',(-66.,9.22340791088078,12.8834108105793));
#61183=CARTESIAN_POINT('Ctrl Pts',(-50.,9.22340791088078,12.8834108105793));
#61184=CARTESIAN_POINT('Ctrl Pts',(-66.,9.19775517072751,12.7817574884561));
#61185=CARTESIAN_POINT('Ctrl Pts',(-50.,9.19775517072751,12.7817574884561));
#61186=CARTESIAN_POINT('Ctrl Pts',(-66.,9.17066324563836,12.6808044286968));
#61187=CARTESIAN_POINT('Ctrl Pts',(-50.,9.17066324563836,12.6808044286968));
#61188=CARTESIAN_POINT('Ctrl Pts',(-66.,9.14215255670447,12.580553936713));
#61189=CARTESIAN_POINT('Ctrl Pts',(-50.,9.14215255670447,12.580553936713));
#61190=CARTESIAN_POINT('Ctrl Pts',(-66.,9.11209941820162,12.4811072394643));
#61191=CARTESIAN_POINT('Ctrl Pts',(-50.,9.11209941820162,12.4811072394643));
#61192=CARTESIAN_POINT('Ctrl Pts',(-66.,9.08015076502197,12.3827223068819));
#61193=CARTESIAN_POINT('Ctrl Pts',(-50.,9.08015076502197,12.3827223068819));
#61194=CARTESIAN_POINT('Ctrl Pts',(-66.,9.04579810233888,12.2857645923749));
#61195=CARTESIAN_POINT('Ctrl Pts',(-50.,9.04579810233888,12.2857645923749));
#61196=CARTESIAN_POINT('Ctrl Pts',(-66.,9.00850531748659,12.1906215239832));
#61197=CARTESIAN_POINT('Ctrl Pts',(-50.,9.00850531748659,12.1906215239832));
#61198=CARTESIAN_POINT('Ctrl Pts',(-66.,8.96782328072592,12.0976260068268));
#61199=CARTESIAN_POINT('Ctrl Pts',(-50.,8.96782328072592,12.0976260068268));
#61200=CARTESIAN_POINT('Ctrl Pts',(-66.,8.9235002736643,12.0069825427185));
#61201=CARTESIAN_POINT('Ctrl Pts',(-50.,8.9235002736643,12.0069825427185));
#61202=CARTESIAN_POINT('Ctrl Pts',(-66.,8.87562220071675,11.9186739006343));
#61203=CARTESIAN_POINT('Ctrl Pts',(-50.,8.87562220071675,11.9186739006343));
#61204=CARTESIAN_POINT('Ctrl Pts',(-66.,8.82454707622628,11.8325025950734));
#61205=CARTESIAN_POINT('Ctrl Pts',(-50.,8.82454707622628,11.8325025950734));
#61206=CARTESIAN_POINT('Ctrl Pts',(-66.,8.77078674197194,11.7481669754252));
#61207=CARTESIAN_POINT('Ctrl Pts',(-50.,8.77078674197194,11.7481669754252));
#61208=CARTESIAN_POINT('Ctrl Pts',(-66.,8.71490619380604,11.6653257040265));
#61209=CARTESIAN_POINT('Ctrl Pts',(-50.,8.71490619380604,11.6653257040265));
#61210=CARTESIAN_POINT('Ctrl Pts',(-66.,8.657420129699,11.5836641450553));
#61211=CARTESIAN_POINT('Ctrl Pts',(-50.,8.657420129699,11.5836641450553));
#61212=CARTESIAN_POINT('Ctrl Pts',(-66.,8.59868074655117,11.5029661588994));
#61213=CARTESIAN_POINT('Ctrl Pts',(-50.,8.59868074655117,11.5029661588994));
#61214=CARTESIAN_POINT('Ctrl Pts',(-66.,8.53889969364915,11.4231012534324));
#61215=CARTESIAN_POINT('Ctrl Pts',(-50.,8.53889969364915,11.4231012534324));
#61216=CARTESIAN_POINT('Ctrl Pts',(-66.,8.49032885019461,11.3598214717827));
#61217=CARTESIAN_POINT('Ctrl Pts',(-50.,8.49032885019461,11.3598214717827));
#61218=CARTESIAN_POINT('Ctrl Pts',(-66.,8.45349838774813,11.3126949862398));
#61219=CARTESIAN_POINT('Ctrl Pts',(-50.,8.45349838774813,11.3126949862398));
#61220=CARTESIAN_POINT('Ctrl Pts',(-66.,8.4287661867593,11.2814252778905));
#61221=CARTESIAN_POINT('Ctrl Pts',(-50.,8.4287661867593,11.2814252778905));
#61222=CARTESIAN_POINT('Ctrl Pts',(-66.,8.416355445468,11.2658274114927));
#61223=CARTESIAN_POINT('Ctrl Pts',(-50.,8.416355445468,11.2658274114927));
#61224=CARTESIAN_POINT('Origin',(-65.75,0.,0.));
#61225=CARTESIAN_POINT('',(-65.5,12.5868597041166,11.239954972725));
#61226=CARTESIAN_POINT('Origin',(-65.5,0.,0.));
#61227=CARTESIAN_POINT('Ctrl Pts',(-65.5,12.5868597041166,11.239954972725));
#61228=CARTESIAN_POINT('Ctrl Pts',(-65.6931595476683,12.5155432620696,11.0298191383741));
#61229=CARTESIAN_POINT('Ctrl Pts',(-65.8611256967109,12.446679493572,10.853246159768));
#61230=CARTESIAN_POINT('Ctrl Pts',(-66.,12.3866518832851,10.7103445379834));
#61231=CARTESIAN_POINT('Origin',(-58.,0.,0.));
#61232=CARTESIAN_POINT('',(-50.5,12.5868597041166,11.239954972725));
#61233=CARTESIAN_POINT('Origin',(-50.5,0.,0.));
#61234=CARTESIAN_POINT('Ctrl Pts',(-50.5,12.5868597041166,11.239954972725));
#61235=CARTESIAN_POINT('Ctrl Pts',(-55.5,12.5868597041166,11.239954972725));
#61236=CARTESIAN_POINT('Ctrl Pts',(-60.5,12.5868597041166,11.239954972725));
#61237=CARTESIAN_POINT('Ctrl Pts',(-65.5,12.5868597041166,11.239954972725));
#61238=CARTESIAN_POINT('Origin',(-50.25,0.,0.));
#61239=CARTESIAN_POINT('Ctrl Pts',(-50.,12.3866518832851,10.7103445379834));
#61240=CARTESIAN_POINT('Ctrl Pts',(-50.138874303285,12.4466794935702,10.8532461597638));
#61241=CARTESIAN_POINT('Ctrl Pts',(-50.3068404523221,12.515543262066,11.0298191383637));
#61242=CARTESIAN_POINT('Ctrl Pts',(-50.5,12.5868597041166,11.239954972725));
#61243=CARTESIAN_POINT('Ctrl Pts',(-66.,11.7720642054939,7.69236053443469));
#61244=CARTESIAN_POINT('Ctrl Pts',(-50.,11.7720642054939,7.69236053443469));
#61245=CARTESIAN_POINT('Ctrl Pts',(-66.,11.7910876778603,7.70593852849788));
#61246=CARTESIAN_POINT('Ctrl Pts',(-50.,11.7910876778603,7.70593852849788));
#61247=CARTESIAN_POINT('Ctrl Pts',(-66.,11.8292726970256,7.73291674422561));
#61248=CARTESIAN_POINT('Ctrl Pts',(-50.,11.8292726970256,7.73291674422561));
#61249=CARTESIAN_POINT('Ctrl Pts',(-66.,11.8869644478727,7.77285076392682));
#61250=CARTESIAN_POINT('Ctrl Pts',(-50.,11.8869644478727,7.77285076392682));
#61251=CARTESIAN_POINT('Ctrl Pts',(-66.,11.96471633848,7.82502798253687));
#61252=CARTESIAN_POINT('Ctrl Pts',(-50.,11.96471633848,7.82502798253687));
#61253=CARTESIAN_POINT('Ctrl Pts',(-66.,12.0633068822383,7.88841516709048));
#61254=CARTESIAN_POINT('Ctrl Pts',(-50.,12.0633068822383,7.88841516709048));
#61255=CARTESIAN_POINT('Ctrl Pts',(-66.,12.1633414705075,7.94981770572398));
#61256=CARTESIAN_POINT('Ctrl Pts',(-50.,12.1633414705075,7.94981770572398));
#61257=CARTESIAN_POINT('Ctrl Pts',(-66.,12.2648981787049,8.00894915338555));
#61258=CARTESIAN_POINT('Ctrl Pts',(-50.,12.2648981787049,8.00894915338555));
#61259=CARTESIAN_POINT('Ctrl Pts',(-66.,12.3681003919172,8.06533132620399));
#61260=CARTESIAN_POINT('Ctrl Pts',(-50.,12.3681003919172,8.06533132620399));
#61261=CARTESIAN_POINT('Ctrl Pts',(-66.,12.4731248803097,8.11836113699226));
#61262=CARTESIAN_POINT('Ctrl Pts',(-50.,12.4731248803097,8.11836113699226));
#61263=CARTESIAN_POINT('Ctrl Pts',(-66.,12.5802161423503,8.16739811498339));
#61264=CARTESIAN_POINT('Ctrl Pts',(-50.,12.5802161423503,8.16739811498339));
#61265=CARTESIAN_POINT('Ctrl Pts',(-66.,12.6896863889879,8.21184725330542));
#61266=CARTESIAN_POINT('Ctrl Pts',(-50.,12.6896863889879,8.21184725330542));
#61267=CARTESIAN_POINT('Ctrl Pts',(-66.,12.8019522591891,8.25123791004828));
#61268=CARTESIAN_POINT('Ctrl Pts',(-50.,12.8019522591891,8.25123791004828));
#61269=CARTESIAN_POINT('Ctrl Pts',(-66.,12.9173840759125,8.28535136048938));
#61270=CARTESIAN_POINT('Ctrl Pts',(-50.,12.9173840759125,8.28535136048938));
#61271=CARTESIAN_POINT('Ctrl Pts',(-66.,13.0360295127074,8.31440717472604));
#61272=CARTESIAN_POINT('Ctrl Pts',(-50.,13.0360295127074,8.31440717472604));
#61273=CARTESIAN_POINT('Ctrl Pts',(-66.,13.1574330841607,8.33917830374554));
#61274=CARTESIAN_POINT('Ctrl Pts',(-50.,13.1574330841607,8.33917830374554));
#61275=CARTESIAN_POINT('Ctrl Pts',(-66.,13.2802774448963,8.36126876569594));
#61276=CARTESIAN_POINT('Ctrl Pts',(-50.,13.2802774448963,8.36126876569594));
#61277=CARTESIAN_POINT('Ctrl Pts',(-66.,13.4026082630414,8.38283636801991));
#61278=CARTESIAN_POINT('Ctrl Pts',(-50.,13.4026082630414,8.38283636801991));
#61279=CARTESIAN_POINT('Ctrl Pts',(-66.,13.5228191963114,8.40557940304509));
#61280=CARTESIAN_POINT('Ctrl Pts',(-50.,13.5228191963114,8.40557940304509));
#61281=CARTESIAN_POINT('Ctrl Pts',(-66.,13.640364394729,8.42999540714673));
#61282=CARTESIAN_POINT('Ctrl Pts',(-50.,13.640364394729,8.42999540714673));
#61283=CARTESIAN_POINT('Ctrl Pts',(-66.,13.7567621705396,8.45433520755552));
#61284=CARTESIAN_POINT('Ctrl Pts',(-50.,13.7567621705396,8.45433520755552));
#61285=CARTESIAN_POINT('Ctrl Pts',(-66.,13.875958756164,8.47424094106369));
#61286=CARTESIAN_POINT('Ctrl Pts',(-50.,13.875958756164,8.47424094106369));
#61287=CARTESIAN_POINT('Ctrl Pts',(-66.,14.0021305064914,8.48513684259561));
#61288=CARTESIAN_POINT('Ctrl Pts',(-50.,14.0021305064914,8.48513684259561));
#61289=CARTESIAN_POINT('Ctrl Pts',(-66.,14.137806636975,8.48427618258244));
#61290=CARTESIAN_POINT('Ctrl Pts',(-50.,14.137806636975,8.48427618258244));
#61291=CARTESIAN_POINT('Ctrl Pts',(-66.,14.2819525688271,8.47282910300502));
#61292=CARTESIAN_POINT('Ctrl Pts',(-50.,14.2819525688271,8.47282910300502));
#61293=CARTESIAN_POINT('Ctrl Pts',(-66.,14.4278073783281,8.45824039235802));
#61294=CARTESIAN_POINT('Ctrl Pts',(-50.,14.4278073783281,8.45824039235802));
#61295=CARTESIAN_POINT('Ctrl Pts',(-66.,14.5645386983009,8.45241481801397));
#61296=CARTESIAN_POINT('Ctrl Pts',(-50.,14.5645386983009,8.45241481801397));
#61297=CARTESIAN_POINT('Ctrl Pts',(-66.,14.6793497169449,8.4694084993151));
#61298=CARTESIAN_POINT('Ctrl Pts',(-50.,14.6793497169449,8.4694084993151));
#61299=CARTESIAN_POINT('Ctrl Pts',(-66.,14.7592704297256,8.52346582726567));
#61300=CARTESIAN_POINT('Ctrl Pts',(-50.,14.7592704297256,8.52346582726567));
#61301=CARTESIAN_POINT('Ctrl Pts',(-66.,14.7934187226467,8.62654198293735));
#61302=CARTESIAN_POINT('Ctrl Pts',(-50.,14.7934187226467,8.62654198293735));
#61303=CARTESIAN_POINT('Ctrl Pts',(-66.,14.7736081480085,8.78763659916624));
#61304=CARTESIAN_POINT('Ctrl Pts',(-50.,14.7736081480085,8.78763659916624));
#61305=CARTESIAN_POINT('Ctrl Pts',(-66.,14.693741955891,9.01345715101332));
#61306=CARTESIAN_POINT('Ctrl Pts',(-50.,14.693741955891,9.01345715101332));
#61307=CARTESIAN_POINT('Ctrl Pts',(-66.,14.5495748988569,9.30867952886707));
#61308=CARTESIAN_POINT('Ctrl Pts',(-50.,14.5495748988569,9.30867952886707));
#61309=CARTESIAN_POINT('Ctrl Pts',(-66.,14.3383413690023,9.67635512109445));
#61310=CARTESIAN_POINT('Ctrl Pts',(-50.,14.3383413690023,9.67635512109445));
#61311=CARTESIAN_POINT('Ctrl Pts',(-66.,14.0584573659516,10.1182370870364));
#61312=CARTESIAN_POINT('Ctrl Pts',(-50.,14.0584573659516,10.1182370870364));
#61313=CARTESIAN_POINT('Ctrl Pts',(-66.,13.7092057944614,10.6351249623533));
#61314=CARTESIAN_POINT('Ctrl Pts',(-50.,13.7092057944614,10.6351249623533));
#61315=CARTESIAN_POINT('Ctrl Pts',(-66.,13.3741952083856,11.108774229215));
#61316=CARTESIAN_POINT('Ctrl Pts',(-50.,13.3741952083856,11.108774229215));
#61317=CARTESIAN_POINT('Ctrl Pts',(-66.,13.0917191157004,11.4977739856956));
#61318=CARTESIAN_POINT('Ctrl Pts',(-50.,13.0917191157004,11.4977739856956));
#61319=CARTESIAN_POINT('Ctrl Pts',(-66.,12.8895454398984,11.7720928899025));
#61320=CARTESIAN_POINT('Ctrl Pts',(-50.,12.8895454398984,11.7720928899025));
#61321=CARTESIAN_POINT('Ctrl Pts',(-66.,12.7849945302975,11.9129987769773));
#61322=CARTESIAN_POINT('Ctrl Pts',(-50.,12.7849945302975,11.9129987769773));
#61323=CARTESIAN_POINT('',(-65.5,14.6001022351665,8.46183430012001));
#61324=CARTESIAN_POINT('Ctrl Pts',(-66.,14.0068170377451,8.48231698718778));
#61325=CARTESIAN_POINT('Ctrl Pts',(-65.7933280154031,14.2432421968242,8.490886556274));
#61326=CARTESIAN_POINT('Ctrl Pts',(-65.6370761749492,14.4529092693668,8.44243802060488));
#61327=CARTESIAN_POINT('Ctrl Pts',(-65.5,14.6001022351665,8.46183430012001));
#61328=CARTESIAN_POINT('',(-66.,11.7720642054939,7.69236053443469));
#61329=CARTESIAN_POINT('',(-50.5,14.6001022351665,8.46183430012001));
#61330=CARTESIAN_POINT('Ctrl Pts',(-50.5,14.6001022351664,8.46183430012001));
#61331=CARTESIAN_POINT('Ctrl Pts',(-50.4518618349121,14.5484112736258,8.45502274949325));
#61332=CARTESIAN_POINT('Ctrl Pts',(-50.4012423593883,14.4890836302746,8.4563570882716));
#61333=CARTESIAN_POINT('Ctrl Pts',(-50.2441129793798,14.2997850218794,8.46854003140394));
#61334=CARTESIAN_POINT('Ctrl Pts',(-50.1366827452942,14.1631770778471,8.48798448116852));
#61335=CARTESIAN_POINT('Ctrl Pts',(-50.,14.0068170377451,8.48231698718778));
#61336=CARTESIAN_POINT('Ctrl Pts',(-65.5,14.6001022351665,8.46183430012001));
#61337=CARTESIAN_POINT('Ctrl Pts',(-60.5,14.6001022351665,8.46183430012001));
#61338=CARTESIAN_POINT('Ctrl Pts',(-55.5,14.6001022351665,8.46183430012001));
#61339=CARTESIAN_POINT('Ctrl Pts',(-50.5,14.6001022351665,8.46183430012001));
#61340=CARTESIAN_POINT('Origin',(-66.,0.,0.));
#61341=CARTESIAN_POINT('',(-66.,10.9536375103364,8.81882824088046));
#61342=CARTESIAN_POINT('Ctrl Pts',(-66.,12.7849945302975,11.9129987769773));
#61343=CARTESIAN_POINT('Ctrl Pts',(-50.,12.7849945302975,11.9129987769773));
#61344=CARTESIAN_POINT('Ctrl Pts',(-66.,12.7795021139826,11.8911698021799));
#61345=CARTESIAN_POINT('Ctrl Pts',(-50.,12.7795021139826,11.8911698021799));
#61346=CARTESIAN_POINT('Ctrl Pts',(-66.,12.768394446285,11.8475941602033));
#61347=CARTESIAN_POINT('Ctrl Pts',(-50.,12.768394446285,11.8475941602033));
#61348=CARTESIAN_POINT('Ctrl Pts',(-66.,12.7513644400631,11.782477619669));
#61349=CARTESIAN_POINT('Ctrl Pts',(-50.,12.7513644400631,11.782477619669));
#61350=CARTESIAN_POINT('Ctrl Pts',(-66.,12.7279197710576,11.6961500709014));
#61351=CARTESIAN_POINT('Ctrl Pts',(-50.,12.7279197710576,11.6961500709014));
#61352=CARTESIAN_POINT('Ctrl Pts',(-66.,12.6973790817813,11.5890684428021));
#61353=CARTESIAN_POINT('Ctrl Pts',(-50.,12.6973790817813,11.5890684428021));
#61354=CARTESIAN_POINT('Ctrl Pts',(-66.,12.6655987763812,11.4828189487479));
#61355=CARTESIAN_POINT('Ctrl Pts',(-50.,12.6655987763812,11.4828189487479));
#61356=CARTESIAN_POINT('Ctrl Pts',(-66.,12.6325770077342,11.3774050800509));
#61357=CARTESIAN_POINT('Ctrl Pts',(-50.,12.6325770077342,11.3774050800509));
#61358=CARTESIAN_POINT('Ctrl Pts',(-66.,12.5983173039631,11.2728282816136));
#61359=CARTESIAN_POINT('Ctrl Pts',(-50.,12.5983173039631,11.2728282816136));
#61360=CARTESIAN_POINT('Ctrl Pts',(-66.,12.562832359397,11.1690856668796));
#61361=CARTESIAN_POINT('Ctrl Pts',(-50.,12.562832359397,11.1690856668796));
#61362=CARTESIAN_POINT('Ctrl Pts',(-66.,12.5261370543444,11.0661765536716));
#61363=CARTESIAN_POINT('Ctrl Pts',(-50.,12.5261370543444,11.0661765536716));
#61364=CARTESIAN_POINT('Ctrl Pts',(-66.,12.488240282666,10.9641099236305));
#61365=CARTESIAN_POINT('Ctrl Pts',(-50.,12.488240282666,10.9641099236305));
#61366=CARTESIAN_POINT('Ctrl Pts',(-66.,12.4491367092919,10.8629121458916));
#61367=CARTESIAN_POINT('Ctrl Pts',(-50.,12.4491367092919,10.8629121458916));
#61368=CARTESIAN_POINT('Ctrl Pts',(-66.,12.4088000060691,10.7626331209311));
#61369=CARTESIAN_POINT('Ctrl Pts',(-50.,12.4088000060691,10.7626331209311));
#61370=CARTESIAN_POINT('Ctrl Pts',(-66.,12.3671719586111,10.6633568623205));
#61371=CARTESIAN_POINT('Ctrl Pts',(-50.,12.3671719586111,10.6633568623205));
#61372=CARTESIAN_POINT('Ctrl Pts',(-66.,12.3241773568055,10.5651848301937));
#61373=CARTESIAN_POINT('Ctrl Pts',(-50.,12.3241773568055,10.5651848301937));
#61374=CARTESIAN_POINT('Ctrl Pts',(-66.,12.2797452870059,10.4682125884904));
#61375=CARTESIAN_POINT('Ctrl Pts',(-50.,12.2797452870059,10.4682125884904));
#61376=CARTESIAN_POINT('Ctrl Pts',(-66.,12.2338301385431,10.3725066547111));
#61377=CARTESIAN_POINT('Ctrl Pts',(-50.,12.2338301385431,10.3725066547111));
#61378=CARTESIAN_POINT('Ctrl Pts',(-66.,12.1864291233458,10.2780853580389));
#61379=CARTESIAN_POINT('Ctrl Pts',(-50.,12.1864291233458,10.2780853580389));
#61380=CARTESIAN_POINT('Ctrl Pts',(-66.,12.1376115714812,10.1848864963973));
#61381=CARTESIAN_POINT('Ctrl Pts',(-50.,12.1376115714812,10.1848864963973));
#61382=CARTESIAN_POINT('Ctrl Pts',(-66.,12.0874846061232,10.0928063773702));
#61383=CARTESIAN_POINT('Ctrl Pts',(-50.,12.0874846061232,10.0928063773702));
#61384=CARTESIAN_POINT('Ctrl Pts',(-66.,12.0361378186387,10.0017624314164));
#61385=CARTESIAN_POINT('Ctrl Pts',(-50.,12.0361378186387,10.0017624314164));
#61386=CARTESIAN_POINT('Ctrl Pts',(-66.,11.9835915618855,9.91175181299999));
#61387=CARTESIAN_POINT('Ctrl Pts',(-50.,11.9835915618855,9.91175181299999));
#61388=CARTESIAN_POINT('Ctrl Pts',(-66.,11.9297512100749,9.82290332823825));
#61389=CARTESIAN_POINT('Ctrl Pts',(-50.,11.9297512100749,9.82290332823825));
#61390=CARTESIAN_POINT('Ctrl Pts',(-66.,11.8743389448017,9.73555464618448));
#61391=CARTESIAN_POINT('Ctrl Pts',(-50.,11.8743389448017,9.73555464618448));
#61392=CARTESIAN_POINT('Ctrl Pts',(-66.,11.8169531311064,9.65018619637799));
#61393=CARTESIAN_POINT('Ctrl Pts',(-50.,11.8169531311064,9.65018619637799));
#61394=CARTESIAN_POINT('Ctrl Pts',(-66.,11.7571708487241,9.56730656089267));
#61395=CARTESIAN_POINT('Ctrl Pts',(-50.,11.7571708487241,9.56730656089267));
#61396=CARTESIAN_POINT('Ctrl Pts',(-66.,11.6946398682888,9.48734988004618));
#61397=CARTESIAN_POINT('Ctrl Pts',(-50.,11.6946398682888,9.48734988004618));
#61398=CARTESIAN_POINT('Ctrl Pts',(-66.,11.629167237137,9.41057683066949));
#61399=CARTESIAN_POINT('Ctrl Pts',(-50.,11.629167237137,9.41057683066949));
#61400=CARTESIAN_POINT('Ctrl Pts',(-66.,11.5608318756571,9.3369493595236));
#61401=CARTESIAN_POINT('Ctrl Pts',(-50.,11.5608318756571,9.3369493595236));
#61402=CARTESIAN_POINT('Ctrl Pts',(-66.,11.4899314378663,9.26618715093123));
#61403=CARTESIAN_POINT('Ctrl Pts',(-50.,11.4899314378663,9.26618715093123));
#61404=CARTESIAN_POINT('Ctrl Pts',(-66.,11.4168866676366,9.19787074131628));
#61405=CARTESIAN_POINT('Ctrl Pts',(-50.,11.4168866676366,9.19787074131628));
#61406=CARTESIAN_POINT('Ctrl Pts',(-66.,11.3421599232118,9.13152900801114));
#61407=CARTESIAN_POINT('Ctrl Pts',(-50.,11.3421599232118,9.13152900801114));
#61408=CARTESIAN_POINT('Ctrl Pts',(-66.,11.2661714856319,9.06672919987649));
#61409=CARTESIAN_POINT('Ctrl Pts',(-50.,11.2661714856319,9.06672919987649));
#61410=CARTESIAN_POINT('Ctrl Pts',(-66.,11.1892087351483,9.00317437991606));
#61411=CARTESIAN_POINT('Ctrl Pts',(-50.,11.1892087351483,9.00317437991606));
#61412=CARTESIAN_POINT('Ctrl Pts',(-66.,11.1114442196238,8.9406855206164));
#61413=CARTESIAN_POINT('Ctrl Pts',(-50.,11.1114442196238,8.9406855206164));
#61414=CARTESIAN_POINT('Ctrl Pts',(-66.,11.0486622767737,8.89147286724882));
#61415=CARTESIAN_POINT('Ctrl Pts',(-50.,11.0486622767737,8.89147286724882));
#61416=CARTESIAN_POINT('Ctrl Pts',(-66.,11.0012690306593,8.85498631045878));
#61417=CARTESIAN_POINT('Ctrl Pts',(-50.,11.0012690306593,8.85498631045878));
#61418=CARTESIAN_POINT('Ctrl Pts',(-66.,10.9695373770028,8.83084964577152));
#61419=CARTESIAN_POINT('Ctrl Pts',(-50.,10.9695373770028,8.83084964577152));
#61420=CARTESIAN_POINT('Ctrl Pts',(-66.,10.9536375103364,8.81882824088047));
#61421=CARTESIAN_POINT('Ctrl Pts',(-50.,10.9536375103364,8.81882824088047));
#61422=CARTESIAN_POINT('Origin',(-65.75,0.,0.));
#61423=CARTESIAN_POINT('',(-65.5,14.9866834948009,7.75660639884882));
#61424=CARTESIAN_POINT('Origin',(-65.5,0.,0.));
#61425=CARTESIAN_POINT('Ctrl Pts',(-65.5,14.9866834948009,7.75660639884882));
#61426=CARTESIAN_POINT('Ctrl Pts',(-65.6931595476747,14.8653489329845,7.57080804606636));
#61427=CARTESIAN_POINT('Ctrl Pts',(-65.8611256967097,14.7547367322848,7.41690815510283));
#61428=CARTESIAN_POINT('Ctrl Pts',(-66.,14.66105681156,7.29342431017219));
#61429=CARTESIAN_POINT('Origin',(-58.,0.,0.));
#61430=CARTESIAN_POINT('',(-50.5,14.9866834948009,7.75660639884882));
#61431=CARTESIAN_POINT('Origin',(-50.5,0.,0.));
#61432=CARTESIAN_POINT('Ctrl Pts',(-50.5,14.9866834948009,7.75660639884881));
#61433=CARTESIAN_POINT('Ctrl Pts',(-55.5,14.9866834948009,7.75660639884881));
#61434=CARTESIAN_POINT('Ctrl Pts',(-60.5,14.9866834948009,7.75660639884881));
#61435=CARTESIAN_POINT('Ctrl Pts',(-65.5,14.9866834948009,7.75660639884881));
#61436=CARTESIAN_POINT('Origin',(-50.25,0.,0.));
#61437=CARTESIAN_POINT('Ctrl Pts',(-50.,14.66105681156,7.29342431017219));
#61438=CARTESIAN_POINT('Ctrl Pts',(-50.1388743032983,14.7547367322901,7.41690815510991));
#61439=CARTESIAN_POINT('Ctrl Pts',(-50.3068404523272,14.8653489329857,7.57080804606814));
#61440=CARTESIAN_POINT('Ctrl Pts',(-50.5,14.9866834948009,7.75660639884881));
#61441=CARTESIAN_POINT('Ctrl Pts',(-66.,13.3152354345065,4.52309756402217));
#61442=CARTESIAN_POINT('Ctrl Pts',(-50.,13.3152354345065,4.52309756402217));
#61443=CARTESIAN_POINT('Ctrl Pts',(-66.,13.3370379593182,4.53151803523741));
#61444=CARTESIAN_POINT('Ctrl Pts',(-50.,13.3370379593182,4.53151803523741));
#61445=CARTESIAN_POINT('Ctrl Pts',(-66.,13.3807325353144,4.54815245260096));
#61446=CARTESIAN_POINT('Ctrl Pts',(-50.,13.3807325353144,4.54815245260096));
#61447=CARTESIAN_POINT('Ctrl Pts',(-66.,13.4465429805744,4.57248451663122));
#61448=CARTESIAN_POINT('Ctrl Pts',(-50.,13.4465429805744,4.57248451663122));
#61449=CARTESIAN_POINT('Ctrl Pts',(-66.,13.5348280991712,4.60368638306948));
#61450=CARTESIAN_POINT('Ctrl Pts',(-50.,13.5348280991712,4.60368638306948));
#61451=CARTESIAN_POINT('Ctrl Pts',(-66.,13.6460849914764,4.64056367145667));
#61452=CARTESIAN_POINT('Ctrl Pts',(-50.,13.6460849914764,4.64056367145667));
#61453=CARTESIAN_POINT('Ctrl Pts',(-66.,13.7582469996088,4.67515954595839));
#61454=CARTESIAN_POINT('Ctrl Pts',(-50.,13.7582469996088,4.67515954595839));
#61455=CARTESIAN_POINT('Ctrl Pts',(-66.,13.8713185101153,4.70717714415409));
#61456=CARTESIAN_POINT('Ctrl Pts',(-50.,13.8713185101153,4.70717714415409));
#61457=CARTESIAN_POINT('Ctrl Pts',(-66.,13.9853001122203,4.73612262057495));
#61458=CARTESIAN_POINT('Ctrl Pts',(-50.,13.9853001122203,4.73612262057495));
#61459=CARTESIAN_POINT('Ctrl Pts',(-66.,14.1002130408447,4.76136787417443));
#61460=CARTESIAN_POINT('Ctrl Pts',(-50.,14.1002130408447,4.76136787417443));
#61461=CARTESIAN_POINT('Ctrl Pts',(-66.,14.2161348344847,4.78223175145606));
#61462=CARTESIAN_POINT('Ctrl Pts',(-50.,14.2161348344847,4.78223175145606));
#61463=CARTESIAN_POINT('Ctrl Pts',(-66.,14.3332199232164,4.79806029507722));
#61464=CARTESIAN_POINT('Ctrl Pts',(-50.,14.3332199232164,4.79806029507722));
#61465=CARTESIAN_POINT('Ctrl Pts',(-66.,14.4517548126435,4.80829403531135));
#61466=CARTESIAN_POINT('Ctrl Pts',(-50.,14.4517548126435,4.80829403531135));
#61467=CARTESIAN_POINT('Ctrl Pts',(-66.,14.5720437967212,4.81262902350044));
#61468=CARTESIAN_POINT('Ctrl Pts',(-50.,14.5720437967212,4.81262902350044));
#61469=CARTESIAN_POINT('Ctrl Pts',(-66.,14.6941876561096,4.81126607561379));
#61470=CARTESIAN_POINT('Ctrl Pts',(-50.,14.6941876561096,4.81126607561379));
#61471=CARTESIAN_POINT('Ctrl Pts',(-66.,14.8179374404009,4.80506713357809));
#61472=CARTESIAN_POINT('Ctrl Pts',(-50.,14.8179374404009,4.80506713357809));
#61473=CARTESIAN_POINT('Ctrl Pts',(-66.,14.9424160941388,4.79591343283465));
#61474=CARTESIAN_POINT('Ctrl Pts',(-50.,14.9424160941388,4.79591343283465));
#61475=CARTESIAN_POINT('Ctrl Pts',(-66.,15.0662673092696,4.78638101191027));
#61476=CARTESIAN_POINT('Ctrl Pts',(-50.,15.0662673092696,4.78638101191027));
#61477=CARTESIAN_POINT('Ctrl Pts',(-66.,15.1883575578327,4.77851428923771));
#61478=CARTESIAN_POINT('Ctrl Pts',(-50.,15.1883575578327,4.77851428923771));
#61479=CARTESIAN_POINT('Ctrl Pts',(-66.,15.3082818709966,4.77293091754137));
#61480=CARTESIAN_POINT('Ctrl Pts',(-50.,15.3082818709966,4.77293091754137));
#61481=CARTESIAN_POINT('Ctrl Pts',(-66.,15.4270758588568,4.76755908862997));
#61482=CARTESIAN_POINT('Ctrl Pts',(-50.,15.4270758588568,4.76755908862997));
#61483=CARTESIAN_POINT('Ctrl Pts',(-66.,15.5474780191768,4.75719646148653));
#61484=CARTESIAN_POINT('Ctrl Pts',(-50.,15.5474780191768,4.75719646148653));
#61485=CARTESIAN_POINT('Ctrl Pts',(-66.,15.6723955524765,4.73637240988335));
#61486=CARTESIAN_POINT('Ctrl Pts',(-50.,15.6723955524765,4.73637240988335));
#61487=CARTESIAN_POINT('Ctrl Pts',(-66.,15.8035951303885,4.70179750750619));
#61488=CARTESIAN_POINT('Ctrl Pts',(-50.,15.8035951303885,4.70179750750619));
#61489=CARTESIAN_POINT('Ctrl Pts',(-66.,15.9403656797971,4.65486242345584));
#61490=CARTESIAN_POINT('Ctrl Pts',(-50.,15.9403656797971,4.65486242345584));
#61491=CARTESIAN_POINT('Ctrl Pts',(-66.,16.0780101274447,4.60445942786333));
#61492=CARTESIAN_POINT('Ctrl Pts',(-50.,16.0780101274447,4.60445942786333));
#61493=CARTESIAN_POINT('Ctrl Pts',(-66.,16.208997020143,4.56481317811384));
#61494=CARTESIAN_POINT('Ctrl Pts',(-50.,16.208997020143,4.56481317811384));
#61495=CARTESIAN_POINT('Ctrl Pts',(-66.,16.3244271961989,4.55272063239585));
#61496=CARTESIAN_POINT('Ctrl Pts',(-50.,16.3244271961989,4.55272063239585));
#61497=CARTESIAN_POINT('Ctrl Pts',(-66.,16.4152805636122,4.5852041769408));
#61498=CARTESIAN_POINT('Ctrl Pts',(-50.,16.4152805636122,4.5852041769408));
#61499=CARTESIAN_POINT('Ctrl Pts',(-66.,16.4739900226401,4.67654967052486));
#61500=CARTESIAN_POINT('Ctrl Pts',(-50.,16.4739900226401,4.67654967052486));
#61501=CARTESIAN_POINT('Ctrl Pts',(-66.,16.4948644355662,4.83750989272408));
#61502=CARTESIAN_POINT('Ctrl Pts',(-50.,16.4948644355662,4.83750989272408));
#61503=CARTESIAN_POINT('Ctrl Pts',(-66.,16.473666674296,5.07609779098593));
#61504=CARTESIAN_POINT('Ctrl Pts',(-50.,16.473666674296,5.07609779098593));
#61505=CARTESIAN_POINT('Ctrl Pts',(-66.,16.4074477103004,5.39789810411011));
#61506=CARTESIAN_POINT('Ctrl Pts',(-50.,16.4074477103004,5.39789810411011));
#61507=CARTESIAN_POINT('Ctrl Pts',(-66.,16.2942876717617,5.80655413420453));
#61508=CARTESIAN_POINT('Ctrl Pts',(-50.,16.2942876717617,5.80655413420453));
#61509=CARTESIAN_POINT('Ctrl Pts',(-66.,16.1330883155878,6.30415788676021));
#61510=CARTESIAN_POINT('Ctrl Pts',(-50.,16.1330883155878,6.30415788676021));
#61511=CARTESIAN_POINT('Ctrl Pts',(-66.,15.9233539118341,6.89166211288976));
#61512=CARTESIAN_POINT('Ctrl Pts',(-50.,15.9233539118341,6.89166211288976));
#61513=CARTESIAN_POINT('Ctrl Pts',(-66.,15.7166600820928,7.43374456190315));
#61514=CARTESIAN_POINT('Ctrl Pts',(-50.,15.7166600820928,7.43374456190315));
#61515=CARTESIAN_POINT('Ctrl Pts',(-66.,15.5397988008428,7.88077212333004));
#61516=CARTESIAN_POINT('Ctrl Pts',(-50.,15.5397988008428,7.88077212333004));
#61517=CARTESIAN_POINT('Ctrl Pts',(-66.,15.412197120172,8.19675134334703));
#61518=CARTESIAN_POINT('Ctrl Pts',(-50.,15.412197120172,8.19675134334703));
#61519=CARTESIAN_POINT('Ctrl Pts',(-66.,15.3459727388094,8.35923116678319));
#61520=CARTESIAN_POINT('Ctrl Pts',(-50.,15.3459727388094,8.35923116678319));
#61521=CARTESIAN_POINT('',(-65.5,16.2457857930433,4.56509243789802));
#61522=CARTESIAN_POINT('Ctrl Pts',(-66.,15.6762335782098,4.73247565248983));
#61523=CARTESIAN_POINT('Ctrl Pts',(-65.7933280154031,15.90736217133,4.68197944667057));
#61524=CARTESIAN_POINT('Ctrl Pts',(-65.6370761749492,16.0983935063691,4.58291093022731));
#61525=CARTESIAN_POINT('Ctrl Pts',(-65.5,16.2457857930433,4.56509243789802));
#61526=CARTESIAN_POINT('',(-66.,13.3152354345065,4.52309756402217));
#61527=CARTESIAN_POINT('',(-50.5,16.2457857930433,4.56509243789802));
#61528=CARTESIAN_POINT('Ctrl Pts',(-50.5,16.2457857930433,4.56509243789802));
#61529=CARTESIAN_POINT('Ctrl Pts',(-50.4518618349122,16.1940248343557,4.57134990405274));
#61530=CARTESIAN_POINT('Ctrl Pts',(-50.4012423593884,16.1368929145766,4.58739650705545));
#61531=CARTESIAN_POINT('Ctrl Pts',(-50.2441129793799,15.9565712448129,4.64627335018861));
#61532=CARTESIAN_POINT('Ctrl Pts',(-50.1366827452942,15.8290907285646,4.69907993099531));
#61533=CARTESIAN_POINT('Ctrl Pts',(-50.,15.6762335782097,4.73247565248984));
#61534=CARTESIAN_POINT('Ctrl Pts',(-65.5,16.2457857930433,4.56509243789802));
#61535=CARTESIAN_POINT('Ctrl Pts',(-60.5,16.2457857930433,4.56509243789802));
#61536=CARTESIAN_POINT('Ctrl Pts',(-55.5,16.2457857930433,4.56509243789803));
#61537=CARTESIAN_POINT('Ctrl Pts',(-50.5,16.2457857930433,4.56509243789803));
#61538=CARTESIAN_POINT('Origin',(-66.,0.,0.));
#61539=CARTESIAN_POINT('',(-66.,12.8026622457696,5.81770965851215));
#61540=CARTESIAN_POINT('Ctrl Pts',(-66.,15.3459727388094,8.35923116678319));
#61541=CARTESIAN_POINT('Ctrl Pts',(-50.,15.3459727388094,8.35923116678319));
#61542=CARTESIAN_POINT('Ctrl Pts',(-66.,15.3352242315735,8.33945389776334));
#61543=CARTESIAN_POINT('Ctrl Pts',(-50.,15.3352242315735,8.33945389776334));
#61544=CARTESIAN_POINT('Ctrl Pts',(-66.,15.3136287101959,8.3000096293358));
#61545=CARTESIAN_POINT('Ctrl Pts',(-50.,15.3136287101959,8.3000096293358));
#61546=CARTESIAN_POINT('Ctrl Pts',(-66.,15.2809399078174,8.24117403498916));
#61547=CARTESIAN_POINT('Ctrl Pts',(-50.,15.2809399078174,8.24117403498916));
#61548=CARTESIAN_POINT('Ctrl Pts',(-66.,15.2367630078382,8.1633890770009));
#61549=CARTESIAN_POINT('Ctrl Pts',(-50.,15.2367630078382,8.1633890770009));
#61550=CARTESIAN_POINT('Ctrl Pts',(-66.,15.1805516924665,8.0672667757277));
#61551=CARTESIAN_POINT('Ctrl Pts',(-50.,15.1805516924665,8.0672667757277));
#61552=CARTESIAN_POINT('Ctrl Pts',(-66.,15.1233466491127,7.97225874547238));
#61553=CARTESIAN_POINT('Ctrl Pts',(-50.,15.1233466491127,7.97225874547238));
#61554=CARTESIAN_POINT('Ctrl Pts',(-66.,15.0651469569388,7.87836882722194));
#61555=CARTESIAN_POINT('Ctrl Pts',(-50.,15.0651469569388,7.87836882722194));
#61556=CARTESIAN_POINT('Ctrl Pts',(-66.,15.0059563925574,7.78559754307594));
#61557=CARTESIAN_POINT('Ctrl Pts',(-50.,15.0059563925574,7.78559754307594));
#61558=CARTESIAN_POINT('Ctrl Pts',(-66.,14.9457865336247,7.69393894021329));
#61559=CARTESIAN_POINT('Ctrl Pts',(-50.,14.9457865336247,7.69393894021329));
#61560=CARTESIAN_POINT('Ctrl Pts',(-66.,14.8846516233064,7.60338865730635));
#61561=CARTESIAN_POINT('Ctrl Pts',(-50.,14.8846516233064,7.60338865730635));
#61562=CARTESIAN_POINT('Ctrl Pts',(-66.,14.8225625096892,7.513953182008));
#61563=CARTESIAN_POINT('Ctrl Pts',(-50.,14.8225625096892,7.513953182008));
#61564=CARTESIAN_POINT('Ctrl Pts',(-66.,14.7595205830519,7.42565938179662));
#61565=CARTESIAN_POINT('Ctrl Pts',(-50.,14.7595205830519,7.42565938179662));
#61566=CARTESIAN_POINT('Ctrl Pts',(-66.,14.6955127521324,7.33856213697858));
#61567=CARTESIAN_POINT('Ctrl Pts',(-50.,14.6955127521324,7.33856213697858));
#61568=CARTESIAN_POINT('Ctrl Pts',(-66.,14.6305035247819,7.2527572990137));
#61569=CARTESIAN_POINT('Ctrl Pts',(-50.,14.6305035247819,7.2527572990137));
#61570=CARTESIAN_POINT('Ctrl Pts',(-66.,14.5644452858612,7.16836184447367));
#61571=CARTESIAN_POINT('Ctrl Pts',(-50.,14.5644452858612,7.16836184447367));
#61572=CARTESIAN_POINT('Ctrl Pts',(-66.,14.497293115392,7.08548597048793));
#61573=CARTESIAN_POINT('Ctrl Pts',(-50.,14.497293115392,7.08548597048793));
#61574=CARTESIAN_POINT('Ctrl Pts',(-66.,14.4290193778776,7.00420544769957));
#61575=CARTESIAN_POINT('Ctrl Pts',(-50.,14.4290193778776,7.00420544769957));
#61576=CARTESIAN_POINT('Ctrl Pts',(-66.,14.3596259311217,6.92453872281182));
#61577=CARTESIAN_POINT('Ctrl Pts',(-50.,14.3596259311217,6.92453872281182));
#61578=CARTESIAN_POINT('Ctrl Pts',(-66.,14.2891644580326,6.84640830625432));
#61579=CARTESIAN_POINT('Ctrl Pts',(-50.,14.2891644580326,6.84640830625432));
#61580=CARTESIAN_POINT('Ctrl Pts',(-66.,14.2177129290574,6.76968712284877));
#61581=CARTESIAN_POINT('Ctrl Pts',(-50.,14.2177129290574,6.76968712284877));
#61582=CARTESIAN_POINT('Ctrl Pts',(-66.,14.1453375866756,6.69427291666095));
#61583=CARTESIAN_POINT('Ctrl Pts',(-50.,14.1453375866756,6.69427291666095));
#61584=CARTESIAN_POINT('Ctrl Pts',(-66.,14.0720574366665,6.62015787000295));
#61585=CARTESIAN_POINT('Ctrl Pts',(-50.,14.0720574366665,6.62015787000295));
#61586=CARTESIAN_POINT('Ctrl Pts',(-66.,13.9978128588633,6.54749027478764));
#61587=CARTESIAN_POINT('Ctrl Pts',(-50.,13.9978128588633,6.54749027478764));
#61588=CARTESIAN_POINT('Ctrl Pts',(-66.,13.9224187379158,6.47666628220192));
#61589=CARTESIAN_POINT('Ctrl Pts',(-50.,13.9224187379158,6.47666628220192));
#61590=CARTESIAN_POINT('Ctrl Pts',(-66.,13.845605534933,6.40825111076043));
#61591=CARTESIAN_POINT('Ctrl Pts',(-50.,13.845605534933,6.40825111076043));
#61592=CARTESIAN_POINT('Ctrl Pts',(-66.,13.7670900956865,6.342842540489));
#61593=CARTESIAN_POINT('Ctrl Pts',(-50.,13.7670900956865,6.342842540489));
#61594=CARTESIAN_POINT('Ctrl Pts',(-66.,13.6866392230503,6.28094866827011));
#61595=CARTESIAN_POINT('Ctrl Pts',(-50.,13.6866392230503,6.28094866827011));
#61596=CARTESIAN_POINT('Ctrl Pts',(-66.,13.6041308540151,6.22286996666888));
#61597=CARTESIAN_POINT('Ctrl Pts',(-50.,13.6041308540151,6.22286996666888));
#61598=CARTESIAN_POINT('Ctrl Pts',(-66.,13.5196319660845,6.16854995125629));
#61599=CARTESIAN_POINT('Ctrl Pts',(-50.,13.5196319660845,6.16854995125629));
#61600=CARTESIAN_POINT('Ctrl Pts',(-66.,13.4333611502533,6.11764308944358));
#61601=CARTESIAN_POINT('Ctrl Pts',(-50.,13.4333611502533,6.11764308944358));
#61602=CARTESIAN_POINT('Ctrl Pts',(-66.,13.3456216156017,6.06963846112818));
#61603=CARTESIAN_POINT('Ctrl Pts',(-50.,13.3456216156017,6.06963846112818));
#61604=CARTESIAN_POINT('Ctrl Pts',(-66.,13.2567440310958,6.02396476100794));
#61605=CARTESIAN_POINT('Ctrl Pts',(-50.,13.2567440310958,6.02396476100794));
#61606=CARTESIAN_POINT('Ctrl Pts',(-66.,13.1670278530422,5.98009831397194));
#61607=CARTESIAN_POINT('Ctrl Pts',(-50.,13.1670278530422,5.98009831397194));
#61608=CARTESIAN_POINT('Ctrl Pts',(-66.,13.0766775878848,5.93768004328337));
#61609=CARTESIAN_POINT('Ctrl Pts',(-50.,13.0766775878848,5.93768004328337));
#61610=CARTESIAN_POINT('Ctrl Pts',(-66.,12.9858158402462,5.89649363499879));
#61611=CARTESIAN_POINT('Ctrl Pts',(-50.,12.9858158402462,5.89649363499879));
#61612=CARTESIAN_POINT('Ctrl Pts',(-66.,12.9127676183656,5.86444032191588));
#61613=CARTESIAN_POINT('Ctrl Pts',(-50.,12.9127676183656,5.86444032191588));
#61614=CARTESIAN_POINT('Ctrl Pts',(-66.,12.8577894805368,5.84088627843006));
#61615=CARTESIAN_POINT('Ctrl Pts',(-50.,12.8577894805368,5.84088627843006));
#61616=CARTESIAN_POINT('Ctrl Pts',(-66.,12.8210521907127,5.82539925281556));
#61617=CARTESIAN_POINT('Ctrl Pts',(-50.,12.8210521907127,5.82539925281556));
#61618=CARTESIAN_POINT('Ctrl Pts',(-66.,12.8026622457696,5.81770965851216));
#61619=CARTESIAN_POINT('Ctrl Pts',(-50.,12.8026622457696,5.81770965851216));
#61620=CARTESIAN_POINT('Origin',(-65.75,0.,0.));
#61621=CARTESIAN_POINT('',(-65.5,16.4448388443404,3.78588171813012));
#61622=CARTESIAN_POINT('Origin',(-65.5,0.,0.));
#61623=CARTESIAN_POINT('Ctrl Pts',(-65.5,16.4448388443404,3.78588171813013));
#61624=CARTESIAN_POINT('Ctrl Pts',(-65.6940750045237,16.2803340862868,3.63538534543884));
#61625=CARTESIAN_POINT('Ctrl Pts',(-65.8621879567711,16.1347706485061,3.51380187308767));
#61626=CARTESIAN_POINT('Ctrl Pts',(-66.,16.0142536207693,3.41823140961461));
#61627=CARTESIAN_POINT('Origin',(-58.,0.,0.));
#61628=CARTESIAN_POINT('',(-50.5,16.4448388443404,3.78588171813012));
#61629=CARTESIAN_POINT('Origin',(-50.5,0.,0.));
#61630=CARTESIAN_POINT('Ctrl Pts',(-50.5,16.4448388443404,3.78588171813013));
#61631=CARTESIAN_POINT('Ctrl Pts',(-55.5,16.4448388443404,3.78588171813013));
#61632=CARTESIAN_POINT('Ctrl Pts',(-60.5,16.4448388443404,3.78588171813012));
#61633=CARTESIAN_POINT('Ctrl Pts',(-65.5,16.4448388443404,3.78588171813012));
#61634=CARTESIAN_POINT('Origin',(-50.25,0.,0.));
#61635=CARTESIAN_POINT('Ctrl Pts',(-50.,16.0142536207693,3.41823140961462));
#61636=CARTESIAN_POINT('Ctrl Pts',(-50.1378120432265,16.134770648504,3.51380187308599));
#61637=CARTESIAN_POINT('Ctrl Pts',(-50.3059249954773,16.2803340862876,3.6353853454396));
#61638=CARTESIAN_POINT('Ctrl Pts',(-50.5,16.4448388443404,3.78588171813012));
#61639=CARTESIAN_POINT('Ctrl Pts',(-66.,14.0217614511585,1.06963173887291));
#61640=CARTESIAN_POINT('Ctrl Pts',(-50.,14.0217614511585,1.06963173887291));
#61641=CARTESIAN_POINT('Ctrl Pts',(-66.,14.0449730955977,1.07236559806543));
#61642=CARTESIAN_POINT('Ctrl Pts',(-50.,14.0449730955977,1.07236559806543));
#61643=CARTESIAN_POINT('Ctrl Pts',(-66.,14.0914317375174,1.07761101544474));
#61644=CARTESIAN_POINT('Ctrl Pts',(-50.,14.0914317375174,1.07761101544474));
#61645=CARTESIAN_POINT('Ctrl Pts',(-66.,14.1612257648809,1.08481225073396));
#61646=CARTESIAN_POINT('Ctrl Pts',(-50.,14.1612257648809,1.08481225073396));
#61647=CARTESIAN_POINT('Ctrl Pts',(-66.,14.2544968327758,1.09307823697967));
#61648=CARTESIAN_POINT('Ctrl Pts',(-50.,14.2544968327758,1.09307823697967));
#61649=CARTESIAN_POINT('Ctrl Pts',(-66.,14.3714293939101,1.1011284935459));
#61650=CARTESIAN_POINT('Ctrl Pts',(-50.,14.3714293939101,1.1011284935459));
#61651=CARTESIAN_POINT('Ctrl Pts',(-66.,14.4886712704316,1.10674391788617));
#61652=CARTESIAN_POINT('Ctrl Pts',(-50.,14.4886712704316,1.10674391788617));
#61653=CARTESIAN_POINT('Ctrl Pts',(-66.,14.6061528843942,1.10963588316888));
#61654=CARTESIAN_POINT('Ctrl Pts',(-50.,14.6061528843942,1.10963588316888));
#61655=CARTESIAN_POINT('Ctrl Pts',(-66.,14.7237519921366,1.10932591245462));
#61656=CARTESIAN_POINT('Ctrl Pts',(-50.,14.7237519921366,1.10932591245462));
#61657=CARTESIAN_POINT('Ctrl Pts',(-66.,14.8413329590673,1.10520035673609));
#61658=CARTESIAN_POINT('Ctrl Pts',(-50.,14.8413329590673,1.10520035673609));
#61659=CARTESIAN_POINT('Ctrl Pts',(-66.,14.9588014916819,1.09658017916666));
#61660=CARTESIAN_POINT('Ctrl Pts',(-50.,14.9588014916819,1.09658017916666));
#61661=CARTESIAN_POINT('Ctrl Pts',(-66.,15.0761445357738,1.08279356247792));
#61662=CARTESIAN_POINT('Ctrl Pts',(-50.,15.0761445357738,1.08279356247792));
#61663=CARTESIAN_POINT('Ctrl Pts',(-66.,15.1935004613832,1.06322736266735));
#61664=CARTESIAN_POINT('Ctrl Pts',(-50.,15.1935004613832,1.06322736266735));
#61665=CARTESIAN_POINT('Ctrl Pts',(-66.,15.3110884135537,1.03751150535353));
#61666=CARTESIAN_POINT('Ctrl Pts',(-50.,15.3110884135537,1.03751150535353));
#61667=CARTESIAN_POINT('Ctrl Pts',(-66.,15.4290559476364,1.00581543437186));
#61668=CARTESIAN_POINT('Ctrl Pts',(-50.,15.4290559476364,1.00581543437186));
#61669=CARTESIAN_POINT('Ctrl Pts',(-66.,15.5473762906989,0.969035923607179));
#61670=CARTESIAN_POINT('Ctrl Pts',(-50.,15.5473762906989,0.969035923607179));
#61671=CARTESIAN_POINT('Ctrl Pts',(-66.,15.6656677858244,0.929213220852553));
#61672=CARTESIAN_POINT('Ctrl Pts',(-50.,15.6656677858244,0.929213220852553));
#61673=CARTESIAN_POINT('Ctrl Pts',(-66.,15.7832573706013,0.889179733744299));
#61674=CARTESIAN_POINT('Ctrl Pts',(-50.,15.7832573706013,0.889179733744299));
#61675=CARTESIAN_POINT('Ctrl Pts',(-66.,15.8995555551237,0.851197548491309));
#61676=CARTESIAN_POINT('Ctrl Pts',(-50.,15.8995555551237,0.851197548491309));
#61677=CARTESIAN_POINT('Ctrl Pts',(-66.,16.014323697387,0.815965624774873));
#61678=CARTESIAN_POINT('Ctrl Pts',(-50.,16.014323697387,0.815965624774873));
#61679=CARTESIAN_POINT('Ctrl Pts',(-66.,16.1280496341459,0.78121969830999));
#61680=CARTESIAN_POINT('Ctrl Pts',(-50.,16.1280496341459,0.78121969830999));
#61681=CARTESIAN_POINT('Ctrl Pts',(-66.,16.2420920586203,0.741239832489433));
#61682=CARTESIAN_POINT('Ctrl Pts',(-50.,16.2420920586203,0.741239832489433));
#61683=CARTESIAN_POINT('Ctrl Pts',(-66.,16.3579063468606,0.690004279498882));
#61684=CARTESIAN_POINT('Ctrl Pts',(-50.,16.3579063468606,0.690004279498882));
#61685=CARTESIAN_POINT('Ctrl Pts',(-66.,16.4763856202025,0.623887603031702));
#61686=CARTESIAN_POINT('Ctrl Pts',(-50.,16.4763856202025,0.623887603031702));
#61687=CARTESIAN_POINT('Ctrl Pts',(-66.,16.5971869905414,0.544413618454469));
#61688=CARTESIAN_POINT('Ctrl Pts',(-50.,16.5971869905414,0.544413618454469));
#61689=CARTESIAN_POINT('Ctrl Pts',(-66.,16.717972369469,0.461363343498776));
#61690=CARTESIAN_POINT('Ctrl Pts',(-50.,16.717972369469,0.461363343498776));
#61691=CARTESIAN_POINT('Ctrl Pts',(-66.,16.8349844466884,0.390387538024311));
#61692=CARTESIAN_POINT('Ctrl Pts',(-50.,16.8349844466884,0.390387538024311));
#61693=CARTESIAN_POINT('Ctrl Pts',(-66.,16.9437808776721,0.349968584407931));
#61694=CARTESIAN_POINT('Ctrl Pts',(-50.,16.9437808776721,0.349968584407931));
#61695=CARTESIAN_POINT('Ctrl Pts',(-66.,17.0398582485081,0.358837284977383));
#61696=CARTESIAN_POINT('Ctrl Pts',(-50.,17.0398582485081,0.358837284977383));
#61697=CARTESIAN_POINT('Ctrl Pts',(-66.,17.119439942414,0.432712543166702));
#61698=CARTESIAN_POINT('Ctrl Pts',(-50.,17.119439942414,0.432712543166702));
#61699=CARTESIAN_POINT('Ctrl Pts',(-66.,17.1796877267693,0.583424648605184));
#61700=CARTESIAN_POINT('Ctrl Pts',(-50.,17.1796877267693,0.583424648605184));
#61701=CARTESIAN_POINT('Ctrl Pts',(-66.,17.2184903296471,0.819788538169111));
#61702=CARTESIAN_POINT('Ctrl Pts',(-50.,17.2184903296471,0.819788538169111));
#61703=CARTESIAN_POINT('Ctrl Pts',(-66.,17.234380239734,1.14794688939137));
#61704=CARTESIAN_POINT('Ctrl Pts',(-50.,17.234380239734,1.14794688939137));
#61705=CARTESIAN_POINT('Ctrl Pts',(-66.,17.2264039539062,1.57190599605025));
#61706=CARTESIAN_POINT('Ctrl Pts',(-50.,17.2264039539062,1.57190599605025));
#61707=CARTESIAN_POINT('Ctrl Pts',(-66.,17.1940179930072,2.09396526138803));
#61708=CARTESIAN_POINT('Ctrl Pts',(-50.,17.1940179930072,2.09396526138803));
#61709=CARTESIAN_POINT('Ctrl Pts',(-66.,17.1369791409271,2.71517078711311));
#61710=CARTESIAN_POINT('Ctrl Pts',(-50.,17.1369791409271,2.71517078711311));
#61711=CARTESIAN_POINT('Ctrl Pts',(-66.,17.0715894010097,3.29162538436688));
#61712=CARTESIAN_POINT('Ctrl Pts',(-50.,17.0715894010097,3.29162538436688));
#61713=CARTESIAN_POINT('Ctrl Pts',(-66.,17.0114557759461,3.76859236500326));
#61714=CARTESIAN_POINT('Ctrl Pts',(-50.,17.0114557759461,3.76859236500326));
#61715=CARTESIAN_POINT('Ctrl Pts',(-66.,16.9664437732891,4.10637776434634));
#61716=CARTESIAN_POINT('Ctrl Pts',(-50.,16.9664437732891,4.10637776434634));
#61717=CARTESIAN_POINT('Ctrl Pts',(-66.,16.942707041602,4.28022231927839));
#61718=CARTESIAN_POINT('Ctrl Pts',(-50.,16.942707041602,4.28022231927839));
#61719=CARTESIAN_POINT('',(-65.5,16.8706868817224,0.381509028567348));
#61720=CARTESIAN_POINT('Ctrl Pts',(-66.,16.3606547098013,0.685275467717999));
#61721=CARTESIAN_POINT('Ctrl Pts',(-65.7933280154031,16.5719640774255,0.578886349316897));
#61722=CARTESIAN_POINT('Ctrl Pts',(-65.6370761749493,16.7323564736163,0.435422691336213));
#61723=CARTESIAN_POINT('Ctrl Pts',(-65.5,16.8706868817224,0.381509028567346));
#61724=CARTESIAN_POINT('',(-66.,14.0217614511585,1.06963173887291));
#61725=CARTESIAN_POINT('',(-50.5,16.8706868817224,0.381509028567348));
#61726=CARTESIAN_POINT('Ctrl Pts',(-50.5,16.8706868817224,0.381509028567348));
#61727=CARTESIAN_POINT('Ctrl Pts',(-50.4879795588757,16.8585564547758,0.386236808645463));
#61728=CARTESIAN_POINT('Ctrl Pts',(-50.4758389600911,16.8462886142405,0.391627729214028));
#61729=CARTESIAN_POINT('Ctrl Pts',(-50.3319788807996,16.7007416155469,0.461359015551984));
#61730=CARTESIAN_POINT('Ctrl Pts',(-50.189657660532,16.5545679796152,0.587644860737737));
#61731=CARTESIAN_POINT('Ctrl Pts',(-50.,16.3606547098013,0.685275467717997));
#61732=CARTESIAN_POINT('Ctrl Pts',(-65.5,16.8706868817224,0.381509028567347));
#61733=CARTESIAN_POINT('Ctrl Pts',(-60.5,16.8706868817224,0.381509028567347));
#61734=CARTESIAN_POINT('Ctrl Pts',(-55.5,16.8706868817224,0.381509028567347));
#61735=CARTESIAN_POINT('Ctrl Pts',(-50.5,16.8706868817224,0.381509028567347));
#61736=CARTESIAN_POINT('Origin',(-66.,0.,0.));
#61737=CARTESIAN_POINT('',(-66.,13.847248627403,2.45104298226008));
#61738=CARTESIAN_POINT('Ctrl Pts',(-66.,16.942707041602,4.28022231927839));
#61739=CARTESIAN_POINT('Ctrl Pts',(-50.,16.942707041602,4.28022231927839));
#61740=CARTESIAN_POINT('Ctrl Pts',(-66.,16.9273778116851,4.26373943458434));
#61741=CARTESIAN_POINT('Ctrl Pts',(-50.,16.9273778116851,4.26373943458434));
#61742=CARTESIAN_POINT('Ctrl Pts',(-66.,16.8966513626585,4.23090496815705));
#61743=CARTESIAN_POINT('Ctrl Pts',(-50.,16.8966513626585,4.23090496815705));
#61744=CARTESIAN_POINT('Ctrl Pts',(-66.,16.8503577217978,4.18204717677295));
#61745=CARTESIAN_POINT('Ctrl Pts',(-50.,16.8503577217978,4.18204717677295));
#61746=CARTESIAN_POINT('Ctrl Pts',(-66.,16.7882243879419,4.11769232454756));
#61747=CARTESIAN_POINT('Ctrl Pts',(-50.,16.7882243879419,4.11769232454756));
#61748=CARTESIAN_POINT('Ctrl Pts',(-66.,16.7098744101503,4.03856906780257));
#61749=CARTESIAN_POINT('Ctrl Pts',(-50.,16.7098744101503,4.03856906780257));
#61750=CARTESIAN_POINT('Ctrl Pts',(-66.,16.6308390321023,3.96077220530218));
#61751=CARTESIAN_POINT('Ctrl Pts',(-50.,16.6308390321023,3.96077220530218));
#61752=CARTESIAN_POINT('Ctrl Pts',(-66.,16.5511183171041,3.88430568636484));
#61753=CARTESIAN_POINT('Ctrl Pts',(-50.,16.5511183171041,3.88430568636484));
#61754=CARTESIAN_POINT('Ctrl Pts',(-66.,16.4707160529602,3.80916907748197));
#61755=CARTESIAN_POINT('Ctrl Pts',(-50.,16.4707160529602,3.80916907748197));
#61756=CARTESIAN_POINT('Ctrl Pts',(-66.,16.3896419731869,3.73535373360533));
#61757=CARTESIAN_POINT('Ctrl Pts',(-50.,16.3896419731869,3.73535373360533));
#61758=CARTESIAN_POINT('Ctrl Pts',(-66.,16.3079087888565,3.66285188829513));
#61759=CARTESIAN_POINT('Ctrl Pts',(-50.,16.3079087888565,3.66285188829513));
#61760=CARTESIAN_POINT('Ctrl Pts',(-66.,16.2255286206571,3.59166712757322));
#61761=CARTESIAN_POINT('Ctrl Pts',(-50.,16.2255286206571,3.59166712757322));
#61762=CARTESIAN_POINT('Ctrl Pts',(-66.,16.1425094968592,3.52182512907851));
#61763=CARTESIAN_POINT('Ctrl Pts',(-50.,16.1425094968592,3.52182512907851));
#61764=CARTESIAN_POINT('Ctrl Pts',(-66.,16.058852385664,3.4533823046161));
#61765=CARTESIAN_POINT('Ctrl Pts',(-50.,16.058852385664,3.4533823046161));
#61766=CARTESIAN_POINT('Ctrl Pts',(-66.,15.9745467472627,3.38644032083441));
#61767=CARTESIAN_POINT('Ctrl Pts',(-50.,15.9745467472627,3.38644032083441));
#61768=CARTESIAN_POINT('Ctrl Pts',(-66.,15.8895755533235,3.32112432067463));
#61769=CARTESIAN_POINT('Ctrl Pts',(-50.,15.8895755533235,3.32112432067463));
#61770=CARTESIAN_POINT('Ctrl Pts',(-66.,15.8039227000236,3.2575522103651));
#61771=CARTESIAN_POINT('Ctrl Pts',(-50.,15.8039227000236,3.2575522103651));
#61772=CARTESIAN_POINT('Ctrl Pts',(-66.,15.7175802634788,3.19580425274334));
#61773=CARTESIAN_POINT('Ctrl Pts',(-50.,15.7175802634788,3.19580425274334));
#61774=CARTESIAN_POINT('Ctrl Pts',(-66.,15.6305546306352,3.13589785295852));
#61775=CARTESIAN_POINT('Ctrl Pts',(-50.,15.6305546306352,3.13589785295852));
#61776=CARTESIAN_POINT('Ctrl Pts',(-66.,15.542876589815,3.07774510290095));
#61777=CARTESIAN_POINT('Ctrl Pts',(-50.,15.542876589815,3.07774510290095));
#61778=CARTESIAN_POINT('Ctrl Pts',(-66.,15.4545900595684,3.02120352923108));
#61779=CARTESIAN_POINT('Ctrl Pts',(-50.,15.4545900595684,3.02120352923108));
#61780=CARTESIAN_POINT('Ctrl Pts',(-66.,15.3657337712291,2.96615761473811));
#61781=CARTESIAN_POINT('Ctrl Pts',(-50.,15.3657337712291,2.96615761473811));
#61782=CARTESIAN_POINT('Ctrl Pts',(-66.,15.2763241892947,2.9125950607961));
#61783=CARTESIAN_POINT('Ctrl Pts',(-50.,15.2763241892947,2.9125950607961));
#61784=CARTESIAN_POINT('Ctrl Pts',(-66.,15.1863404453747,2.86067432738731));
#61785=CARTESIAN_POINT('Ctrl Pts',(-50.,15.1863404453747,2.86067432738731));
#61786=CARTESIAN_POINT('Ctrl Pts',(-66.,15.0957017586521,2.81082515619622));
#61787=CARTESIAN_POINT('Ctrl Pts',(-50.,15.0957017586521,2.81082515619622));
#61788=CARTESIAN_POINT('Ctrl Pts',(-66.,15.0042876224246,2.76366203995482));
#61789=CARTESIAN_POINT('Ctrl Pts',(-50.,15.0042876224246,2.76366203995482));
#61790=CARTESIAN_POINT('Ctrl Pts',(-66.,14.9119724401214,2.71983439592332));
#61791=CARTESIAN_POINT('Ctrl Pts',(-50.,14.9119724401214,2.71983439592332));
#61792=CARTESIAN_POINT('Ctrl Pts',(-66.,14.8186566994895,2.67989235195328));
#61793=CARTESIAN_POINT('Ctrl Pts',(-50.,14.8186566994895,2.67989235195328));
#61794=CARTESIAN_POINT('Ctrl Pts',(-66.,14.7242968968419,2.64415729654763));
#61795=CARTESIAN_POINT('Ctrl Pts',(-50.,14.7242968968419,2.64415729654763));
#61796=CARTESIAN_POINT('Ctrl Pts',(-66.,14.6289438583545,2.61255786321175));
#61797=CARTESIAN_POINT('Ctrl Pts',(-50.,14.6289438583545,2.61255786321175));
#61798=CARTESIAN_POINT('Ctrl Pts',(-66.,14.5327233771235,2.58470501352874));
#61799=CARTESIAN_POINT('Ctrl Pts',(-50.,14.5327233771235,2.58470501352874));
#61800=CARTESIAN_POINT('Ctrl Pts',(-66.,14.4358020756955,2.56002847385863));
#61801=CARTESIAN_POINT('Ctrl Pts',(-50.,14.4358020756955,2.56002847385863));
#61802=CARTESIAN_POINT('Ctrl Pts',(-66.,14.338358156612,2.53789265347798));
#61803=CARTESIAN_POINT('Ctrl Pts',(-50.,14.338358156612,2.53789265347798));
#61804=CARTESIAN_POINT('Ctrl Pts',(-66.,14.2405514355047,2.51771585773738));
#61805=CARTESIAN_POINT('Ctrl Pts',(-50.,14.2405514355047,2.51771585773738));
#61806=CARTESIAN_POINT('Ctrl Pts',(-66.,14.1424906951186,2.49909943227153));
#61807=CARTESIAN_POINT('Ctrl Pts',(-50.,14.1424906951186,2.49909943227153));
#61808=CARTESIAN_POINT('Ctrl Pts',(-66.,14.0442408931361,2.48180336850756));
#61809=CARTESIAN_POINT('Ctrl Pts',(-50.,14.0442408931361,2.48180336850756));
#61810=CARTESIAN_POINT('Ctrl Pts',(-66.,13.9655162806582,2.46892342325417));
#61811=CARTESIAN_POINT('Ctrl Pts',(-50.,13.9655162806582,2.46892342325417));
#61812=CARTESIAN_POINT('Ctrl Pts',(-66.,13.9064077297103,2.45978188025048));
#61813=CARTESIAN_POINT('Ctrl Pts',(-50.,13.9064077297103,2.45978188025048));
#61814=CARTESIAN_POINT('Ctrl Pts',(-66.,13.8669731427486,2.45391760048539));
#61815=CARTESIAN_POINT('Ctrl Pts',(-50.,13.8669731427486,2.45391760048539));
#61816=CARTESIAN_POINT('Ctrl Pts',(-66.,13.847248627403,2.45104298226009));
#61817=CARTESIAN_POINT('Ctrl Pts',(-50.,13.847248627403,2.45104298226009));
#61818=CARTESIAN_POINT('Origin',(-65.75,0.,0.));
#61819=CARTESIAN_POINT('Origin',(-65.5,0.,0.));
#61820=CARTESIAN_POINT('Origin',(-58.,0.,0.));
#61821=CARTESIAN_POINT('Origin',(-50.5,0.,0.));
#61822=CARTESIAN_POINT('Origin',(-50.25,0.,0.));
#61823=CARTESIAN_POINT('Origin',(-35.75,0.,0.));
#61824=CARTESIAN_POINT('Origin',(-21.5,0.,0.));
#61825=CARTESIAN_POINT('Origin',(-21.25,0.,0.));
#65541=UNCERTAINTY_MEASURE_WITH_UNIT(LENGTH_MEASURE(0.01),#65564,
'DISTANCE_ACCURACY_VALUE',
'Maximum model space distance between geometric entities at asserted c
onnectivities');
#65550=UNCERTAINTY_MEASURE_WITH_UNIT(LENGTH_MEASURE(0.01),#65564,
'DISTANCE_ACCURACY_VALUE',
'Maximum model space distance between geometric entities at asserted c
onnectivities');
#65554=(
GEOMETRIC_REPRESENTATION_CONTEXT(3)
GLOBAL_UNCERTAINTY_ASSIGNED_CONTEXT((#65541))
GLOBAL_UNIT_ASSIGNED_CONTEXT((#65564,#65566,#65567))
REPRESENTATION_CONTEXT('','3D')
);
#65563=(
GEOMETRIC_REPRESENTATION_CONTEXT(3)
GLOBAL_UNCERTAINTY_ASSIGNED_CONTEXT((#65550))
GLOBAL_UNIT_ASSIGNED_CONTEXT((#65564,#65566,#65567))
REPRESENTATION_CONTEXT('','3D')
);
#65564=(
LENGTH_UNIT()
NAMED_UNIT(*)
SI_UNIT(.MILLI.,.METRE.)
);
#65566=(
NAMED_UNIT(*)
PLANE_ANGLE_UNIT()
SI_UNIT($,.RADIAN.)
);
#65567=(
NAMED_UNIT(*)
SI_UNIT($,.STERADIAN.)
SOLID_ANGLE_UNIT()
);
#65571=SHAPE_DEFINITION_REPRESENTATION(#65583,#65616);
#65583=PRODUCT_DEFINITION_SHAPE('',$,#65629);
#65616=SHAPE_REPRESENTATION('',(#21298),#65554);
#65625=PRODUCT_DEFINITION_CONTEXT('part definition',#65663,'design');
#65629=PRODUCT_DEFINITION('2026-10-10-05-45-24-894',
'03_Compound_Planet_Pinion_Z25-Z14_M1.25',#65641,#65625);
#65641=PRODUCT_DEFINITION_FORMATION('',$,#65668);
#65663=APPLICATION_CONTEXT(
'Core Data for Automotive Mechanical Design Process');
#65664=PRODUCT_CONTEXT('part definition',#65663,'mechanical');
#65668=PRODUCT('2026-10-10-05-45-24-894',
'03_Compound_Planet_Pinion_Z25-Z14_M1.25',$,(#65664));
#65796=COLOUR_RGB('Off White',0.89,0.88,0.83);
#65797=FILL_AREA_STYLE_COLOUR('',#65796);
#65798=FILL_AREA_STYLE('',(#65797));
#65799=SURFACE_STYLE_FILL_AREA(#65798);
#65800=SURFACE_SIDE_STYLE('',(#65799));
#65801=SURFACE_STYLE_USAGE(.BOTH.,#65800);
#65802=PRESENTATION_STYLE_ASSIGNMENT((#65801));
ENDSEC;
END-ISO-10303-21;
